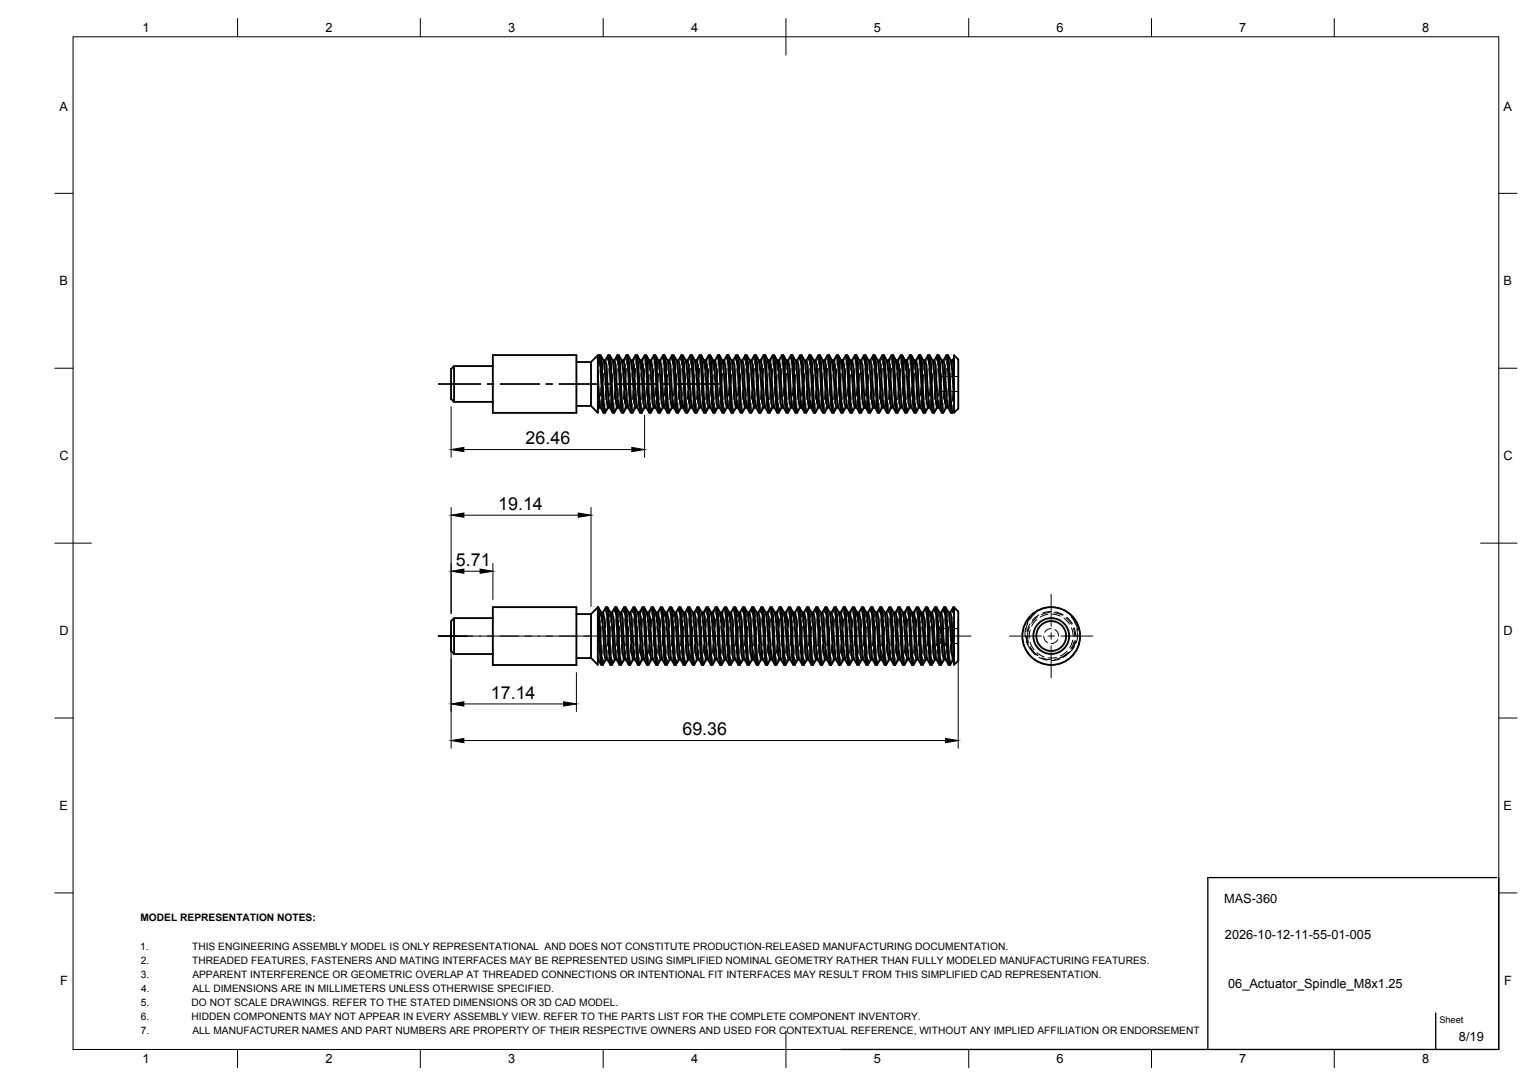
ISO-10303-21;
HEADER;
/* Generated by software containing ST-Developer
 * from STEP Tools, Inc. (www.steptools.com) 
 */

FILE_DESCRIPTION(
/* description */ (''),
/* implementation_level */ '2;1');

FILE_NAME(
/* name */ '06_Actuator_Spindle_M8x1.25.step',
/* time_stamp */ '2026-11-04T18:53:29-08:00',
/* author */ (''),
/* organization */ (''),
/* preprocessor_version */ 'ST-DEVELOPER v20.2',
/* originating_system */ 'Autodesk Translation Framework v15.17.0.0',
/* authorisation */ '');

FILE_SCHEMA (('AUTOMOTIVE_DESIGN { 1 0 10303 214 3 1 1 }'));
ENDSEC;

DATA;
#10=MECHANICAL_DESIGN_GEOMETRIC_PRESENTATION_REPRESENTATION('',(#1332),#100031);
#232=CONICAL_SURFACE('',#21595,3.6736,0.785398163397448);
#233=CONICAL_SURFACE('',#21596,3.5,0.78539816339745);
#234=CONICAL_SURFACE('',#21608,2.244,0.785398163397449);
#784=CIRCLE('',#21539,3.22275);
#785=CIRCLE('',#21579,3.933);
#786=CIRCLE('',#21580,3.933);
#787=CIRCLE('',#21582,3.22275);
#788=CIRCLE('',#21584,1.02);
#789=CIRCLE('',#21585,1.02);
#790=CIRCLE('',#21588,3.933);
#791=CIRCLE('',#21589,3.933);
#792=CIRCLE('',#21591,3.933);
#793=CIRCLE('',#21592,3.933);
#794=CIRCLE('',#21594,3.3472);
#795=CIRCLE('',#21597,3.);
#796=CIRCLE('',#21599,3.);
#797=CIRCLE('',#21601,3.95);
#798=CIRCLE('',#21603,3.95);
#799=CIRCLE('',#21605,2.448);
#800=CIRCLE('',#21607,2.448);
#801=CIRCLE('',#21609,2.04);
#1296=SHAPE_REPRESENTATION_RELATIONSHIP('SRR','None',#100106,#1314);
#1314=ADVANCED_BREP_SHAPE_REPRESENTATION('',(#1350),#100018);
#1332=STYLED_ITEM('',(#100200),#1350);
#1350=MANIFOLD_SOLID_BREP('Body1',#20122);
#1522=PLANE('',#21586);
#1523=PLANE('',#21587);
#1524=PLANE('',#21590);
#1525=PLANE('',#21593);
#1526=PLANE('',#21600);
#1527=PLANE('',#21604);
#1528=PLANE('',#21610);
#1757=FACE_BOUND('',#6951,.T.);
#1758=FACE_BOUND('',#6956,.T.);
#1759=FACE_BOUND('',#6959,.T.);
#2740=LINE('',#61994,#4027);
#2741=LINE('',#62177,#4028);
#2742=LINE('',#62607,#4029);
#2743=LINE('',#63034,#4030);
#2744=LINE('',#63490,#4031);
#2745=LINE('',#63954,#4032);
#2746=LINE('',#64297,#4033);
#2747=LINE('',#64695,#4034);
#2748=LINE('',#65028,#4035);
#2749=LINE('',#65420,#4036);
#2750=LINE('',#65803,#4037);
#2751=LINE('',#66202,#4038);
#2752=LINE('',#66758,#4039);
#2753=LINE('',#67219,#4040);
#2754=LINE('',#67749,#4041);
#2755=LINE('',#68202,#4042);
#2756=LINE('',#68741,#4043);
#2757=LINE('',#69203,#4044);
#2758=LINE('',#69714,#4045);
#2759=LINE('',#70197,#4046);
#2760=LINE('',#70661,#4047);
#2761=LINE('',#71128,#4048);
#2762=LINE('',#71592,#4049);
#2763=LINE('',#72044,#4050);
#2764=LINE('',#72530,#4051);
#2765=LINE('',#72983,#4052);
#2766=LINE('',#73456,#4053);
#2767=LINE('',#73924,#4054);
#2768=LINE('',#74396,#4055);
#2769=LINE('',#74858,#4056);
#2770=LINE('',#75318,#4057);
#2771=LINE('',#75804,#4058);
#2772=LINE('',#76261,#4059);
#2773=LINE('',#76732,#4060);
#2774=LINE('',#77194,#4061);
#2775=LINE('',#77655,#4062);
#2776=LINE('',#78092,#4063);
#2777=LINE('',#78388,#4064);
#2778=LINE('',#78748,#4065);
#2779=LINE('',#88562,#4066);
#2780=LINE('',#90954,#4067);
#2781=LINE('',#90957,#4068);
#2782=LINE('',#90962,#4069);
#2783=LINE('',#90969,#4070);
#2784=LINE('',#90976,#4071);
#2785=LINE('',#90979,#4072);
#4027=VECTOR('',#25695,3.22275);
#4028=VECTOR('',#25700,3.22275);
#4029=VECTOR('',#25703,3.22275);
#4030=VECTOR('',#25706,3.22275);
#4031=VECTOR('',#25709,3.22275);
#4032=VECTOR('',#25712,3.22275);
#4033=VECTOR('',#25715,3.22275);
#4034=VECTOR('',#25718,3.22275);
#4035=VECTOR('',#25721,3.22275);
#4036=VECTOR('',#25724,3.22275);
#4037=VECTOR('',#25727,3.22275);
#4038=VECTOR('',#25730,3.22275);
#4039=VECTOR('',#25733,3.22275);
#4040=VECTOR('',#25736,3.22275);
#4041=VECTOR('',#25739,3.22275);
#4042=VECTOR('',#25742,3.22275);
#4043=VECTOR('',#25745,3.22275);
#4044=VECTOR('',#25748,3.22275);
#4045=VECTOR('',#25751,3.22275);
#4046=VECTOR('',#25754,3.22275);
#4047=VECTOR('',#25757,3.22275);
#4048=VECTOR('',#25760,3.22275);
#4049=VECTOR('',#25763,3.22275);
#4050=VECTOR('',#25766,3.22275);
#4051=VECTOR('',#25769,3.22275);
#4052=VECTOR('',#25772,3.22275);
#4053=VECTOR('',#25775,3.22275);
#4054=VECTOR('',#25778,3.22275);
#4055=VECTOR('',#25781,3.22275);
#4056=VECTOR('',#25784,3.22275);
#4057=VECTOR('',#25787,3.22275);
#4058=VECTOR('',#25790,3.22275);
#4059=VECTOR('',#25793,3.22275);
#4060=VECTOR('',#25796,3.22275);
#4061=VECTOR('',#25799,3.22275);
#4062=VECTOR('',#25802,3.22275);
#4063=VECTOR('',#25805,3.22275);
#4064=VECTOR('',#25808,3.22275);
#4065=VECTOR('',#25811,3.22275);
#4066=VECTOR('',#25826,1.02);
#4067=VECTOR('',#25849,3.6736);
#4068=VECTOR('',#25852,3.5);
#4069=VECTOR('',#25859,3.);
#4070=VECTOR('',#25868,3.95);
#4071=VECTOR('',#25877,2.448);
#4072=VECTOR('',#25880,2.244);
#4817=CYLINDRICAL_SURFACE('',#21538,3.22275);
#4818=CYLINDRICAL_SURFACE('',#21540,3.22275);
#4819=CYLINDRICAL_SURFACE('',#21541,3.22275);
#4820=CYLINDRICAL_SURFACE('',#21542,3.22275);
#4821=CYLINDRICAL_SURFACE('',#21543,3.22275);
#4822=CYLINDRICAL_SURFACE('',#21544,3.22275);
#4823=CYLINDRICAL_SURFACE('',#21545,3.22275);
#4824=CYLINDRICAL_SURFACE('',#21546,3.22275);
#4825=CYLINDRICAL_SURFACE('',#21547,3.22275);
#4826=CYLINDRICAL_SURFACE('',#21548,3.22275);
#4827=CYLINDRICAL_SURFACE('',#21549,3.22275);
#4828=CYLINDRICAL_SURFACE('',#21550,3.22275);
#4829=CYLINDRICAL_SURFACE('',#21551,3.22275);
#4830=CYLINDRICAL_SURFACE('',#21552,3.22275);
#4831=CYLINDRICAL_SURFACE('',#21553,3.22275);
#4832=CYLINDRICAL_SURFACE('',#21554,3.22275);
#4833=CYLINDRICAL_SURFACE('',#21555,3.22275);
#4834=CYLINDRICAL_SURFACE('',#21556,3.22275);
#4835=CYLINDRICAL_SURFACE('',#21557,3.22275);
#4836=CYLINDRICAL_SURFACE('',#21558,3.22275);
#4837=CYLINDRICAL_SURFACE('',#21559,3.22275);
#4838=CYLINDRICAL_SURFACE('',#21560,3.22275);
#4839=CYLINDRICAL_SURFACE('',#21561,3.22275);
#4840=CYLINDRICAL_SURFACE('',#21562,3.22275);
#4841=CYLINDRICAL_SURFACE('',#21563,3.22275);
#4842=CYLINDRICAL_SURFACE('',#21564,3.22275);
#4843=CYLINDRICAL_SURFACE('',#21565,3.22275);
#4844=CYLINDRICAL_SURFACE('',#21566,3.22275);
#4845=CYLINDRICAL_SURFACE('',#21567,3.22275);
#4846=CYLINDRICAL_SURFACE('',#21568,3.22275);
#4847=CYLINDRICAL_SURFACE('',#21569,3.22275);
#4848=CYLINDRICAL_SURFACE('',#21570,3.22275);
#4849=CYLINDRICAL_SURFACE('',#21571,3.22275);
#4850=CYLINDRICAL_SURFACE('',#21572,3.22275);
#4851=CYLINDRICAL_SURFACE('',#21573,3.22275);
#4852=CYLINDRICAL_SURFACE('',#21574,3.22275);
#4853=CYLINDRICAL_SURFACE('',#21575,3.22275);
#4854=CYLINDRICAL_SURFACE('',#21576,3.22275);
#4855=CYLINDRICAL_SURFACE('',#21577,3.22275);
#4856=CYLINDRICAL_SURFACE('',#21578,3.933);
#4857=CYLINDRICAL_SURFACE('',#21581,3.22275);
#4858=CYLINDRICAL_SURFACE('',#21583,1.02);
#4859=CYLINDRICAL_SURFACE('',#21598,3.);
#4860=CYLINDRICAL_SURFACE('',#21602,3.95);
#4861=CYLINDRICAL_SURFACE('',#21606,2.448);
#5683=FACE_OUTER_BOUND('',#6903,.T.);
#5684=FACE_OUTER_BOUND('',#6904,.T.);
#5685=FACE_OUTER_BOUND('',#6905,.T.);
#5686=FACE_OUTER_BOUND('',#6906,.T.);
#5687=FACE_OUTER_BOUND('',#6907,.T.);
#5688=FACE_OUTER_BOUND('',#6908,.T.);
#5689=FACE_OUTER_BOUND('',#6909,.T.);
#5690=FACE_OUTER_BOUND('',#6910,.T.);
#5691=FACE_OUTER_BOUND('',#6911,.T.);
#5692=FACE_OUTER_BOUND('',#6912,.T.);
#5693=FACE_OUTER_BOUND('',#6913,.T.);
#5694=FACE_OUTER_BOUND('',#6914,.T.);
#5695=FACE_OUTER_BOUND('',#6915,.T.);
#5696=FACE_OUTER_BOUND('',#6916,.T.);
#5697=FACE_OUTER_BOUND('',#6917,.T.);
#5698=FACE_OUTER_BOUND('',#6918,.T.);
#5699=FACE_OUTER_BOUND('',#6919,.T.);
#5700=FACE_OUTER_BOUND('',#6920,.T.);
#5701=FACE_OUTER_BOUND('',#6921,.T.);
#5702=FACE_OUTER_BOUND('',#6922,.T.);
#5703=FACE_OUTER_BOUND('',#6923,.T.);
#5704=FACE_OUTER_BOUND('',#6924,.T.);
#5705=FACE_OUTER_BOUND('',#6925,.T.);
#5706=FACE_OUTER_BOUND('',#6926,.T.);
#5707=FACE_OUTER_BOUND('',#6927,.T.);
#5708=FACE_OUTER_BOUND('',#6928,.T.);
#5709=FACE_OUTER_BOUND('',#6929,.T.);
#5710=FACE_OUTER_BOUND('',#6930,.T.);
#5711=FACE_OUTER_BOUND('',#6931,.T.);
#5712=FACE_OUTER_BOUND('',#6932,.T.);
#5713=FACE_OUTER_BOUND('',#6933,.T.);
#5714=FACE_OUTER_BOUND('',#6934,.T.);
#5715=FACE_OUTER_BOUND('',#6935,.T.);
#5716=FACE_OUTER_BOUND('',#6936,.T.);
#5717=FACE_OUTER_BOUND('',#6937,.T.);
#5718=FACE_OUTER_BOUND('',#6938,.T.);
#5719=FACE_OUTER_BOUND('',#6939,.T.);
#5720=FACE_OUTER_BOUND('',#6940,.T.);
#5721=FACE_OUTER_BOUND('',#6941,.T.);
#5722=FACE_OUTER_BOUND('',#6942,.T.);
#5723=FACE_OUTER_BOUND('',#6943,.T.);
#5724=FACE_OUTER_BOUND('',#6944,.T.);
#5725=FACE_OUTER_BOUND('',#6945,.T.);
#5726=FACE_OUTER_BOUND('',#6946,.T.);
#5727=FACE_OUTER_BOUND('',#6947,.T.);
#5728=FACE_OUTER_BOUND('',#6948,.T.);
#5729=FACE_OUTER_BOUND('',#6949,.T.);
#5730=FACE_OUTER_BOUND('',#6950,.T.);
#5731=FACE_OUTER_BOUND('',#6952,.T.);
#5732=FACE_OUTER_BOUND('',#6953,.T.);
#5733=FACE_OUTER_BOUND('',#6954,.T.);
#5734=FACE_OUTER_BOUND('',#6955,.T.);
#5735=FACE_OUTER_BOUND('',#6957,.T.);
#5736=FACE_OUTER_BOUND('',#6958,.T.);
#5737=FACE_OUTER_BOUND('',#6960,.T.);
#5738=FACE_OUTER_BOUND('',#6961,.T.);
#5739=FACE_OUTER_BOUND('',#6962,.T.);
#6903=EDGE_LOOP('',(#16151,#16152,#16153,#16154));
#6904=EDGE_LOOP('',(#16155,#16156,#16157,#16158,#16159,#16160));
#6905=EDGE_LOOP('',(#16161,#16162,#16163,#16164,#16165,#16166));
#6906=EDGE_LOOP('',(#16167,#16168,#16169,#16170,#16171,#16172));
#6907=EDGE_LOOP('',(#16173,#16174,#16175,#16176,#16177));
#6908=EDGE_LOOP('',(#16178,#16179,#16180,#16181,#16182,#16183));
#6909=EDGE_LOOP('',(#16184,#16185,#16186,#16187,#16188));
#6910=EDGE_LOOP('',(#16189,#16190,#16191,#16192,#16193,#16194));
#6911=EDGE_LOOP('',(#16195,#16196,#16197,#16198,#16199));
#6912=EDGE_LOOP('',(#16200,#16201,#16202,#16203,#16204,#16205));
#6913=EDGE_LOOP('',(#16206,#16207,#16208,#16209,#16210));
#6914=EDGE_LOOP('',(#16211,#16212,#16213,#16214,#16215,#16216));
#6915=EDGE_LOOP('',(#16217,#16218,#16219,#16220,#16221));
#6916=EDGE_LOOP('',(#16222,#16223,#16224,#16225,#16226,#16227));
#6917=EDGE_LOOP('',(#16228,#16229,#16230,#16231,#16232));
#6918=EDGE_LOOP('',(#16233,#16234,#16235,#16236,#16237,#16238));
#6919=EDGE_LOOP('',(#16239,#16240,#16241,#16242,#16243));
#6920=EDGE_LOOP('',(#16244,#16245,#16246,#16247,#16248,#16249));
#6921=EDGE_LOOP('',(#16250,#16251,#16252,#16253,#16254));
#6922=EDGE_LOOP('',(#16255,#16256,#16257,#16258,#16259,#16260));
#6923=EDGE_LOOP('',(#16261,#16262,#16263,#16264,#16265));
#6924=EDGE_LOOP('',(#16266,#16267,#16268,#16269,#16270,#16271));
#6925=EDGE_LOOP('',(#16272,#16273,#16274,#16275,#16276));
#6926=EDGE_LOOP('',(#16277,#16278,#16279,#16280,#16281,#16282));
#6927=EDGE_LOOP('',(#16283,#16284,#16285,#16286,#16287,#16288));
#6928=EDGE_LOOP('',(#16289,#16290,#16291,#16292,#16293));
#6929=EDGE_LOOP('',(#16294,#16295,#16296,#16297,#16298,#16299));
#6930=EDGE_LOOP('',(#16300,#16301,#16302,#16303,#16304));
#6931=EDGE_LOOP('',(#16305,#16306,#16307,#16308,#16309,#16310));
#6932=EDGE_LOOP('',(#16311,#16312,#16313,#16314,#16315));
#6933=EDGE_LOOP('',(#16316,#16317,#16318,#16319,#16320,#16321));
#6934=EDGE_LOOP('',(#16322,#16323,#16324,#16325,#16326,#16327));
#6935=EDGE_LOOP('',(#16328,#16329,#16330,#16331,#16332));
#6936=EDGE_LOOP('',(#16333,#16334,#16335,#16336,#16337,#16338));
#6937=EDGE_LOOP('',(#16339,#16340,#16341,#16342,#16343));
#6938=EDGE_LOOP('',(#16344,#16345,#16346,#16347,#16348,#16349));
#6939=EDGE_LOOP('',(#16350,#16351,#16352,#16353,#16354,#16355));
#6940=EDGE_LOOP('',(#16356,#16357,#16358,#16359,#16360,#16361));
#6941=EDGE_LOOP('',(#16362,#16363,#16364,#16365,#16366,#16367));
#6942=EDGE_LOOP('',(#16368,#16369,#16370,#16371,#16372,#16373,#16374,#16375,
#16376,#16377,#16378,#16379,#16380,#16381,#16382,#16383,#16384,#16385,#16386,
#16387,#16388,#16389,#16390,#16391,#16392,#16393,#16394,#16395,#16396,#16397,
#16398,#16399,#16400,#16401,#16402,#16403,#16404,#16405,#16406,#16407,#16408,
#16409,#16410,#16411,#16412,#16413,#16414,#16415,#16416,#16417,#16418,#16419,
#16420,#16421,#16422,#16423,#16424,#16425,#16426,#16427,#16428,#16429,#16430,
#16431,#16432,#16433,#16434,#16435,#16436,#16437,#16438,#16439,#16440,#16441,
#16442,#16443,#16444,#16445,#16446,#16447,#16448,#16449));
#6943=EDGE_LOOP('',(#16450,#16451,#16452,#16453,#16454,#16455));
#6944=EDGE_LOOP('',(#16456,#16457,#16458,#16459));
#6945=EDGE_LOOP('',(#16460));
#6946=EDGE_LOOP('',(#16461,#16462,#16463,#16464,#16465));
#6947=EDGE_LOOP('',(#16466,#16467,#16468,#16469,#16470,#16471,#16472,#16473,
#16474,#16475,#16476,#16477,#16478,#16479,#16480,#16481,#16482,#16483,#16484,
#16485,#16486,#16487,#16488,#16489,#16490,#16491,#16492,#16493,#16494,#16495,
#16496,#16497,#16498,#16499,#16500,#16501,#16502,#16503,#16504,#16505,#16506,
#16507,#16508,#16509,#16510,#16511,#16512,#16513,#16514,#16515,#16516,#16517,
#16518,#16519,#16520,#16521,#16522,#16523,#16524,#16525,#16526,#16527,#16528,
#16529,#16530,#16531,#16532,#16533,#16534,#16535,#16536,#16537,#16538,#16539,
#16540,#16541,#16542,#16543,#16544,#16545,#16546,#16547,#16548,#16549,#16550,
#16551,#16552,#16553,#16554,#16555,#16556,#16557,#16558,#16559,#16560,#16561,
#16562,#16563,#16564,#16565,#16566,#16567,#16568,#16569,#16570,#16571,#16572,
#16573,#16574,#16575,#16576,#16577,#16578,#16579,#16580,#16581,#16582,#16583,
#16584,#16585,#16586,#16587));
#6948=EDGE_LOOP('',(#16588,#16589,#16590,#16591,#16592));
#6949=EDGE_LOOP('',(#16593,#16594,#16595,#16596,#16597,#16598,#16599,#16600,
#16601,#16602,#16603,#16604,#16605,#16606,#16607,#16608,#16609,#16610,#16611,
#16612,#16613,#16614,#16615,#16616,#16617,#16618,#16619,#16620,#16621,#16622,
#16623,#16624,#16625,#16626,#16627,#16628,#16629,#16630,#16631,#16632,#16633,
#16634,#16635,#16636,#16637,#16638,#16639,#16640,#16641,#16642,#16643,#16644,
#16645,#16646,#16647,#16648,#16649,#16650,#16651,#16652,#16653,#16654,#16655,
#16656,#16657,#16658,#16659,#16660,#16661,#16662,#16663,#16664,#16665,#16666,
#16667,#16668,#16669,#16670,#16671,#16672,#16673,#16674,#16675,#16676,#16677,
#16678,#16679,#16680,#16681,#16682,#16683,#16684,#16685,#16686,#16687,#16688,
#16689,#16690,#16691,#16692,#16693,#16694,#16695,#16696,#16697,#16698,#16699));
#6950=EDGE_LOOP('',(#16700));
#6951=EDGE_LOOP('',(#16701));
#6952=EDGE_LOOP('',(#16702,#16703,#16704,#16705,#16706,#16707,#16708));
#6953=EDGE_LOOP('',(#16709,#16710,#16711,#16712,#16713,#16714,#16715));
#6954=EDGE_LOOP('',(#16716,#16717,#16718,#16719));
#6955=EDGE_LOOP('',(#16720));
#6956=EDGE_LOOP('',(#16721));
#6957=EDGE_LOOP('',(#16722,#16723,#16724,#16725));
#6958=EDGE_LOOP('',(#16726));
#6959=EDGE_LOOP('',(#16727));
#6960=EDGE_LOOP('',(#16728,#16729,#16730,#16731));
#6961=EDGE_LOOP('',(#16732,#16733,#16734,#16735));
#6962=EDGE_LOOP('',(#16736));
#7699=B_SPLINE_CURVE_WITH_KNOTS('',3,(#61996,#61997,#61998,#61999,#62000,
#62001,#62002,#62003,#62004,#62005,#62006,#62007,#62008,#62009,#62010,#62011,
#62012,#62013,#62014,#62015,#62016,#62017,#62018,#62019,#62020,#62021,#62022,
#62023,#62024,#62025,#62026,#62027,#62028,#62029,#62030,#62031,#62032,#62033,
#62034,#62035,#62036,#62037,#62038,#62039,#62040,#62041,#62042,#62043,#62044,
#62045,#62046,#62047,#62048,#62049,#62050,#62051,#62052,#62053,#62054,#62055,
#62056,#62057,#62058,#62059,#62060,#62061,#62062,#62063,#62064,#62065,#62066,
#62067,#62068,#62069,#62070,#62071,#62072,#62073,#62074,#62075,#62076,#62077,
#62078,#62079,#62080,#62081,#62082,#62083,#62084,#62085,#62086,#62087,#62088,
#62089,#62090,#62091,#62092,#62093,#62094,#62095,#62096,#62097,#62098,#62099,
#62100,#62101,#62102,#62103,#62104),.UNSPECIFIED.,.F.,.F.,(4,3,3,3,3,3,
3,3,3,3,3,3,3,3,3,3,3,3,3,3,3,3,3,3,3,3,3,3,3,3,3,3,3,3,3,3,4),(10.3762744482256,
10.4685616448508,10.5607276261043,10.6547964435211,10.7468093354631,10.8387943991844,
10.9307772613786,11.0264024873936,11.1185108557443,11.2106815902354,11.3029864495802,
11.3132781654386,11.4065164375908,11.4996317690644,11.5926515496584,11.6856071336555,
11.7785297343733,11.8714439672823,11.9643744342891,12.0574057190744,12.15049000187,
12.2437296619365,12.3127933039653,12.4057444841292,12.4985679912201,12.5912916301099,
12.6839457888757,12.7765638151076,12.8691706791047,12.9617913353808,13.0545109207409,
13.1472819693773,13.2402091284387,13.3123084424921,13.4054129193392,13.4983783998293,
13.5490822577306),.UNSPECIFIED.);
#7700=B_SPLINE_CURVE_WITH_KNOTS('',3,(#62107,#62108,#62109,#62110,#62111,
#62112,#62113,#62114,#62115,#62116,#62117,#62118,#62119,#62120,#62121,#62122,
#62123,#62124,#62125,#62126,#62127,#62128,#62129,#62130,#62131,#62132,#62133,
#62134,#62135,#62136,#62137,#62138,#62139,#62140,#62141,#62142,#62143,#62144,
#62145,#62146,#62147,#62148,#62149,#62150,#62151,#62152,#62153,#62154,#62155,
#62156,#62157,#62158,#62159,#62160,#62161,#62162,#62163,#62164,#62165,#62166,
#62167,#62168,#62169,#62170,#62171,#62172,#62173),.UNSPECIFIED.,.F.,.F.,
(4,3,3,3,3,3,3,3,3,3,3,3,3,3,3,3,3,3,3,3,3,3,4),(11.6152142277551,11.7104709514056,
11.805672798299,11.9008419087062,11.9960272735159,12.0912269901345,12.186461164303,
12.2817499296462,12.3771800378493,12.472688391674,12.5683655133993,12.6147293662818,
12.7068652367845,12.7988611340536,12.8925181866135,12.9843156369482,13.0760684890777,
13.1678025610073,13.2628813093886,13.3547002092736,13.4465675973497,13.5385499644351,
13.5481175545326),.UNSPECIFIED.);
#7701=B_SPLINE_CURVE_WITH_KNOTS('',3,(#62179,#62180,#62181,#62182,#62183,
#62184,#62185,#62186,#62187,#62188,#62189,#62190,#62191,#62192,#62193,#62194,
#62195,#62196,#62197,#62198,#62199,#62200,#62201,#62202,#62203,#62204,#62205,
#62206,#62207,#62208,#62209,#62210,#62211,#62212,#62213,#62214,#62215,#62216,
#62217,#62218,#62219,#62220,#62221,#62222,#62223,#62224,#62225,#62226,#62227,
#62228,#62229,#62230,#62231,#62232,#62233,#62234,#62235,#62236,#62237,#62238,
#62239,#62240,#62241,#62242,#62243,#62244,#62245,#62246,#62247,#62248,#62249,
#62250,#62251,#62252,#62253,#62254,#62255,#62256,#62257,#62258,#62259,#62260,
#62261,#62262,#62263,#62264,#62265,#62266,#62267,#62268,#62269,#62270,#62271,
#62272,#62273,#62274,#62275,#62276,#62277,#62278,#62279,#62280,#62281,#62282,
#62283,#62284,#62285,#62286,#62287,#62288,#62289,#62290,#62291,#62292,#62293,
#62294,#62295,#62296,#62297,#62298,#62299,#62300,#62301,#62302,#62303,#62304,
#62305,#62306,#62307,#62308,#62309,#62310,#62311,#62312,#62313,#62314,#62315,
#62316,#62317),.UNSPECIFIED.,.F.,.F.,(4,3,3,3,3,3,3,3,3,3,3,3,3,3,3,3,3,
3,3,3,3,3,3,3,3,3,3,3,3,3,3,3,3,3,3,3,3,3,3,3,3,3,3,3,3,3,4),(15.7079632679493,
15.801862704237,15.8957881015399,15.9897621227233,16.0838725098807,16.1780606852298,
16.2724168889073,16.3108538580724,16.403934049719,16.4968882171655,16.5897439863011,
16.6825319537682,16.775284780659,16.8680272835037,16.9607842637073,17.053640404213,
17.1465483531614,17.2396115558221,17.3103689965991,17.403446464583,17.4963979243741,
17.5892510054323,17.6820363258165,17.7747865316696,17.8675264427482,17.9602808637086,
18.0531345118179,18.1460400015679,18.2391008256502,18.3098841351259,18.4029568890223,
18.495903548684,18.5887517503804,18.6815320919292,18.7742772593972,18.8670120783317,
18.9597613591359,19.0526098238704,19.1455100981482,19.2385657080346,19.3093992736527,
19.4024726918571,19.4954250802269,19.5882679505022,19.681046896648,19.7737939705685,
19.8316169097465),.UNSPECIFIED.);
#7702=B_SPLINE_CURVE_WITH_KNOTS('',3,(#62318,#62319,#62320,#62321,#62322,
#62323,#62324,#62325,#62326,#62327,#62328,#62329,#62330,#62331,#62332,#62333,
#62334,#62335,#62336,#62337,#62338,#62339,#62340,#62341,#62342,#62343,#62344,
#62345,#62346,#62347,#62348,#62349,#62350,#62351,#62352,#62353,#62354,#62355,
#62356,#62357,#62358,#62359,#62360,#62361,#62362,#62363,#62364,#62365,#62366,
#62367,#62368,#62369,#62370,#62371,#62372,#62373,#62374,#62375,#62376,#62377,
#62378,#62379,#62380,#62381,#62382,#62383,#62384,#62385,#62386,#62387,#62388,
#62389,#62390),.UNSPECIFIED.,.F.,.F.,(4,3,3,3,3,3,3,3,3,3,3,3,3,3,3,3,3,
3,3,3,3,3,3,3,4),(13.5490822577306,13.6444249231416,13.7372107374818,13.8299755857438,
13.9227442480459,14.0200140812891,14.1129202918713,14.20589203575,14.2990021749612,
14.3118235810189,14.4049182756249,14.4978873068571,14.5907582790323,14.6835618991959,
14.7763306500945,14.8690893301786,14.9618627229779,15.054735542364,15.1476603440171,
15.2407405112384,15.3113387195456,15.4149720236937,15.5182945666206,15.6210595353514,
15.7079632677657),.UNSPECIFIED.);
#7703=B_SPLINE_CURVE_WITH_KNOTS('',3,(#62392,#62393,#62394,#62395,#62396,
#62397,#62398,#62399,#62400,#62401,#62402,#62403,#62404,#62405,#62406,#62407,
#62408,#62409,#62410,#62411,#62412,#62413,#62414,#62415,#62416,#62417,#62418,
#62419,#62420,#62421,#62422,#62423,#62424,#62425,#62426,#62427,#62428,#62429,
#62430,#62431,#62432,#62433,#62434,#62435,#62436,#62437,#62438,#62439,#62440,
#62441,#62442,#62443,#62444,#62445,#62446,#62447,#62448,#62449,#62450,#62451,
#62452,#62453,#62454,#62455,#62456,#62457,#62458,#62459,#62460,#62461,#62462,
#62463,#62464),.UNSPECIFIED.,.F.,.F.,(4,3,3,3,3,3,3,3,3,3,3,3,3,3,3,3,3,
3,3,3,3,3,3,3,4),(13.5481175545326,13.6142445048086,13.7074539898319,13.8005374759601,
13.8935224081086,13.9864387418312,14.079319398333,14.1721890329815,14.2650722854203,
14.358052555288,14.4510836331598,14.5442670228022,14.6137596433353,14.7069979410332,
14.8001132987202,14.8931331061577,14.9860887178402,15.0790113467516,15.1719256083309,
15.264856104453,15.357887418871,15.4509717316316,15.5442114219034,15.6132747818621,
15.7079632679492),.UNSPECIFIED.);
#7704=B_SPLINE_CURVE_WITH_KNOTS('',3,(#62465,#62466,#62467,#62468,#62469,
#62470,#62471,#62472,#62473,#62474,#62475,#62476,#62477,#62478,#62479,#62480,
#62481,#62482,#62483,#62484,#62485,#62486,#62487,#62488,#62489,#62490,#62491,
#62492,#62493,#62494,#62495,#62496,#62497,#62498,#62499,#62500,#62501,#62502,
#62503,#62504,#62505,#62506,#62507,#62508,#62509,#62510,#62511,#62512,#62513,
#62514,#62515,#62516,#62517,#62518,#62519,#62520,#62521,#62522,#62523,#62524,
#62525,#62526,#62527,#62528,#62529,#62530,#62531,#62532,#62533,#62534,#62535,
#62536,#62537,#62538,#62539,#62540,#62541,#62542,#62543,#62544,#62545,#62546,
#62547,#62548,#62549,#62550,#62551,#62552,#62553,#62554,#62555,#62556,#62557,
#62558,#62559,#62560,#62561,#62562,#62563,#62564,#62565,#62566,#62567,#62568,
#62569,#62570,#62571,#62572,#62573,#62574,#62575,#62576,#62577,#62578,#62579,
#62580,#62581,#62582,#62583,#62584,#62585,#62586,#62587,#62588,#62589,#62590,
#62591,#62592,#62593,#62594,#62595,#62596,#62597,#62598,#62599,#62600,#62601,
#62602,#62603),.UNSPECIFIED.,.F.,.F.,(4,3,3,3,3,3,3,3,3,3,3,3,3,3,3,3,3,
3,3,3,3,3,3,3,3,3,3,3,3,3,3,3,3,3,3,3,3,3,3,3,3,3,3,3,3,3,4),(15.7079632682196,
15.7997431632769,15.8914080252224,15.9829843740528,16.0745131018752,16.1660202549873,
16.2575318536328,16.3491336017902,16.4407804137139,16.5325825781659,16.6127899203889,
16.7058910985793,16.7988663175293,16.8917431744402,16.984552195471,17.0773260480196,
17.1700895232903,17.2628673973129,17.3557441784495,17.4486726596649,17.5417560010965,
17.6123050589156,17.7053997604146,17.7983687987123,17.8912397781156,17.9840434057244,
18.076812164199,18.1695708519817,18.262344252594,18.3552170799245,18.448141889607,
18.5412220649159,18.6118201974424,18.7048774940281,18.7978084850565,18.890640828656,
18.9834050917185,19.0761340503132,19.1688525487697,19.2615854161865,19.354417423974,
19.4473011913083,19.5403403836925,19.6113353359692,19.7044230626322,19.7973722083033,
19.8322838807155),.UNSPECIFIED.);
#7705=B_SPLINE_CURVE_WITH_KNOTS('',3,(#62609,#62610,#62611,#62612,#62613,
#62614,#62615,#62616,#62617,#62618,#62619,#62620,#62621,#62622,#62623,#62624,
#62625,#62626,#62627,#62628,#62629,#62630,#62631,#62632,#62633,#62634,#62635,
#62636,#62637,#62638,#62639,#62640,#62641,#62642,#62643,#62644,#62645,#62646,
#62647,#62648,#62649,#62650,#62651,#62652,#62653,#62654,#62655,#62656,#62657,
#62658,#62659,#62660,#62661,#62662,#62663,#62664,#62665,#62666,#62667,#62668,
#62669,#62670,#62671,#62672,#62673,#62674,#62675,#62676,#62677,#62678,#62679,
#62680,#62681,#62682,#62683,#62684,#62685,#62686,#62687,#62688,#62689,#62690,
#62691,#62692,#62693,#62694,#62695,#62696,#62697,#62698,#62699,#62700,#62701,
#62702,#62703,#62704,#62705,#62706,#62707,#62708,#62709,#62710,#62711,#62712,
#62713,#62714,#62715,#62716,#62717,#62718,#62719,#62720,#62721,#62722,#62723,
#62724,#62725,#62726,#62727,#62728,#62729,#62730,#62731,#62732,#62733,#62734,
#62735,#62736,#62737,#62738,#62739,#62740,#62741,#62742,#62743,#62744),
 .UNSPECIFIED.,.F.,.F.,(4,3,3,3,3,3,3,3,3,3,3,3,3,3,3,3,3,3,3,3,3,3,3,3,
3,3,3,3,3,3,3,3,3,3,3,3,3,3,3,3,3,3,3,3,3,4),(21.9911485752977,22.1009390578722,
22.2120192264695,22.307944689233,22.4010201395792,22.4939695339534,22.5868205047926,
22.67960365598,22.7723516570805,22.8650893303511,22.9578414829215,23.0506928288605,
23.1435959940919,23.2366544809095,23.3074598277597,23.4005351530306,23.4934844215758,
23.5863352660045,23.679118290433,23.7718661646011,23.8646037109164,23.9573557366592,
24.0502069567598,24.1431099965046,24.2361683597274,24.3069749662865,24.4000502264934,
24.4929994285521,24.585850205167,24.6786331600566,24.7713809636478,24.8641184384285,
24.9568703917587,25.049721538522,25.1426245043015,25.2356827932911,25.3064901048132,
25.3995782757944,25.4925102707237,25.5853528984435,25.6781310827416,25.7708696868248,
25.8636232533134,25.9563823167374,26.0492200497298,26.1142762800646),
 .UNSPECIFIED.);
#7706=B_SPLINE_CURVE_WITH_KNOTS('',3,(#62745,#62746,#62747,#62748,#62749,
#62750,#62751,#62752,#62753,#62754,#62755,#62756,#62757,#62758,#62759,#62760,
#62761,#62762,#62763,#62764,#62765,#62766,#62767,#62768,#62769,#62770,#62771,
#62772,#62773,#62774,#62775,#62776,#62777,#62778,#62779,#62780,#62781,#62782,
#62783,#62784,#62785,#62786,#62787,#62788,#62789,#62790,#62791,#62792,#62793,
#62794,#62795,#62796,#62797,#62798,#62799,#62800,#62801,#62802,#62803,#62804,
#62805,#62806,#62807,#62808,#62809,#62810,#62811,#62812,#62813,#62814,#62815,
#62816,#62817),.UNSPECIFIED.,.F.,.F.,(4,3,3,3,3,3,3,3,3,3,3,3,3,3,3,3,3,
3,3,3,3,3,3,3,4),(19.8316169097465,19.9243614290183,20.0204996748086,20.1133834001034,
20.2111489061414,20.3089144121794,20.4019899358734,20.4949394080688,20.5877904610795,
20.6805737006823,20.7733217940077,20.8660595632167,20.9588118153459,21.0516632658938,
21.1445665387003,21.2376251368815,21.3084295507062,21.4011773356687,21.4938045011336,
21.5863363897949,21.67879825315,21.7712257642586,21.8636335735842,21.9560698252548,
21.9911485751289),.UNSPECIFIED.);
#7707=B_SPLINE_CURVE_WITH_KNOTS('',3,(#62819,#62820,#62821,#62822,#62823,
#62824,#62825,#62826,#62827,#62828,#62829,#62830,#62831,#62832,#62833,#62834,
#62835,#62836,#62837,#62838,#62839,#62840,#62841,#62842,#62843,#62844,#62845,
#62846,#62847,#62848,#62849,#62850,#62851,#62852,#62853,#62854,#62855,#62856,
#62857,#62858,#62859,#62860,#62861,#62862,#62863,#62864,#62865,#62866,#62867,
#62868,#62869,#62870,#62871,#62872,#62873,#62874,#62875,#62876,#62877,#62878,
#62879,#62880,#62881,#62882,#62883,#62884,#62885,#62886,#62887,#62888,#62889,
#62890,#62891),.UNSPECIFIED.,.F.,.F.,(4,3,3,3,3,3,3,3,3,3,3,3,3,3,3,3,3,
3,3,3,3,3,3,3,4),(19.8322838807155,19.9296047049381,20.0223747342139,20.1151201566221,
20.2078657798381,20.3006364048605,20.3935117970783,20.4864484588977,20.5795288783454,
20.6108504744959,20.7039279435914,20.796879404527,20.8897324867605,20.9825178083623,
21.0752680154586,21.1680079278048,21.2607623500554,21.353615999483,21.446521490569,
21.5395823160024,21.6103656130227,21.7152591306476,21.8197981287288,21.9237013079083,
21.9911485749378),.UNSPECIFIED.);
#7708=B_SPLINE_CURVE_WITH_KNOTS('',3,(#62892,#62893,#62894,#62895,#62896,
#62897,#62898,#62899,#62900,#62901,#62902,#62903,#62904,#62905,#62906,#62907,
#62908,#62909,#62910,#62911,#62912,#62913,#62914,#62915,#62916,#62917,#62918,
#62919,#62920,#62921,#62922,#62923,#62924,#62925,#62926,#62927,#62928,#62929,
#62930,#62931,#62932,#62933,#62934,#62935,#62936,#62937,#62938,#62939,#62940,
#62941,#62942,#62943,#62944,#62945,#62946,#62947,#62948,#62949,#62950,#62951,
#62952,#62953,#62954,#62955,#62956,#62957,#62958,#62959,#62960,#62961,#62962,
#62963,#62964,#62965,#62966,#62967,#62968,#62969,#62970,#62971,#62972,#62973,
#62974,#62975,#62976,#62977,#62978,#62979,#62980,#62981,#62982,#62983,#62984,
#62985,#62986,#62987,#62988,#62989,#62990,#62991,#62992,#62993,#62994,#62995,
#62996,#62997,#62998,#62999,#63000,#63001,#63002,#63003,#63004,#63005,#63006,
#63007,#63008,#63009,#63010,#63011,#63012,#63013,#63014,#63015,#63016,#63017,
#63018,#63019,#63020,#63021,#63022,#63023,#63024,#63025,#63026,#63027,#63028,
#63029,#63030),.UNSPECIFIED.,.F.,.F.,(4,3,3,3,3,3,3,3,3,3,3,3,3,3,3,3,3,
3,3,3,3,3,3,3,3,3,3,3,3,3,3,3,3,3,3,3,3,3,3,3,3,3,3,3,3,3,4),(21.9911485751288,
22.0847067914567,22.1782793405872,22.2718895786102,22.3656265377757,22.4594329192013,
22.5534084578545,22.6098807515494,22.7029569153201,22.7959070291147,22.8887587243788,
22.9815426045203,23.0742913371258,23.1670297435889,23.2597826301769,23.3526347068616,
23.4455386021667,23.5385978103277,23.6093958900762,23.702471413893,23.7954208862163,
23.8882719393601,23.9810551791027,24.0738032725722,24.1665410419292,24.2592932942106,
24.3521447449158,24.4450480178827,24.5381066162279,24.608911028603,24.7019859816036,
24.79493487186,24.8877853325149,24.9805679664762,25.0733154461881,25.166052594514,
25.2588042191871,25.3516550358887,25.4445576703103,25.5376156292532,25.6084261671297,
25.7015007924706,25.7944540138807,25.8872964718783,25.9800748558386,26.0728176554707,
26.1148515779882),.UNSPECIFIED.);
#7709=B_SPLINE_CURVE_WITH_KNOTS('',3,(#63036,#63037,#63038,#63039,#63040,
#63041,#63042,#63043,#63044,#63045,#63046,#63047,#63048,#63049,#63050,#63051,
#63052,#63053,#63054,#63055,#63056,#63057,#63058,#63059,#63060,#63061,#63062,
#63063,#63064,#63065,#63066,#63067,#63068,#63069,#63070,#63071,#63072,#63073,
#63074,#63075,#63076,#63077,#63078,#63079,#63080,#63081,#63082,#63083,#63084,
#63085,#63086,#63087,#63088,#63089,#63090,#63091,#63092,#63093,#63094,#63095,
#63096,#63097,#63098,#63099,#63100,#63101,#63102,#63103,#63104,#63105,#63106,
#63107,#63108,#63109,#63110,#63111,#63112,#63113,#63114,#63115,#63116,#63117,
#63118,#63119,#63120,#63121,#63122,#63123,#63124,#63125,#63126,#63127,#63128,
#63129,#63130,#63131,#63132,#63133,#63134,#63135,#63136,#63137,#63138,#63139,
#63140,#63141,#63142,#63143,#63144,#63145,#63146,#63147,#63148,#63149,#63150,
#63151,#63152,#63153,#63154,#63155,#63156,#63157,#63158,#63159,#63160,#63161,
#63162,#63163,#63164,#63165,#63166,#63167,#63168,#63169,#63170,#63171,#63172,
#63173,#63174),.UNSPECIFIED.,.F.,.F.,(4,3,3,3,3,3,3,3,3,3,3,3,3,3,3,3,3,
3,3,3,3,3,3,3,3,3,3,3,3,3,3,3,3,3,3,3,3,3,3,3,3,3,3,3,3,3,4),(28.2743338823085,
28.3050355203935,28.3981108323836,28.4910600870279,28.583910916957,28.6766939260394,
28.7694417843463,28.8621793143023,28.9549313232044,29.0477825258147,29.1406855476817,
29.2337438925711,29.3045506589203,29.3976259671484,29.4905752179945,29.5834260440944,
29.6762090493171,29.7689569037467,29.8616944298121,29.9544464348151,30.0472976335374,
30.1402006515163,30.2332589925582,30.3040657974471,30.3971411050901,30.4900903553313,
30.5829411808073,30.6757241853799,30.7684720391435,30.861209564528,30.9539615688355,
31.0468127668442,31.1397157840982,31.2327741244043,31.3035809359738,31.3966562449754,
31.4896054965963,31.5824563234711,31.6752393294658,31.7679871846652,31.8607247114976,
31.9534767172635,32.0463279167379,32.1392309354639,32.2322892772372,32.3030960745006,
32.398493560417),.UNSPECIFIED.);
#7710=B_SPLINE_CURVE_WITH_KNOTS('',3,(#63175,#63176,#63177,#63178,#63179,
#63180,#63181,#63182,#63183,#63184,#63185,#63186,#63187,#63188,#63189,#63190,
#63191,#63192,#63193,#63194,#63195,#63196,#63197,#63198,#63199,#63200,#63201,
#63202,#63203,#63204,#63205,#63206,#63207,#63208,#63209,#63210,#63211,#63212,
#63213,#63214,#63215,#63216,#63217,#63218,#63219,#63220,#63221,#63222,#63223,
#63224,#63225,#63226,#63227,#63228,#63229,#63230,#63231,#63232,#63233,#63234,
#63235,#63236,#63237,#63238,#63239,#63240,#63241,#63242,#63243,#63244,#63245,
#63246,#63247),.UNSPECIFIED.,.F.,.F.,(4,3,3,3,3,3,3,3,3,3,3,3,3,3,3,3,3,
3,3,3,3,3,3,3,4),(26.1142762800646,26.2101407617023,26.30600524334,26.3990805521692,
26.4920298036781,26.5848806305009,26.6776636365352,26.7704114918303,26.8631490188147,
26.9559010247892,27.048752224559,27.1416552436292,27.2347135858238,27.3055203818668,
27.398127088502,27.4906081096177,27.5829916645036,27.6753091644605,27.7675934136574,
27.8598697536049,27.9521635127291,28.0445556641859,28.137003309307,28.2295960455401,
28.2743338820371),.UNSPECIFIED.);
#7711=B_SPLINE_CURVE_WITH_KNOTS('',3,(#63249,#63250,#63251,#63252,#63253,
#63254,#63255,#63256,#63257,#63258,#63259,#63260,#63261,#63262,#63263,#63264,
#63265,#63266,#63267,#63268,#63269,#63270,#63271,#63272,#63273,#63274,#63275,
#63276,#63277,#63278,#63279,#63280,#63281,#63282,#63283,#63284,#63285,#63286,
#63287,#63288,#63289,#63290,#63291,#63292,#63293,#63294,#63295,#63296,#63297,
#63298,#63299,#63300,#63301,#63302,#63303,#63304,#63305,#63306,#63307,#63308,
#63309,#63310,#63311,#63312,#63313,#63314,#63315,#63316,#63317,#63318,#63319,
#63320,#63321,#63322,#63323,#63324),.UNSPECIFIED.,.F.,.F.,(4,3,3,3,3,3,
3,3,3,3,3,3,3,3,3,3,3,3,3,3,3,3,3,3,3,4),(26.1148515779882,26.2075927385225,
26.3003596186431,26.3932316639966,26.48616563344,26.5792426776218,26.6079413056565,
26.7010166309318,26.793965899482,26.8868167439165,26.9795997683517,27.0723476425272,
27.1650851888503,27.257837214602,27.3506884347121,27.4435914744667,27.5366498377001,
27.6074564441833,27.7004615096694,27.7933436061491,27.8861277750852,27.983179301891,
28.0758475566346,28.1684942988224,28.2611592745444,28.2743338823084),
 .UNSPECIFIED.);
#7712=B_SPLINE_CURVE_WITH_KNOTS('',3,(#63325,#63326,#63327,#63328,#63329,
#63330,#63331,#63332,#63333,#63334,#63335,#63336,#63337,#63338,#63339,#63340,
#63341,#63342,#63343,#63344,#63345,#63346,#63347,#63348,#63349,#63350,#63351,
#63352,#63353,#63354,#63355,#63356,#63357,#63358,#63359,#63360,#63361,#63362,
#63363,#63364,#63365,#63366,#63367,#63368,#63369,#63370,#63371,#63372,#63373,
#63374,#63375,#63376,#63377,#63378,#63379,#63380,#63381,#63382,#63383,#63384,
#63385,#63386,#63387,#63388,#63389,#63390,#63391,#63392,#63393,#63394,#63395,
#63396,#63397,#63398,#63399,#63400,#63401,#63402,#63403,#63404,#63405,#63406,
#63407,#63408,#63409,#63410,#63411,#63412,#63413,#63414,#63415,#63416,#63417,
#63418,#63419,#63420,#63421,#63422,#63423,#63424,#63425,#63426,#63427,#63428,
#63429,#63430,#63431,#63432,#63433,#63434,#63435,#63436,#63437,#63438,#63439,
#63440,#63441,#63442,#63443,#63444,#63445,#63446,#63447,#63448,#63449,#63450,
#63451,#63452,#63453,#63454,#63455,#63456,#63457,#63458,#63459,#63460,#63461,
#63462,#63463,#63464,#63465,#63466,#63467,#63468,#63469,#63470,#63471,#63472,
#63473,#63474,#63475,#63476,#63477,#63478,#63479,#63480,#63481,#63482,#63483,
#63484,#63485,#63486),.UNSPECIFIED.,.F.,.F.,(4,2,2,2,2,2,2,2,2,2,2,2,2,
2,2,2,2,2,2,2,2,2,2,2,2,2,2,2,2,2,2,2,2,2,2,2,2,2,2,2,2,2,2,2,2,2,2,2,2,
2,2,2,2,2,2,2,2,2,2,2,2,2,2,2,2,2,2,2,2,2,2,2,2,2,2,2,2,2,2,2,4),(-4.06009964275302,
-3.97992804425977,-3.96517398667009,-3.95678377382771,-3.95452870825207,
-3.9531780547404,-3.95196135775498,-3.95038794534511,-3.94698733061644,
-3.91886649491486,-3.91045137537565,-3.85776107645835,-3.82255752159171,
-3.80754592901665,-3.79758773386062,-3.79413282759724,-3.79210932390034,
-3.78993640432826,-3.78714302821738,-3.78266268571291,-3.75832162644589,
-3.70528286411963,-3.66421138389992,-3.64457413495014,-3.63430714257539,
-3.63189422565866,-3.63050841326076,-3.62929859484687,-3.62775822086802,
-3.62471682384807,-3.60590243236951,-3.5725571285863,-3.48761628522174,
-3.47943881250414,-3.47327952724946,-3.47042080337634,-3.46836213818299,
-3.46632966626124,-3.46357617879369,-3.45819033677073,-3.39359557716868,
-3.31963054963236,-3.31109910549482,-3.30883090241771,-3.30747727247695,
-3.30626125705462,-3.30469314677703,-3.30132078000891,-3.2742951446889,
-3.18912983371585,-3.16632631665581,-3.15261180098397,-3.14870379115348,
-3.1463089258773,-3.14413616406669,-3.14134342034613,-3.13686495810699,
-3.11255043628448,-3.10990108166594,-3.09652553009939,-3.09486150594946,
-3.09394210084471,-3.01861394134868,-2.9988052292843,-2.9884762911639,-2.98605865522537,
-2.98467177976948,-2.98346207776363,-2.9819232178282,-2.97878652000038,
-2.95864089803314,-2.86592438364308,-2.84329961633336,-2.82966428311039,
-2.82576435743104,-2.82337134818679,-2.82119823648568,-2.81840219482107,
-2.81260245303326,-2.73661235803911,-2.72814588356085),.UNSPECIFIED.);
#7713=B_SPLINE_CURVE_WITH_KNOTS('',3,(#63492,#63493,#63494,#63495,#63496,
#63497,#63498,#63499,#63500,#63501,#63502,#63503,#63504,#63505,#63506,#63507,
#63508,#63509,#63510,#63511,#63512,#63513,#63514,#63515,#63516,#63517,#63518,
#63519,#63520,#63521,#63522,#63523,#63524,#63525,#63526,#63527,#63528,#63529,
#63530,#63531,#63532,#63533,#63534,#63535,#63536,#63537,#63538,#63539,#63540,
#63541,#63542,#63543,#63544,#63545,#63546,#63547,#63548,#63549,#63550,#63551,
#63552,#63553,#63554,#63555,#63556,#63557,#63558,#63559,#63560,#63561,#63562,
#63563,#63564,#63565,#63566,#63567,#63568,#63569,#63570,#63571,#63572,#63573,
#63574,#63575,#63576,#63577,#63578,#63579,#63580,#63581,#63582,#63583,#63584,
#63585,#63586,#63587,#63588,#63589,#63590,#63591,#63592,#63593,#63594,#63595,
#63596,#63597,#63598,#63599,#63600,#63601,#63602,#63603,#63604,#63605,#63606,
#63607,#63608,#63609,#63610,#63611,#63612,#63613,#63614,#63615,#63616,#63617,
#63618,#63619,#63620,#63621,#63622,#63623,#63624,#63625,#63626,#63627),
 .UNSPECIFIED.,.F.,.F.,(4,3,3,3,3,3,3,3,3,3,3,3,3,3,3,3,3,3,3,3,3,3,3,3,
3,3,3,3,3,3,3,3,3,3,3,3,3,3,3,3,3,3,3,3,3,4),(34.557519189488,34.6505344770621,
34.7422837385077,34.8340075184537,34.9257316641358,35.0197091206221,35.1115640588596,
35.2066027744702,35.3016414900809,35.3947167985334,35.4876660495984,35.5805168759114,
35.6732998813377,35.7660477359647,35.8587852622214,35.951537267409,36.0443884663047,
36.1372914844509,36.2303498256485,36.3011566286076,36.3942319370643,36.4871811881334,
36.5800320144501,36.6728150198798,36.7655628745103,36.8583004007699,36.951052405961,
37.0439036048593,37.136806623008,37.2298649642077,37.3006717671344,37.3937470756148,
37.486696326708,37.5795471530493,37.672330158504,37.7650780131595,37.8578155394447,
37.9505675446612,38.0434187435853,38.1363217617599,38.2293801029855,38.3001869056612,
38.3955381070791,38.4884751037719,38.5850334075524,38.6815917113328),
 .UNSPECIFIED.);
#7714=B_SPLINE_CURVE_WITH_KNOTS('',3,(#63628,#63629,#63630,#63631,#63632,
#63633,#63634,#63635,#63636,#63637,#63638,#63639,#63640,#63641,#63642,#63643,
#63644,#63645,#63646,#63647,#63648,#63649,#63650,#63651,#63652,#63653,#63654,
#63655,#63656,#63657,#63658,#63659,#63660,#63661,#63662,#63663,#63664,#63665,
#63666,#63667,#63668,#63669,#63670,#63671,#63672,#63673,#63674,#63675,#63676,
#63677,#63678,#63679,#63680,#63681,#63682,#63683,#63684,#63685,#63686,#63687,
#63688,#63689,#63690,#63691,#63692,#63693,#63694,#63695,#63696,#63697,#63698,
#63699,#63700),.UNSPECIFIED.,.F.,.F.,(4,3,3,3,3,3,3,3,3,3,3,3,3,3,3,3,3,
3,3,3,3,3,3,3,4),(32.398493560417,32.4914400181045,32.584288739484,32.6770705647979,
32.7698178594356,32.862555445206,32.9553081292875,33.0481603497384,33.1410649461116,
33.234124163174,33.3026112130273,33.3956865213933,33.48863577237,33.5814865985929,
33.6742696039268,33.7670174584601,33.859754984622,33.9525069897136,34.0453581885121,
34.1382612065603,34.2313195476595,34.3021263515541,34.4230279815628,34.5413368973612,
34.5575191892658),.UNSPECIFIED.);
#7715=B_SPLINE_CURVE_WITH_KNOTS('',3,(#63701,#63702,#63703,#63704,#63705,
#63706,#63707,#63708,#63709,#63710,#63711,#63712,#63713,#63714,#63715,#63716,
#63717,#63718,#63719,#63720,#63721,#63722,#63723,#63724,#63725,#63726,#63727,
#63728,#63729,#63730,#63731,#63732,#63733,#63734,#63735,#63736,#63737,#63738,
#63739,#63740,#63741,#63742,#63743,#63744,#63745,#63746,#63747,#63748,#63749,
#63750,#63751,#63752,#63753,#63754,#63755,#63756,#63757,#63758,#63759,#63760,
#63761,#63762,#63763,#63764,#63765,#63766,#63767,#63768,#63769,#63770,#63771,
#63772,#63773,#63774,#63775,#63776,#63777,#63778,#63779,#63780,#63781,#63782,
#63783,#63784,#63785,#63786,#63787,#63788,#63789,#63790,#63791,#63792,#63793,
#63794,#63795,#63796,#63797,#63798,#63799,#63800,#63801,#63802,#63803,#63804,
#63805,#63806,#63807,#63808,#63809,#63810,#63811,#63812,#63813,#63814,#63815,
#63816,#63817,#63818,#63819,#63820,#63821,#63822,#63823,#63824,#63825,#63826,
#63827,#63828,#63829,#63830,#63831,#63832,#63833,#63834,#63835,#63836,#63837,
#63838,#63839,#63840,#63841,#63842,#63843,#63844,#63845,#63846,#63847,#63848,
#63849,#63850,#63851,#63852,#63853,#63854,#63855,#63856,#63857,#63858,#63859,
#63860,#63861,#63862,#63863,#63864,#63865,#63866,#63867,#63868,#63869,#63870,
#63871,#63872,#63873,#63874,#63875,#63876,#63877,#63878,#63879,#63880,#63881,
#63882,#63883,#63884,#63885,#63886,#63887,#63888,#63889,#63890,#63891,#63892,
#63893,#63894,#63895,#63896,#63897,#63898,#63899,#63900,#63901,#63902,#63903,
#63904,#63905,#63906,#63907,#63908,#63909,#63910,#63911,#63912,#63913,#63914,
#63915,#63916,#63917,#63918,#63919,#63920,#63921,#63922,#63923,#63924,#63925,
#63926,#63927,#63928,#63929,#63930,#63931,#63932,#63933,#63934,#63935,#63936,
#63937,#63938,#63939,#63940,#63941,#63942,#63943,#63944,#63945,#63946,#63947,
#63948,#63949,#63950),.UNSPECIFIED.,.F.,.F.,(4,2,2,2,2,2,2,2,2,2,2,2,2,
2,2,2,2,2,2,2,2,2,2,2,2,2,2,2,2,2,2,2,2,2,2,2,2,2,2,2,2,2,2,2,2,2,2,2,2,
2,2,2,2,2,2,2,2,2,2,2,2,2,2,2,2,2,2,2,2,2,2,2,2,2,2,2,2,2,2,2,2,2,2,2,2,
2,2,2,2,2,2,2,2,2,2,2,2,2,2,2,2,2,2,2,2,2,2,2,2,2,2,2,2,2,2,2,2,2,2,2,2,
2,2,2,4),(-2.72814588356085,-2.69177019645693,-2.67469536912849,-2.6653842791166,
-2.66304772262018,-2.66167889882582,-2.66046631150317,-2.65889895582188,
-2.65561775181486,-2.63158790163194,-2.62226201497484,-2.58316380457146,
-2.53923007112731,-2.50878040828248,-2.50381151041301,-2.50118462972761,
-2.49923549235549,-2.49680525591804,-2.49273872662273,-2.48427542112654,
-2.39726184509183,-2.37454583812146,-2.35350537375744,-2.3427389936437,
-2.34028905285507,-2.33889500416378,-2.33768617044934,-2.33615765294834,
-2.3331718265721,-2.31558103914529,-2.3114885611968,-2.21984808954366,-2.19740622093779,
-2.18385187173493,-2.17996005560742,-2.17756878509788,-2.17539512226456,
-2.17259538194739,-2.16677713791361,-2.12156670703388,-2.05122762924548,
-2.03046261082839,-2.02873442653731,-2.01974902820571,-2.01735889172253,
-2.01596410454751,-2.01475542108896,-2.01322811613195,-2.01014890330072,
-1.98368475041267,-1.93598780387023,-1.86441515715643,-1.8585190716148,
-1.85573432728855,-1.85355637139788,-1.8511808486918,-1.84735993970525,
-1.83448580519281,-1.81355154928986,-1.73889503830003,-1.7219793371213,
-1.69829405485457,-1.69502441251635,-1.69345924589282,-1.69224683121482,
-1.69087653377583,-1.68853364736509,-1.67914819348075,-1.66188264541755,
-1.61609963980977,-1.5414427893468,-1.53560596690257,-1.53280254004759,
-1.53062834547738,-1.52823883758531,-1.52435515703171,-1.51088134676842,
-1.48861763988004,-1.39802364593873,-1.39223862795602,-1.3749313452562,
-1.37196007320653,-1.37043463216816,-1.36922597841465,-1.36782958747718,
-1.36536929923475,-1.35445976583099,-1.33301233667467,-1.281722969468,-1.21874264275385,
-1.21334850096477,-1.21059263099112,-1.20855930969112,-1.20635326583741,
-1.20334556885714,-1.19640858621183,-1.12672517474231,-1.08757374952794,
-1.07608608943866,-1.05245554303779,-1.04918756186492,-1.04762263744003,
-1.04641015718119,-1.0450395089811,-1.04269538767841,-1.03329678168576,
-1.01599754217349,-0.97008734354019,-0.895598191242403,-0.889757955984397,
-0.886953712970418,-0.884779250325259,-0.882389815124442,-0.878507075747928,
-0.86504464698163,-0.842807184137572,-0.752802436087622,-0.729463685135623,
-0.726205556361693,-0.724642475779657,-0.723430104813524,-0.722058136793483,
-0.719755606108128,-0.710772727979108,-0.698275120787947),.UNSPECIFIED.);
#7716=B_SPLINE_CURVE_WITH_KNOTS('',3,(#63956,#63957,#63958,#63959,#63960,
#63961,#63962,#63963),.UNSPECIFIED.,.F.,.F.,(4,1,1,1,1,4),(40.8407078890674,
41.2987323212414,42.2982474597682,43.297762598295,44.2972777368217,44.9636567851415),
 .UNSPECIFIED.);
#7717=B_SPLINE_CURVE_WITH_KNOTS('',3,(#63964,#63965,#63966,#63967,#63968,
#63969,#63970,#63971,#63972,#63973,#63974,#63975,#63976,#63977,#63978,#63979,
#63980,#63981,#63982,#63983,#63984,#63985,#63986,#63987,#63988,#63989,#63990,
#63991,#63992,#63993,#63994,#63995,#63996,#63997,#63998,#63999,#64000,#64001,
#64002,#64003,#64004,#64005,#64006,#64007,#64008,#64009,#64010,#64011,#64012,
#64013,#64014,#64015,#64016,#64017,#64018,#64019,#64020,#64021,#64022,#64023,
#64024,#64025,#64026,#64027,#64028,#64029,#64030,#64031,#64032,#64033,#64034,
#64035,#64036),.UNSPECIFIED.,.F.,.F.,(4,3,3,3,3,3,3,3,3,3,3,3,3,3,3,3,3,
3,3,3,3,3,3,3,4),(38.6815917113328,38.7743373141285,38.8670751954702,38.9598301622261,
39.0526857539774,39.1455955076823,39.2386576504075,39.2997020441879,39.3927773526555,
39.4857266037357,39.578577430063,39.6713604355043,39.7641082901464,39.8568458164183,
39.9495978216212,40.0424490205317,40.1353520386925,40.2284103799043,40.2992171827147,
40.3954403882719,40.4915029124347,40.5873785224333,40.6831438364891,40.7787909004466,
40.8407044966676),.UNSPECIFIED.);
#7718=B_SPLINE_CURVE_WITH_KNOTS('',3,(#64038,#64039,#64040,#64041,#64042,
#64043,#64044,#64045,#64046,#64047,#64048,#64049,#64050,#64051,#64052,#64053,
#64054,#64055,#64056,#64057,#64058,#64059,#64060,#64061,#64062,#64063,#64064,
#64065,#64066,#64067,#64068,#64069,#64070,#64071,#64072,#64073,#64074,#64075,
#64076,#64077,#64078,#64079,#64080,#64081,#64082,#64083,#64084,#64085,#64086,
#64087,#64088,#64089,#64090,#64091,#64092,#64093,#64094,#64095,#64096,#64097,
#64098,#64099,#64100,#64101,#64102,#64103,#64104,#64105,#64106,#64107,#64108,
#64109,#64110,#64111,#64112,#64113,#64114,#64115,#64116,#64117,#64118,#64119,
#64120,#64121,#64122,#64123),.UNSPECIFIED.,.F.,.F.,(4,2,2,2,2,2,2,2,2,2,
2,2,2,2,2,2,2,2,2,2,2,2,2,2,2,2,2,2,2,2,2,2,2,2,2,2,2,2,2,2,2,2,4),(-0.698275120787947,
-0.694481754168329,-0.65359834429961,-0.578887684233614,-0.576569126139477,
-0.568139734998153,-0.564785870407424,-0.562739283312044,-0.560542299228753,
-0.55758817756562,-0.551187301956559,-0.518818663659694,-0.456087107595393,
-0.407076956377958,-0.40346512407881,-0.401852332517518,-0.40062951497057,
-0.399297883999417,-0.397128777122514,-0.39078755961723,-0.380253630449211,
-0.342088828524308,-0.30547068583101,-0.249936696390069,-0.244560221483311,
-0.241808730477856,-0.239776381400394,-0.237569209632325,-0.234556060611483,
-0.23122828167922,-0.209077898377296,-0.177515406120868,-0.150746248996183,
-0.112175633548954,-0.083931029342986,-0.0805266912655971,-0.0789523815532209,
-0.0777353548320273,-0.0763847196102382,-0.0749803046708111,-0.0728817699842837,
-0.0690783852891989,-0.000960649026662135),.UNSPECIFIED.);
#7719=B_SPLINE_CURVE_WITH_KNOTS('',3,(#64124,#64125,#64126,#64127,#64128,
#64129,#64130,#64131,#64132,#64133,#64134,#64135,#64136,#64137,#64138,#64139,
#64140,#64141,#64142,#64143,#64144,#64145,#64146,#64147,#64148,#64149,#64150,
#64151,#64152,#64153,#64154,#64155,#64156,#64157,#64158,#64159,#64160,#64161,
#64162,#64163,#64164,#64165,#64166,#64167,#64168,#64169,#64170,#64171,#64172,
#64173,#64174,#64175,#64176,#64177,#64178,#64179,#64180,#64181,#64182,#64183,
#64184,#64185,#64186,#64187,#64188,#64189,#64190,#64191,#64192,#64193,#64194,
#64195,#64196,#64197,#64198,#64199,#64200,#64201,#64202,#64203,#64204,#64205,
#64206,#64207,#64208,#64209,#64210,#64211,#64212,#64213,#64214,#64215,#64216,
#64217,#64218,#64219,#64220,#64221,#64222,#64223,#64224,#64225,#64226,#64227,
#64228,#64229,#64230,#64231,#64232,#64233,#64234,#64235,#64236,#64237,#64238,
#64239,#64240,#64241,#64242,#64243,#64244,#64245,#64246,#64247,#64248,#64249,
#64250,#64251,#64252,#64253,#64254,#64255,#64256,#64257,#64258,#64259,#64260,
#64261,#64262,#64263,#64264,#64265,#64266,#64267,#64268,#64269,#64270,#64271,
#64272,#64273,#64274,#64275,#64276,#64277,#64278,#64279,#64280,#64281,#64282,
#64283,#64284,#64285,#64286,#64287,#64288,#64289,#64290,#64291,#64292,#64293),
 .UNSPECIFIED.,.F.,.F.,(4,2,2,2,2,2,2,2,2,2,2,2,2,2,2,2,2,2,2,2,2,2,2,2,
2,2,2,2,2,2,2,2,2,2,2,2,2,2,2,2,2,2,2,2,2,2,2,2,2,2,2,2,2,2,2,2,2,2,2,2,
2,2,2,2,2,2,2,2,2,2,2,2,2,2,2,2,2,2,2,2,2,2,2,2,4),(-4.0612507056947,-3.99202977575391,
-3.98577881057836,-3.98222911984111,-3.97979640459323,-3.97742408197083,
-3.97524503370926,-3.97245334071522,-3.96652141533724,-3.89685826979705,
-3.86584932583547,-3.8236133732283,-3.81861094457848,-3.81717794025091,
-3.8158073704685,-3.81459495984103,-3.81303013495953,-3.8097623808746,-3.7861333078054,
-3.77473796988285,-3.7542447443314,-3.71336236918133,-3.6797773212617,-3.66791235714937,
-3.65962581215465,-3.65713960343181,-3.65473005278243,-3.6525601792093,
-3.64979354641334,-3.6454015300522,-3.62249741686864,-3.61044938039733,
-3.5968227551182,-3.54055228905148,-3.5022385741652,-3.49630373938915,-3.4942794784051,
-3.49293703422616,-3.49171784914348,-3.49012803862183,-3.48745817868347,
-3.47097173587069,-3.46779248679077,-3.43521151009245,-3.35011627573823,
-3.33783876516051,-3.33409499609949,-3.3317195680478,-3.32954142462936,
-3.32675606230569,-3.32085724289751,-3.27111715895282,-3.2322756078014,
-3.19641892663022,-3.18194008908594,-3.17366279865676,-3.17141824798157,
-3.17006989349282,-3.16885249613876,-3.16727450776883,-3.16464470905579,
-3.14895241260511,-3.05240067973554,-3.0291282786678,-3.01520770265688,
-3.0112791872356,-3.0088798054648,-3.00670819738217,-3.00392425108982,-2.99947457783985,
-2.97561243519846,-2.97408799060702,-2.97263934896084,-2.95434332048045,
-2.88206334934274,-2.86162985528179,-2.85107770609007,-2.84864352035311,
-2.84725302616619,-2.84604387431351,-2.84451053707853,-2.84150191877917,
-2.82340927730233,-2.72895044739071,-2.72876388076409),.UNSPECIFIED.);
#7720=B_SPLINE_CURVE_WITH_KNOTS('',3,(#64299,#64300,#64301,#64302,#64303,
#64304,#64305,#64306,#64307,#64308,#64309,#64310,#64311,#64312,#64313,#64314,
#64315,#64316,#64317,#64318,#64319,#64320,#64321,#64322,#64323,#64324,#64325,
#64326,#64327,#64328,#64329,#64330,#64331,#64332,#64333,#64334,#64335,#64336,
#64337,#64338,#64339,#64340,#64341,#64342,#64343,#64344,#64345,#64346,#64347,
#64348,#64349,#64350,#64351,#64352,#64353,#64354,#64355,#64356,#64357,#64358,
#64359,#64360,#64361,#64362,#64363,#64364,#64365,#64366,#64367,#64368,#64369,
#64370,#64371,#64372,#64373,#64374,#64375,#64376,#64377,#64378,#64379,#64380,
#64381,#64382,#64383,#64384,#64385,#64386,#64387,#64388,#64389,#64390,#64391,
#64392,#64393,#64394,#64395,#64396,#64397,#64398,#64399,#64400,#64401,#64402,
#64403,#64404,#64405,#64406,#64407,#64408,#64409,#64410,#64411,#64412,#64413,
#64414,#64415,#64416,#64417,#64418,#64419,#64420,#64421,#64422,#64423,#64424,
#64425,#64426,#64427,#64428,#64429,#64430,#64431,#64432,#64433,#64434,#64435,
#64436,#64437),.UNSPECIFIED.,.F.,.F.,(4,3,3,3,3,3,3,3,3,3,3,3,3,3,3,3,3,
3,3,3,3,3,3,3,3,3,3,3,3,3,3,3,3,3,3,3,3,3,3,3,3,3,3,3,3,3,4),(47.1238898038472,
47.2690103312467,47.295823152402,47.3888984608709,47.4818477119524,47.5746985382818,
47.6674815437246,47.7602293983682,47.8529669246414,47.9457189298455,48.0385701287575,
48.1314731469199,48.2245314881333,48.2953382909288,48.3884135993978,48.4813628504793,
48.5742136768088,48.6669966822516,48.7597445368951,48.8524820631684,48.9452340683726,
49.0380852672846,49.1309882854469,49.2240466266604,49.2948534294556,49.3879287379245,
49.4808779890061,49.5737288153355,49.6665118207783,49.7592596754218,49.8519972016951,
49.9447492068992,50.0376004058112,50.1305034239736,50.2235617651871,50.2943685679823,
50.3874468243774,50.480398265598,50.5762688023673,50.6690483864422,50.7617925555681,
50.8545261311983,50.9472739191532,51.0401081233949,51.1329944299035,51.2260053885434,
51.2473625597526),.UNSPECIFIED.);
#7721=B_SPLINE_CURVE_WITH_KNOTS('',3,(#64438,#64439,#64440,#64441,#64442,
#64443),.UNSPECIFIED.,.F.,.F.,(4,1,1,4),(44.9636567851415,45.2967928753485,
46.2963080138753,47.1238839646002),.UNSPECIFIED.);
#7722=B_SPLINE_CURVE_WITH_KNOTS('',3,(#64444,#64445,#64446,#64447,#64448,
#64449,#64450,#64451,#64452,#64453,#64454,#64455,#64456,#64457,#64458,#64459,
#64460,#64461,#64462,#64463,#64464,#64465,#64466,#64467,#64468,#64469,#64470,
#64471,#64472,#64473,#64474,#64475,#64476,#64477,#64478,#64479,#64480,#64481,
#64482,#64483,#64484,#64485,#64486,#64487,#64488,#64489,#64490,#64491,#64492,
#64493,#64494,#64495,#64496,#64497,#64498,#64499,#64500,#64501,#64502,#64503,
#64504,#64505,#64506,#64507,#64508,#64509,#64510,#64511,#64512,#64513,#64514,
#64515,#64516,#64517,#64518,#64519,#64520,#64521,#64522,#64523,#64524,#64525,
#64526,#64527,#64528,#64529,#64530,#64531,#64532,#64533,#64534,#64535,#64536,
#64537,#64538,#64539,#64540,#64541,#64542,#64543,#64544,#64545,#64546,#64547,
#64548,#64549,#64550,#64551,#64552,#64553,#64554,#64555,#64556,#64557,#64558,
#64559,#64560,#64561,#64562,#64563,#64564,#64565,#64566,#64567,#64568,#64569,
#64570,#64571,#64572,#64573,#64574,#64575,#64576,#64577,#64578,#64579,#64580,
#64581,#64582,#64583,#64584,#64585,#64586,#64587,#64588,#64589,#64590,#64591,
#64592,#64593,#64594,#64595,#64596,#64597,#64598,#64599,#64600,#64601,#64602,
#64603,#64604,#64605,#64606,#64607,#64608,#64609,#64610,#64611,#64612,#64613,
#64614,#64615,#64616,#64617,#64618,#64619,#64620,#64621,#64622,#64623,#64624,
#64625,#64626,#64627,#64628,#64629,#64630,#64631,#64632,#64633,#64634,#64635,
#64636,#64637,#64638,#64639,#64640,#64641,#64642,#64643,#64644,#64645,#64646,
#64647,#64648,#64649,#64650,#64651,#64652,#64653,#64654,#64655,#64656,#64657,
#64658,#64659,#64660,#64661,#64662,#64663,#64664,#64665,#64666,#64667,#64668,
#64669,#64670,#64671,#64672,#64673,#64674,#64675,#64676,#64677,#64678,#64679,
#64680,#64681,#64682,#64683,#64684,#64685,#64686,#64687,#64688,#64689,#64690,
#64691),.UNSPECIFIED.,.F.,.F.,(4,2,2,2,2,2,2,2,2,2,2,2,2,2,2,2,2,2,2,2,
2,2,2,2,2,2,2,2,2,2,2,2,2,2,2,2,2,2,2,2,2,2,2,2,2,2,2,2,2,2,2,2,2,2,2,2,
2,2,2,2,2,2,2,2,2,2,2,2,2,2,2,2,2,2,2,2,2,2,2,2,2,2,2,2,2,2,2,2,2,2,2,2,
2,2,2,2,2,2,2,2,2,2,2,2,2,2,2,2,2,2,2,2,2,2,2,2,2,2,2,2,2,2,2,4),(-2.72876388076409,
-2.70602756235829,-2.69226073086636,-2.68834769640442,-2.68595185125752,
-2.68377957454858,-2.68098937381791,-2.67521891085425,-2.5980940570774,
-2.53558913764033,-2.52768699829943,-2.52547884152408,-2.52413869965223,
-2.52291909162726,-2.52132535198181,-2.51864161040144,-2.50186592293099,
-2.49699869828275,-2.48767090755633,-2.4445283258113,-2.37305419959333,
-2.36697078421131,-2.36411985033116,-2.36193931598696,-2.3598631099989,
-2.35694252463151,-2.34915560857357,-2.34605591497491,-2.26875091452462,
-2.21225011000985,-2.20472664652994,-2.20255672876644,-2.20122508894515,
-2.20000261584029,-2.19839076081773,-2.19478300369353,-2.15157901288759,
-2.13963522134518,-2.08940052766873,-2.06236063068565,-2.04684165996687,
-2.04276264129758,-2.04032955827826,-2.03816420018406,-2.03543801766571,
-2.03117758609425,-2.00596574729667,-1.9496717496429,-1.88867971437931,
-1.8819080804077,-1.8797373446587,-1.87853822289915,-1.87744802182779,-1.87595362009319,
-1.87303552811591,-1.85260943450499,-1.81963255525067,-1.73231608544955,
-1.72708474619877,-1.72172197231819,-1.71897428525977,-1.7169431841603,
-1.71473585613343,-1.71171977789322,-1.70473385443277,-1.64117642788127,
-1.59865860289724,-1.5782920231787,-1.56051261179462,-1.55751723321027,
-1.55598671581549,-1.55477778106601,-1.55338527508967,-1.55094209177177,
-1.54026747308313,-1.51949089623647,-1.44927318145286,-1.40402799963735,
-1.39820944487283,-1.39540963885789,-1.39323596155489,-1.3908447119159,
-1.38695301317143,-1.37339996795555,-1.35095797420423,-1.25928426084271,
-1.2553040496369,-1.23757931627163,-1.23458650537719,-1.2330564434065,-1.23184742982321,
-1.23045433970987,-1.22800893195824,-1.21730619280207,-1.19645074136639,
-1.12648050037713,-1.08108697270815,-1.07526514695507,-1.07246451857569,
-1.07029053698862,-1.06789928970158,-1.06400835211364,-1.05046548273603,
-1.02804727024587,-0.936520137852073,-0.932813543499302,-0.914648270766425,
-0.911635716583265,-0.910101318196676,-0.9088918114962,-0.907501443260302,
-0.905068778167366,-0.89454260015925,-0.874187499231618,-0.783057456156521,
-0.756866100645749,-0.75228490523195,-0.749491188763659,-0.7473117221757,
-0.744940117456575,-0.741137677410085,-0.72868292852517,-0.708565803663826,
-0.698900011106378),.UNSPECIFIED.);
#7723=B_SPLINE_CURVE_WITH_KNOTS('',3,(#64697,#64698,#64699,#64700,#64701,
#64702,#64703,#64704),.UNSPECIFIED.,.F.,.F.,(4,1,1,1,1,4),(53.4070839884957,
54.2924291220894,55.2919442606161,56.2914593991429,57.2909745376696,57.5317208912133),
 .UNSPECIFIED.);
#7724=B_SPLINE_CURVE_WITH_KNOTS('',3,(#64705,#64706,#64707,#64708,#64709,
#64710,#64711,#64712,#64713,#64714,#64715,#64716,#64717,#64718,#64719,#64720,
#64721,#64722,#64723,#64724,#64725,#64726,#64727,#64728,#64729,#64730,#64731,
#64732,#64733,#64734,#64735,#64736,#64737,#64738,#64739,#64740,#64741,#64742,
#64743,#64744,#64745,#64746,#64747,#64748,#64749,#64750,#64751,#64752,#64753,
#64754,#64755,#64756,#64757,#64758,#64759,#64760,#64761,#64762,#64763,#64764,
#64765,#64766,#64767,#64768,#64769,#64770,#64771,#64772,#64773,#64774,#64775,
#64776,#64777),.UNSPECIFIED.,.F.,.F.,(4,3,3,3,3,3,3,3,3,3,3,3,3,3,3,3,3,
3,3,3,3,3,3,3,4),(51.2473625597526,51.2938837065091,51.386959014978,51.4799082660596,
51.5727590923892,51.6655420978319,51.7582899524755,51.8510274787487,51.9437794839529,
52.0366306828649,52.1295337010273,52.2225920422408,52.2933988450358,52.3864741535047,
52.4794234045863,52.5722742309156,52.6650572363584,52.7578050910019,52.8505426172751,
52.9432946224792,53.0361458213912,53.1290488395536,53.222107180767,53.2929139835626,
53.4070751110268),.UNSPECIFIED.);
#7725=B_SPLINE_CURVE_WITH_KNOTS('',3,(#64779,#64780,#64781,#64782,#64783,
#64784,#64785,#64786,#64787,#64788,#64789,#64790,#64791,#64792,#64793,#64794,
#64795,#64796,#64797,#64798,#64799,#64800,#64801,#64802,#64803,#64804,#64805,
#64806,#64807,#64808,#64809,#64810,#64811,#64812,#64813,#64814,#64815,#64816,
#64817,#64818,#64819,#64820,#64821,#64822,#64823,#64824,#64825,#64826,#64827,
#64828,#64829,#64830,#64831,#64832,#64833,#64834,#64835,#64836,#64837,#64838,
#64839,#64840,#64841,#64842,#64843,#64844,#64845,#64846,#64847,#64848,#64849,
#64850,#64851,#64852,#64853,#64854,#64855,#64856,#64857,#64858,#64859,#64860,
#64861,#64862),.UNSPECIFIED.,.F.,.F.,(4,2,2,2,2,2,2,2,2,2,2,2,2,2,2,2,2,
2,2,2,2,2,2,2,2,2,2,2,2,2,2,2,2,2,2,2,2,2,2,2,2,4),(-0.698900011106378,
-0.664621630843526,-0.616528634413205,-0.592100740903726,-0.588805704293141,
-0.587252280301598,-0.586038107846558,-0.584675991467339,-0.582416399969052,
-0.573965824956321,-0.50096915406343,-0.473014118631769,-0.459328988812959,
-0.456875210752135,-0.433699831937314,-0.429291313732653,-0.426519650652467,
-0.424349205785662,-0.42194248599253,-0.417982213918182,-0.404016206776864,
-0.380538053041719,-0.313060341648312,-0.269698333722163,-0.266089288043848,
-0.264477082834381,-0.26325443855795,-0.261922709538034,-0.260545508384321,
-0.256155984822727,-0.221941283444193,-0.195052399865455,-0.118521449148602,
-0.116433301572504,-0.107893624668228,-0.104521269988041,-0.102471308191436,
-0.100276752428945,-0.097336400912601,-0.0907751578210967,-0.0820187210215503,
-0.00096106920673559),.UNSPECIFIED.);
#7726=B_SPLINE_CURVE_WITH_KNOTS('',3,(#64863,#64864,#64865,#64866,#64867,
#64868,#64869,#64870,#64871,#64872,#64873,#64874,#64875,#64876,#64877,#64878,
#64879,#64880,#64881,#64882,#64883,#64884,#64885,#64886,#64887,#64888,#64889,
#64890,#64891,#64892,#64893,#64894,#64895,#64896,#64897,#64898,#64899,#64900,
#64901,#64902,#64903,#64904,#64905,#64906,#64907,#64908,#64909,#64910,#64911,
#64912,#64913,#64914,#64915,#64916,#64917,#64918,#64919,#64920,#64921,#64922,
#64923,#64924,#64925,#64926,#64927,#64928,#64929,#64930,#64931,#64932,#64933,
#64934,#64935,#64936,#64937,#64938,#64939,#64940,#64941,#64942,#64943,#64944,
#64945,#64946,#64947,#64948,#64949,#64950,#64951,#64952,#64953,#64954,#64955,
#64956,#64957,#64958,#64959,#64960,#64961,#64962,#64963,#64964,#64965,#64966,
#64967,#64968,#64969,#64970,#64971,#64972,#64973,#64974,#64975,#64976,#64977,
#64978,#64979,#64980,#64981,#64982,#64983,#64984,#64985,#64986,#64987,#64988,
#64989,#64990,#64991,#64992,#64993,#64994,#64995,#64996,#64997,#64998,#64999,
#65000,#65001,#65002,#65003,#65004,#65005,#65006,#65007,#65008,#65009,#65010,
#65011,#65012,#65013,#65014,#65015,#65016,#65017,#65018,#65019,#65020,#65021,
#65022,#65023,#65024),.UNSPECIFIED.,.F.,.F.,(4,2,2,2,2,2,2,2,2,2,2,2,2,
2,2,2,2,2,2,2,2,2,2,2,2,2,2,2,2,2,2,2,2,2,2,2,2,2,2,2,2,2,2,2,2,2,2,2,2,
2,2,2,2,2,2,2,2,2,2,2,2,2,2,2,2,2,2,2,2,2,2,2,2,2,2,2,2,2,2,2,4),(-4.06068215332971,
-4.01016739059331,-4.00563546502231,-4.0034750215586,-4.00204496752844,
-4.00067647320423,-3.99946368735555,-3.99789541860962,-3.99460996949297,
-3.97046173073304,-3.94341465850605,-3.92453635391737,-3.90748724446368,
-3.85923553553613,-3.84585301283487,-3.84194707613627,-3.83955247588097,
-3.83737929525466,-3.83458509090088,-3.82879611066212,-3.75232872134662,
-3.70466219579208,-3.68981300428414,-3.68141227696476,-3.67915992946697,
-3.67779944745224,-3.67658487540966,-3.67502853482328,-3.67171841939994,
-3.64683347272879,-3.5986079407557,-3.5277772219995,-3.52091448859619,-3.51791991256651,
-3.51571617170279,-3.51367980834526,-3.5103799048344,-3.50227006628849,
-3.49960685706945,-3.4225178097056,-3.36580317974603,-3.35829040904099,
-3.35612722825411,-3.3547870362861,-3.35356705766937,-3.35197239791703,
-3.34928616392161,-3.33246838087751,-3.23688512807977,-3.21377106282806,
-3.19991935773195,-3.19599730288214,-3.19359912742348,-3.19142682324009,
-3.188639494635,-3.18417941815438,-3.16015656097722,-3.15886779619432,-3.15733800062712,
-3.13904129165035,-3.1137563079839,-3.0656739991336,-3.04605268995558,-3.03579126197613,
-3.03337866513771,-3.03199287042536,-3.03078296031161,-3.02924233038554,
-3.02609695918307,-3.00574312816377,-2.91319853156648,-2.89060292282442,
-2.87698036037882,-2.87308162481383,-2.87068881823995,-2.86851554397552,
-2.86571880733699,-2.85991586749835,-2.81554783012779,-2.74408992563194,
-2.72867715037577),.UNSPECIFIED.);
#7727=B_SPLINE_CURVE_WITH_KNOTS('',3,(#65030,#65031,#65032,#65033,#65034,
#65035,#65036,#65037,#65038,#65039,#65040,#65041,#65042,#65043,#65044,#65045,
#65046,#65047,#65048,#65049,#65050,#65051,#65052,#65053,#65054,#65055,#65056,
#65057,#65058,#65059,#65060,#65061,#65062,#65063,#65064,#65065,#65066,#65067,
#65068,#65069,#65070,#65071,#65072,#65073,#65074,#65075,#65076,#65077,#65078,
#65079,#65080,#65081,#65082,#65083,#65084,#65085,#65086,#65087,#65088,#65089,
#65090,#65091,#65092,#65093,#65094,#65095,#65096,#65097,#65098,#65099,#65100,
#65101,#65102,#65103,#65104,#65105,#65106,#65107,#65108,#65109,#65110,#65111,
#65112,#65113,#65114,#65115,#65116,#65117,#65118,#65119,#65120,#65121,#65122,
#65123,#65124,#65125,#65126,#65127,#65128,#65129,#65130,#65131,#65132,#65133,
#65134,#65135,#65136,#65137,#65138,#65139,#65140,#65141,#65142,#65143,#65144,
#65145,#65146,#65147,#65148,#65149,#65150,#65151,#65152,#65153,#65154,#65155,
#65156,#65157,#65158,#65159,#65160,#65161,#65162,#65163,#65164,#65165,#65166,
#65167,#65168),.UNSPECIFIED.,.F.,.F.,(4,3,3,3,3,3,3,3,3,3,3,3,3,3,3,3,3,
3,3,3,3,3,3,3,3,3,3,3,3,3,3,3,3,3,3,3,3,3,3,3,3,3,3,3,3,3,4),(59.6902604182064,
59.7842625762968,59.8782936636862,59.9723761264494,60.0665973185503,60.1608983242092,
60.2553670544362,60.2895199532499,60.3825952617188,60.4755445128005,60.5683953391299,
60.6611783445727,60.7539261992163,60.8466637254895,60.9394157306936,61.0322669296056,
61.125169947768,61.2182282889814,61.2890350917767,61.3821104002456,61.4750596513273,
61.5679104776568,61.6606934830996,61.7534413377431,61.8461788640163,61.9389308692204,
62.0317820681324,62.1246850862947,62.2177434275082,62.2885502303035,62.3816255387724,
62.474574789854,62.5674256161836,62.6602086216264,62.75295647627,62.8456940025433,
62.9384460077475,63.0312972066595,63.1242002248218,63.2172585660352,63.2880653688302,
63.3811374997221,63.4740886781739,63.5669306360504,63.659708699058,63.7524558212429,
63.8139030978781),.UNSPECIFIED.);
#7728=B_SPLINE_CURVE_WITH_KNOTS('',3,(#65169,#65170,#65171,#65172,#65173,
#65174),.UNSPECIFIED.,.F.,.F.,(4,1,1,4),(57.5317208912133,58.2904896761964,
59.2900048147232,59.6902534604737),.UNSPECIFIED.);
#7729=B_SPLINE_CURVE_WITH_KNOTS('',3,(#65175,#65176,#65177,#65178,#65179,
#65180,#65181,#65182,#65183,#65184,#65185,#65186,#65187,#65188,#65189,#65190,
#65191,#65192,#65193,#65194,#65195,#65196,#65197,#65198,#65199,#65200,#65201,
#65202,#65203,#65204,#65205,#65206,#65207,#65208,#65209,#65210,#65211,#65212,
#65213,#65214,#65215,#65216,#65217,#65218,#65219,#65220,#65221,#65222,#65223,
#65224,#65225,#65226,#65227,#65228,#65229,#65230,#65231,#65232,#65233,#65234,
#65235,#65236,#65237,#65238,#65239,#65240,#65241,#65242,#65243,#65244,#65245,
#65246,#65247,#65248,#65249,#65250,#65251,#65252,#65253,#65254,#65255,#65256,
#65257,#65258,#65259,#65260,#65261,#65262,#65263,#65264,#65265,#65266,#65267,
#65268,#65269,#65270,#65271,#65272,#65273,#65274,#65275,#65276,#65277,#65278,
#65279,#65280,#65281,#65282,#65283,#65284,#65285,#65286,#65287,#65288,#65289,
#65290,#65291,#65292,#65293,#65294,#65295,#65296,#65297,#65298,#65299,#65300,
#65301,#65302,#65303,#65304,#65305,#65306,#65307,#65308,#65309,#65310,#65311,
#65312,#65313,#65314,#65315,#65316,#65317,#65318,#65319,#65320,#65321,#65322,
#65323,#65324,#65325,#65326,#65327,#65328,#65329,#65330,#65331,#65332,#65333,
#65334,#65335,#65336,#65337,#65338,#65339,#65340,#65341,#65342,#65343,#65344,
#65345,#65346,#65347,#65348,#65349,#65350,#65351,#65352,#65353,#65354,#65355,
#65356,#65357,#65358,#65359,#65360,#65361,#65362,#65363,#65364,#65365,#65366,
#65367,#65368,#65369,#65370,#65371,#65372,#65373,#65374,#65375,#65376,#65377,
#65378,#65379,#65380,#65381,#65382,#65383,#65384,#65385,#65386,#65387,#65388,
#65389,#65390,#65391,#65392,#65393,#65394,#65395,#65396,#65397,#65398,#65399,
#65400,#65401,#65402,#65403,#65404,#65405,#65406,#65407,#65408,#65409,#65410,
#65411,#65412,#65413,#65414,#65415,#65416),.UNSPECIFIED.,.F.,.F.,(4,2,2,
2,2,2,2,2,2,2,2,2,2,2,2,2,2,2,2,2,2,2,2,2,2,2,2,2,2,2,2,2,2,2,2,2,2,2,2,
2,2,2,2,2,2,2,2,2,2,2,2,2,2,2,2,2,2,2,2,2,2,2,2,2,2,2,2,2,2,2,2,2,2,2,2,
2,2,2,2,2,2,2,2,2,2,2,2,2,2,2,2,2,2,2,2,2,2,2,2,2,2,2,2,2,2,2,2,2,2,2,2,
2,2,2,2,2,2,2,2,2,4),(-2.72867715037577,-2.72350407496648,-2.71289780256903,
-2.71045956996983,-2.7090681448379,-2.70785905156677,-2.70632691622698,
-2.7033240763568,-2.6853563718748,-2.68156789265345,-2.59001279875908,-2.56758563996592,
-2.55403799014216,-2.55014696977012,-2.54775594541731,-2.54558234649511,
-2.54278246399505,-2.53696310998938,-2.49167948101183,-2.42159372062447,
-2.40070650571641,-2.38999416984859,-2.38754828733318,-2.38615521232169,
-2.38494638716493,-2.38341679765986,-2.38042561307028,-2.36272687962605,
-2.30347046810249,-2.23548875402994,-2.22901404479245,-2.22608979732971,
-2.22389810728979,-2.22184417016827,-2.21844985692808,-2.20977639605324,
-2.20785070940592,-2.13190923664674,-2.07019963873847,-2.06572801028936,
-2.06395013605944,-2.06270319861711,-2.06157159851997,-2.06003674240042,
-2.05703041579629,-2.03124821076372,-1.98393231425603,-1.96311396042574,
-1.91178647330223,-1.90586452634126,-1.90307477011337,-1.90089603121276,
-1.89852283013627,-1.89471261053369,-1.88193890002056,-1.86122446382206,
-1.80297127806423,-1.7460374583062,-1.74250172915425,-1.74090302913681,
-1.73968256174143,-1.73834460923278,-1.73614666178869,-1.72834864008394,
-1.66756532909262,-1.59504583184413,-1.59273614794498,-1.58429649915555,
-1.58094122807485,-1.57889461635511,-1.57669824672687,-1.57374606860842,
-1.56711899847704,-1.55825199323859,-1.53608757523221,-1.44611393163774,
-1.42265032937607,-1.41938806983371,-1.41782425288784,-1.41661188217892,
-1.41524053939206,-1.41289334816374,-1.40345803212728,-1.38606288984755,
-1.33982106713559,-1.26581435253348,-1.25996542384353,-1.25715945918686,
-1.25498474766144,-1.25259613138786,-1.2487171680703,-1.23529188428178,
-1.21313777151261,-1.12323423133126,-1.09967625403648,-1.09641051067266,
-1.09484592602631,-1.09363337371947,-1.09226227760491,-1.08991654809614,
-1.08050059269318,-1.06315678286072,-1.01708785574675,-0.942809611863748,
-0.936966950096965,-0.934162055932783,-0.931987316175677,-0.929597805724423,
-0.925715457600736,-0.912259444858125,-0.890037214079459,-0.799709511656546,
-0.776638477923404,-0.773389424747365,-0.771828023925658,-0.770615724651503,
-0.769242488722856,-0.766887502364802,-0.757361245570541,-0.739728680357567,
-0.698670975029854),.UNSPECIFIED.);
#7730=B_SPLINE_CURVE_WITH_KNOTS('',3,(#65422,#65423,#65424,#65425,#65426,
#65427,#65428,#65429),.UNSPECIFIED.,.F.,.F.,(4,1,1,1,1,4),(65.9734521657886,
66.2866107844105,67.2861259229373,68.285641061464,69.2851561999908,70.0962929016582),
 .UNSPECIFIED.);
#7731=B_SPLINE_CURVE_WITH_KNOTS('',3,(#65430,#65431,#65432,#65433,#65434,
#65435,#65436,#65437,#65438,#65439,#65440,#65441,#65442,#65443,#65444,#65445,
#65446,#65447,#65448,#65449,#65450,#65451,#65452,#65453,#65454,#65455,#65456,
#65457,#65458,#65459,#65460,#65461,#65462,#65463,#65464,#65465,#65466,#65467,
#65468,#65469,#65470,#65471,#65472,#65473,#65474,#65475,#65476,#65477,#65478,
#65479,#65480,#65481,#65482,#65483,#65484,#65485,#65486,#65487,#65488,#65489,
#65490,#65491,#65492,#65493,#65494,#65495,#65496,#65497,#65498,#65499,#65500,
#65501,#65502),.UNSPECIFIED.,.F.,.F.,(4,3,3,3,3,3,3,3,3,3,3,3,3,3,3,3,3,
3,3,3,3,3,3,3,4),(63.8139030978781,63.9066474418343,64.001880708215,64.0947651897081,
64.1911728485326,64.287580507357,64.380655815826,64.4736050669074,64.5664558932367,
64.6592388986794,64.751986753323,64.8447242795962,64.9374762848006,65.0303274837126,
65.123230501875,65.2162888430884,65.2870956458838,65.37978898859,65.4723622086882,
65.564840709142,65.6572498016576,65.7496260993385,65.8419832821929,65.9343713417692,
65.973445725386),.UNSPECIFIED.);
#7732=B_SPLINE_CURVE_WITH_KNOTS('',3,(#65504,#65505,#65506,#65507,#65508,
#65509,#65510,#65511,#65512,#65513,#65514,#65515,#65516,#65517,#65518,#65519,
#65520,#65521,#65522,#65523,#65524,#65525,#65526,#65527,#65528,#65529,#65530,
#65531,#65532,#65533,#65534,#65535,#65536,#65537,#65538,#65539,#65540,#65541,
#65542,#65543,#65544,#65545,#65546,#65547,#65548,#65549,#65550,#65551,#65552,
#65553,#65554,#65555,#65556,#65557,#65558,#65559,#65560,#65561,#65562,#65563,
#65564,#65565,#65566,#65567,#65568,#65569,#65570,#65571,#65572,#65573,#65574,
#65575,#65576,#65577,#65578,#65579,#65580,#65581,#65582,#65583,#65584,#65585,
#65586,#65587,#65588,#65589),.UNSPECIFIED.,.F.,.F.,(4,2,2,2,2,2,2,2,2,2,
2,2,2,2,2,2,2,2,2,2,2,2,2,2,2,2,2,2,2,2,2,2,2,2,2,2,2,2,2,2,2,2,4),(-0.698670975029854,
-0.692823758210332,-0.619834095291595,-0.613960179767915,-0.61117919205671,
-0.609001231608271,-0.60670600431764,-0.603057183924118,-0.598757398167659,
-0.590584728168661,-0.505518213053075,-0.472576763803538,-0.471041835003278,
-0.453279465037479,-0.450284201222689,-0.448753387532379,-0.447544037092701,
-0.446150848025735,-0.4437059697061,-0.433016337434033,-0.412200570169519,
-0.366623274314038,-0.296924322599318,-0.291577216408451,-0.28883307806977,
-0.286802414879055,-0.284744543073832,-0.281876158665878,-0.275661204429219,
-0.267397018166896,-0.247307535613368,-0.203469221567176,-0.163588703485155,
-0.155263457366295,-0.130778221950257,-0.127480746525178,-0.125926659863407,
-0.124712189090788,-0.123349980676063,-0.12104447028807,-0.1121016596629,
-0.0959764796556443,-0.000961420122294117),.UNSPECIFIED.);
#7733=B_SPLINE_CURVE_WITH_KNOTS('',3,(#65590,#65591,#65592,#65593,#65594,
#65595,#65596,#65597,#65598,#65599,#65600,#65601,#65602,#65603,#65604,#65605,
#65606,#65607,#65608,#65609,#65610,#65611,#65612,#65613,#65614,#65615,#65616,
#65617,#65618,#65619,#65620,#65621,#65622,#65623,#65624,#65625,#65626,#65627,
#65628,#65629,#65630,#65631,#65632,#65633,#65634,#65635,#65636,#65637,#65638,
#65639,#65640,#65641,#65642,#65643,#65644,#65645,#65646,#65647,#65648,#65649,
#65650,#65651,#65652,#65653,#65654,#65655,#65656,#65657,#65658,#65659,#65660,
#65661,#65662,#65663,#65664,#65665,#65666,#65667,#65668,#65669,#65670,#65671,
#65672,#65673,#65674,#65675,#65676,#65677,#65678,#65679,#65680,#65681,#65682,
#65683,#65684,#65685,#65686,#65687,#65688,#65689,#65690,#65691,#65692,#65693,
#65694,#65695,#65696,#65697,#65698,#65699,#65700,#65701,#65702,#65703,#65704,
#65705,#65706,#65707,#65708,#65709,#65710,#65711,#65712,#65713,#65714,#65715,
#65716,#65717,#65718,#65719,#65720,#65721,#65722,#65723,#65724,#65725,#65726,
#65727,#65728,#65729,#65730,#65731,#65732,#65733,#65734,#65735,#65736,#65737,
#65738,#65739,#65740,#65741,#65742,#65743,#65744,#65745,#65746,#65747,#65748,
#65749,#65750,#65751,#65752,#65753,#65754,#65755,#65756,#65757,#65758,#65759,
#65760,#65761,#65762,#65763,#65764,#65765,#65766,#65767,#65768,#65769,#65770,
#65771,#65772,#65773,#65774,#65775,#65776,#65777,#65778,#65779,#65780,#65781,
#65782,#65783,#65784,#65785,#65786,#65787,#65788,#65789,#65790,#65791,#65792,
#65793,#65794,#65795,#65796,#65797,#65798,#65799),.UNSPECIFIED.,.F.,.F.,
(4,2,2,2,2,2,2,2,2,2,2,2,2,2,2,2,2,2,2,2,2,2,2,2,2,2,2,2,2,2,2,2,2,2,2,
2,2,2,2,2,2,2,2,2,2,2,2,2,2,2,2,2,2,2,2,2,2,2,2,2,2,2,2,2,2,2,2,2,2,2,2,
2,2,2,2,2,2,2,2,2,2,2,2,2,2,2,2,2,2,2,2,2,2,2,2,2,2,2,2,2,2,2,2,2,4),(-4.03619647859404,
-4.00809560787024,-4.00448225059761,-4.00202961525425,-4.00000131875697,
-3.99805863747667,-3.99555167918774,-3.99121004393426,-3.97419108135287,
-3.97153499754223,-3.95858297357044,-3.91144482001015,-3.85027590673282,
-3.84248202592952,-3.84029403739073,-3.83896400863578,-3.83775209233207,
-3.83616637406576,-3.83266647616008,-3.77540646349739,-3.7262991672328,
-3.70047909168305,-3.69061502854576,-3.68569640163624,-3.68162020687213,
-3.67921365188643,-3.67920325006476,-3.67919269124366,-3.67918197277497,
-3.67917109195598,-3.67916004607431,-3.67914883235244,-3.6791374479344,
-3.67912588994352,-3.67911415545363,-3.67910224146535,-3.67909014493247,
-3.6790778627553,-3.67906539177035,-3.6790527287561,-3.6790398704526,-3.67902681353936,
-3.67901355459893,-3.67900009018701,-3.6789864166821,-3.67897268481082,
-3.67895802553466,-3.6789423755487,-3.67892566713863,-3.67890782795825,
-3.67674380707064,-3.67397297347634,-3.6680914963686,-3.61764329708662,
-3.5629577084575,-3.52519736541063,-3.52088099693056,-3.51913529924332,
-3.51790067272656,-3.51677258600318,-3.51523195235049,-3.51218254848548,
-3.48396307303133,-3.39891886334032,-3.3774930570738,-3.36885471474969,
-3.36438786215256,-3.36061713192714,-3.35828193829274,-3.35612484208294,
-3.35335910345943,-3.34765699647645,-3.27008450488472,-3.20884616877966,
-3.20104817914338,-3.19885982728458,-3.1975297444059,-3.19631789735988,
-3.19473242895523,-3.19205856183358,-3.17523020180477,-3.08041523800341,
-3.05747873455699,-3.04373049714645,-3.03983625825116,-3.03745477821521,
-3.03529739268434,-3.0325289217795,-3.02681273198776,-2.94973204157224,
-2.88806015314576,-2.88023589715105,-2.87804497313629,-2.87671433692944,
-2.87550270319164,-2.87391847662165,-2.87042634739002,-2.8128213530936,
-2.76383108936271,-2.73816152981094,-2.72324021783761,-2.71923333894717,
-2.71682661077525,-2.71467416823324,-2.71282346300387),.UNSPECIFIED.);
#7734=B_SPLINE_CURVE_WITH_KNOTS('',3,(#65805,#65806,#65807,#65808,#65809,
#65810,#65811,#65812,#65813,#65814,#65815,#65816,#65817,#65818,#65819,#65820,
#65821,#65822,#65823,#65824,#65825,#65826,#65827,#65828,#65829,#65830,#65831,
#65832,#65833,#65834,#65835,#65836,#65837,#65838,#65839,#65840,#65841,#65842,
#65843,#65844,#65845,#65846,#65847,#65848,#65849,#65850,#65851,#65852,#65853,
#65854,#65855,#65856,#65857,#65858,#65859,#65860,#65861,#65862,#65863,#65864,
#65865,#65866,#65867,#65868,#65869,#65870,#65871,#65872,#65873,#65874,#65875,
#65876,#65877,#65878,#65879,#65880,#65881,#65882,#65883,#65884,#65885,#65886,
#65887,#65888,#65889,#65890,#65891,#65892,#65893,#65894,#65895,#65896,#65897,
#65898,#65899,#65900,#65901,#65902,#65903,#65904,#65905,#65906,#65907,#65908,
#65909,#65910,#65911,#65912,#65913,#65914,#65915,#65916,#65917,#65918,#65919,
#65920,#65921,#65922,#65923,#65924,#65925,#65926,#65927,#65928,#65929,#65930,
#65931,#65932,#65933,#65934,#65935,#65936,#65937,#65938,#65939,#65940,#65941,
#65942,#65943,#65944,#65945,#65946),.UNSPECIFIED.,.F.,.F.,(4,3,3,3,3,3,
3,3,3,3,3,3,3,3,3,3,3,3,3,3,3,3,3,3,3,3,3,3,3,3,3,3,3,3,3,3,3,3,3,3,3,3,
3,3,3,3,3,4),(72.2566310325656,72.2837016155711,72.37677692404,72.4697261751215,
72.5625770014511,72.6553600068939,72.7481078615374,72.8408453878106,72.9335973930147,
73.0264485919267,73.1193516100891,73.2124099513025,73.2832167540979,73.3762920625668,
73.4692413136484,73.5620921399779,73.6548751454206,73.7476230000642,73.8403605263374,
73.9331125315415,74.0259637304535,74.1188667486159,74.2119250898294,74.2827318926246,
74.3758072010935,74.468756452175,74.5616072785045,74.6543902839473,74.7471381385908,
74.839875664864,74.9326276700682,75.0254788689801,75.1183818871425,75.211440228356,
75.2822470311514,75.3753223396203,75.4682715907019,75.5611224170314,75.6539054224742,
75.7466532771177,75.8393908033909,75.9321428085951,76.0249940075071,76.1178970256695,
76.210955366883,76.2817621696781,76.374851433623,76.380801467099),
 .UNSPECIFIED.);
#7735=B_SPLINE_CURVE_WITH_KNOTS('',3,(#65947,#65948,#65949,#65950,#65951,
#65952),.UNSPECIFIED.,.F.,.F.,(4,1,1,4),(70.0962929016582,70.2846713385176,
71.2841864770443,72.2566272414748),.UNSPECIFIED.);
#7736=B_SPLINE_CURVE_WITH_KNOTS('',3,(#65953,#65954,#65955,#65956,#65957,
#65958,#65959,#65960,#65961,#65962,#65963,#65964,#65965,#65966,#65967,#65968,
#65969,#65970,#65971,#65972,#65973,#65974,#65975,#65976,#65977,#65978,#65979,
#65980,#65981,#65982,#65983,#65984,#65985,#65986,#65987,#65988,#65989,#65990,
#65991,#65992,#65993,#65994,#65995,#65996,#65997,#65998,#65999,#66000,#66001,
#66002,#66003,#66004,#66005,#66006,#66007,#66008,#66009,#66010,#66011,#66012,
#66013,#66014,#66015,#66016,#66017,#66018,#66019,#66020,#66021,#66022,#66023,
#66024,#66025,#66026,#66027,#66028,#66029,#66030,#66031,#66032,#66033,#66034,
#66035,#66036,#66037,#66038,#66039,#66040,#66041,#66042,#66043,#66044,#66045,
#66046,#66047,#66048,#66049,#66050,#66051,#66052,#66053,#66054,#66055,#66056,
#66057,#66058,#66059,#66060,#66061,#66062,#66063,#66064,#66065,#66066,#66067,
#66068,#66069,#66070,#66071,#66072,#66073,#66074,#66075,#66076,#66077,#66078,
#66079,#66080,#66081,#66082,#66083,#66084,#66085,#66086,#66087,#66088,#66089,
#66090,#66091,#66092,#66093,#66094,#66095,#66096,#66097,#66098,#66099,#66100,
#66101,#66102,#66103,#66104,#66105,#66106,#66107,#66108,#66109,#66110,#66111,
#66112,#66113,#66114,#66115,#66116,#66117,#66118,#66119,#66120,#66121,#66122,
#66123,#66124,#66125,#66126,#66127,#66128,#66129,#66130,#66131,#66132,#66133,
#66134,#66135,#66136,#66137,#66138,#66139,#66140,#66141,#66142,#66143,#66144,
#66145,#66146,#66147,#66148,#66149,#66150,#66151,#66152,#66153,#66154,#66155,
#66156,#66157,#66158,#66159,#66160,#66161,#66162,#66163,#66164,#66165,#66166,
#66167,#66168,#66169,#66170,#66171,#66172,#66173,#66174,#66175,#66176,#66177,
#66178,#66179,#66180,#66181,#66182,#66183,#66184,#66185,#66186,#66187,#66188,
#66189,#66190,#66191,#66192,#66193,#66194,#66195,#66196,#66197,#66198),
 .UNSPECIFIED.,.F.,.F.,(4,2,2,2,2,2,2,2,2,2,2,2,2,2,2,2,2,2,2,2,2,2,2,2,
2,2,2,2,2,2,2,2,2,2,2,2,2,2,2,2,2,2,2,2,2,2,2,2,2,2,2,2,2,2,2,2,2,2,2,2,
2,2,2,2,2,2,2,2,2,2,2,2,2,2,2,2,2,2,2,2,2,2,2,2,2,2,2,2,2,2,2,2,2,2,2,2,
2,2,2,2,2,2,2,2,2,2,2,2,2,2,2,2,2,2,2,2,2,2,2,2,2,2,4),(-2.71282346300387,
-2.71195001267204,-2.70766508087925,-2.68614652012974,-2.59027107316476,
-2.57026216330264,-2.5598826085674,-2.55747199598722,-2.55609227919899,
-2.55489080165277,-2.55336498530999,-2.55036438706897,-2.53213835472559,
-2.53155062342198,-2.49852763948949,-2.41412170693746,-2.40185705050541,
-2.39811859083517,-2.39577148623095,-2.393604037411,-2.3908111081901,-2.38619997321621,
-2.35901042891315,-2.34699181388133,-2.3450678046571,-2.34442344452801,
-2.27062411729961,-2.24980866519993,-2.23914361759669,-2.2367120766484,
-2.23532774382593,-2.23412686365069,-2.23260779242953,-2.22963857897059,
-2.21210268904967,-2.20809273471183,-2.11706870009749,-2.09477709593845,
-2.08131325677669,-2.07744730149775,-2.07507189348216,-2.07291263164853,
-2.07013141496413,-2.06435157391243,-2.01943223056741,-1.94998010095846,
-1.9404679404936,-1.91955881753204,-1.91640663883009,-1.91487075813651,
-1.91366840032819,-1.91229549358337,-1.90991540464985,-1.89993594979191,
-1.88103433376462,-1.77069743540713,-1.767724277275,-1.75931203894651,-1.75597457548543,
-1.7539409924426,-1.75176026778187,-1.74883201311585,-1.74227081926397,
-1.73349895408688,-1.71160660346678,-1.6230273179456,-1.59881209953064,
-1.59554106945206,-1.59399853115264,-1.59279267210641,-1.59143966663562,
-1.58914870702585,-1.58024989926437,-1.56419027039911,-1.54003092374437,
-1.48200758979014,-1.46790802729868,-1.44185251571303,-1.43730028268749,
-1.43452493998363,-1.43236023742578,-1.43000513236345,-1.42623009320188,
-1.41363054025839,-1.39324757705729,-1.37106249507141,-1.29548306605084,
-1.27775242624812,-1.27477340730196,-1.27325229440039,-1.27205132246873,
-1.2706685888863,-1.26824400916414,-1.25767293758014,-1.23712697205462,
-1.16679448607912,-1.12228766638433,-1.11651573685802,-1.11373608906869,
-1.11157704807818,-1.10920087608156,-1.10533141352298,-1.09183287044736,
-1.06945994169842,-0.977920863755642,-0.957170174292333,-0.954024060577004,
-0.95248930389804,-0.951286960949317,-0.949913110514963,-0.947529108902472,
-0.937500993239768,-0.918467300685122,-0.85724353276297,-0.801741171713293,
-0.796398138609899,-0.793664512253074,-0.791645723315301,-0.789453630618654,
-0.786461699382029,-0.779546580694334,-0.723083846394838,-0.696237685186134),
 .UNSPECIFIED.);
#7737=B_SPLINE_CURVE_WITH_KNOTS('',3,(#66204,#66205,#66206,#66207,#66208,
#66209,#66210,#66211,#66212,#66213,#66214,#66215,#66216,#66217,#66218,#66219,
#66220,#66221,#66222,#66223,#66224,#66225,#66226,#66227,#66228,#66229,#66230,
#66231,#66232,#66233,#66234,#66235,#66236,#66237,#66238,#66239,#66240,#66241,
#66242,#66243,#66244,#66245,#66246,#66247,#66248,#66249,#66250,#66251,#66252,
#66253,#66254,#66255,#66256,#66257,#66258,#66259,#66260,#66261,#66262,#66263,
#66264,#66265,#66266,#66267,#66268,#66269,#66270,#66271,#66272,#66273,#66274,
#66275,#66276,#66277,#66278,#66279,#66280,#66281,#66282,#66283,#66284,#66285,
#66286,#66287,#66288,#66289,#66290,#66291,#66292,#66293,#66294,#66295,#66296,
#66297,#66298,#66299,#66300,#66301,#66302,#66303,#66304,#66305,#66306,#66307,
#66308,#66309,#66310,#66311,#66312,#66313,#66314,#66315,#66316,#66317,#66318,
#66319,#66320,#66321,#66322,#66323,#66324,#66325,#66326,#66327,#66328,#66329,
#66330,#66331,#66332,#66333,#66334,#66335,#66336,#66337,#66338,#66339,#66340,
#66341,#66342),.UNSPECIFIED.,.F.,.F.,(4,3,3,3,3,3,3,3,3,3,3,3,3,3,3,3,3,
3,3,3,3,3,3,3,3,3,3,3,3,3,3,3,3,3,3,3,3,3,3,3,3,3,3,3,3,3,4),(78.5398163397452,
78.6323777454344,78.7241557666759,78.8159095945813,78.9076650481199,79.0008256824045,
79.0927135108167,79.1865105480376,79.2803075852584,79.3733828937274,79.4663321448089,
79.5591829711384,79.6519659765812,79.7447138312248,79.837451357498,79.9302033627021,
80.023054561614,80.1159575797763,80.2090159209898,80.2798227237852,80.3728980322541,
80.4658472833355,80.5586981096652,80.6514811151079,80.7442289697515,80.8369664960247,
80.929718501229,81.022569700141,81.1154727183036,81.2085310595171,81.2793378623119,
81.3724131707809,81.4653624218621,81.5582132481916,81.6509962536344,81.7437441082779,
81.8364816345511,81.9292336397553,82.0220848386673,82.1149878568298,82.2080461980432,
82.2788530008387,82.375109601286,82.4680451601066,82.5608939237312,82.6536708061284,
82.663879402628),.UNSPECIFIED.);
#7738=B_SPLINE_CURVE_WITH_KNOTS('',3,(#66343,#66344,#66345,#66346,#66347,
#66348,#66349,#66350,#66351,#66352,#66353,#66354,#66355,#66356,#66357,#66358,
#66359,#66360,#66361,#66362,#66363,#66364,#66365,#66366,#66367,#66368,#66369,
#66370,#66371,#66372,#66373,#66374,#66375,#66376,#66377,#66378,#66379,#66380,
#66381,#66382,#66383,#66384,#66385,#66386,#66387,#66388,#66389,#66390,#66391,
#66392,#66393,#66394,#66395,#66396,#66397,#66398,#66399,#66400,#66401,#66402,
#66403,#66404,#66405,#66406,#66407,#66408,#66409,#66410,#66411,#66412,#66413,
#66414,#66415),.UNSPECIFIED.,.F.,.F.,(4,3,3,3,3,3,3,3,3,3,3,3,3,3,3,3,3,
3,3,3,3,3,3,3,4),(76.380801467099,76.4737435786687,76.5665890335125,76.6593690393854,
76.7521154870988,76.8448531975143,76.9376069776423,77.0304608283556,77.1233679280772,
77.2164285534006,77.2812773082049,77.3743526166739,77.4673018677554,77.5601526940849,
77.6529356995276,77.7456835541712,77.8384210804444,77.9311730856486,78.0240242845606,
78.116927302723,78.2099856439365,78.2807924467317,78.4009736434012,78.5186931112108,
78.5398163394889),.UNSPECIFIED.);
#7739=B_SPLINE_CURVE_WITH_KNOTS('',3,(#66417,#66418,#66419,#66420,#66421,
#66422,#66423,#66424,#66425,#66426,#66427,#66428,#66429,#66430,#66431,#66432,
#66433,#66434,#66435,#66436,#66437,#66438,#66439,#66440,#66441,#66442,#66443,
#66444,#66445,#66446,#66447,#66448,#66449,#66450,#66451,#66452,#66453,#66454,
#66455,#66456,#66457,#66458,#66459,#66460,#66461,#66462,#66463,#66464,#66465,
#66466,#66467,#66468,#66469,#66470,#66471,#66472,#66473,#66474,#66475,#66476,
#66477,#66478,#66479,#66480,#66481,#66482,#66483,#66484,#66485,#66486,#66487,
#66488,#66489,#66490,#66491,#66492,#66493,#66494,#66495,#66496,#66497,#66498,
#66499,#66500,#66501,#66502,#66503,#66504,#66505,#66506,#66507,#66508,#66509,
#66510,#66511,#66512,#66513,#66514,#66515,#66516,#66517,#66518,#66519,#66520,
#66521,#66522,#66523,#66524,#66525,#66526,#66527,#66528,#66529,#66530,#66531,
#66532,#66533,#66534,#66535,#66536,#66537,#66538,#66539,#66540,#66541,#66542,
#66543,#66544,#66545,#66546,#66547,#66548,#66549,#66550,#66551,#66552,#66553,
#66554,#66555,#66556,#66557,#66558,#66559,#66560,#66561,#66562,#66563,#66564,
#66565,#66566,#66567,#66568,#66569,#66570,#66571,#66572,#66573,#66574,#66575,
#66576,#66577,#66578),.UNSPECIFIED.,.F.,.F.,(4,2,2,2,2,2,2,2,2,2,2,2,2,
2,2,2,2,2,2,2,2,2,2,2,2,2,2,2,2,2,2,2,2,2,2,2,2,2,2,2,2,2,2,2,2,2,2,2,2,
2,2,2,2,2,2,2,2,2,2,2,2,2,2,2,2,2,2,2,2,2,2,2,2,2,2,2,2,2,2,2,4),(-0.696237685186134,
-0.675519558018449,-0.63707121428382,-0.633868815383757,-0.632289699751432,
-0.631151450179954,-0.62994933489026,-0.628297395338522,-0.626437311549927,
-0.623224737378464,-0.59937290706623,-0.551993457336766,-0.480880591906853,
-0.475023217996447,-0.472256733081436,-0.470093047332004,-0.467733078494461,
-0.463937163530348,-0.451147023877335,-0.430349155678461,-0.37587278332947,
-0.348494934235186,-0.316229019233684,-0.312760130818892,-0.311180063771606,
-0.3100031458416,-0.309999456281614,-0.309995806463445,-0.309992189866261,
-0.309988606157959,-0.309985054915406,-0.309981535819848,-0.309978048491879,
-0.309974592527943,-0.309971167610816,-0.309967773405964,-0.309964409568612,
-0.309961075745882,-0.309957771642774,-0.309954496902071,-0.30995125121917,
-0.309948034197928,-0.309944845575585,-0.30994168509736,-0.309938552419312,
-0.309935447209036,-0.309932369207409,-0.309929318090706,-0.309926293635987,
-0.30992329550613,-0.309920323410833,-0.309917377125776,-0.309915182175273,
-0.309912971521832,-0.309910765262554,-0.309908563412812,-0.309906365965786,
-0.309904172890775,-0.309901984153585,-0.309899799744197,-0.309897619594419,
-0.309895443784985,-0.309893272298244,-0.30989110505302,-0.308550667851128,
-0.307131486242876,-0.304997177291619,-0.301101797104602,-0.292132144811765,
-0.262433051302041,-0.164279929548461,-0.162678479377572,-0.154449448137997,
-0.151129851316645,-0.149090120683716,-0.146889582561246,-0.143911480787282,
-0.137139189781584,-0.128027141416022,-0.104998842794788,-0.000961222373964137),
 .UNSPECIFIED.);
#7740=B_SPLINE_CURVE_WITH_KNOTS('',3,(#66579,#66580,#66581,#66582,#66583,
#66584,#66585,#66586,#66587,#66588,#66589,#66590,#66591,#66592,#66593,#66594,
#66595,#66596,#66597,#66598,#66599,#66600,#66601,#66602,#66603,#66604,#66605,
#66606,#66607,#66608,#66609,#66610,#66611,#66612,#66613,#66614,#66615,#66616,
#66617,#66618,#66619,#66620,#66621,#66622,#66623,#66624,#66625,#66626,#66627,
#66628,#66629,#66630,#66631,#66632,#66633,#66634,#66635,#66636,#66637,#66638,
#66639,#66640,#66641,#66642,#66643,#66644,#66645,#66646,#66647,#66648,#66649,
#66650,#66651,#66652,#66653,#66654,#66655,#66656,#66657,#66658,#66659,#66660,
#66661,#66662,#66663,#66664,#66665,#66666,#66667,#66668,#66669,#66670,#66671,
#66672,#66673,#66674,#66675,#66676,#66677,#66678,#66679,#66680,#66681,#66682,
#66683,#66684,#66685,#66686,#66687,#66688,#66689,#66690,#66691,#66692,#66693,
#66694,#66695,#66696,#66697,#66698,#66699,#66700,#66701,#66702,#66703,#66704,
#66705,#66706,#66707,#66708,#66709,#66710,#66711,#66712,#66713,#66714,#66715,
#66716,#66717,#66718,#66719,#66720,#66721,#66722,#66723,#66724,#66725,#66726,
#66727,#66728,#66729,#66730,#66731,#66732,#66733,#66734,#66735,#66736,#66737,
#66738,#66739,#66740,#66741,#66742,#66743,#66744,#66745,#66746,#66747,#66748,
#66749,#66750,#66751,#66752,#66753,#66754),.UNSPECIFIED.,.F.,.F.,(4,2,2,
2,2,2,2,2,2,2,2,2,2,2,2,2,2,2,2,2,2,2,2,2,2,2,2,2,2,2,2,2,2,2,2,2,2,2,2,
2,2,2,2,2,2,2,2,2,2,2,2,2,2,2,2,2,2,2,2,2,2,2,2,2,2,2,2,2,2,2,2,2,2,2,2,
2,2,2,2,2,2,2,2,2,2,2,2,4),(-4.05943779606569,-4.05345026639121,-4.04937125481813,
-4.04778731189876,-4.04658704028464,-4.04542945739733,-4.04427265622474,
-4.04231135777569,-4.03703563664029,-4.02875353085773,-3.95031088242969,
-3.92314694508256,-3.89313164899935,-3.88818239634357,-3.88556062224259,
-3.88340436345589,-3.88089933367909,-3.8766058757658,-3.86029037889877,
-3.85691847335429,-3.84967007276564,-3.83128400784498,-3.7578363111733,
-3.73768340141623,-3.73077027769674,-3.72754503646094,-3.7256764746319,
-3.72401795386332,-3.72280903317128,-3.7216637241096,-3.72007428244317,
-3.71684927119908,-3.67775103490949,-3.63533718282447,-3.57269258993827,
-3.56634300135146,-3.56344278369877,-3.56125578350722,-3.55919647411765,
-3.55577034916008,-3.54689076585914,-3.4449722742975,-3.40946946957931,
-3.4055134280881,-3.40335586861807,-3.40192725752373,-3.40058160606482,
-3.39940508476045,-3.39786762443795,-3.39473597666216,-3.37468828546699,
-3.28193568244436,-3.25930760931743,-3.24567235800386,-3.24177351831663,
-3.23938140286203,-3.23720925216673,-3.23441465623715,-3.22861866947255,
-3.15261089554197,-3.08915493135136,-3.08119750761457,-3.07898443646193,
-3.07764351047602,-3.07642474020449,-3.07483418114361,-3.07146685277802,
-3.04290505166636,-3.00097468545075,-2.92786175903349,-2.92093316603533,
-2.91792795207206,-2.91572328851612,-2.91369092657029,-2.91093587962425,
-2.90554190084967,-2.84431123868312,-2.79134437728056,-2.76985703612609,
-2.75893672734631,-2.75647660291086,-2.75508072570095,-2.75387277482531,
-2.75234856053968,-2.7493806904627,-2.73211639887814,-2.73136055880086,
-2.72791817214398),.UNSPECIFIED.);
#7741=B_SPLINE_CURVE_WITH_KNOTS('',3,(#66760,#66761,#66762,#66763,#66764,
#66765,#66766,#66767,#66768,#66769,#66770,#66771,#66772,#66773,#66774,#66775,
#66776,#66777,#66778,#66779,#66780,#66781,#66782,#66783,#66784,#66785,#66786,
#66787,#66788,#66789,#66790,#66791,#66792,#66793,#66794,#66795,#66796,#66797,
#66798,#66799,#66800,#66801,#66802,#66803,#66804,#66805,#66806,#66807,#66808,
#66809,#66810,#66811,#66812,#66813,#66814,#66815,#66816,#66817,#66818,#66819,
#66820,#66821,#66822,#66823,#66824,#66825,#66826,#66827,#66828,#66829,#66830,
#66831,#66832,#66833,#66834,#66835,#66836,#66837,#66838,#66839,#66840,#66841,
#66842,#66843,#66844,#66845,#66846,#66847,#66848,#66849,#66850,#66851,#66852,
#66853,#66854,#66855,#66856,#66857,#66858,#66859,#66860,#66861,#66862,#66863,
#66864,#66865,#66866,#66867,#66868,#66869,#66870,#66871,#66872,#66873,#66874,
#66875,#66876,#66877,#66878,#66879,#66880,#66881,#66882,#66883,#66884,#66885,
#66886,#66887,#66888,#66889,#66890,#66891,#66892,#66893,#66894,#66895,#66896,
#66897,#66898),.UNSPECIFIED.,.F.,.F.,(4,3,3,3,3,3,3,3,3,3,3,3,3,3,3,3,3,
3,3,3,3,3,3,3,3,3,3,3,3,3,3,3,3,3,3,3,3,3,3,3,3,3,3,3,3,3,4),(84.8230016471138,
84.9221960598312,85.0217585077651,85.1215123023174,85.2215704894812,85.277398416419,
85.3704737248879,85.4634229759694,85.5562738022989,85.6490568077416,85.7418046623852,
85.8345421886584,85.9272941938625,86.0201453927745,86.1130484109369,86.2061067521504,
86.2769135549458,86.3699888634147,86.4629381144963,86.5557889408258,86.6485719462685,
86.7413198009121,86.8340573271853,86.9268093323895,87.0196605313014,87.1125635494638,
87.2056218906773,87.2764286934725,87.3695040019414,87.4624532530229,87.5553040793525,
87.6480870847952,87.7408349394388,87.833572465712,87.9263244709162,88.0191756698281,
88.1120786879905,88.205137029204,88.2759438319993,88.3690008063904,88.461940195998,
88.5547870208806,88.6475662149387,88.740312112707,88.8330399906779,88.925793178824,
88.9462551936448),.UNSPECIFIED.);
#7742=B_SPLINE_CURVE_WITH_KNOTS('',3,(#66899,#66900,#66901,#66902,#66903,
#66904,#66905,#66906,#66907,#66908,#66909,#66910,#66911,#66912,#66913,#66914,
#66915,#66916,#66917,#66918,#66919,#66920,#66921,#66922,#66923,#66924,#66925,
#66926,#66927,#66928,#66929,#66930,#66931,#66932,#66933,#66934,#66935,#66936,
#66937,#66938,#66939,#66940,#66941,#66942,#66943,#66944,#66945,#66946,#66947,
#66948,#66949,#66950,#66951,#66952,#66953,#66954,#66955,#66956,#66957,#66958,
#66959,#66960,#66961,#66962,#66963,#66964,#66965,#66966,#66967,#66968,#66969,
#66970,#66971),.UNSPECIFIED.,.F.,.F.,(4,3,3,3,3,3,3,3,3,3,3,3,3,3,3,3,3,
3,3,3,3,3,3,3,4),(82.663879402628,82.756624238485,82.8493623215592,82.9421184586138,
83.034975745376,83.1278880647113,83.2209516972694,83.2783681393655,83.3714434478346,
83.4643926989164,83.5572435252462,83.6500265306889,83.7427743853325,83.8355119116059,
83.9282639168099,84.0211151157219,84.1140181338843,84.2070764750979,84.2778832778922,
84.3739789574075,84.4699157807353,84.5656692160942,84.6613146280951,84.7568461508212,
84.8230016469248),.UNSPECIFIED.);
#7743=B_SPLINE_CURVE_WITH_KNOTS('',3,(#66972,#66973,#66974,#66975,#66976,
#66977,#66978,#66979,#66980,#66981,#66982,#66983,#66984,#66985,#66986,#66987,
#66988,#66989,#66990,#66991,#66992,#66993,#66994,#66995,#66996,#66997,#66998,
#66999,#67000,#67001,#67002,#67003,#67004,#67005,#67006,#67007,#67008,#67009,
#67010,#67011,#67012,#67013,#67014,#67015,#67016,#67017,#67018,#67019,#67020,
#67021,#67022,#67023,#67024,#67025,#67026,#67027,#67028,#67029,#67030,#67031,
#67032,#67033,#67034,#67035,#67036,#67037,#67038,#67039,#67040,#67041,#67042,
#67043,#67044,#67045,#67046,#67047,#67048,#67049,#67050,#67051,#67052,#67053,
#67054,#67055,#67056,#67057,#67058,#67059,#67060,#67061,#67062,#67063,#67064,
#67065,#67066,#67067,#67068,#67069,#67070,#67071,#67072,#67073,#67074,#67075,
#67076,#67077,#67078,#67079,#67080,#67081,#67082,#67083,#67084,#67085,#67086,
#67087,#67088,#67089,#67090,#67091,#67092,#67093,#67094,#67095,#67096,#67097,
#67098,#67099,#67100,#67101,#67102,#67103,#67104,#67105,#67106,#67107,#67108,
#67109,#67110,#67111,#67112,#67113,#67114,#67115,#67116,#67117,#67118,#67119,
#67120,#67121,#67122,#67123,#67124,#67125,#67126,#67127,#67128,#67129,#67130,
#67131,#67132,#67133,#67134,#67135,#67136,#67137,#67138,#67139,#67140,#67141,
#67142,#67143,#67144,#67145,#67146,#67147,#67148,#67149,#67150,#67151,#67152,
#67153,#67154,#67155,#67156,#67157,#67158,#67159,#67160,#67161,#67162,#67163,
#67164,#67165,#67166,#67167,#67168,#67169,#67170,#67171,#67172,#67173,#67174,
#67175,#67176,#67177,#67178,#67179,#67180,#67181,#67182,#67183,#67184,#67185,
#67186,#67187,#67188,#67189,#67190,#67191,#67192,#67193,#67194,#67195,#67196,
#67197,#67198,#67199,#67200,#67201,#67202,#67203,#67204,#67205,#67206,#67207,
#67208,#67209,#67210,#67211,#67212,#67213,#67214,#67215),.UNSPECIFIED.,
 .F.,.F.,(4,2,2,2,2,2,2,2,2,2,2,2,2,2,2,2,2,2,2,2,2,2,2,2,2,2,2,2,2,2,2,
2,2,2,2,2,2,2,2,2,2,2,2,2,2,2,2,2,2,2,2,2,2,2,2,2,2,2,2,2,2,2,2,2,2,2,2,
2,2,2,2,2,2,2,2,2,2,2,2,2,2,2,2,2,2,2,2,2,2,2,2,2,2,2,2,2,2,2,2,2,2,2,2,
2,2,2,2,2,2,2,2,2,2,2,2,2,2,2,2,2,2,4),(-2.72791817214398,-2.72757626591806,
-2.63606423622718,-2.61364743619176,-2.60010597703889,-2.59621670021499,
-2.59382673984744,-2.59165410327153,-2.58885545353705,-2.58303863684278,
-2.53777278075375,-2.46757445614939,-2.4468006529931,-2.43612968947032,
-2.43368754860676,-2.4322956772014,-2.4310873152038,-2.42955755808693,-2.42656376975906,
-2.40879609562139,-2.40362799523738,-2.36164703988015,-2.31387673393604,
-2.29115522479557,-2.27747843013807,-2.27357525369854,-2.27118208793889,
-2.26901004012297,-2.26621705573284,-2.26042974982179,-2.18406065452215,
-2.13955489082282,-2.12253517903094,-2.11324633531875,-2.11091222739375,
-2.10954426436202,-2.10833205980341,-2.10676469062215,-2.10348165207084,
-2.0793708307666,-2.07038120131137,-2.03098267213065,-2.00150754288925,
-1.98320508308051,-1.9569259361281,-1.95234162313692,-1.94954767734819,
-1.94736904150918,-1.94499935936886,-1.94120222235277,-1.9285404958871,
-1.90806703907829,-1.86348636951593,-1.85221772371789,-1.79250429774525,
-1.78936577225568,-1.78779773404084,-1.78665788573919,-1.78541928043255,
-1.78368315126966,-1.77946496675649,-1.77353820369554,-1.75739282920614,
-1.73312304476404,-1.67426543170373,-1.66107005697728,-1.65678086589297,
-1.63388940415156,-1.62949949223706,-1.62673412195209,-1.62456520901261,
-1.62215669461167,-1.618185424533,-1.60382042053993,-1.57951830025907,-1.47524112956354,
-1.46763106527624,-1.46535938045523,-1.46400507216974,-1.46291118894332,
-1.46138455471068,-1.45830817447062,-1.43196075869977,-1.38442482316929,
-1.31258924828251,-1.30669155012857,-1.30390667812202,-1.30172889928891,
-1.29935385059284,-1.2955343206081,-1.28267057289477,-1.26175827083863,
-1.18787387231184,-1.14697220243633,-1.14373246823237,-1.14213897733664,
-1.14099222527729,-1.13975828868846,-1.1380491629104,-1.13399267647375,
-1.12835480743113,-1.05489408021853,-0.989838763503215,-0.984451155629457,
-0.98169725921509,-0.979664731717884,-0.977458909751686,-0.974450370147237,
-0.967506352156097,-0.958102665041172,-0.934031818129519,-0.831849242160278,
-0.822171057473247,-0.819712181452299,-0.818301385567433,-0.817094137215332,
-0.815588126430419,-0.812613955076298,-0.790352774030541,-0.752809828950054,
-0.72170275952839,-0.698709454689423),.UNSPECIFIED.);
#7744=B_SPLINE_CURVE_WITH_KNOTS('',3,(#67221,#67222,#67223,#67224,#67225,
#67226,#67227,#67228,#67229,#67230,#67231,#67232,#67233,#67234,#67235,#67236,
#67237,#67238,#67239,#67240,#67241,#67242,#67243,#67244,#67245,#67246,#67247,
#67248,#67249,#67250,#67251,#67252,#67253,#67254,#67255,#67256,#67257,#67258,
#67259,#67260,#67261,#67262,#67263,#67264,#67265,#67266,#67267,#67268,#67269,
#67270,#67271,#67272,#67273,#67274,#67275,#67276,#67277,#67278,#67279,#67280,
#67281,#67282,#67283,#67284,#67285,#67286,#67287,#67288,#67289,#67290,#67291,
#67292,#67293,#67294,#67295,#67296,#67297,#67298,#67299,#67300,#67301,#67302,
#67303,#67304,#67305,#67306,#67307,#67308,#67309,#67310,#67311,#67312,#67313,
#67314,#67315,#67316,#67317,#67318,#67319,#67320,#67321,#67322,#67323,#67324,
#67325,#67326,#67327,#67328,#67329,#67330,#67331,#67332,#67333,#67334,#67335,
#67336,#67337,#67338,#67339,#67340,#67341,#67342,#67343,#67344,#67345,#67346,
#67347,#67348,#67349,#67350,#67351,#67352,#67353,#67354,#67355,#67356,#67357,
#67358,#67359),.UNSPECIFIED.,.F.,.F.,(4,3,3,3,3,3,3,3,3,3,3,3,3,3,3,3,3,
3,3,3,3,3,3,3,3,3,3,3,3,3,3,3,3,3,3,3,3,3,3,3,3,3,3,3,3,3,4),(91.1061869541044,
91.2531720643649,91.2744892475796,91.3675645560485,91.46051380713,91.5533646334596,
91.6461476389023,91.7388954935459,91.8316330198191,91.9243850250232,92.0172362239352,
92.1101392420976,92.2031975833111,92.2740043861063,92.3670796945753,92.4600289456567,
92.5528797719863,92.6456627774291,92.7384106320726,92.8311481583459,92.9239001635501,
93.0167513624621,93.1096543806244,93.2027127218379,93.2735195246331,93.366594833102,
93.4595440841836,93.5523949105131,93.6451779159559,93.7379257705994,93.8306632968727,
93.9234153020768,94.0162665009888,94.1091695191512,94.2022278603647,94.2730346631599,
94.3661126845117,94.4590639501153,94.5553905369303,94.6481700190462,94.7409142923435,
94.8336481781563,94.9263964823739,95.0192322633309,95.11212029076,95.2051350095969,
95.2296766446352),.UNSPECIFIED.);
#7745=B_SPLINE_CURVE_WITH_KNOTS('',3,(#67360,#67361,#67362,#67363,#67364,
#67365,#67366,#67367,#67368,#67369,#67370,#67371,#67372,#67373,#67374,#67375,
#67376,#67377,#67378,#67379,#67380,#67381,#67382,#67383,#67384,#67385,#67386,
#67387,#67388,#67389,#67390,#67391,#67392,#67393,#67394,#67395,#67396,#67397,
#67398,#67399,#67400,#67401,#67402,#67403,#67404,#67405,#67406,#67407,#67408,
#67409,#67410,#67411,#67412,#67413,#67414,#67415,#67416,#67417,#67418,#67419,
#67420,#67421,#67422,#67423,#67424,#67425,#67426,#67427,#67428,#67429,#67430,
#67431,#67432),.UNSPECIFIED.,.F.,.F.,(4,3,3,3,3,3,3,3,3,3,3,3,3,3,3,3,3,
3,3,3,3,3,3,3,4),(88.9462551936448,89.0391158747113,89.1320332819789,89.2250999323282,
89.2754589705261,89.368534278995,89.4614835300766,89.5543343564061,89.6471173618489,
89.7398652164924,89.8326027427657,89.9253547479699,90.0182059468818,90.1111089650442,
90.2041673062577,90.2749741090528,90.3666596755061,90.4591005853075,90.5505540119022,
90.6419502073382,90.7333153498863,90.8265332508942,90.9179528502677,91.0120699020928,
91.1061869539178),.UNSPECIFIED.);
#7746=B_SPLINE_CURVE_WITH_KNOTS('',3,(#67434,#67435,#67436,#67437,#67438,
#67439,#67440,#67441,#67442,#67443,#67444,#67445,#67446,#67447,#67448,#67449,
#67450,#67451,#67452,#67453,#67454,#67455,#67456,#67457,#67458,#67459,#67460,
#67461,#67462,#67463,#67464,#67465,#67466,#67467,#67468,#67469,#67470,#67471,
#67472,#67473,#67474,#67475,#67476,#67477,#67478,#67479,#67480,#67481,#67482,
#67483,#67484,#67485,#67486,#67487,#67488,#67489,#67490,#67491,#67492,#67493,
#67494,#67495,#67496,#67497,#67498,#67499,#67500,#67501,#67502,#67503,#67504,
#67505,#67506,#67507,#67508,#67509,#67510,#67511,#67512,#67513,#67514,#67515,
#67516,#67517,#67518,#67519,#67520,#67521,#67522,#67523,#67524,#67525,#67526,
#67527,#67528,#67529),.UNSPECIFIED.,.F.,.F.,(4,2,2,2,2,2,2,2,2,2,2,2,2,
2,2,2,2,2,2,2,2,2,2,2,2,2,2,2,2,2,2,2,2,2,2,2,2,2,2,2,2,2,2,2,2,2,2,4),
(-0.698709454689423,-0.666843047260533,-0.661476341095949,-0.65872745721161,
-0.656695869584792,-0.654533359844537,-0.651607160765785,-0.648348827884347,
-0.642816925899491,-0.60419136741942,-0.522692176465372,-0.518714738765864,
-0.500239647899331,-0.49721286352588,-0.495675406849351,-0.494465613389275,
-0.493077291147427,-0.490653923314244,-0.480253064841465,-0.460248997720133,
-0.432060003842914,-0.393483763796674,-0.343849805060601,-0.337942919617727,
-0.335155682029959,-0.333024184723614,-0.330711578533513,-0.328309636399378,
-0.324834993657877,-0.318771010917819,-0.272728776753478,-0.221750380227524,
-0.178215503478459,-0.174605378645141,-0.172992857261096,-0.17177004161356,
-0.170438198229673,-0.16826830305091,-0.160748296120402,-0.104322696345831,
-0.0266090166975272,-0.0167918801592759,-0.0132205824828429,-0.0111319304901992,
-0.00903511934187455,-0.00692965682314765,-0.00390544029746683,-0.000960255622328456),
 .UNSPECIFIED.);
#7747=B_SPLINE_CURVE_WITH_KNOTS('',3,(#67530,#67531,#67532,#67533,#67534,
#67535,#67536,#67537,#67538,#67539,#67540,#67541,#67542,#67543,#67544,#67545,
#67546,#67547,#67548,#67549,#67550,#67551,#67552,#67553,#67554,#67555,#67556,
#67557,#67558,#67559,#67560,#67561,#67562,#67563,#67564,#67565,#67566,#67567,
#67568,#67569,#67570,#67571,#67572,#67573,#67574,#67575,#67576,#67577,#67578,
#67579,#67580,#67581,#67582,#67583,#67584,#67585,#67586,#67587,#67588,#67589,
#67590,#67591,#67592,#67593,#67594,#67595,#67596,#67597,#67598,#67599,#67600,
#67601,#67602,#67603,#67604,#67605,#67606,#67607,#67608,#67609,#67610,#67611,
#67612,#67613,#67614,#67615,#67616,#67617,#67618,#67619,#67620,#67621,#67622,
#67623,#67624,#67625,#67626,#67627,#67628,#67629,#67630,#67631,#67632,#67633,
#67634,#67635,#67636,#67637,#67638,#67639,#67640,#67641,#67642,#67643,#67644,
#67645,#67646,#67647,#67648,#67649,#67650,#67651,#67652,#67653,#67654,#67655,
#67656,#67657,#67658,#67659,#67660,#67661,#67662,#67663,#67664,#67665,#67666,
#67667,#67668,#67669,#67670,#67671,#67672,#67673,#67674,#67675,#67676,#67677,
#67678,#67679,#67680,#67681,#67682,#67683,#67684,#67685,#67686,#67687,#67688,
#67689,#67690,#67691,#67692,#67693,#67694,#67695,#67696,#67697,#67698,#67699,
#67700,#67701,#67702,#67703,#67704,#67705,#67706,#67707,#67708,#67709,#67710,
#67711,#67712,#67713,#67714,#67715,#67716,#67717,#67718,#67719,#67720,#67721,
#67722,#67723,#67724,#67725,#67726,#67727,#67728,#67729,#67730,#67731,#67732,
#67733,#67734,#67735,#67736,#67737,#67738,#67739,#67740,#67741,#67742,#67743,
#67744,#67745),.UNSPECIFIED.,.F.,.F.,(4,2,2,2,2,2,2,2,2,2,2,2,2,2,2,2,2,
2,2,2,2,2,2,2,2,2,2,2,2,2,2,2,2,2,2,2,2,2,2,2,2,2,2,2,2,2,2,2,2,2,2,2,2,
2,2,2,2,2,2,2,2,2,2,2,2,2,2,2,2,2,2,2,2,2,2,2,2,2,2,2,2,2,2,2,2,2,2,2,2,
2,2,2,2,2,2,2,2,2,2,2,2,2,2,2,2,2,2,4),(-4.07343079861933,-4.05868086012299,
-4.00070276921845,-3.94757887152325,-3.93322662474479,-3.92499404069726,
-3.92274888238868,-3.92139757638515,-3.92017571218205,-3.91858954295225,
-3.91513791088693,-3.88524540260387,-3.84114529928722,-3.76918518529934,
-3.76518640952024,-3.76256311752847,-3.76009117896046,-3.76007768496206,
-3.76006641279559,-3.76005478721725,-3.76004279342015,-3.76003041574761,
-3.76001763766328,-3.76000444167587,-3.75999080921395,-3.75997672065096,
-3.7599621551369,-3.75994709050131,-3.75993150320342,-3.75991536818062,
-3.75989865870716,-3.75988134626247,-3.75986340042684,-3.75984478867069,
-3.75982547613537,-3.75980542545279,-3.75978459651623,-3.7597629461998,
-3.75974042808431,-3.75971699210076,-3.75969258416886,-3.75966714577552,
-3.75964061362145,-3.75961407793517,-3.75747458745472,-3.75467131028805,
-3.74903269843729,-3.67049183693619,-3.62629931062385,-3.61011557126601,
-3.60417269546198,-3.59994234018484,-3.5982003266796,-3.59695721127157,
-3.59581297562757,-3.59423857414969,-3.5910863099696,-3.53129239165828,
-3.48233396966627,-3.44807027094141,-3.44286467798937,-3.43973730486539,
-3.43690281053057,-3.43475000691286,-3.43268445406497,-3.42925470231979,
-3.42040355244149,-3.41907416512816,-3.33567645248822,-3.29983126820865,
-3.28534028525411,-3.27705013432687,-3.27479938695166,-3.27344676232086,
-3.27222512888126,-3.27064114535644,-3.26800028572343,-3.25221357285803,
-3.18228815148936,-3.12209639384945,-3.11578947928084,-3.11289038014352,
-3.11069660767051,-3.10862529989861,-3.10573986943086,-3.09821343094713,
-3.09470483027559,-3.01714854722788,-2.96042814404654,-2.95287698461928,
-2.95069935961224,-2.9493630513823,-2.94813633708804,-2.94651895044135,
-2.94289906091532,-2.89964953477856,-2.88756018818637,-2.82321089587945,
-2.79577825945987,-2.79092530355689,-2.78831755263476,-2.78617382284054,
-2.78364519987737,-2.77927657401761,-2.76227589742534,-2.75942583678824,
-2.7523504486624,-2.73686895463578),.UNSPECIFIED.);
#7748=B_SPLINE_CURVE_WITH_KNOTS('',3,(#67751,#67752,#67753,#67754,#67755,
#67756,#67757,#67758,#67759,#67760,#67761,#67762,#67763,#67764,#67765,#67766,
#67767,#67768,#67769,#67770,#67771,#67772,#67773,#67774,#67775,#67776,#67777,
#67778,#67779,#67780,#67781,#67782,#67783,#67784,#67785,#67786,#67787,#67788,
#67789,#67790,#67791,#67792,#67793,#67794,#67795,#67796,#67797,#67798,#67799,
#67800,#67801,#67802,#67803,#67804,#67805,#67806,#67807,#67808,#67809,#67810,
#67811,#67812,#67813,#67814,#67815,#67816,#67817,#67818,#67819,#67820,#67821,
#67822,#67823,#67824,#67825,#67826,#67827,#67828,#67829,#67830,#67831,#67832,
#67833,#67834,#67835,#67836,#67837,#67838,#67839,#67840,#67841,#67842,#67843,
#67844,#67845,#67846,#67847,#67848,#67849,#67850,#67851,#67852,#67853,#67854,
#67855,#67856,#67857,#67858,#67859,#67860,#67861,#67862,#67863,#67864,#67865,
#67866,#67867,#67868,#67869,#67870,#67871,#67872,#67873,#67874,#67875,#67876,
#67877,#67878,#67879,#67880,#67881,#67882,#67883,#67884,#67885,#67886,#67887,
#67888,#67889),.UNSPECIFIED.,.F.,.F.,(4,3,3,3,3,3,3,3,3,3,3,3,3,3,3,3,3,
3,3,3,3,3,3,3,3,3,3,3,3,3,3,3,3,3,3,3,3,3,3,3,3,3,3,3,3,3,4),(97.389372261552,
97.4811078775329,97.5727347819261,97.6642817274812,97.7557867563104,97.8472759289302,
97.9387752853951,98.0303675879002,98.1220101752803,98.2138004326156,98.2710952172669,
98.3641705257358,98.4571197768173,98.5499706031467,98.6427536085893,98.7355014632329,
98.828238989506,98.9209909947099,99.0138421936218,99.1067452117843,99.1998035529977,
99.2706103557937,99.3636856642626,99.4566349153438,99.5494857416735,99.6422687471163,
99.7350166017598,99.8277541280328,99.9205061332367,100.013357332149,100.106260350311,
100.199318691524,100.27012549432,100.363200802789,100.45615005387,100.5490008802,
100.641783885643,100.734531740286,100.827269266559,100.920021271764,101.012872470675,
101.105775488838,101.198833830051,101.269640632847,101.362717406679,101.455655050019,
101.513685257635),.UNSPECIFIED.);
#7749=B_SPLINE_CURVE_WITH_KNOTS('',3,(#67890,#67891,#67892,#67893,#67894,
#67895,#67896,#67897,#67898,#67899,#67900,#67901,#67902,#67903,#67904,#67905,
#67906,#67907,#67908,#67909,#67910,#67911,#67912,#67913,#67914,#67915,#67916,
#67917,#67918,#67919,#67920,#67921,#67922,#67923,#67924,#67925,#67926,#67927,
#67928,#67929,#67930,#67931,#67932,#67933,#67934,#67935,#67936,#67937,#67938,
#67939,#67940,#67941,#67942,#67943,#67944,#67945,#67946,#67947,#67948,#67949,
#67950,#67951,#67952,#67953,#67954,#67955,#67956,#67957,#67958,#67959,#67960,
#67961,#67962),.UNSPECIFIED.,.F.,.F.,(4,3,3,3,3,3,3,3,3,3,3,3,3,3,3,3,3,
3,3,3,3,3,3,3,4),(95.2296766446352,95.2725498016866,95.3656251101555,95.4585743612371,
95.5514251875666,95.6442081930094,95.736956047653,95.8296935739262,95.9224455791303,
96.0152967780422,96.1081997962046,96.2012581374181,96.2720649402134,96.3651402486823,
96.458089499764,96.5509403260934,96.6437233315362,96.7364711861798,96.829208712453,
96.9219607176573,97.0148119165692,97.1077149347317,97.2007732759451,97.2715800787402,
97.389372261284),.UNSPECIFIED.);
#7750=B_SPLINE_CURVE_WITH_KNOTS('',3,(#67963,#67964,#67965,#67966,#67967,
#67968,#67969,#67970,#67971,#67972,#67973,#67974,#67975,#67976,#67977,#67978,
#67979,#67980,#67981,#67982,#67983,#67984,#67985,#67986,#67987,#67988,#67989,
#67990,#67991,#67992,#67993,#67994,#67995,#67996,#67997,#67998,#67999,#68000,
#68001,#68002,#68003,#68004,#68005,#68006,#68007,#68008,#68009,#68010,#68011,
#68012,#68013,#68014,#68015,#68016,#68017,#68018,#68019,#68020,#68021,#68022,
#68023,#68024,#68025,#68026,#68027,#68028,#68029,#68030,#68031,#68032,#68033,
#68034,#68035,#68036,#68037,#68038,#68039,#68040,#68041,#68042,#68043,#68044,
#68045,#68046,#68047,#68048,#68049,#68050,#68051,#68052,#68053,#68054,#68055,
#68056,#68057,#68058,#68059,#68060,#68061,#68062,#68063,#68064,#68065,#68066,
#68067,#68068,#68069,#68070,#68071,#68072,#68073,#68074,#68075,#68076,#68077,
#68078,#68079,#68080,#68081,#68082,#68083,#68084,#68085,#68086,#68087,#68088,
#68089,#68090,#68091,#68092,#68093,#68094,#68095,#68096,#68097,#68098,#68099,
#68100,#68101,#68102,#68103,#68104,#68105,#68106,#68107,#68108,#68109,#68110,
#68111,#68112,#68113,#68114,#68115,#68116,#68117,#68118,#68119,#68120,#68121,
#68122,#68123,#68124,#68125,#68126,#68127,#68128,#68129,#68130,#68131,#68132,
#68133,#68134,#68135,#68136,#68137,#68138,#68139,#68140,#68141,#68142,#68143,
#68144,#68145,#68146,#68147,#68148,#68149,#68150,#68151,#68152,#68153,#68154,
#68155,#68156,#68157,#68158,#68159,#68160,#68161,#68162,#68163,#68164,#68165,
#68166,#68167,#68168,#68169,#68170,#68171,#68172,#68173,#68174,#68175,#68176,
#68177,#68178,#68179,#68180,#68181,#68182,#68183,#68184,#68185,#68186,#68187,
#68188,#68189,#68190,#68191,#68192,#68193,#68194,#68195,#68196,#68197,#68198),
 .UNSPECIFIED.,.F.,.F.,(4,2,2,2,2,2,2,2,2,2,2,2,2,2,2,2,2,2,2,2,2,2,2,2,
2,2,2,2,2,2,2,2,2,2,2,2,2,2,2,2,2,2,2,2,2,2,2,2,2,2,2,2,2,2,2,2,2,2,2,2,
2,2,2,2,2,2,2,2,2,2,2,2,2,2,2,2,2,2,2,2,2,2,2,2,2,2,2,2,2,2,2,2,2,2,2,2,
2,2,2,2,2,2,2,2,2,2,2,2,2,2,2,2,2,2,2,2,2,4),(-2.73686895463578,-2.73388730285763,
-2.66011865704339,-2.63988763936745,-2.6293958949297,-2.62696028404078,
-2.62556643453363,-2.62435276064524,-2.62281159969532,-2.61967941241045,
-2.59983448907064,-2.58191759228708,-2.53965441226648,-2.47516168097801,
-2.46814886853108,-2.46512174206217,-2.46290653940541,-2.46086833666914,
-2.4581112612923,-2.45273078577678,-2.39846961740717,-2.36789471114992,
-2.30864033319991,-2.30411095537683,-2.30232010844391,-2.30106744101009,
-2.29993312179565,-2.29839794978084,-2.29540098596644,-2.27026090131758,
-2.25842758730487,-2.21615921911973,-2.14971664683455,-2.14368826812459,
-2.14084178207042,-2.13865544145626,-2.13656674090385,-2.13301890294904,
-2.12340974795611,-2.03651462736593,-1.99755993244561,-1.98218304391205,
-1.97956310119471,-1.97798514365945,-1.97676418151719,-1.97540796471224,
-1.97314182278633,-1.96469028643018,-1.89264997288797,-1.82552428878395,
-1.82014081083182,-1.81738292016307,-1.81534447340827,-1.81312935298962,
-1.8101029698597,-1.80309471206197,-1.73997465401417,-1.69748958517456,
-1.67433022377027,-1.65820723893921,-1.65554908162721,-1.65395992169028,
-1.65273743118205,-1.65138723380575,-1.64914780072375,-1.6409780263386,
-1.62677989769963,-1.59201912493646,-1.50700320710355,-1.5040027496952,
-1.49645892661612,-1.49357055413664,-1.49149835632751,-1.48930476274978,
-1.48640779825481,-1.48011304796233,-1.42040269999896,-1.35099130777964,
-1.33420361338767,-1.33151255295096,-1.32991376317028,-1.32868986548002,
-1.32734455212532,-1.32512690971973,-1.31718074812204,-1.25420022609978,
-1.17713917059732,-1.17134014377745,-1.1685383275136,-1.16635798993175,
-1.16395425009545,-1.16003057412773,-1.14624918161625,-1.12332016493283,
-1.02892694259301,-1.01022124786251,-1.00717659223332,-1.00563227182597,
-1.00441819657332,-1.00302621045053,-1.00059944440604,-0.990228090045812,
-0.970336686344806,-0.894802018007452,-0.893861286757274,-0.892185982919815,
-0.878754979068072,-0.876472456611157,-0.851775628695121,-0.847261070117154,
-0.844452129634196,-0.842270673831992,-0.839870173828236,-0.835961861536232,
-0.822335439318625,-0.799757619653653,-0.707428796331635,-0.699700907542827),
 .UNSPECIFIED.);
#7751=B_SPLINE_CURVE_WITH_KNOTS('',3,(#68204,#68205,#68206,#68207,#68208,
#68209,#68210,#68211,#68212,#68213,#68214,#68215,#68216,#68217,#68218,#68219,
#68220,#68221,#68222,#68223,#68224,#68225,#68226,#68227,#68228,#68229,#68230,
#68231,#68232,#68233,#68234,#68235,#68236,#68237,#68238,#68239,#68240,#68241,
#68242,#68243,#68244,#68245,#68246,#68247,#68248,#68249,#68250,#68251,#68252,
#68253,#68254,#68255,#68256,#68257,#68258,#68259,#68260,#68261,#68262,#68263,
#68264,#68265,#68266,#68267,#68268,#68269,#68270,#68271,#68272,#68273,#68274,
#68275,#68276,#68277,#68278,#68279,#68280,#68281,#68282,#68283,#68284,#68285,
#68286,#68287,#68288,#68289,#68290,#68291,#68292,#68293,#68294,#68295,#68296,
#68297,#68298,#68299,#68300,#68301,#68302,#68303,#68304,#68305,#68306,#68307,
#68308,#68309,#68310,#68311,#68312,#68313,#68314,#68315,#68316,#68317,#68318,
#68319,#68320,#68321,#68322,#68323,#68324,#68325,#68326,#68327,#68328,#68329,
#68330,#68331,#68332,#68333,#68334,#68335,#68336,#68337,#68338,#68339,#68340,
#68341,#68342),.UNSPECIFIED.,.F.,.F.,(4,3,3,3,3,3,3,3,3,3,3,3,3,3,3,3,3,
3,3,3,3,3,3,3,3,3,3,3,3,3,3,3,3,3,3,3,3,3,3,3,3,3,3,3,3,3,4),(103.672557568464,
103.766647671507,103.860769614952,103.954945648423,104.049262783787,104.143661761202,
104.238228269711,104.268186048427,104.361261356896,104.454210607977,104.547061434307,
104.63984443975,104.732592294393,104.825329820666,104.91808182587,105.010933024782,
105.103836042945,105.196894384158,105.267701186954,105.360776495423,105.453725746505,
105.546576572834,105.639359578277,105.73210743292,105.824844959194,105.917596964398,
106.01044816331,106.103351181473,106.196409522686,106.267216325481,106.36029163395,
106.453240885032,106.546091711361,106.638874716804,106.731622571448,106.824360097721,
106.917112102925,107.009963301837,107.10286632,107.195924661213,107.266731464008,
107.359803164529,107.452753997043,107.545595921847,107.638373985326,107.731122073524,
107.796189056121),.UNSPECIFIED.);
#7752=B_SPLINE_CURVE_WITH_KNOTS('',3,(#68343,#68344,#68345,#68346,#68347,
#68348,#68349,#68350,#68351,#68352,#68353,#68354,#68355,#68356,#68357,#68358,
#68359,#68360,#68361,#68362,#68363,#68364,#68365,#68366,#68367,#68368,#68369,
#68370,#68371,#68372,#68373,#68374,#68375,#68376,#68377,#68378,#68379,#68380,
#68381,#68382,#68383,#68384,#68385,#68386,#68387,#68388,#68389,#68390,#68391,
#68392,#68393,#68394,#68395,#68396,#68397,#68398,#68399,#68400,#68401,#68402,
#68403,#68404,#68405,#68406,#68407,#68408,#68409,#68410,#68411,#68412),
 .UNSPECIFIED.,.F.,.F.,(4,3,3,3,3,3,3,3,3,3,3,3,3,3,3,3,3,3,3,3,3,3,3,4),
(101.513685257635,101.608119071853,101.700876645965,101.793615016353,101.886358993441,
101.982058187924,102.074941828636,102.172048800005,102.269155771374,102.362231079843,
102.455180330925,102.548031157254,102.640814162697,102.733562017341,102.826299543614,
102.919051548818,103.01190274773,103.104805765893,103.197864107106,103.268670909901,
103.371807499052,103.474650856928,103.576968184871,103.672557568288),
 .UNSPECIFIED.);
#7753=B_SPLINE_CURVE_WITH_KNOTS('',3,(#68414,#68415,#68416,#68417,#68418,
#68419,#68420,#68421,#68422,#68423,#68424,#68425,#68426,#68427,#68428,#68429,
#68430,#68431,#68432,#68433,#68434,#68435,#68436,#68437,#68438,#68439,#68440,
#68441,#68442,#68443,#68444,#68445,#68446,#68447,#68448,#68449,#68450,#68451,
#68452,#68453,#68454,#68455,#68456,#68457,#68458,#68459,#68460,#68461,#68462,
#68463,#68464,#68465,#68466,#68467,#68468,#68469,#68470,#68471,#68472,#68473,
#68474,#68475,#68476,#68477,#68478,#68479,#68480,#68481,#68482,#68483,#68484,
#68485,#68486,#68487,#68488,#68489,#68490,#68491,#68492,#68493,#68494,#68495,
#68496,#68497,#68498,#68499,#68500,#68501,#68502,#68503,#68504,#68505,#68506,
#68507,#68508,#68509,#68510,#68511,#68512,#68513,#68514,#68515,#68516,#68517,
#68518,#68519,#68520,#68521,#68522,#68523,#68524,#68525,#68526,#68527,#68528,
#68529,#68530,#68531,#68532,#68533,#68534,#68535,#68536,#68537,#68538,#68539,
#68540,#68541,#68542,#68543,#68544,#68545,#68546,#68547,#68548,#68549,#68550,
#68551,#68552,#68553,#68554,#68555,#68556,#68557,#68558,#68559,#68560,#68561,
#68562,#68563,#68564,#68565,#68566,#68567,#68568,#68569,#68570,#68571,#68572,
#68573),.UNSPECIFIED.,.F.,.F.,(4,2,2,2,2,2,2,2,2,2,2,2,2,2,2,2,2,2,2,2,
2,2,2,2,2,2,2,2,2,2,2,2,2,2,2,2,2,2,2,2,2,2,2,2,2,2,2,2,2,2,2,2,2,2,2,2,
2,2,2,2,2,2,2,2,2,2,2,2,2,2,2,2,2,2,2,2,2,2,2,4),(-0.699700907542827,-0.686276977291691,
-0.683090925269945,-0.681538817046756,-0.680323886225827,-0.67896463697359,
-0.676645519823317,-0.673816968646951,-0.668059250540234,-0.587081823132608,
-0.529188097564907,-0.52377856154388,-0.521013837396152,-0.518973503301894,
-0.51675938760021,-0.51373985575832,-0.506771888317632,-0.433021140757069,
-0.396756974035746,-0.362681609868573,-0.359151545261417,-0.357550439722318,
-0.356326037876926,-0.356323848908466,-0.356321668848628,-0.35631949503184,
-0.356317327499221,-0.356315166128531,-0.35631301087063,-0.356310861764773,
-0.356308718876209,-0.356306582117758,-0.356304451406605,-0.356302326795541,
-0.356300208305847,-0.356298095798876,-0.356295989256645,-0.356293888744311,
-0.356291794264536,-0.356289705718492,-0.356287623082072,-0.356285546382978,
-0.356283475636906,-0.356281410790512,-0.356279351818326,-0.356277298610011,
-0.356275251223554,-0.356273209631598,-0.356271173873063,-0.356269143935612,
-0.356267119756429,-0.356265101212907,-0.356263088398756,-0.356261081377777,
-0.354927488733254,-0.352714821937657,-0.350038332508006,-0.344697150099441,
-0.330767951082596,-0.295818739667679,-0.211059178126563,-0.207945712296062,
-0.200515320845831,-0.19765094718273,-0.195589496447442,-0.193401317782504,
-0.190501403999757,-0.184159968387535,-0.121984694899469,-0.0691891517033401,
-0.0603199487069786,-0.0391893757664143,-0.0360126303896894,-0.0344656778862046,
-0.0332550758510056,-0.0321181940600108,-0.0307556468514484,-0.0287583570317623,
-0.021127039844488,-0.000959563674068928),.UNSPECIFIED.);
#7754=B_SPLINE_CURVE_WITH_KNOTS('',3,(#68574,#68575,#68576,#68577,#68578,
#68579,#68580,#68581,#68582,#68583,#68584,#68585,#68586,#68587,#68588,#68589,
#68590,#68591,#68592,#68593,#68594,#68595,#68596,#68597,#68598,#68599,#68600,
#68601,#68602,#68603,#68604,#68605,#68606,#68607,#68608,#68609,#68610,#68611,
#68612,#68613,#68614,#68615,#68616,#68617,#68618,#68619,#68620,#68621,#68622,
#68623,#68624,#68625,#68626,#68627,#68628,#68629,#68630,#68631,#68632,#68633,
#68634,#68635,#68636,#68637,#68638,#68639,#68640,#68641,#68642,#68643,#68644,
#68645,#68646,#68647,#68648,#68649,#68650,#68651,#68652,#68653,#68654,#68655,
#68656,#68657,#68658,#68659,#68660,#68661,#68662,#68663,#68664,#68665,#68666,
#68667,#68668,#68669,#68670,#68671,#68672,#68673,#68674,#68675,#68676,#68677,
#68678,#68679,#68680,#68681,#68682,#68683,#68684,#68685,#68686,#68687,#68688,
#68689,#68690,#68691,#68692,#68693,#68694,#68695,#68696,#68697,#68698,#68699,
#68700,#68701,#68702,#68703,#68704,#68705,#68706,#68707,#68708,#68709,#68710,
#68711,#68712,#68713,#68714,#68715,#68716,#68717,#68718,#68719,#68720,#68721,
#68722,#68723,#68724,#68725,#68726,#68727,#68728,#68729,#68730,#68731,#68732,
#68733,#68734,#68735,#68736,#68737),.UNSPECIFIED.,.F.,.F.,(4,2,2,2,2,2,
2,2,2,2,2,2,2,2,2,2,2,2,2,2,2,2,2,2,2,2,2,2,2,2,2,2,2,2,2,2,2,2,2,2,2,2,
2,2,2,2,2,2,2,2,2,2,2,2,2,2,2,2,2,2,2,2,2,2,2,2,2,2,2,2,2,2,2,2,2,2,2,2,
2,2,2,4),(-4.06129944956447,-3.97151586264303,-3.95158912669357,-3.93917790955167,
-3.93540729509048,-3.93304290918269,-3.93086148363844,-3.92805330769949,
-3.92342290913847,-3.89628110083149,-3.88370298359696,-3.82449984179205,
-3.79387526844183,-3.78197789163054,-3.77720478610657,-3.77368640709198,
-3.7720720349562,-3.77091915711506,-3.76976961872058,-3.76816585116467,
-3.76399544257687,-3.75809392296904,-3.68917863719632,-3.62163510889708,
-3.61463414732928,-3.6116154975118,-3.6094077678175,-3.60737732831911,-3.60463210061525,
-3.59927873050048,-3.53116209791604,-3.47478810332283,-3.46036544553658,
-3.4548915060975,-3.45216734064375,-3.44993412374128,-3.44859050843053,
-3.44737828965449,-3.44581465811106,-3.44255273325622,-3.41908873370272,
-3.32918274164586,-3.30702628181322,-3.29816119141286,-3.29153503242736,
-3.28858317450383,-3.2863870081591,-3.28434055739519,-3.2809854956126,-3.27254604705071,
-3.27023564293484,-3.19767550216652,-3.16159285770879,-3.14041018890563,
-3.12959450428564,-3.12714121018804,-3.12574651895218,-3.12453791794615,
-3.1230107162738,-3.12003053070776,-3.10254433619555,-3.00756772688076,
-2.98455719726473,-2.97075187851068,-2.96683505873477,-2.96443841173925,
-2.96226639903812,-2.95947792022273,-2.95501294001386,-2.93090117019321,
-2.9122987851847,-2.91164859934651,-2.83687096950397,-2.81698081522216,
-2.80662296006521,-2.80420334496349,-2.80281613370736,-2.8016066461644,
-2.80006872129379,-2.79693615006555,-2.77688322487906,-2.72883210508927),
 .UNSPECIFIED.);
#7755=B_SPLINE_CURVE_WITH_KNOTS('',3,(#68743,#68744,#68745,#68746,#68747,
#68748,#68749,#68750,#68751,#68752,#68753,#68754,#68755,#68756,#68757,#68758,
#68759,#68760,#68761,#68762,#68763,#68764,#68765,#68766,#68767,#68768,#68769,
#68770,#68771,#68772,#68773,#68774,#68775,#68776,#68777,#68778,#68779,#68780,
#68781,#68782,#68783,#68784,#68785,#68786,#68787,#68788,#68789,#68790,#68791,
#68792,#68793,#68794,#68795,#68796,#68797,#68798,#68799,#68800,#68801,#68802,
#68803,#68804,#68805,#68806,#68807,#68808,#68809,#68810,#68811,#68812,#68813,
#68814,#68815,#68816,#68817,#68818,#68819,#68820,#68821,#68822,#68823,#68824,
#68825,#68826,#68827,#68828,#68829,#68830,#68831,#68832,#68833,#68834,#68835,
#68836,#68837,#68838,#68839,#68840,#68841,#68842,#68843,#68844,#68845,#68846,
#68847,#68848,#68849,#68850,#68851,#68852,#68853,#68854,#68855,#68856,#68857,
#68858,#68859,#68860,#68861,#68862,#68863,#68864,#68865,#68866,#68867,#68868,
#68869,#68870,#68871,#68872,#68873,#68874,#68875,#68876,#68877,#68878),
 .UNSPECIFIED.,.F.,.F.,(4,3,3,3,3,3,3,3,3,3,3,3,3,3,3,3,3,3,3,3,3,3,3,3,
3,3,3,3,3,3,3,3,3,3,3,3,3,3,3,3,3,3,3,3,3,4),(109.955742875803,110.066352379532,
110.178347846238,110.265276879588,110.358352188057,110.451301439139,110.544152265468,
110.636935270911,110.729683125555,110.822420651828,110.915172657032,111.008023855944,
111.100926874107,111.19398521532,111.264792018115,111.357867326584,111.450816577665,
111.543667403995,111.636450409438,111.729198264081,111.821935790354,111.914687795559,
112.007538994471,112.100442012633,112.193500353846,112.264307156642,112.357382465111,
112.450331716192,112.543182542522,112.635965547965,112.728713402608,112.821450928881,
112.914202934085,113.007054132997,113.09995715116,113.193015492373,113.263822295168,
113.356909923667,113.449841610519,113.542684098276,113.635462310275,113.728201109468,
113.820956427048,113.913717308636,114.00656069971,114.078874363373),
 .UNSPECIFIED.);
#7756=B_SPLINE_CURVE_WITH_KNOTS('',3,(#68879,#68880,#68881,#68882,#68883,
#68884,#68885,#68886,#68887,#68888,#68889,#68890,#68891,#68892,#68893,#68894,
#68895,#68896,#68897,#68898,#68899,#68900,#68901,#68902,#68903,#68904,#68905,
#68906,#68907,#68908,#68909,#68910,#68911,#68912,#68913,#68914,#68915,#68916,
#68917,#68918,#68919,#68920,#68921,#68922,#68923,#68924,#68925,#68926,#68927,
#68928,#68929,#68930,#68931,#68932,#68933,#68934,#68935,#68936,#68937,#68938,
#68939,#68940,#68941,#68942,#68943,#68944,#68945,#68946,#68947,#68948,#68949,
#68950,#68951),.UNSPECIFIED.,.F.,.F.,(4,3,3,3,3,3,3,3,3,3,3,3,3,3,3,3,3,
3,3,3,3,3,3,3,4),(107.796189056121,107.888934141404,107.983262256686,108.076148385988,
108.171197494262,108.266246602535,108.359321911004,108.452271162085,108.545121988415,
108.637904993858,108.730652848501,108.823390374774,108.916142379978,109.00899357889,
109.101896597053,109.194954938266,109.265761741061,109.358401812315,109.450922236623,
109.543348474802,109.635705896307,109.728032055204,109.820339659303,109.912680590917,
109.955742875643),.UNSPECIFIED.);
#7757=B_SPLINE_CURVE_WITH_KNOTS('',3,(#68952,#68953,#68954,#68955,#68956,
#68957,#68958,#68959,#68960,#68961,#68962,#68963,#68964,#68965,#68966,#68967,
#68968,#68969,#68970,#68971,#68972,#68973,#68974,#68975,#68976,#68977,#68978,
#68979,#68980,#68981,#68982,#68983,#68984,#68985,#68986,#68987,#68988,#68989,
#68990,#68991,#68992,#68993,#68994,#68995,#68996,#68997,#68998,#68999,#69000,
#69001,#69002,#69003,#69004,#69005,#69006,#69007,#69008,#69009,#69010,#69011,
#69012,#69013,#69014,#69015,#69016,#69017,#69018,#69019,#69020,#69021,#69022,
#69023,#69024,#69025,#69026,#69027,#69028,#69029,#69030,#69031,#69032,#69033,
#69034,#69035,#69036,#69037,#69038,#69039,#69040,#69041,#69042,#69043,#69044,
#69045,#69046,#69047,#69048,#69049,#69050,#69051,#69052,#69053,#69054,#69055,
#69056,#69057,#69058,#69059,#69060,#69061,#69062,#69063,#69064,#69065,#69066,
#69067,#69068,#69069,#69070,#69071,#69072,#69073,#69074,#69075,#69076,#69077,
#69078,#69079,#69080,#69081,#69082,#69083,#69084,#69085,#69086,#69087,#69088,
#69089,#69090,#69091,#69092,#69093,#69094,#69095,#69096,#69097,#69098,#69099,
#69100,#69101,#69102,#69103,#69104,#69105,#69106,#69107,#69108,#69109,#69110,
#69111,#69112,#69113,#69114,#69115,#69116,#69117,#69118,#69119,#69120,#69121,
#69122,#69123,#69124,#69125,#69126,#69127,#69128,#69129,#69130,#69131,#69132,
#69133,#69134,#69135,#69136,#69137,#69138,#69139,#69140,#69141,#69142,#69143,
#69144,#69145,#69146,#69147,#69148,#69149,#69150,#69151,#69152,#69153,#69154,
#69155,#69156,#69157,#69158,#69159,#69160,#69161,#69162,#69163,#69164,#69165,
#69166,#69167,#69168,#69169,#69170,#69171,#69172,#69173,#69174,#69175,#69176,
#69177,#69178,#69179,#69180,#69181,#69182,#69183,#69184,#69185,#69186,#69187,
#69188,#69189,#69190,#69191,#69192,#69193,#69194,#69195,#69196,#69197,#69198,
#69199),.UNSPECIFIED.,.F.,.F.,(4,2,2,2,2,2,2,2,2,2,2,2,2,2,2,2,2,2,2,2,
2,2,2,2,2,2,2,2,2,2,2,2,2,2,2,2,2,2,2,2,2,2,2,2,2,2,2,2,2,2,2,2,2,2,2,2,
2,2,2,2,2,2,2,2,2,2,2,2,2,2,2,2,2,2,2,2,2,2,2,2,2,2,2,2,2,2,2,2,2,2,2,2,
2,2,2,2,2,2,2,2,2,2,2,2,2,2,2,2,2,2,2,2,2,2,2,2,2,2,2,2,2,2,2,4),(-2.72883210508927,
-2.6841013492052,-2.66146619148852,-2.64782669258225,-2.64392664933061,
-2.64153379778537,-2.6393609802297,-2.63656552850915,-2.63076777465074,
-2.55473613567879,-2.50993870810493,-2.49287229865924,-2.48356477933245,
-2.48122871033572,-2.47986009745189,-2.47864764736345,-2.4770804028602,
-2.47379919688275,-2.44976056957312,-2.44050155878647,-2.39639801574435,
-2.32997950921624,-2.32304639898441,-2.32003989149577,-2.31783453259101,
-2.31580170768498,-2.31304630455377,-2.30765243667475,-2.24501528304617,
-2.19337101920306,-2.1719123281163,-2.16100097949913,-2.15854102102134,
-2.15714494235822,-2.15593663334916,-2.15441172994718,-2.15144180856355,
-2.13414924667854,-2.09658843617803,-2.03156058092475,-2.03115640637577,
-2.02774431840743,-2.00409062487207,-1.99965389048755,-1.9968739845647,
-1.99470301124488,-1.99230176301732,-1.98836434117902,-1.97435177457992,
-1.95086494018577,-1.85290350080089,-1.8387391983045,-1.83619038522102,
-1.83463637041616,-1.83342220206355,-1.83206060483199,-1.82975673906367,
-1.82082769340627,-1.80473550240286,-1.79142580027802,-1.69024688906587,
-1.68833882962245,-1.67850324606158,-1.67492935530327,-1.67284063072717,
-1.67066521932038,-1.66785080218272,-1.66195654730544,-1.61618253528898,
-1.52504637561318,-1.51514132746889,-1.51266220554993,-1.51124681249597,
-1.51004002260378,-1.50854012896904,-1.5055953042289,-1.48431844973386,
-1.44908562752498,-1.36528407491663,-1.36323806846359,-1.35498641881049,
-1.35166285507353,-1.34962226533088,-1.34742202800553,-1.34444649872162,
-1.33768940068295,-1.32860323088797,-1.30566737323272,-1.21109256500193,
-1.19305057683538,-1.19004395938819,-1.18851090748547,-1.18730160743296,
-1.18591051780852,-1.18347427146321,-1.17289763340506,-1.15239965219208,
-1.08045093077643,-1.03648697106238,-1.03069121398188,-1.0278956565347,
-1.02572227912818,-1.02332832774368,-1.01942540299238,-1.00576496657007,
-0.983081827162041,-0.889992956048792,-0.870192546954515,-0.867069731336651,
-0.865533440972608,-0.864323729552294,-0.862934566324437,-0.860507480771691,
-0.850057292791093,-0.829915631721224,-0.756292265417527,-0.737894637092599,
-0.732583435711295,-0.711756182889704,-0.707496295141879,-0.704770004335944,
-0.702604276151083,-0.700219330519851,-0.698829799056907),.UNSPECIFIED.);
#7758=B_SPLINE_CURVE_WITH_KNOTS('',3,(#69205,#69206,#69207,#69208,#69209,
#69210,#69211,#69212,#69213,#69214,#69215,#69216,#69217,#69218,#69219,#69220,
#69221,#69222,#69223,#69224,#69225,#69226,#69227,#69228,#69229,#69230,#69231,
#69232,#69233,#69234,#69235,#69236,#69237,#69238,#69239,#69240,#69241,#69242,
#69243,#69244,#69245,#69246,#69247,#69248,#69249,#69250,#69251,#69252,#69253,
#69254,#69255,#69256,#69257,#69258,#69259,#69260,#69261,#69262,#69263,#69264,
#69265,#69266,#69267,#69268,#69269,#69270,#69271,#69272,#69273,#69274,#69275,
#69276,#69277,#69278,#69279,#69280,#69281,#69282,#69283,#69284,#69285,#69286,
#69287,#69288,#69289,#69290,#69291,#69292,#69293,#69294,#69295,#69296,#69297,
#69298,#69299,#69300,#69301,#69302,#69303,#69304,#69305,#69306,#69307,#69308,
#69309,#69310,#69311,#69312,#69313,#69314,#69315,#69316,#69317,#69318,#69319,
#69320,#69321,#69322,#69323,#69324,#69325,#69326,#69327,#69328,#69329,#69330,
#69331,#69332,#69333,#69334,#69335,#69336,#69337,#69338,#69339,#69340,#69341,
#69342,#69343,#69344,#69345,#69346),.UNSPECIFIED.,.F.,.F.,(4,3,3,3,3,3,
3,3,3,3,3,3,3,3,3,3,3,3,3,3,3,3,3,3,3,3,3,3,3,3,3,3,3,3,3,3,3,3,3,3,3,3,
3,3,3,3,3,4),(116.238928182823,116.262367710749,116.355443019218,116.448392270299,
116.541243096629,116.634026102072,116.726773956715,116.819511482989,116.912263488193,
117.005114687105,117.098017705267,117.191076046481,117.261882849275,117.354958157744,
117.447907408825,117.540758235155,117.633541240597,117.726289095241,117.819026621514,
117.911778626718,118.00462982563,118.097532843793,118.190591185006,118.261397987802,
118.354473296271,118.447422547353,118.540273373682,118.633056379125,118.725804233769,
118.818541760042,118.911293765246,119.004144964158,119.097047982321,119.190106323534,
119.260913126329,119.353988434798,119.446937685879,119.539788512209,119.632571517652,
119.725319372295,119.818056898568,119.910808903772,120.003660102684,120.096563120847,
120.18962146206,120.260428264856,120.353515438102,120.36310897423),
 .UNSPECIFIED.);
#7759=B_SPLINE_CURVE_WITH_KNOTS('',3,(#69347,#69348,#69349,#69350,#69351,
#69352,#69353,#69354,#69355,#69356,#69357,#69358,#69359,#69360,#69361,#69362,
#69363,#69364,#69365,#69366,#69367,#69368,#69369,#69370,#69371,#69372,#69373,
#69374,#69375,#69376,#69377,#69378,#69379,#69380,#69381,#69382,#69383,#69384,
#69385,#69386,#69387,#69388,#69389,#69390,#69391,#69392,#69393,#69394,#69395,
#69396,#69397,#69398,#69399,#69400,#69401,#69402,#69403,#69404,#69405,#69406,
#69407,#69408,#69409,#69410,#69411,#69412,#69413,#69414,#69415,#69416,#69417,
#69418,#69419),.UNSPECIFIED.,.F.,.F.,(4,3,3,3,3,3,3,3,3,3,3,3,3,3,3,3,3,
3,3,3,3,3,3,3,4),(114.078874363373,114.171925674316,114.263337433695,114.356412742164,
114.449361993246,114.542212819575,114.634995825018,114.727743679662,114.820481205935,
114.913233211139,115.006084410051,115.098987428214,115.192045769427,115.262852572222,
115.355560923056,115.44814349422,115.540628385212,115.633046882578,115.725431735228,
115.817808179262,115.910201437255,116.002693497524,116.095240289185,116.187934829135,
116.238928182608),.UNSPECIFIED.);
#7760=B_SPLINE_CURVE_WITH_KNOTS('',3,(#69421,#69422,#69423,#69424,#69425,
#69426,#69427,#69428,#69429,#69430,#69431,#69432,#69433,#69434,#69435,#69436,
#69437,#69438,#69439,#69440,#69441,#69442,#69443,#69444,#69445,#69446,#69447,
#69448,#69449,#69450,#69451,#69452,#69453,#69454,#69455,#69456,#69457,#69458,
#69459,#69460,#69461,#69462,#69463,#69464,#69465,#69466,#69467,#69468,#69469,
#69470,#69471,#69472,#69473,#69474,#69475,#69476,#69477,#69478,#69479,#69480,
#69481,#69482,#69483,#69484,#69485,#69486,#69487,#69488,#69489,#69490,#69491,
#69492,#69493,#69494,#69495,#69496,#69497,#69498,#69499,#69500,#69501,#69502,
#69503,#69504,#69505,#69506,#69507,#69508,#69509,#69510,#69511,#69512,#69513,
#69514,#69515,#69516,#69517,#69518),.UNSPECIFIED.,.F.,.F.,(4,2,2,2,2,2,
2,2,2,2,2,2,2,2,2,2,2,2,2,2,2,2,2,2,2,2,2,2,2,2,2,2,2,2,2,2,2,2,2,2,2,2,
2,2,2,2,2,2,4),(-0.698829799056907,-0.696283571084546,-0.691577884397476,
-0.682320401807412,-0.658777460441537,-0.594435323804517,-0.548031763846652,
-0.544415798399543,-0.54280221646017,-0.541579234139466,-0.540247882620269,
-0.538080176332597,-0.53058121904335,-0.474473115536343,-0.407688301766228,
-0.403537468993245,-0.395057480192895,-0.386288396708483,-0.382878033263585,
-0.380820634461199,-0.378629963688585,-0.375773329976131,-0.36961868589772,
-0.361453985045792,-0.341698772604676,-0.301511021545795,-0.256424265931702,
-0.250739562221718,-0.246149332569339,-0.242452966807125,-0.224275436340046,
-0.221262349514428,-0.219727851903959,-0.218518354530284,-0.217128095134346,
-0.21469585739779,-0.204175085882081,-0.183835028169646,-0.117555057193131,
-0.104050809409281,-0.0673725117839966,-0.0618635266257452,-0.0590867455823338,
-0.0569155169559284,-0.0548907916827107,-0.0525321504819316,-0.0491630845345916,
-0.0363424731010816,-0.000959780702671639),.UNSPECIFIED.);
#7761=B_SPLINE_CURVE_WITH_KNOTS('',3,(#69519,#69520,#69521,#69522,#69523,
#69524,#69525,#69526,#69527,#69528,#69529,#69530,#69531,#69532,#69533,#69534,
#69535,#69536,#69537,#69538,#69539,#69540,#69541,#69542,#69543,#69544,#69545,
#69546,#69547,#69548,#69549,#69550,#69551,#69552,#69553,#69554,#69555,#69556,
#69557,#69558,#69559,#69560,#69561,#69562,#69563,#69564,#69565,#69566,#69567,
#69568,#69569,#69570,#69571,#69572,#69573,#69574,#69575,#69576,#69577,#69578,
#69579,#69580,#69581,#69582,#69583,#69584,#69585,#69586,#69587,#69588,#69589,
#69590,#69591,#69592,#69593,#69594,#69595,#69596,#69597,#69598,#69599,#69600,
#69601,#69602,#69603,#69604,#69605,#69606,#69607,#69608,#69609,#69610,#69611,
#69612,#69613,#69614,#69615,#69616,#69617,#69618,#69619,#69620,#69621,#69622,
#69623,#69624,#69625,#69626,#69627,#69628,#69629,#69630,#69631,#69632,#69633,
#69634,#69635,#69636,#69637,#69638,#69639,#69640,#69641,#69642,#69643,#69644,
#69645,#69646,#69647,#69648,#69649,#69650,#69651,#69652,#69653,#69654,#69655,
#69656,#69657,#69658,#69659,#69660,#69661,#69662,#69663,#69664,#69665,#69666,
#69667,#69668,#69669,#69670,#69671,#69672,#69673,#69674,#69675,#69676,#69677,
#69678,#69679,#69680,#69681,#69682,#69683,#69684,#69685,#69686,#69687,#69688,
#69689,#69690,#69691,#69692,#69693,#69694,#69695,#69696,#69697,#69698,#69699,
#69700,#69701,#69702,#69703,#69704,#69705,#69706,#69707,#69708,#69709,#69710),
 .UNSPECIFIED.,.F.,.F.,(4,2,2,2,2,2,2,2,2,2,2,2,2,2,2,2,2,2,2,2,2,2,2,2,
2,2,2,2,2,2,2,2,2,2,2,2,2,2,2,2,2,2,2,2,2,2,2,2,2,2,2,2,2,2,2,2,2,2,2,2,
2,2,2,2,2,2,2,2,2,2,2,2,2,2,2,2,2,2,2,2,2,2,2,2,2,2,2,2,2,2,2,2,2,2,2,4),
(-4.05953948686282,-4.02804717577849,-3.96639928240388,-3.95854999347298,
-3.95634738771327,-3.9550086713052,-3.9537889795346,-3.95219327647582,-3.94950221092906,
-3.93256736994538,-3.9111114248824,-3.8606273404071,-3.82470830543548,-3.80955149306956,
-3.79952132351166,-3.79607170407889,-3.79404796095421,-3.79187750704361,
-3.78910054767651,-3.7846730447942,-3.76116755294912,-3.75483229669635,
-3.69956780167767,-3.63946713098213,-3.6349485083312,-3.63316339283032,
-3.63191523201871,-3.63078535967416,-3.62925670285534,-3.62627392473511,
-3.60133038383909,-3.59959761812075,-3.56742826705854,-3.51147451009267,
-3.49038028512578,-3.48182197790361,-3.47737701085475,-3.47363453691837,
-3.47128784834473,-3.47128420386158,-3.47128054925519,-3.4712768844594,
-3.47127320949574,-3.47126952428425,-3.47126582877831,-3.47126212291703,
-3.47125840666092,-3.47125467999486,-3.47125094285677,-3.47124719524596,
-3.471243437102,-3.47123966835957,-3.47123588900434,-3.46905960782723,-3.46628384948736,
-3.46043259606198,-3.38656982718402,-3.3402154807693,-3.32279031209362,
-3.31334540447379,-3.31099794060826,-3.30962682601396,-3.30841490733978,
-3.30685201653149,-3.30359288322983,-3.28019472580136,-3.19516950811749,
-3.16978371419665,-3.15495502179838,-3.15093967076339,-3.14852122248431,
-3.14635408162173,-3.14360559448257,-3.13927118409039,-3.11727380187453,
-3.1133801939102,-3.09496196018341,-3.02118365504073,-3.00109466504002,
-2.99066586918709,-2.98824112673003,-2.98685287582207,-2.98564368408787,
-2.98410770285012,-2.98098433340946,-2.96114515167558,-2.86819425500871,
-2.84553086029295,-2.83187926459257,-2.82797827943683,-2.82558538826315,
-2.82341288808368,-2.82061833962584,-2.81482424680385,-2.7708603527225,
-2.72806160371598),.UNSPECIFIED.);
#7762=B_SPLINE_CURVE_WITH_KNOTS('',3,(#69716,#69717,#69718,#69719,#69720,
#69721,#69722,#69723,#69724,#69725,#69726,#69727,#69728,#69729,#69730,#69731,
#69732,#69733,#69734,#69735,#69736,#69737,#69738,#69739,#69740,#69741,#69742,
#69743,#69744,#69745,#69746,#69747,#69748,#69749,#69750,#69751,#69752,#69753,
#69754,#69755,#69756,#69757,#69758,#69759,#69760,#69761,#69762,#69763,#69764,
#69765,#69766,#69767,#69768,#69769,#69770,#69771,#69772,#69773,#69774,#69775,
#69776,#69777,#69778,#69779,#69780,#69781,#69782,#69783,#69784,#69785,#69786,
#69787,#69788,#69789,#69790,#69791,#69792,#69793,#69794,#69795,#69796,#69797,
#69798,#69799,#69800,#69801,#69802,#69803,#69804,#69805,#69806,#69807,#69808,
#69809,#69810,#69811,#69812,#69813,#69814,#69815,#69816,#69817,#69818,#69819,
#69820,#69821,#69822,#69823,#69824,#69825,#69826,#69827,#69828,#69829,#69830,
#69831,#69832,#69833,#69834,#69835,#69836,#69837,#69838,#69839,#69840,#69841,
#69842,#69843,#69844,#69845,#69846,#69847,#69848,#69849,#69850,#69851,#69852,
#69853,#69854),.UNSPECIFIED.,.F.,.F.,(4,3,3,3,3,3,3,3,3,3,3,3,3,3,3,3,3,
3,3,3,3,3,3,3,3,3,3,3,3,3,3,3,3,3,3,3,3,3,3,3,3,3,3,3,3,3,4),(122.522113490002,
122.614221013806,122.706029130239,122.797814360325,122.889602493242,122.98194529004,
123.073867389215,123.166420534826,123.258973680436,123.352048988905,123.444998239987,
123.537849066316,123.630632071759,123.723379926402,123.816117452676,123.90886945788,
124.001720656792,124.094623674954,124.187682016168,124.258488818963,124.351564127432,
124.444513378513,124.537364204843,124.630147210286,124.722895064929,124.815632591202,
124.908384596407,125.001235795318,125.094138813481,125.187197154694,125.25800395749,
125.351079265959,125.44402851704,125.53687934337,125.629662348812,125.722410203456,
125.815147729729,125.907899734933,126.000750933845,126.093653952008,126.186712293221,
126.257519096016,126.354681067361,126.447615201551,126.540462792668,126.633238985787,
126.646166981397),.UNSPECIFIED.);
#7763=B_SPLINE_CURVE_WITH_KNOTS('',3,(#69855,#69856,#69857,#69858,#69859,
#69860,#69861,#69862,#69863,#69864,#69865,#69866,#69867,#69868,#69869,#69870,
#69871,#69872,#69873,#69874,#69875,#69876,#69877,#69878,#69879,#69880,#69881,
#69882,#69883,#69884,#69885,#69886,#69887,#69888,#69889,#69890,#69891,#69892,
#69893,#69894,#69895,#69896,#69897,#69898,#69899,#69900,#69901,#69902,#69903,
#69904,#69905,#69906,#69907,#69908,#69909,#69910,#69911,#69912,#69913,#69914,
#69915,#69916,#69917,#69918,#69919,#69920,#69921,#69922,#69923,#69924,#69925,
#69926,#69927),.UNSPECIFIED.,.F.,.F.,(4,3,3,3,3,3,3,3,3,3,3,3,3,3,3,3,3,
3,3,3,3,3,3,3,4),(120.36310897423,120.456046782208,120.54888901282,120.641667237396,
120.734412876219,120.827150749232,120.91990566331,121.012761178263,121.105670815306,
121.198732890817,121.259943403382,121.353018711851,121.445967962932,121.538818789262,
121.631601794705,121.724349649348,121.817087175621,121.909839180825,122.002690379737,
122.095593397899,122.188651739113,122.259458541909,122.378943455942,122.496088061442,
122.522113489712),.UNSPECIFIED.);
#7764=B_SPLINE_CURVE_WITH_KNOTS('',3,(#69928,#69929,#69930,#69931,#69932,
#69933,#69934,#69935,#69936,#69937,#69938,#69939,#69940,#69941,#69942,#69943,
#69944,#69945,#69946,#69947,#69948,#69949,#69950,#69951,#69952,#69953,#69954,
#69955,#69956,#69957,#69958,#69959,#69960,#69961,#69962,#69963,#69964,#69965,
#69966,#69967,#69968,#69969,#69970,#69971,#69972,#69973,#69974,#69975,#69976,
#69977,#69978,#69979,#69980,#69981,#69982,#69983,#69984,#69985,#69986,#69987,
#69988,#69989,#69990,#69991,#69992,#69993,#69994,#69995,#69996,#69997,#69998,
#69999,#70000,#70001,#70002,#70003,#70004,#70005,#70006,#70007,#70008,#70009,
#70010,#70011,#70012,#70013,#70014,#70015,#70016,#70017,#70018,#70019,#70020,
#70021,#70022,#70023,#70024,#70025,#70026,#70027,#70028,#70029,#70030,#70031,
#70032,#70033,#70034,#70035,#70036,#70037,#70038,#70039,#70040,#70041,#70042,
#70043,#70044,#70045,#70046,#70047,#70048,#70049,#70050,#70051,#70052,#70053,
#70054,#70055,#70056,#70057,#70058,#70059,#70060,#70061,#70062,#70063,#70064,
#70065,#70066,#70067,#70068,#70069,#70070,#70071,#70072,#70073,#70074,#70075,
#70076,#70077,#70078,#70079,#70080,#70081,#70082,#70083,#70084,#70085,#70086,
#70087,#70088,#70089,#70090,#70091,#70092,#70093,#70094,#70095,#70096,#70097,
#70098,#70099,#70100,#70101,#70102,#70103,#70104,#70105,#70106,#70107,#70108,
#70109,#70110,#70111,#70112,#70113,#70114,#70115,#70116,#70117,#70118,#70119,
#70120,#70121,#70122,#70123,#70124,#70125,#70126,#70127,#70128,#70129,#70130,
#70131,#70132,#70133,#70134,#70135,#70136,#70137,#70138,#70139,#70140,#70141,
#70142,#70143,#70144,#70145,#70146,#70147,#70148,#70149,#70150,#70151,#70152,
#70153,#70154,#70155,#70156,#70157,#70158,#70159,#70160,#70161,#70162,#70163,
#70164,#70165,#70166,#70167,#70168,#70169,#70170,#70171,#70172,#70173,#70174,
#70175,#70176,#70177,#70178,#70179,#70180,#70181,#70182,#70183,#70184,#70185,
#70186,#70187,#70188,#70189,#70190,#70191,#70192,#70193),.UNSPECIFIED.,
 .F.,.F.,(4,2,2,2,2,2,2,2,2,2,2,2,2,2,2,2,2,2,2,2,2,2,2,2,2,2,2,2,2,2,2,
2,2,2,2,2,2,2,2,2,2,2,2,2,2,2,2,2,2,2,2,2,2,2,2,2,2,2,2,2,2,2,2,2,2,2,2,
2,2,2,2,2,2,2,2,2,2,2,2,2,2,2,2,2,2,2,2,2,2,2,2,2,2,2,2,2,2,2,2,2,2,2,2,
2,2,2,2,2,2,2,2,2,2,2,2,2,2,2,2,2,2,2,2,2,2,2,2,2,2,2,2,2,4),(-2.72806160371598,
-2.69888338142189,-2.67839882741157,-2.66782932224088,-2.66539423811918,
-2.66400374012005,-2.66279490550071,-2.66126238715696,-2.65825664047353,
-2.64026252180287,-2.63538895716395,-2.6270834926754,-2.54340626855923,
-2.52203106568523,-2.508956214092,-2.50511476799622,-2.50273514854462,-2.5005592320277,
-2.49778502694809,-2.49194113288248,-2.41780109569306,-2.37163929988056,
-2.35427337529901,-2.34485131700401,-2.34250587520145,-2.34113528022046,
-2.33992338574495,-2.33835994563103,-2.33509761985756,-2.31160129531681,
-2.30823998944257,-2.26456356245751,-2.19125805651105,-2.18431857555433,
-2.18131119871924,-2.17910592268382,-2.17707367981462,-2.1743198360413,
-2.16893131379304,-2.11123761132658,-2.0305335632662,-2.02205832394373,
-2.01969181789282,-2.01831646417313,-2.01722657586411,-2.01573275322975,
-2.01281629785216,-1.99242185431692,-1.95952371040605,-1.87212020111034,
-1.86792491119328,-1.86137627378458,-1.85868818720353,-1.85667220563599,
-1.85445271214574,-1.85136742998131,-1.84397572512746,-1.81167326964969,
-1.71214799531086,-1.69970928484751,-1.69726635150294,-1.69572776854459,
-1.6945181913891,-1.69313134864069,-1.69071351622612,-1.68037985450563,
-1.66056012468515,-1.58531909736759,-1.58436809280869,-1.58271914516889,
-1.56929482908524,-1.56722009427172,-1.54245182500913,-1.53794814689526,
-1.53514783971042,-1.53297423732035,-1.53058353811107,-1.52669378654129,
-1.51315796654392,-1.49075411318256,-1.39930497583082,-1.39597207984956,
-1.37739183906319,-1.37436075142821,-1.37282255047578,-1.3716129005424,
-1.37022555762943,-1.36780585411014,-1.35744952599924,-1.33756770196131,
-1.26270629800734,-1.26188754619618,-1.2614466864697,-1.2598540866088,-1.24630564923713,
-1.24467196781882,-1.2435717746257,-1.21946138662273,-1.21499601683425,
-1.2122071870316,-1.21003484446982,-1.20763777607806,-1.2037201382674,-1.18991068920238,
-1.16688886543605,-1.07180623019604,-1.05435244406824,-1.05137349378257,
-1.04984637142369,-1.04863754927178,-1.04724227673317,-1.04478717249939,
-1.03395102234872,-1.01271493268722,-0.971951618413559,-0.89790973947994,
-0.892058985882461,-0.88928272211937,-0.887105716227925,-0.884725442045078,
-0.880884125927783,-0.867821042142076,-0.846472329926201,-0.763267470149372,
-0.755653994097213,-0.731814253632982,-0.728538875876849,-0.726972421183132,
-0.725759674828243,-0.724389729536665,-0.722049112380113,-0.712877250629526,
-0.698254248219955),.UNSPECIFIED.);
#7765=B_SPLINE_CURVE_WITH_KNOTS('',3,(#70199,#70200,#70201,#70202,#70203,
#70204,#70205,#70206,#70207,#70208,#70209,#70210,#70211,#70212,#70213,#70214,
#70215,#70216,#70217,#70218,#70219,#70220,#70221,#70222,#70223,#70224,#70225,
#70226,#70227,#70228,#70229,#70230,#70231,#70232,#70233,#70234,#70235,#70236,
#70237,#70238,#70239,#70240,#70241,#70242,#70243,#70244,#70245,#70246,#70247,
#70248,#70249,#70250,#70251,#70252,#70253,#70254,#70255,#70256,#70257,#70258,
#70259,#70260,#70261,#70262,#70263,#70264,#70265,#70266,#70267,#70268,#70269,
#70270,#70271,#70272,#70273,#70274,#70275,#70276,#70277,#70278,#70279,#70280,
#70281,#70282,#70283,#70284,#70285,#70286,#70287,#70288,#70289,#70290,#70291,
#70292,#70293,#70294,#70295,#70296,#70297,#70298,#70299,#70300,#70301,#70302,
#70303,#70304,#70305,#70306,#70307,#70308,#70309,#70310,#70311,#70312,#70313,
#70314,#70315,#70316,#70317,#70318,#70319,#70320,#70321,#70322,#70323,#70324,
#70325,#70326,#70327,#70328,#70329,#70330,#70331,#70332,#70333,#70334,#70335,
#70336,#70337),.UNSPECIFIED.,.F.,.F.,(4,3,3,3,3,3,3,3,3,3,3,3,3,3,3,3,3,
3,3,3,3,3,3,3,3,3,3,3,3,3,3,3,3,3,3,3,3,3,3,3,3,3,3,3,3,3,4),(128.805298797385,
128.904677691686,129.004435593514,129.104391172187,129.204654417159,129.256064511597,
129.349139820066,129.442089071147,129.534939897477,129.62772290292,129.720470757563,
129.813208283837,129.905960289041,129.998811487953,130.091714506115,130.184772847329,
130.255579650123,130.348654958592,130.441604209673,130.534455036003,130.627238041446,
130.719985896089,130.812723422362,130.905475427566,130.998326626478,131.091229644641,
131.184287985854,131.25509478865,131.348170097119,131.441119348201,131.53397017453,
131.626753179973,131.719501034617,131.81223856089,131.904990566094,131.997841765006,
132.090744783169,132.183803124382,132.254609927177,132.347666574696,132.440605721842,
132.533452388277,132.626231507612,132.718977855737,132.811706217422,132.904461102758,
132.928545070227),.UNSPECIFIED.);
#7766=B_SPLINE_CURVE_WITH_KNOTS('',3,(#70338,#70339,#70340,#70341,#70342,
#70343,#70344,#70345,#70346,#70347,#70348,#70349,#70350,#70351,#70352,#70353,
#70354,#70355,#70356,#70357,#70358,#70359,#70360,#70361,#70362,#70363,#70364,
#70365,#70366,#70367,#70368,#70369,#70370,#70371,#70372,#70373,#70374,#70375,
#70376,#70377,#70378,#70379,#70380,#70381,#70382,#70383,#70384,#70385,#70386,
#70387,#70388,#70389,#70390,#70391,#70392,#70393,#70394,#70395,#70396,#70397,
#70398,#70399,#70400,#70401,#70402,#70403,#70404,#70405,#70406,#70407,#70408,
#70409,#70410),.UNSPECIFIED.,.F.,.F.,(4,3,3,3,3,3,3,3,3,3,3,3,3,3,3,3,3,
3,3,3,3,3,3,3,4),(126.646166981397,126.738911088157,126.83164941077,126.924406755924,
127.017265771619,127.110180690541,127.203245854743,127.257034234543,127.350109543012,
127.443058794094,127.535909620423,127.628692625866,127.721440480509,127.814178006783,
127.906930011986,127.999781210898,128.092684229061,128.185742570274,128.25654937307,
128.352519890112,128.448333313375,128.543966784371,128.639494412394,128.734912471125,
128.805298797182),.UNSPECIFIED.);
#7767=B_SPLINE_CURVE_WITH_KNOTS('',3,(#70412,#70413,#70414,#70415,#70416,
#70417,#70418,#70419,#70420,#70421,#70422,#70423,#70424,#70425,#70426,#70427,
#70428,#70429,#70430,#70431,#70432,#70433,#70434,#70435,#70436,#70437,#70438,
#70439,#70440,#70441,#70442,#70443,#70444,#70445,#70446,#70447,#70448,#70449,
#70450,#70451,#70452,#70453,#70454,#70455,#70456,#70457,#70458,#70459,#70460,
#70461,#70462,#70463,#70464,#70465,#70466,#70467,#70468,#70469,#70470,#70471,
#70472,#70473,#70474,#70475,#70476,#70477,#70478,#70479,#70480,#70481,#70482,
#70483,#70484,#70485,#70486,#70487,#70488,#70489,#70490,#70491,#70492,#70493,
#70494,#70495,#70496,#70497),.UNSPECIFIED.,.F.,.F.,(4,2,2,2,2,2,2,2,2,2,
2,2,2,2,2,2,2,2,2,2,2,2,2,2,2,2,2,2,2,2,2,2,2,2,2,2,2,2,2,2,2,2,4),(-0.698254248219955,
-0.696102458516538,-0.635703733506079,-0.57518441543688,-0.569787984618583,
-0.567031427577486,-0.56499783329478,-0.56279171896029,-0.56061624404223,
-0.555477492209153,-0.522551661170759,-0.460002500985555,-0.435548709256675,
-0.409042994892415,-0.405726524438106,-0.404145618701489,-0.402927650588259,
-0.401580471982622,-0.399341792948716,-0.391326356640898,-0.37740592219274,
-0.343734221167373,-0.305915556585983,-0.252260526407009,-0.246902563946533,
-0.24415582419305,-0.242124683685358,-0.239916596334023,-0.237737657931382,
-0.234827254215558,-0.220808933442814,-0.183594512867419,-0.155274513005722,
-0.135713331536938,-0.0865880444975021,-0.082976479782648,-0.0813637553983931,
-0.0801409672278459,-0.0788093454703919,-0.0766402066409501,-0.0740683031706375,
-0.069014208624824,-0.000960727163108736),.UNSPECIFIED.);
#7768=B_SPLINE_CURVE_WITH_KNOTS('',3,(#70498,#70499,#70500,#70501,#70502,
#70503,#70504,#70505,#70506,#70507,#70508,#70509,#70510,#70511,#70512,#70513,
#70514,#70515,#70516,#70517,#70518,#70519,#70520,#70521,#70522,#70523,#70524,
#70525,#70526,#70527,#70528,#70529,#70530,#70531,#70532,#70533,#70534,#70535,
#70536,#70537,#70538,#70539,#70540,#70541,#70542,#70543,#70544,#70545,#70546,
#70547,#70548,#70549,#70550,#70551,#70552,#70553,#70554,#70555,#70556,#70557,
#70558,#70559,#70560,#70561,#70562,#70563,#70564,#70565,#70566,#70567,#70568,
#70569,#70570,#70571,#70572,#70573,#70574,#70575,#70576,#70577,#70578,#70579,
#70580,#70581,#70582,#70583,#70584,#70585,#70586,#70587,#70588,#70589,#70590,
#70591,#70592,#70593,#70594,#70595,#70596,#70597,#70598,#70599,#70600,#70601,
#70602,#70603,#70604,#70605,#70606,#70607,#70608,#70609,#70610,#70611,#70612,
#70613,#70614,#70615,#70616,#70617,#70618,#70619,#70620,#70621,#70622,#70623,
#70624,#70625,#70626,#70627,#70628,#70629,#70630,#70631,#70632,#70633,#70634,
#70635,#70636,#70637,#70638,#70639,#70640,#70641,#70642,#70643,#70644,#70645,
#70646,#70647,#70648,#70649,#70650,#70651,#70652,#70653,#70654,#70655,#70656,
#70657),.UNSPECIFIED.,.F.,.F.,(4,2,2,2,2,2,2,2,2,2,2,2,2,2,2,2,2,2,2,2,
2,2,2,2,2,2,2,2,2,2,2,2,2,2,2,2,2,2,2,2,2,2,2,2,2,2,2,2,2,2,2,2,2,2,2,2,
2,2,2,2,2,2,2,2,2,2,2,2,2,2,2,2,2,2,2,2,2,2,2,4),(-4.06075106093832,-3.99275036976407,
-3.9870394039298,-3.98370816777374,-3.98069268381622,-3.97848566267548,
-3.97645475111405,-3.97370717918828,-3.96834418522565,-3.90077993838917,
-3.86942222463597,-3.82865236952972,-3.82115784686525,-3.81895120518124,
-3.81761144710722,-3.81639180828979,-3.81479751869627,-3.81128481555614,
-3.75311507797128,-3.70942281512221,-3.67988888438663,-3.6690300230973,
-3.66130573155778,-3.65887183688258,-3.65649879022691,-3.65432033547206,
-3.65153113825552,-3.64696413637091,-3.62102581528763,-3.60265705529881,
-3.54800463754439,-3.50467275325379,-3.49836723347806,-3.49617304162426,
-3.49483604299982,-3.49361549207006,-3.49201540129283,-3.48847143678877,
-3.45269017344621,-3.37752958586565,-3.35410805051516,-3.34488481108031,
-3.33809530996548,-3.33508634047439,-3.33288044749564,-3.33084802253915,
-3.32809452057118,-3.32270841780889,-3.26569571332101,-3.22603231864836,
-3.20121539918965,-3.18483342318615,-3.17884583715928,-3.17459385746229,
-3.17285187725894,-3.17161196867734,-3.17047308885195,-3.16890941538682,
-3.16578898478335,-3.10338486944329,-3.02806989536521,-3.01671510848104,
-3.01306663349531,-3.01072957300689,-3.00853879031984,-3.00566914982275,
-3.00082878499004,-2.96898495607456,-2.87514949668317,-2.86088624025076,
-2.85269824021717,-2.85046225338921,-2.84911585911558,-2.84789801161689,
-2.84631649294655,-2.84367454400887,-2.82774200210274,-2.82025644963418,
-2.72989675923859,-2.72842990354347),.UNSPECIFIED.);
#7769=B_SPLINE_CURVE_WITH_KNOTS('',3,(#70663,#70664,#70665,#70666,#70667,
#70668,#70669,#70670,#70671,#70672,#70673,#70674,#70675,#70676,#70677,#70678,
#70679,#70680,#70681,#70682,#70683,#70684,#70685,#70686,#70687,#70688,#70689,
#70690,#70691,#70692,#70693,#70694,#70695,#70696,#70697,#70698,#70699,#70700,
#70701,#70702,#70703,#70704,#70705,#70706,#70707,#70708,#70709,#70710,#70711,
#70712,#70713,#70714,#70715,#70716,#70717,#70718,#70719,#70720,#70721,#70722,
#70723,#70724,#70725,#70726,#70727,#70728,#70729,#70730,#70731,#70732,#70733,
#70734,#70735,#70736,#70737,#70738,#70739,#70740,#70741,#70742,#70743,#70744,
#70745,#70746,#70747,#70748,#70749,#70750,#70751,#70752,#70753,#70754,#70755,
#70756,#70757,#70758,#70759,#70760,#70761,#70762,#70763,#70764,#70765,#70766,
#70767,#70768,#70769,#70770,#70771,#70772,#70773,#70774,#70775,#70776,#70777,
#70778,#70779,#70780,#70781,#70782,#70783,#70784,#70785,#70786,#70787,#70788,
#70789,#70790,#70791,#70792,#70793,#70794,#70795,#70796,#70797,#70798,#70799,
#70800,#70801),.UNSPECIFIED.,.F.,.F.,(4,3,3,3,3,3,3,3,3,3,3,3,3,3,3,3,3,
3,3,3,3,3,3,3,3,3,3,3,3,3,3,3,3,3,3,3,3,3,3,3,3,3,3,3,3,3,4),(135.088484104361,
135.237436223158,135.253155342757,135.346230651226,135.439179902308,135.532030728637,
135.62481373408,135.717561588724,135.810299114997,135.903051120201,135.995902319113,
136.088805337276,136.181863678489,136.252670481284,136.345745789753,136.438695040834,
136.531545867164,136.624328872607,136.71707672725,136.809814253523,136.902566258727,
136.995417457639,137.088320475802,137.181378817015,137.252185619811,137.34526092828,
137.438210179361,137.531061005691,137.623844011134,137.716591865777,137.80932939205,
137.902081397254,137.994932596166,138.087835614329,138.180893955542,138.251700758337,
138.344778545276,138.4377296359,138.534512329863,138.627291714081,138.720036095634,
138.81277029574,138.905519120361,138.998356489675,139.091246249693,139.184264767409,
139.211991187604),.UNSPECIFIED.);
#7770=B_SPLINE_CURVE_WITH_KNOTS('',3,(#70802,#70803,#70804,#70805,#70806,
#70807,#70808,#70809,#70810,#70811,#70812,#70813,#70814,#70815,#70816,#70817,
#70818,#70819,#70820,#70821,#70822,#70823,#70824,#70825,#70826,#70827,#70828,
#70829,#70830,#70831,#70832,#70833,#70834,#70835,#70836,#70837,#70838,#70839,
#70840,#70841,#70842,#70843,#70844,#70845,#70846,#70847,#70848,#70849,#70850,
#70851,#70852,#70853,#70854,#70855,#70856,#70857,#70858,#70859,#70860,#70861,
#70862,#70863,#70864,#70865,#70866,#70867,#70868,#70869,#70870,#70871,#70872,
#70873,#70874),.UNSPECIFIED.,.F.,.F.,(4,3,3,3,3,3,3,3,3,3,3,3,3,3,3,3,3,
3,3,3,3,3,3,3,4),(132.928545070227,133.021407547004,133.114327621085,133.207395885124,
133.254125065704,133.347200374173,133.440149625254,133.533000451584,133.625783457027,
133.71853131167,133.811268837943,133.904020843148,133.99687204206,134.089775060222,
134.182833401435,134.25364020423,134.345326368138,134.438221085142,134.529675013034,
134.621071924508,134.712437996792,134.806449523636,134.897871489002,134.993177796584,
135.088484104166),.UNSPECIFIED.);
#7771=B_SPLINE_CURVE_WITH_KNOTS('',3,(#70875,#70876,#70877,#70878,#70879,
#70880,#70881,#70882,#70883,#70884,#70885,#70886,#70887,#70888,#70889,#70890,
#70891,#70892,#70893,#70894,#70895,#70896,#70897,#70898,#70899,#70900,#70901,
#70902,#70903,#70904,#70905,#70906,#70907,#70908,#70909,#70910,#70911,#70912,
#70913,#70914,#70915,#70916,#70917,#70918,#70919,#70920,#70921,#70922,#70923,
#70924,#70925,#70926,#70927,#70928,#70929,#70930,#70931,#70932,#70933,#70934,
#70935,#70936,#70937,#70938,#70939,#70940,#70941,#70942,#70943,#70944,#70945,
#70946,#70947,#70948,#70949,#70950,#70951,#70952,#70953,#70954,#70955,#70956,
#70957,#70958,#70959,#70960,#70961,#70962,#70963,#70964,#70965,#70966,#70967,
#70968,#70969,#70970,#70971,#70972,#70973,#70974,#70975,#70976,#70977,#70978,
#70979,#70980,#70981,#70982,#70983,#70984,#70985,#70986,#70987,#70988,#70989,
#70990,#70991,#70992,#70993,#70994,#70995,#70996,#70997,#70998,#70999,#71000,
#71001,#71002,#71003,#71004,#71005,#71006,#71007,#71008,#71009,#71010,#71011,
#71012,#71013,#71014,#71015,#71016,#71017,#71018,#71019,#71020,#71021,#71022,
#71023,#71024,#71025,#71026,#71027,#71028,#71029,#71030,#71031,#71032,#71033,
#71034,#71035,#71036,#71037,#71038,#71039,#71040,#71041,#71042,#71043,#71044,
#71045,#71046,#71047,#71048,#71049,#71050,#71051,#71052,#71053,#71054,#71055,
#71056,#71057,#71058,#71059,#71060,#71061,#71062,#71063,#71064,#71065,#71066,
#71067,#71068,#71069,#71070,#71071,#71072,#71073,#71074,#71075,#71076,#71077,
#71078,#71079,#71080,#71081,#71082,#71083,#71084,#71085,#71086,#71087,#71088,
#71089,#71090,#71091,#71092,#71093,#71094,#71095,#71096,#71097,#71098,#71099,
#71100,#71101,#71102,#71103,#71104,#71105,#71106,#71107,#71108,#71109,#71110,
#71111,#71112,#71113,#71114,#71115,#71116,#71117,#71118,#71119,#71120,#71121,
#71122,#71123,#71124),.UNSPECIFIED.,.F.,.F.,(4,2,2,2,2,2,2,2,2,2,2,2,2,
2,2,2,2,2,2,2,2,2,2,2,2,2,2,2,2,2,2,2,2,2,2,2,2,2,2,2,2,2,2,2,2,2,2,2,2,
2,2,2,2,2,2,2,2,2,2,2,2,2,2,2,2,2,2,2,2,2,2,2,2,2,2,2,2,2,2,2,2,2,2,2,2,
2,2,2,2,2,2,2,2,2,2,2,2,2,2,2,2,2,2,2,2,2,2,2,2,2,2,2,2,2,2,2,2,2,2,2,2,
2,2,2,4),(-2.72842990354347,-2.70766769512995,-2.6942083450261,-2.69032641412718,
-2.68793745525578,-2.68576341178936,-2.68295968932953,-2.67712046877146,
-2.63063934267072,-2.5880968797651,-2.55250460569061,-2.53809976652567,
-2.52985337158713,-2.52761196869737,-2.52626444661439,-2.52504706458398,
-2.52346812029311,-2.52003765440959,-2.49066090251216,-2.44506140859784,
-2.37653288206304,-2.36952857624585,-2.36650951654422,-2.36430187674465,
-2.36227179210575,-2.35952745695151,-2.3541770481256,-2.28584341494831,
-2.23778788037546,-2.21777201815287,-2.20736906762255,-2.20494608305251,
-2.20355813185942,-2.20234875391929,-2.20081195290185,-2.1977868448031,
-2.17933208759673,-2.1753358924617,-2.08437847485296,-2.06205206729347,
-2.05313873604425,-2.04648403466199,-2.0435272227084,-2.04133043614501,
-2.0392856062088,-2.03648311220173,-2.030903432398,-1.97413015221405,-1.92470006520282,
-1.9015739586996,-1.88541533275022,-1.88276232408945,-1.88117770976386,
-1.87995959945233,-1.8786151925395,-1.87638740526087,-1.8682819902373,-1.85421801922655,
-1.81989185582541,-1.73472430248931,-1.7293547575476,-1.72342226494308,
-1.72058897177721,-1.71840420938142,-1.71605222655256,-1.71233554621172,
-1.70039715851024,-1.61408834712132,-1.59029772359292,-1.56321271142551,
-1.55983930037145,-1.55827120114759,-1.55705541744229,-1.55570227929214,
-1.55343542648626,-1.54491496137658,-1.47115370504828,-1.44011485971511,
-1.43564879486142,-1.42803458413242,-1.40474841923989,-1.4003341190964,
-1.39756113872085,-1.39539111341917,-1.39298634665299,-1.38903270132803,
-1.37485292224637,-1.35098092468692,-1.25034652258437,-1.23908396608546,
-1.23672112735015,-1.23520707213294,-1.23399943703651,-1.23259510849258,
-1.23009818647201,-1.21865563785451,-1.14229811453678,-1.08350902914624,
-1.07811614283608,-1.07536084387891,-1.07332790972965,-1.07112225295888,
-1.0681150247259,-1.06117886109398,-0.990354423422638,-0.952969625905835,
-0.940083104741701,-0.933118628276231,-0.916759211860557,-0.914095936035225,
-0.912508195943698,-0.911289487506822,-0.90994636280351,-0.907724848615461,
-0.899686326135728,-0.834882493174149,-0.760393619317092,-0.754552239014083,
-0.751748112899278,-0.749574036381803,-0.747185322837953,-0.743304422160899,
-0.72985492972577,-0.707644843877127,-0.69888673766205),.UNSPECIFIED.);
#7772=B_SPLINE_CURVE_WITH_KNOTS('',3,(#71130,#71131,#71132,#71133,#71134,
#71135,#71136,#71137,#71138,#71139,#71140,#71141,#71142,#71143,#71144,#71145,
#71146,#71147,#71148,#71149,#71150,#71151,#71152,#71153,#71154,#71155,#71156,
#71157,#71158,#71159,#71160,#71161,#71162,#71163,#71164,#71165,#71166,#71167,
#71168,#71169,#71170,#71171,#71172,#71173,#71174,#71175,#71176,#71177,#71178,
#71179,#71180,#71181,#71182,#71183,#71184,#71185,#71186,#71187,#71188,#71189,
#71190,#71191,#71192,#71193,#71194,#71195,#71196,#71197,#71198,#71199,#71200,
#71201,#71202,#71203,#71204,#71205,#71206,#71207,#71208,#71209,#71210,#71211,
#71212,#71213,#71214,#71215,#71216,#71217,#71218,#71219,#71220,#71221,#71222,
#71223,#71224,#71225,#71226,#71227,#71228,#71229,#71230,#71231,#71232,#71233,
#71234,#71235,#71236,#71237,#71238,#71239,#71240,#71241,#71242,#71243,#71244,
#71245,#71246,#71247,#71248,#71249,#71250,#71251,#71252,#71253,#71254,#71255,
#71256,#71257,#71258,#71259,#71260,#71261,#71262,#71263,#71264,#71265,#71266,
#71267,#71268),.UNSPECIFIED.,.F.,.F.,(4,3,3,3,3,3,3,3,3,3,3,3,3,3,3,3,3,
3,3,3,3,3,3,3,3,3,3,3,3,3,3,3,3,3,3,3,3,3,3,3,3,3,3,3,3,3,4),(141.371669411806,
141.463384214536,141.554991223589,141.646519531568,141.738006772963,141.829479020253,
141.920962326293,142.012539031028,142.104166831879,142.195941236867,142.249761312444,
142.342836620913,142.435785871994,142.528636698324,142.621419703766,142.71416755841,
142.806905084683,142.899657089887,142.992508288799,143.085411306962,143.178469648175,
143.249276450971,143.34235175944,143.435301010522,143.528151836851,143.620934842294,
143.713682696937,143.806420223211,143.899172228415,143.992023427327,144.084926445489,
144.177984786703,144.248791589498,144.341866897967,144.434816149048,144.527666975378,
144.620449980821,144.713197835464,144.805935361737,144.898687366942,144.991538565854,
145.084441584016,145.17749992523,145.248306728025,145.341382587312,145.434319351534,
145.495979852349),.UNSPECIFIED.);
#7773=B_SPLINE_CURVE_WITH_KNOTS('',3,(#71269,#71270,#71271,#71272,#71273,
#71274,#71275,#71276,#71277,#71278,#71279,#71280,#71281,#71282,#71283,#71284,
#71285,#71286,#71287,#71288,#71289,#71290,#71291,#71292,#71293,#71294,#71295,
#71296,#71297,#71298,#71299,#71300,#71301,#71302,#71303,#71304,#71305,#71306,
#71307,#71308,#71309,#71310,#71311,#71312,#71313,#71314,#71315,#71316,#71317,
#71318,#71319,#71320,#71321,#71322,#71323,#71324,#71325,#71326,#71327,#71328,
#71329,#71330,#71331,#71332,#71333,#71334,#71335,#71336,#71337,#71338,#71339,
#71340,#71341),.UNSPECIFIED.,.F.,.F.,(4,3,3,3,3,3,3,3,3,3,3,3,3,3,3,3,3,
3,3,3,3,3,3,3,4),(139.211991187604,139.251215896864,139.344291205333,139.437240456415,
139.530091282744,139.622874288187,139.715622142831,139.808359669104,139.901111674308,
139.99396287322,140.086865891383,140.179924232596,140.250731035391,140.34380634386,
140.436755594941,140.529606421271,140.622389426714,140.715137281357,140.807874807631,
140.900626812835,140.993478011747,141.086381029909,141.179439371123,141.250246173918,
141.371669411541),.UNSPECIFIED.);
#7774=B_SPLINE_CURVE_WITH_KNOTS('',3,(#71343,#71344,#71345,#71346,#71347,
#71348,#71349,#71350,#71351,#71352,#71353,#71354,#71355,#71356,#71357,#71358,
#71359,#71360,#71361,#71362,#71363,#71364,#71365,#71366,#71367,#71368,#71369,
#71370,#71371,#71372,#71373,#71374,#71375,#71376,#71377,#71378,#71379,#71380,
#71381,#71382,#71383,#71384,#71385,#71386,#71387,#71388,#71389,#71390,#71391,
#71392,#71393,#71394,#71395,#71396,#71397,#71398,#71399,#71400,#71401,#71402,
#71403,#71404,#71405,#71406,#71407,#71408,#71409,#71410,#71411,#71412,#71413,
#71414,#71415,#71416,#71417,#71418,#71419,#71420),.UNSPECIFIED.,.F.,.F.,
(4,2,2,2,2,2,2,2,2,2,2,2,2,2,2,2,2,2,2,2,2,2,2,2,2,2,2,2,2,2,2,2,2,2,2,
2,2,2,4),(-0.69888673766205,-0.61737787321185,-0.594275608976044,-0.591026220873479,
-0.589465041978538,-0.588253091333074,-0.587117868684638,-0.585062158207513,
-0.578589646343834,-0.535932535679405,-0.486495518521697,-0.437574746740716,
-0.431689648993861,-0.428906969588854,-0.426729261503032,-0.424352620734406,
-0.420526861896465,-0.407607888619948,-0.386575505212662,-0.314006926819699,
-0.271968688127983,-0.268365761394296,-0.266754730065773,-0.265532332063873,
-0.264200190209017,-0.262822357527625,-0.258425659352045,-0.225457271361734,
-0.198905423977322,-0.168653175776428,-0.114842416928233,-0.109483429210097,
-0.106736599750281,-0.104705605295463,-0.102497882458647,-0.0994803463246609,
-0.0924869291109943,-0.0829993670765108,-0.000961141795237354),
 .UNSPECIFIED.);
#7775=B_SPLINE_CURVE_WITH_KNOTS('',3,(#71421,#71422,#71423,#71424,#71425,
#71426,#71427,#71428,#71429,#71430,#71431,#71432,#71433,#71434,#71435,#71436,
#71437,#71438,#71439,#71440,#71441,#71442,#71443,#71444,#71445,#71446,#71447,
#71448,#71449,#71450,#71451,#71452,#71453,#71454,#71455,#71456,#71457,#71458,
#71459,#71460,#71461,#71462,#71463,#71464,#71465,#71466,#71467,#71468,#71469,
#71470,#71471,#71472,#71473,#71474,#71475,#71476,#71477,#71478,#71479,#71480,
#71481,#71482,#71483,#71484,#71485,#71486,#71487,#71488,#71489,#71490,#71491,
#71492,#71493,#71494,#71495,#71496,#71497,#71498,#71499,#71500,#71501,#71502,
#71503,#71504,#71505,#71506,#71507,#71508,#71509,#71510,#71511,#71512,#71513,
#71514,#71515,#71516,#71517,#71518,#71519,#71520,#71521,#71522,#71523,#71524,
#71525,#71526,#71527,#71528,#71529,#71530,#71531,#71532,#71533,#71534,#71535,
#71536,#71537,#71538,#71539,#71540,#71541,#71542,#71543,#71544,#71545,#71546,
#71547,#71548,#71549,#71550,#71551,#71552,#71553,#71554,#71555,#71556,#71557,
#71558,#71559,#71560,#71561,#71562,#71563,#71564,#71565,#71566,#71567,#71568,
#71569,#71570,#71571,#71572,#71573,#71574,#71575,#71576,#71577,#71578,#71579,
#71580,#71581,#71582,#71583,#71584,#71585,#71586,#71587,#71588),
 .UNSPECIFIED.,.F.,.F.,(4,2,2,2,2,2,2,2,2,2,2,2,2,2,2,2,2,2,2,2,2,2,2,2,
2,2,2,2,2,2,2,2,2,2,2,2,2,2,2,2,2,2,2,2,2,2,2,2,2,2,2,2,2,2,2,2,2,2,2,2,
2,2,2,2,2,2,2,2,2,2,2,2,2,2,2,2,2,2,2,2,2,2,2,4),(-4.06093435138946,-4.01153152329989,
-4.00789799007013,-4.00586629122596,-4.00448963764063,-4.0031583524371,
-4.00193575656261,-4.00032313025772,-3.99671113649732,-3.94836980179485,
-3.93081203940535,-3.91540010078564,-3.8783489475813,-3.85346745779512,
-3.84649300711091,-3.84347886169196,-3.841271802689,-3.83924014409437,-3.83649047935593,
-3.83112019156007,-3.77619062026438,-3.74501588752085,-3.70204042269368,
-3.69068050460192,-3.68378080101615,-3.68168021627958,-3.68054226929608,
-3.67933272562805,-3.67779581283627,-3.67477078687394,-3.65632486505783,
-3.65227377042139,-3.60355190709301,-3.53018787326717,-3.52350438671813,
-3.52054201660475,-3.51834394656903,-3.51629995882664,-3.51295859473903,
-3.50460146736822,-3.50270997680874,-3.41873810735623,-3.3835693899566,
-3.369279173774,-3.36110458940688,-3.35887608705832,-3.35752108400561,-3.35630532340663,
-3.35473949451488,-3.35215100395849,-3.3372448520238,-3.23999313708196,
-3.2166081869537,-3.20263822828317,-3.19870472567385,-3.19630417514178,
-3.19413273119173,-3.19135069325714,-3.18562245873916,-3.10696899088985,
-3.04581173522982,-3.03799123386341,-3.0357910532956,-3.03445261470516,
-3.03323232429893,-3.03163469322602,-3.02810467681065,-2.97096909782754,
-2.92135992783375,-2.8951429948549,-2.87996436177344,-2.87591591822703,
-2.87348960525738,-2.87132304597746,-2.86858561631221,-2.86428873470835,
-2.84289084550076,-2.83880702740414,-2.83710395355222,-2.82351885727087,
-2.82195046521615,-2.82092381306869,-2.74570799838588,-2.72901630049176),
 .UNSPECIFIED.);
#7776=B_SPLINE_CURVE_WITH_KNOTS('',3,(#71594,#71595,#71596,#71597,#71598,
#71599,#71600,#71601,#71602,#71603,#71604,#71605,#71606,#71607,#71608,#71609,
#71610,#71611,#71612,#71613,#71614,#71615,#71616,#71617,#71618,#71619,#71620,
#71621,#71622,#71623,#71624,#71625,#71626,#71627,#71628,#71629,#71630,#71631,
#71632,#71633,#71634,#71635,#71636,#71637,#71638,#71639,#71640,#71641,#71642,
#71643,#71644,#71645,#71646,#71647,#71648,#71649,#71650,#71651,#71652,#71653,
#71654,#71655,#71656,#71657,#71658,#71659,#71660,#71661,#71662,#71663,#71664,
#71665,#71666,#71667,#71668,#71669,#71670,#71671,#71672,#71673,#71674,#71675,
#71676,#71677,#71678,#71679,#71680,#71681,#71682,#71683,#71684,#71685,#71686,
#71687,#71688,#71689,#71690,#71691,#71692,#71693,#71694,#71695,#71696,#71697,
#71698,#71699,#71700,#71701,#71702,#71703,#71704,#71705,#71706,#71707,#71708,
#71709,#71710,#71711,#71712,#71713,#71714,#71715,#71716,#71717,#71718,#71719,
#71720,#71721,#71722,#71723,#71724,#71725,#71726,#71727,#71728,#71729,#71730,
#71731,#71732),.UNSPECIFIED.,.F.,.F.,(4,3,3,3,3,3,3,3,3,3,3,3,3,3,3,3,3,
3,3,3,3,3,3,3,3,3,3,3,3,3,3,3,3,3,3,3,3,3,3,3,3,3,3,3,3,3,4),(147.654854718721,
147.749034590717,147.843249280477,147.937520831394,148.031935902181,148.126434874257,
148.221101205661,148.246852143605,148.339927452074,148.432876703156,148.525727529485,
148.618510534928,148.711258389572,148.803995915845,148.896747921049,148.989599119961,
149.082502138124,149.175560479337,149.246367282132,149.339442590601,149.432391841682,
149.525242668012,149.618025673454,149.710773528098,149.803511054371,149.896263059575,
149.989114258487,150.08201727665,150.175075617863,150.245882420659,150.338957729128,
150.431906980209,150.524757806539,150.617540811982,150.710288666625,150.803026192899,
150.895778198103,150.988629397015,151.081532415177,151.174590756391,151.245397559185,
151.338468831933,151.431419321105,151.524261223258,151.617039297619,151.709788393534,
151.778475043453),.UNSPECIFIED.);
#7777=B_SPLINE_CURVE_WITH_KNOTS('',3,(#71733,#71734,#71735,#71736,#71737,
#71738,#71739,#71740,#71741,#71742,#71743,#71744,#71745,#71746,#71747,#71748,
#71749,#71750,#71751,#71752,#71753,#71754,#71755,#71756,#71757,#71758,#71759,
#71760,#71761,#71762,#71763,#71764,#71765,#71766,#71767,#71768,#71769,#71770,
#71771,#71772,#71773,#71774,#71775,#71776,#71777,#71778,#71779,#71780,#71781,
#71782,#71783,#71784,#71785,#71786,#71787,#71788,#71789,#71790,#71791,#71792,
#71793,#71794,#71795,#71796,#71797,#71798,#71799,#71800,#71801,#71802),
 .UNSPECIFIED.,.F.,.F.,(4,3,3,3,3,3,3,3,3,3,3,3,3,3,3,3,3,3,3,3,3,3,3,4),
(145.495979852349,145.589960104124,145.682716610858,145.775454763184,145.868199371119,
145.963104994977,146.055990070736,146.151905968644,146.247821866552,146.340897175021,
146.433846426103,146.526697252432,146.619480257875,146.712228112519,146.804965638792,
146.897717643997,146.990568842909,147.083471861071,147.176530202285,147.247337005078,
147.350216986418,147.452811717714,147.554895483707,147.654854718549),
 .UNSPECIFIED.);
#7778=B_SPLINE_CURVE_WITH_KNOTS('',3,(#71803,#71804,#71805,#71806,#71807,
#71808,#71809,#71810,#71811,#71812,#71813,#71814,#71815,#71816,#71817,#71818,
#71819,#71820,#71821,#71822,#71823,#71824,#71825,#71826,#71827,#71828,#71829,
#71830,#71831,#71832,#71833,#71834,#71835,#71836,#71837,#71838,#71839,#71840,
#71841,#71842,#71843,#71844,#71845,#71846,#71847,#71848,#71849,#71850,#71851,
#71852,#71853,#71854,#71855,#71856,#71857,#71858,#71859,#71860,#71861,#71862,
#71863,#71864,#71865,#71866,#71867,#71868,#71869,#71870,#71871,#71872,#71873,
#71874,#71875,#71876,#71877,#71878,#71879,#71880,#71881,#71882,#71883,#71884,
#71885,#71886,#71887,#71888,#71889,#71890,#71891,#71892,#71893,#71894,#71895,
#71896,#71897,#71898,#71899,#71900,#71901,#71902,#71903,#71904,#71905,#71906,
#71907,#71908,#71909,#71910,#71911,#71912,#71913,#71914,#71915,#71916,#71917,
#71918,#71919,#71920,#71921,#71922,#71923,#71924,#71925,#71926,#71927,#71928,
#71929,#71930,#71931,#71932,#71933,#71934,#71935,#71936,#71937,#71938,#71939,
#71940,#71941,#71942,#71943,#71944,#71945,#71946,#71947,#71948,#71949,#71950,
#71951,#71952,#71953,#71954,#71955,#71956,#71957,#71958,#71959,#71960,#71961,
#71962,#71963,#71964,#71965,#71966,#71967,#71968,#71969,#71970,#71971,#71972,
#71973,#71974,#71975,#71976,#71977,#71978,#71979,#71980,#71981,#71982,#71983,
#71984,#71985,#71986,#71987,#71988,#71989,#71990,#71991,#71992,#71993,#71994,
#71995,#71996,#71997,#71998,#71999,#72000,#72001,#72002,#72003,#72004,#72005,
#72006,#72007,#72008,#72009,#72010,#72011,#72012,#72013,#72014,#72015,#72016,
#72017,#72018,#72019,#72020,#72021,#72022,#72023,#72024,#72025,#72026,#72027,
#72028,#72029,#72030,#72031,#72032,#72033,#72034,#72035,#72036,#72037,#72038,
#72039,#72040),.UNSPECIFIED.,.F.,.F.,(4,2,2,2,2,2,2,2,2,2,2,2,2,2,2,2,2,
2,2,2,2,2,2,2,2,2,2,2,2,2,2,2,2,2,2,2,2,2,2,2,2,2,2,2,2,2,2,2,2,2,2,2,2,
2,2,2,2,2,2,2,2,2,2,2,2,2,2,2,2,2,2,2,2,2,2,2,2,2,2,2,2,2,2,2,2,2,2,2,2,
2,2,2,2,2,2,2,2,2,2,2,2,2,2,2,2,2,2,2,2,2,2,2,2,2,2,2,2,2,4),(-2.72901630049176,
-2.72588029484488,-2.71554420431033,-2.71312586823548,-2.71173875403762,
-2.71052894744365,-2.70899008968555,-2.70595629961924,-2.6873194778769,
-2.59330998046564,-2.57046281203296,-2.55672882229577,-2.55281870986864,
-2.55042328960037,-2.54825050475498,-2.54545840305993,-2.53967951871034,
-2.46283569056572,-2.4000599990981,-2.39214097159969,-2.38993093493505,
-2.38859024706071,-2.38737056367352,-2.38577729038927,-2.38309555495988,
-2.36636665265747,-2.36348263533094,-2.3080487493928,-2.23712415971649,
-2.23126258824115,-2.22845421704563,-2.22627925759363,-2.22418772303356,
-2.22060091265583,-2.21068025805306,-2.12938578572331,-2.09248124940335,
-2.07769558917056,-2.06929209686111,-2.0670355730592,-2.06568446694449,
-2.06446765524131,-2.06289447889109,-2.05949583878602,-2.03146916409239,
-1.98357305133032,-1.91431881122955,-1.9089700478127,-1.90622580222741,
-1.90419542231494,-1.9019871110333,-1.89896650844108,-1.89195582167329,
-1.82240058939648,-1.77796017705985,-1.74836136439719,-1.74492514771631,
-1.74334489704457,-1.74212709261085,-1.74077972603305,-1.73853993891986,
-1.73031419686828,-1.71596244845137,-1.680570361235,-1.59700231945177,-1.59465226744745,
-1.58660505333646,-1.58331582383525,-1.58128151727221,-1.57907643227049,
-1.57607366703063,-1.56916411469123,-1.55981954888957,-1.53596303824289,
-1.43546509614923,-1.42402577210174,-1.42164993718324,-1.42013165984848,
-1.41892341312118,-1.41752150841245,-1.41503670331932,-1.40377937417503,
-1.32822615235987,-1.2683871392199,-1.26299112223109,-1.26023463817137,
-1.25820103060483,-1.25599483710384,-1.25298722417104,-1.24605171485911,
-1.1821508514095,-1.13971819026412,-1.12039022732583,-1.1017834573835,-1.09875077771291,
-1.09721207318116,-1.0960021810802,-1.09461473225072,-1.0921952559819,-1.08184595260976,
-1.06198529371962,-0.98695710065982,-0.945058158606808,-0.939326159771434,
-0.936543030143212,-0.93437106551414,-0.931970277146261,-0.928037154741231,
-0.914076572114394,-0.890711584586582,-0.793545756854862,-0.77844788971629,
-0.775848604212841,-0.774279368708628,-0.773062877220329,-0.771709140413467,
-0.769441699493578,-0.760923745953994,-0.698659185575319),.UNSPECIFIED.);
#7779=B_SPLINE_CURVE_WITH_KNOTS('',3,(#72046,#72047,#72048,#72049,#72050,
#72051,#72052,#72053,#72054,#72055,#72056,#72057,#72058,#72059,#72060,#72061,
#72062,#72063,#72064,#72065,#72066,#72067,#72068,#72069,#72070,#72071,#72072,
#72073,#72074,#72075,#72076,#72077,#72078,#72079,#72080,#72081,#72082,#72083,
#72084,#72085,#72086,#72087,#72088,#72089,#72090,#72091,#72092,#72093,#72094,
#72095,#72096,#72097,#72098,#72099,#72100,#72101,#72102,#72103,#72104,#72105,
#72106,#72107,#72108,#72109,#72110,#72111,#72112,#72113,#72114,#72115,#72116,
#72117,#72118,#72119,#72120,#72121,#72122,#72123,#72124,#72125,#72126,#72127,
#72128,#72129,#72130,#72131,#72132,#72133,#72134,#72135,#72136,#72137,#72138,
#72139,#72140,#72141,#72142,#72143,#72144,#72145,#72146,#72147,#72148,#72149,
#72150,#72151,#72152,#72153,#72154,#72155,#72156,#72157,#72158,#72159,#72160,
#72161,#72162,#72163,#72164,#72165,#72166,#72167,#72168,#72169,#72170,#72171,
#72172,#72173,#72174,#72175,#72176,#72177,#72178,#72179,#72180,#72181),
 .UNSPECIFIED.,.F.,.F.,(4,3,3,3,3,3,3,3,3,3,3,3,3,3,3,3,3,3,3,3,3,3,3,3,
3,3,3,3,3,3,3,3,3,3,3,3,3,3,3,3,3,3,3,3,3,4),(153.938040026209,154.04907363987,
154.161545321533,154.243942974766,154.337018283235,154.429967534316,154.522818360646,
154.615601366089,154.708349220732,154.801086747005,154.893838752209,154.986689951121,
155.079592969284,155.172651310497,155.243458113292,155.336533421761,155.429482672842,
155.522333499172,155.615116504615,155.707864359258,155.800601885531,155.893353890736,
155.986205089648,156.07910810781,156.172166449023,156.242973251819,156.336048560288,
156.42899781137,156.521848637699,156.614631643142,156.707379497786,156.800117024059,
156.892869029263,156.985720228175,157.078623246338,157.171681587551,157.242488390346,
157.335575759881,157.428507308114,157.521349741414,157.614127982882,157.706866895333,
157.799623116126,157.892384934503,157.985231229661,158.0611738712),
 .UNSPECIFIED.);
#7780=B_SPLINE_CURVE_WITH_KNOTS('',3,(#72182,#72183,#72184,#72185,#72186,
#72187,#72188,#72189,#72190,#72191,#72192,#72193,#72194,#72195,#72196,#72197,
#72198,#72199,#72200,#72201,#72202,#72203,#72204,#72205,#72206,#72207,#72208,
#72209,#72210,#72211,#72212,#72213,#72214,#72215,#72216,#72217,#72218,#72219,
#72220,#72221,#72222,#72223,#72224,#72225,#72226,#72227,#72228,#72229,#72230,
#72231,#72232,#72233,#72234,#72235,#72236,#72237,#72238,#72239,#72240,#72241,
#72242,#72243,#72244,#72245,#72246,#72247,#72248,#72249,#72250,#72251,#72252,
#72253,#72254),.UNSPECIFIED.,.F.,.F.,(4,3,3,3,3,3,3,3,3,3,3,3,3,3,3,3,3,
3,3,3,3,3,3,3,4),(151.778475043453,151.871220907862,151.964643855325,152.057531651525,
152.151222174619,152.244912697712,152.337988006181,152.430937257262,152.523788083591,
152.616571089034,152.709318943678,152.802056469951,152.894808475155,152.987659674067,
153.08056269223,153.173621033443,153.244427836239,153.337016135053,153.429485246562,
153.521860686742,153.614167880084,153.706445323099,153.798704748058,153.890999970072,
153.9380400259),.UNSPECIFIED.);
#7781=B_SPLINE_CURVE_WITH_KNOTS('',3,(#72256,#72257,#72258,#72259,#72260,
#72261,#72262,#72263,#72264,#72265,#72266,#72267,#72268,#72269,#72270,#72271,
#72272,#72273,#72274,#72275,#72276,#72277,#72278,#72279,#72280,#72281,#72282,
#72283,#72284,#72285,#72286,#72287,#72288,#72289,#72290,#72291,#72292,#72293,
#72294,#72295,#72296,#72297,#72298,#72299,#72300,#72301,#72302,#72303,#72304,
#72305,#72306,#72307,#72308,#72309,#72310,#72311,#72312,#72313,#72314,#72315,
#72316,#72317,#72318,#72319,#72320,#72321,#72322,#72323,#72324,#72325,#72326,
#72327,#72328,#72329,#72330,#72331,#72332,#72333,#72334,#72335,#72336,#72337,
#72338,#72339,#72340,#72341,#72342,#72343,#72344,#72345,#72346,#72347,#72348,
#72349,#72350,#72351,#72352,#72353,#72354,#72355,#72356,#72357,#72358,#72359,
#72360,#72361,#72362,#72363,#72364,#72365,#72366,#72367,#72368,#72369,#72370,
#72371,#72372,#72373,#72374,#72375,#72376,#72377,#72378,#72379,#72380,#72381,
#72382,#72383,#72384,#72385,#72386,#72387),.UNSPECIFIED.,.F.,.F.,(4,2,2,
2,2,2,2,2,2,2,2,2,2,2,2,2,2,2,2,2,2,2,2,2,2,2,2,2,2,2,2,2,2,2,2,2,2,2,2,
2,2,2,2,2,2,2,2,2,2,2,2,2,2,2,2,2,2,2,2,2,2,2,2,2,2,4),(-0.698659185575319,
-0.687266515453911,-0.622356187764353,-0.616969918375531,-0.614215814685308,
-0.612182701337184,-0.610019936900468,-0.607121258634964,-0.603881266552389,
-0.598394520947855,-0.560376419496656,-0.490122354470279,-0.48025461911514,
-0.456084254210486,-0.452797334160289,-0.451245263777175,-0.450031031409607,
-0.448667611165948,-0.446356722551842,-0.437352533337298,-0.421071586591021,
-0.371014250546084,-0.299259701627354,-0.29336012398568,-0.290574201590711,
-0.288395530193951,-0.288370833317646,-0.288347238818523,-0.288324689518502,
-0.288303131734123,-0.288282515070775,-0.288262792170785,-0.288243918504708,
-0.288225852161942,-0.288208553689533,-0.288191985917783,-0.288176113790564,
-0.288160904224996,-0.288146325992296,-0.288132349575939,-0.288118947105193,
-0.288106092203015,-0.288093759882848,-0.288081926500809,-0.288068418482872,
-0.288055037864439,-0.288041781084367,-0.288028646155354,-0.288015631104619,
-0.288002734006105,-0.285546058246958,-0.281311570021109,-0.276154174713262,
-0.265653300801223,-0.237507845314393,-0.170139024840153,-0.157172011659093,
-0.13312383978533,-0.129841074410973,-0.128289806795767,-0.127075677672748,
-0.125711792394532,-0.12339880635479,-0.114370410182652,-0.0980277981269592,
-0.000961400426472246),.UNSPECIFIED.);
#7782=B_SPLINE_CURVE_WITH_KNOTS('',3,(#72388,#72389,#72390,#72391,#72392,
#72393,#72394,#72395,#72396,#72397,#72398,#72399,#72400,#72401,#72402,#72403,
#72404,#72405,#72406,#72407,#72408,#72409,#72410,#72411,#72412,#72413,#72414,
#72415,#72416,#72417,#72418,#72419,#72420,#72421,#72422,#72423,#72424,#72425,
#72426,#72427,#72428,#72429,#72430,#72431,#72432,#72433,#72434,#72435,#72436,
#72437,#72438,#72439,#72440,#72441,#72442,#72443,#72444,#72445,#72446,#72447,
#72448,#72449,#72450,#72451,#72452,#72453,#72454,#72455,#72456,#72457,#72458,
#72459,#72460,#72461,#72462,#72463,#72464,#72465,#72466,#72467,#72468,#72469,
#72470,#72471,#72472,#72473,#72474,#72475,#72476,#72477,#72478,#72479,#72480,
#72481,#72482,#72483,#72484,#72485,#72486,#72487,#72488,#72489,#72490,#72491,
#72492,#72493,#72494,#72495,#72496,#72497,#72498,#72499,#72500,#72501,#72502,
#72503,#72504,#72505,#72506,#72507,#72508,#72509,#72510,#72511,#72512,#72513,
#72514,#72515,#72516,#72517,#72518,#72519,#72520,#72521,#72522,#72523,#72524,
#72525,#72526),.UNSPECIFIED.,.F.,.F.,(4,3,3,3,3,3,3,3,3,3,3,3,3,3,3,3,3,
3,3,3,3,3,3,3,3,3,3,3,3,3,3,3,3,3,3,3,3,3,3,3,3,3,3,3,3,3,4),(153.9380400259,
154.031841518464,154.125665311938,154.219534280467,154.313536546128,154.407613950455,
154.50185962512,154.545879037082,154.638954345551,154.731903596633,154.824754422962,
154.917537428405,155.010285283049,155.103022809322,155.195774814526,155.288626013438,
155.381529031601,155.474587372814,155.545394175609,155.638469484078,155.731418735159,
155.824269561489,155.917052566932,156.009800421575,156.102537947848,156.195289953053,
156.288141151965,156.381044170127,156.47410251134,156.544909314136,156.637984622605,
156.730933873686,156.823784700016,156.916567705459,157.009315560102,157.102053086375,
157.194805091579,157.287656290491,157.380559308654,157.473617649867,157.544424452662,
157.637497610758,157.730449616904,157.823291694321,157.916069797578,158.008814802925,
158.061709245204),.UNSPECIFIED.);
#7783=B_SPLINE_CURVE_WITH_KNOTS('',3,(#72532,#72533,#72534,#72535,#72536,
#72537,#72538,#72539,#72540,#72541,#72542,#72543,#72544,#72545,#72546,#72547,
#72548,#72549,#72550,#72551,#72552,#72553,#72554,#72555,#72556,#72557,#72558,
#72559,#72560,#72561,#72562,#72563,#72564,#72565,#72566,#72567,#72568,#72569,
#72570,#72571,#72572,#72573,#72574,#72575,#72576,#72577,#72578,#72579,#72580,
#72581,#72582,#72583,#72584,#72585,#72586,#72587,#72588,#72589,#72590,#72591,
#72592,#72593,#72594,#72595,#72596,#72597,#72598,#72599,#72600,#72601,#72602,
#72603,#72604,#72605,#72606,#72607,#72608,#72609,#72610,#72611,#72612,#72613,
#72614,#72615,#72616,#72617,#72618,#72619,#72620,#72621,#72622,#72623,#72624,
#72625,#72626,#72627,#72628,#72629,#72630,#72631,#72632,#72633,#72634,#72635,
#72636,#72637,#72638,#72639,#72640,#72641,#72642,#72643,#72644,#72645,#72646,
#72647,#72648,#72649,#72650,#72651,#72652,#72653,#72654,#72655,#72656,#72657,
#72658,#72659,#72660,#72661,#72662,#72663,#72664,#72665,#72666,#72667,#72668,
#72669,#72670,#72671,#72672,#72673),.UNSPECIFIED.,.F.,.F.,(4,3,3,3,3,3,
3,3,3,3,3,3,3,3,3,3,3,3,3,3,3,3,3,3,3,3,3,3,3,3,3,3,3,3,3,3,3,3,3,3,3,3,
3,3,3,3,3,4),(160.22122533308,160.241033805926,160.334109114395,160.427058365477,
160.519909191806,160.612692197249,160.705440051892,160.798177578166,160.89092958337,
160.983780782282,161.076683800445,161.169742141658,161.240548944453,161.333624252922,
161.426573504003,161.519424330333,161.612207335776,161.704955190419,161.797692716692,
161.890444721897,161.983295920809,162.076198938971,162.169257280184,162.24006408298,
162.333139391449,162.42608864253,162.51893946886,162.611722474303,162.704470328946,
162.797207855219,162.889959860423,162.982811059335,163.075714077498,163.168772418711,
163.239579221506,163.332654529975,163.425603781056,163.518454607386,163.611237612829,
163.703985467472,163.796722993745,163.88947499895,163.982326197861,164.075229216024,
164.168287557237,164.239094360033,164.332179484883,164.345416085528),
 .UNSPECIFIED.);
#7784=B_SPLINE_CURVE_WITH_KNOTS('',3,(#72674,#72675,#72676,#72677,#72678,
#72679,#72680,#72681,#72682,#72683,#72684,#72685,#72686,#72687,#72688,#72689,
#72690,#72691,#72692,#72693,#72694,#72695,#72696,#72697,#72698,#72699,#72700,
#72701,#72702,#72703,#72704,#72705,#72706,#72707,#72708,#72709,#72710,#72711,
#72712,#72713,#72714,#72715,#72716,#72717,#72718,#72719,#72720,#72721,#72722,
#72723,#72724,#72725,#72726,#72727,#72728,#72729,#72730,#72731,#72732,#72733,
#72734,#72735,#72736,#72737,#72738,#72739,#72740,#72741,#72742,#72743,#72744,
#72745,#72746),.UNSPECIFIED.,.F.,.F.,(4,3,3,3,3,3,3,3,3,3,3,3,3,3,3,3,3,
3,3,3,3,3,3,3,4),(158.0611738712,158.154226324278,158.242003528873,158.335078837342,
158.428028088423,158.520878914753,158.613661920196,158.706409774839,158.799147301112,
158.891899306317,158.984750505229,159.077653523391,159.170711864604,159.241518667399,
159.334279950863,159.426915408281,159.519453075191,159.611924161267,159.704361393212,
159.796789950703,159.889234999661,159.98177900834,160.074377343998,160.167124708233,
160.221225332896),.UNSPECIFIED.);
#7785=B_SPLINE_CURVE_WITH_KNOTS('',3,(#72748,#72749,#72750,#72751,#72752,
#72753,#72754,#72755,#72756,#72757,#72758,#72759,#72760,#72761,#72762,#72763,
#72764,#72765,#72766,#72767,#72768,#72769,#72770,#72771,#72772,#72773,#72774,
#72775,#72776,#72777,#72778,#72779,#72780,#72781,#72782,#72783,#72784,#72785,
#72786,#72787,#72788,#72789,#72790,#72791,#72792,#72793,#72794,#72795,#72796,
#72797,#72798,#72799,#72800,#72801,#72802,#72803,#72804,#72805,#72806,#72807,
#72808,#72809,#72810,#72811,#72812,#72813,#72814,#72815,#72816,#72817,#72818,
#72819,#72820,#72821,#72822,#72823),.UNSPECIFIED.,.F.,.F.,(4,3,3,3,3,3,
3,3,3,3,3,3,3,3,3,3,3,3,3,3,3,3,3,3,3,4),(158.061709245204,158.154451987715,
158.251823888583,158.344704552456,158.43765085974,158.530736002963,158.543939591189,
158.637014899658,158.729964150739,158.822814977069,158.915597982512,159.008345837155,
159.101083363429,159.193835368633,159.286686567545,159.379589585707,159.472647926921,
159.543454729716,159.636279965892,159.72898388903,159.821591754,159.914128724522,
160.006629196486,160.099109132765,160.191614229513,160.22122533308),
 .UNSPECIFIED.);
#7786=B_SPLINE_CURVE_WITH_KNOTS('',3,(#72824,#72825,#72826,#72827,#72828,
#72829,#72830,#72831,#72832,#72833,#72834,#72835,#72836,#72837,#72838,#72839,
#72840,#72841,#72842,#72843,#72844,#72845,#72846,#72847,#72848,#72849,#72850,
#72851,#72852,#72853,#72854,#72855,#72856,#72857,#72858,#72859,#72860,#72861,
#72862,#72863,#72864,#72865,#72866,#72867,#72868,#72869,#72870,#72871,#72872,
#72873,#72874,#72875,#72876,#72877,#72878,#72879,#72880,#72881,#72882,#72883,
#72884,#72885,#72886,#72887,#72888,#72889,#72890,#72891,#72892,#72893,#72894,
#72895,#72896,#72897,#72898,#72899,#72900,#72901,#72902,#72903,#72904,#72905,
#72906,#72907,#72908,#72909,#72910,#72911,#72912,#72913,#72914,#72915,#72916,
#72917,#72918,#72919,#72920,#72921,#72922,#72923,#72924,#72925,#72926,#72927,
#72928,#72929,#72930,#72931,#72932,#72933,#72934,#72935,#72936,#72937,#72938,
#72939,#72940,#72941,#72942,#72943,#72944,#72945,#72946,#72947,#72948,#72949,
#72950,#72951,#72952,#72953,#72954,#72955,#72956,#72957,#72958,#72959,#72960,
#72961,#72962,#72963,#72964,#72965,#72966,#72967,#72968,#72969,#72970,#72971,
#72972,#72973,#72974,#72975,#72976,#72977,#72978,#72979),.UNSPECIFIED.,
 .F.,.F.,(4,2,2,2,2,2,2,2,2,2,2,2,2,2,2,2,2,2,2,2,2,2,2,2,2,2,2,2,2,2,2,
2,2,2,2,2,2,2,2,2,2,2,2,2,2,2,2,2,2,2,2,2,2,2,2,2,2,2,2,2,2,2,2,2,2,2,2,
2,2,2,2,2,2,2,2,2,2,4),(-4.05945128562048,-4.041155615787,-3.96822305735629,
-3.95974543906513,-3.95748283761133,-3.95613082929757,-3.95491508830725,
-3.95334577591954,-3.9499649216044,-3.9225742929906,-3.91027746944697,-3.86234400841248,
-3.82583015536063,-3.81066255166307,-3.80062850272235,-3.79718115304648,
-3.79515755425338,-3.79298773552869,-3.79021391736335,-3.78579606338421,
-3.76244312156547,-3.7563929350647,-3.70573924716846,-3.64476492051424,
-3.6369572793063,-3.63475894152135,-3.63342124781676,-3.63220136847798,
-3.63060391511297,-3.62707284668614,-3.56994341699948,-3.51539368170489,
-3.49248589976508,-3.48340788196599,-3.47670951636516,-3.47375105999008,
-3.47154383658876,-3.46951425843179,-3.46677079532305,-3.46142264065606,
-3.39273544649311,-3.34509188086973,-3.32505480631329,-3.31464494853154,
-3.31222180014704,-3.31083399522521,-3.30962489668847,-3.30808864885882,
-3.30496345058287,-3.28507478640793,-3.26523581763717,-3.22340431140956,
-3.16086200942504,-3.15398071286598,-3.15098361266331,-3.14878015255424,
-3.14674555589994,-3.14345187975107,-3.13537402198371,-3.13267340178628,
-3.05582409796174,-2.99894158311332,-2.99139393853123,-2.98922186692513,
-2.98788995657361,-2.98666799641334,-2.98505785126534,-2.98145816821869,
-2.93978845584888,-2.88546371535253,-2.83676602464008,-2.83075906639412,
-2.8279230611756,-2.82574492911033,-2.82366419049867,-2.82013017169038,
-2.8105608213515,-2.72811779794129),.UNSPECIFIED.);
#7787=B_SPLINE_CURVE_WITH_KNOTS('',3,(#72985,#72986,#72987,#72988,#72989,
#72990,#72991,#72992,#72993,#72994,#72995,#72996,#72997,#72998,#72999,#73000,
#73001,#73002,#73003,#73004,#73005,#73006,#73007,#73008,#73009,#73010,#73011,
#73012,#73013,#73014,#73015,#73016,#73017,#73018,#73019,#73020,#73021,#73022,
#73023,#73024,#73025,#73026,#73027,#73028,#73029,#73030,#73031,#73032,#73033,
#73034,#73035,#73036,#73037,#73038,#73039,#73040,#73041,#73042,#73043,#73044,
#73045,#73046,#73047,#73048,#73049,#73050,#73051,#73052,#73053,#73054,#73055,
#73056,#73057,#73058,#73059,#73060,#73061,#73062,#73063,#73064,#73065,#73066,
#73067,#73068,#73069,#73070,#73071,#73072,#73073,#73074,#73075,#73076,#73077,
#73078,#73079,#73080,#73081,#73082,#73083,#73084,#73085,#73086,#73087,#73088,
#73089,#73090,#73091,#73092,#73093,#73094,#73095,#73096,#73097,#73098,#73099,
#73100,#73101,#73102,#73103,#73104,#73105,#73106,#73107,#73108,#73109,#73110,
#73111,#73112,#73113,#73114,#73115,#73116,#73117,#73118,#73119,#73120,#73121,
#73122,#73123),.UNSPECIFIED.,.F.,.F.,(4,3,3,3,3,3,3,3,3,3,3,3,3,3,3,3,3,
3,3,3,3,3,3,3,3,3,3,3,3,3,3,3,3,3,3,3,3,3,3,3,3,3,3,3,3,3,4),(166.504410640259,
166.596297384287,166.688136850633,166.779954822237,166.871777056864,166.963690802419,
167.055648939086,167.147767225871,167.237639775614,167.330715084083,167.423664335165,
167.516515161494,167.609298166937,167.702046021581,167.794783547854,167.887535553058,
167.98038675197,168.073289770132,168.166348111346,168.23715491414,168.330230222609,
168.42317947369,168.51603030002,168.608813305462,168.701561160106,168.794298686379,
168.887050691583,168.979901890495,169.072804908657,169.165863249871,169.236670052667,
169.329745361136,169.422694612218,169.515545438547,169.60832844399,169.701076298634,
169.793813824907,169.886565830111,169.979417029023,170.072320047186,170.165378388399,
170.236185191194,170.329275020313,170.422212993343,170.515063477816,170.607841724268,
170.6284544512),.UNSPECIFIED.);
#7788=B_SPLINE_CURVE_WITH_KNOTS('',3,(#73124,#73125,#73126,#73127,#73128,
#73129,#73130,#73131,#73132,#73133,#73134,#73135,#73136,#73137,#73138,#73139,
#73140,#73141,#73142,#73143,#73144,#73145,#73146,#73147,#73148,#73149,#73150,
#73151,#73152,#73153,#73154,#73155,#73156,#73157,#73158,#73159,#73160,#73161,
#73162,#73163,#73164,#73165,#73166,#73167,#73168,#73169,#73170,#73171,#73172,
#73173,#73174,#73175,#73176,#73177,#73178,#73179,#73180,#73181,#73182,#73183,
#73184,#73185,#73186,#73187,#73188,#73189,#73190,#73191,#73192,#73193,#73194,
#73195,#73196),.UNSPECIFIED.,.F.,.F.,(4,3,3,3,3,3,3,3,3,3,3,3,3,3,3,3,3,
3,3,3,3,3,3,3,4),(164.345416085528,164.438349632499,164.531188681243,164.623965162733,
164.716710030763,164.809448104393,164.90220419039,164.995061403628,165.087973612034,
165.181037179722,165.23860949856,165.331684807029,165.42463405811,165.51748488444,
165.610267889883,165.703015744526,165.795753270799,165.888505276004,165.981356474916,
166.074259493078,166.167317834292,166.238124637087,166.356936113553,166.47352002816,
166.504410640098),.UNSPECIFIED.);
#7789=B_SPLINE_CURVE_WITH_KNOTS('',3,(#73197,#73198,#73199,#73200,#73201,
#73202,#73203,#73204,#73205,#73206,#73207,#73208,#73209,#73210,#73211,#73212,
#73213,#73214,#73215,#73216,#73217,#73218,#73219,#73220,#73221,#73222,#73223,
#73224,#73225,#73226,#73227,#73228,#73229,#73230,#73231,#73232,#73233,#73234,
#73235,#73236,#73237,#73238,#73239,#73240,#73241,#73242,#73243,#73244,#73245,
#73246,#73247,#73248,#73249,#73250,#73251,#73252,#73253,#73254,#73255,#73256,
#73257,#73258,#73259,#73260,#73261,#73262,#73263,#73264,#73265,#73266,#73267,
#73268,#73269,#73270,#73271,#73272,#73273,#73274,#73275,#73276,#73277,#73278,
#73279,#73280,#73281,#73282,#73283,#73284,#73285,#73286,#73287,#73288,#73289,
#73290,#73291,#73292,#73293,#73294,#73295,#73296,#73297,#73298,#73299,#73300,
#73301,#73302,#73303,#73304,#73305,#73306,#73307,#73308,#73309,#73310,#73311,
#73312,#73313,#73314,#73315,#73316,#73317,#73318,#73319,#73320,#73321,#73322,
#73323,#73324,#73325,#73326,#73327,#73328,#73329,#73330,#73331,#73332,#73333,
#73334,#73335,#73336,#73337,#73338,#73339,#73340,#73341,#73342,#73343,#73344,
#73345,#73346,#73347,#73348,#73349,#73350,#73351,#73352,#73353,#73354,#73355,
#73356,#73357,#73358,#73359,#73360,#73361,#73362,#73363,#73364,#73365,#73366,
#73367,#73368,#73369,#73370,#73371,#73372,#73373,#73374,#73375,#73376,#73377,
#73378,#73379,#73380,#73381,#73382,#73383,#73384,#73385,#73386,#73387,#73388,
#73389,#73390,#73391,#73392,#73393,#73394,#73395,#73396,#73397,#73398,#73399,
#73400,#73401,#73402,#73403,#73404,#73405,#73406,#73407,#73408,#73409,#73410,
#73411,#73412,#73413,#73414,#73415,#73416,#73417,#73418,#73419,#73420,#73421,
#73422,#73423,#73424,#73425,#73426,#73427,#73428,#73429,#73430,#73431,#73432,
#73433,#73434,#73435,#73436,#73437,#73438,#73439,#73440,#73441,#73442,#73443,
#73444,#73445,#73446,#73447,#73448,#73449,#73450,#73451,#73452),
 .UNSPECIFIED.,.F.,.F.,(4,2,2,2,2,2,2,2,2,2,2,2,2,2,2,2,2,2,2,2,2,2,2,2,
2,2,2,2,2,2,2,2,2,2,2,2,2,2,2,2,2,2,2,2,2,2,2,2,2,2,2,2,2,2,2,2,2,2,2,2,
2,2,2,2,2,2,2,2,2,2,2,2,2,2,2,2,2,2,2,2,2,2,2,2,2,2,2,2,2,2,2,2,2,2,2,2,
2,2,2,2,2,2,2,2,2,2,2,2,2,2,2,2,2,2,2,2,2,2,2,2,2,2,2,2,2,2,2,4),(-2.72811779794129,
-2.72395110668382,-2.67214372911574,-2.66770327696862,-2.66593056720559,
-2.66468478331899,-2.66355240133755,-2.66201398564284,-2.65899323474141,
-2.63265304698429,-2.62727950601053,-2.58612276171778,-2.54256551362552,
-2.522557501376,-2.51010895070006,-2.50633454472439,-2.50396952913755,-2.50178871273713,
-2.49898297806673,-2.49436014269696,-2.46735794526941,-2.45451366521268,
-2.45257996453047,-2.42732072097454,-2.35444894230556,-2.34597271640488,
-2.34370972377173,-2.34235733079876,-2.34114114016076,-2.3395711107769,
-2.33618819295914,-2.30875441231986,-2.22227930203469,-2.2006097493273,
-2.19188462749187,-2.18534205429394,-2.18240550078208,-2.18021194879892,
-2.17816159727414,-2.17478554877441,-2.16622125912555,-2.16412020904491,
-2.08915274747851,-2.03056794345043,-2.02305692286148,-2.02079664516133,
-2.01944485868361,-2.01835037092282,-2.0168193746106,-2.0137214999958,-1.9863704763543,
-1.98179260014154,-1.91866485598044,-1.86807240373345,-1.86216145073006,
-1.85937396663502,-1.85719573536469,-1.85482180445761,-1.85100760403844,
-1.8381945786011,-1.8173935604341,-1.74966121054221,-1.70246644744588,-1.69885221381119,
-1.69723921972435,-1.69601660680437,-1.69468557699312,-1.69251822885215,
-1.6850189049682,-1.62888906401457,-1.55123210913802,-1.5471206336117,-1.54005485758152,
-1.53725177005974,-1.53520665040658,-1.53300968839347,-1.5300528838765,
-1.52339923649665,-1.51448732470994,-1.49216475184124,-1.40120640086452,
-1.39713375453935,-1.37866987777084,-1.37564401409106,-1.37410692220622,
-1.37289736368568,-1.37150925279333,-1.36908611389428,-1.35868416845536,
-1.33867537156219,-1.26448736477213,-1.24604259680287,-1.24474684748415,
-1.22073604873522,-1.21627691660736,-1.21348996404287,-1.21131783025235,
-1.20891971810611,-1.20499748437284,-1.1911423305844,-1.16801659902872,
-1.07231322063664,-1.05557206801261,-1.0528895752296,-1.05129602192942,
-1.05007622009373,-1.04873550241299,-1.04652563350474,-1.03860937833421,
-0.975893656646214,-0.89903356947111,-0.893254984098914,-0.890462776620163,
-0.888289796714404,-0.885894047037265,-0.881983139126685,-0.868243816872639,
-0.845382206504173,-0.755778912812782,-0.749368840161065,-0.732556805166441,
-0.729870738587598,-0.728276089402476,-0.727056060560214,-0.725715748591423,
-0.723507933882403,-0.715781123137751,-0.698279883412001),.UNSPECIFIED.);
#7790=B_SPLINE_CURVE_WITH_KNOTS('',3,(#73458,#73459,#73460,#73461,#73462,
#73463,#73464,#73465,#73466,#73467,#73468,#73469,#73470,#73471,#73472,#73473,
#73474,#73475,#73476,#73477,#73478,#73479,#73480,#73481,#73482,#73483,#73484,
#73485,#73486,#73487,#73488,#73489,#73490,#73491,#73492,#73493,#73494,#73495,
#73496,#73497,#73498,#73499,#73500,#73501,#73502,#73503,#73504,#73505,#73506,
#73507,#73508,#73509,#73510,#73511,#73512,#73513,#73514,#73515,#73516,#73517,
#73518,#73519,#73520,#73521,#73522,#73523,#73524,#73525,#73526,#73527,#73528,
#73529,#73530,#73531,#73532,#73533,#73534,#73535,#73536,#73537,#73538,#73539,
#73540,#73541,#73542,#73543,#73544,#73545,#73546,#73547,#73548,#73549,#73550,
#73551,#73552,#73553,#73554,#73555,#73556,#73557,#73558,#73559,#73560,#73561,
#73562,#73563,#73564,#73565,#73566,#73567,#73568,#73569,#73570,#73571,#73572,
#73573,#73574,#73575,#73576,#73577,#73578,#73579,#73580,#73581,#73582,#73583,
#73584,#73585,#73586,#73587,#73588,#73589,#73590,#73591,#73592,#73593,#73594,
#73595,#73596),.UNSPECIFIED.,.F.,.F.,(4,3,3,3,3,3,3,3,3,3,3,3,3,3,3,3,3,
3,3,3,3,3,3,3,3,3,3,3,3,3,3,3,3,3,3,3,3,3,3,3,3,3,3,3,3,3,4),(172.787595947656,
172.8871626731,172.987119762976,173.087281060253,173.187753394168,173.234730606774,
173.327805915243,173.420755166325,173.513605992654,173.606388998097,173.699136852741,
173.791874379014,173.884626384218,173.97747758313,174.070380601293,174.163438942506,
174.234245745301,174.32732105377,174.420270304851,174.513121131181,174.605904136624,
174.698651991267,174.79138951754,174.884141522745,174.976992721657,175.069895739819,
175.162954081032,175.233760883828,175.326836192297,175.419785443378,175.512636269708,
175.605419275151,175.698167129794,175.790904656067,175.883656661271,175.976507860183,
176.069410878346,176.162469219559,176.233276022354,176.326332345594,176.419271252874,
176.512117763458,176.604896810671,176.697643619617,176.79037247548,176.883129099829,
176.910835117971),.UNSPECIFIED.);
#7791=B_SPLINE_CURVE_WITH_KNOTS('',3,(#73597,#73598,#73599,#73600,#73601,
#73602,#73603,#73604,#73605,#73606,#73607,#73608,#73609,#73610,#73611,#73612,
#73613,#73614,#73615,#73616,#73617,#73618,#73619,#73620,#73621,#73622,#73623,
#73624,#73625,#73626,#73627,#73628,#73629,#73630,#73631,#73632,#73633,#73634,
#73635,#73636,#73637,#73638,#73639,#73640,#73641,#73642,#73643,#73644,#73645,
#73646,#73647,#73648,#73649,#73650,#73651,#73652,#73653,#73654,#73655,#73656,
#73657,#73658,#73659,#73660,#73661,#73662,#73663,#73664,#73665,#73666,#73667,
#73668,#73669),.UNSPECIFIED.,.F.,.F.,(4,3,3,3,3,3,3,3,3,3,3,3,3,3,3,3,3,
3,3,3,3,3,3,3,4),(170.6284544512,170.721197866704,170.813936466662,170.906695057718,
170.999555836272,171.092473388744,171.185540126405,171.235700329721,171.32877563819,
171.421724889271,171.514575715601,171.607358721043,171.700106575687,171.79284410196,
171.885596107164,171.978447306076,172.071350324239,172.164408665452,172.235215468247,
172.331063150332,172.426755440666,172.522271127769,172.617683064162,172.712989713064,
172.787595947439),.UNSPECIFIED.);
#7792=B_SPLINE_CURVE_WITH_KNOTS('',3,(#73671,#73672,#73673,#73674,#73675,
#73676,#73677,#73678,#73679,#73680,#73681,#73682,#73683,#73684,#73685,#73686,
#73687,#73688,#73689,#73690,#73691,#73692,#73693,#73694,#73695,#73696,#73697,
#73698,#73699,#73700,#73701,#73702,#73703,#73704,#73705,#73706,#73707,#73708,
#73709,#73710,#73711,#73712,#73713,#73714,#73715,#73716,#73717,#73718,#73719,
#73720,#73721,#73722,#73723,#73724,#73725,#73726,#73727,#73728,#73729,#73730,
#73731,#73732,#73733,#73734,#73735,#73736,#73737,#73738,#73739,#73740,#73741,
#73742,#73743,#73744,#73745,#73746,#73747,#73748,#73749,#73750,#73751,#73752,
#73753,#73754,#73755,#73756,#73757,#73758),.UNSPECIFIED.,.F.,.F.,(4,2,2,
2,2,2,2,2,2,2,2,2,2,2,2,2,2,2,2,2,2,2,2,2,2,2,2,2,2,2,2,2,2,2,2,2,2,2,2,
2,2,2,2,4),(-0.698279883412001,-0.655716239155022,-0.582384763997299,-0.580089716678059,
-0.571647991594463,-0.568292023643063,-0.566245027112785,-0.564048275461205,
-0.561889775826729,-0.556910973500573,-0.52418670685209,-0.461881483768417,
-0.429319886945314,-0.425595040338129,-0.409551507910414,-0.406903546297833,
-0.405320093762229,-0.404101759828532,-0.402755900656432,-0.400523120639394,
-0.392568704408371,-0.378793281726092,-0.345569525091147,-0.306496731668398,
-0.253420285334502,-0.248068499169068,-0.245323342899425,-0.243292601448471,
-0.241084199689339,-0.238904706007487,-0.235992792150057,-0.22194899313286,
-0.185427869244203,-0.157367425044713,-0.110411449899891,-0.0872156099288681,
-0.0839625211221422,-0.0824004538400775,-0.0811882228664128,-0.0798157059024843,
-0.0774634337029379,-0.0746186557645858,-0.0688073377720556,-0.000960765454798418),
 .UNSPECIFIED.);
#7793=B_SPLINE_CURVE_WITH_KNOTS('',3,(#73759,#73760,#73761,#73762,#73763,
#73764,#73765,#73766,#73767,#73768,#73769,#73770,#73771,#73772,#73773,#73774,
#73775,#73776,#73777,#73778,#73779,#73780,#73781,#73782,#73783,#73784,#73785,
#73786,#73787,#73788,#73789,#73790,#73791,#73792,#73793,#73794,#73795,#73796,
#73797,#73798,#73799,#73800,#73801,#73802,#73803,#73804,#73805,#73806,#73807,
#73808,#73809,#73810,#73811,#73812,#73813,#73814,#73815,#73816,#73817,#73818,
#73819,#73820,#73821,#73822,#73823,#73824,#73825,#73826,#73827,#73828,#73829,
#73830,#73831,#73832,#73833,#73834,#73835,#73836,#73837,#73838,#73839,#73840,
#73841,#73842,#73843,#73844,#73845,#73846,#73847,#73848,#73849,#73850,#73851,
#73852,#73853,#73854,#73855,#73856,#73857,#73858,#73859,#73860,#73861,#73862,
#73863,#73864,#73865,#73866,#73867,#73868,#73869,#73870,#73871,#73872,#73873,
#73874,#73875,#73876,#73877,#73878,#73879,#73880,#73881,#73882,#73883,#73884,
#73885,#73886,#73887,#73888,#73889,#73890,#73891,#73892,#73893,#73894,#73895,
#73896,#73897,#73898,#73899,#73900,#73901,#73902,#73903,#73904,#73905,#73906,
#73907,#73908,#73909,#73910,#73911,#73912,#73913,#73914,#73915,#73916,#73917,
#73918,#73919,#73920),.UNSPECIFIED.,.F.,.F.,(4,2,2,2,2,2,2,2,2,2,2,2,2,
2,2,2,2,2,2,2,2,2,2,2,2,2,2,2,2,2,2,2,2,2,2,2,2,2,2,2,2,2,2,2,2,2,2,2,2,
2,2,2,2,2,2,2,2,2,2,2,2,2,2,2,2,2,2,2,2,2,2,2,2,2,2,2,2,2,2,2,4),(-4.0614106989193,
-3.99228506372147,-3.9876033094368,-3.98469694766783,-3.98251988180079,
-3.98031316472839,-3.97828193046893,-3.97553300655311,-3.97016465951742,
-3.90361299184908,-3.87182005557505,-3.83040509925833,-3.82297583915289,
-3.82077735713258,-3.81943943627122,-3.81821925041248,-3.81662126200902,
-3.8130884750255,-3.75601465138605,-3.71827807558768,-3.683855053423,-3.67179005332648,
-3.66339375805551,-3.6608980041791,-3.65848190585864,-3.65631387026672,
-3.65356015755285,-3.64797400788947,-3.61102704137617,-3.58185610201154,
-3.5087902943652,-3.50054759970581,-3.49817514379088,-3.49678754776283,
-3.49557802092071,-3.49404043260096,-3.49101194429058,-3.47248585425543,
-3.45310768893786,-3.37788492837381,-3.35541179000501,-3.34645631485711,
-3.33982506483717,-3.33684465478391,-3.3346436528514,-3.33260437061923,
-3.32982411963792,-3.32289272752485,-3.31858543406109,-3.24097232964601,
-3.18473761487104,-3.17723174205773,-3.17506364343871,-3.17373240724197,
-3.17250978747459,-3.17089703598277,-3.16728437570639,-3.11928508348387,
-3.05839292779267,-3.03369225449793,-3.01915348230543,-3.01516469340242,
-3.01275174097405,-3.01058280133526,-3.00782284075543,-3.0022062971183,
-2.96431096727881,-2.96194062159995,-2.96100161645296,-2.96004101568985,
-2.88505864429494,-2.86519668185836,-2.85484839930311,-2.85242921512255,
-2.85104194936685,-2.84983222304432,-2.8482937448214,-2.84515920897857,
-2.82506877194222,-2.73229937467288,-2.72904212225825),.UNSPECIFIED.);
#7794=B_SPLINE_CURVE_WITH_KNOTS('',3,(#73926,#73927,#73928,#73929,#73930,
#73931,#73932,#73933,#73934,#73935,#73936,#73937,#73938,#73939,#73940,#73941,
#73942,#73943,#73944,#73945,#73946,#73947,#73948,#73949,#73950,#73951,#73952,
#73953,#73954,#73955,#73956,#73957,#73958,#73959,#73960,#73961,#73962,#73963,
#73964,#73965,#73966,#73967,#73968,#73969,#73970,#73971,#73972,#73973,#73974,
#73975,#73976,#73977,#73978,#73979,#73980,#73981,#73982,#73983,#73984,#73985,
#73986,#73987,#73988,#73989,#73990,#73991,#73992,#73993,#73994,#73995,#73996,
#73997,#73998,#73999,#74000,#74001,#74002,#74003,#74004,#74005,#74006,#74007,
#74008,#74009,#74010,#74011,#74012,#74013,#74014,#74015,#74016,#74017,#74018,
#74019,#74020,#74021,#74022,#74023,#74024,#74025,#74026,#74027,#74028,#74029,
#74030,#74031,#74032,#74033,#74034,#74035,#74036,#74037,#74038,#74039,#74040,
#74041,#74042,#74043,#74044,#74045,#74046,#74047,#74048,#74049,#74050,#74051,
#74052,#74053,#74054,#74055,#74056,#74057,#74058,#74059,#74060,#74061,#74062,
#74063,#74064),.UNSPECIFIED.,.F.,.F.,(4,3,3,3,3,3,3,3,3,3,3,3,3,3,3,3,3,
3,3,3,3,3,3,3,3,3,3,3,3,3,3,3,3,3,3,3,3,3,3,3,3,3,3,3,3,3,4),(179.070781254618,
179.221807303043,179.231821437935,179.324896746404,179.417845997485,179.510696823815,
179.603479829258,179.696227683901,179.788965210175,179.881717215379,179.974568414291,
180.067471432453,180.160529773666,180.231336576461,180.32441188493,180.417361136011,
180.510211962341,180.602994967784,180.695742822427,180.7884803487,180.881232353904,
180.974083552816,181.066986570979,181.160044912192,181.230851714988,181.323927023457,
181.416876274539,181.509727100868,181.602510106311,181.695257960955,181.787995487228,
181.880747492432,181.973598691344,182.066501709507,182.15956005072,182.230366853515,
182.323444406673,182.416395322955,182.513634181647,182.606413472028,182.699157965924,
182.791892484436,182.884641833602,182.97748080292,183.070372307203,183.163394662495,
183.194306192493),.UNSPECIFIED.);
#7795=B_SPLINE_CURVE_WITH_KNOTS('',3,(#74065,#74066,#74067,#74068,#74069,
#74070,#74071,#74072,#74073,#74074,#74075,#74076,#74077,#74078,#74079,#74080,
#74081,#74082,#74083,#74084,#74085,#74086,#74087,#74088,#74089,#74090,#74091,
#74092,#74093,#74094,#74095,#74096,#74097,#74098,#74099,#74100,#74101,#74102,
#74103,#74104,#74105,#74106,#74107,#74108,#74109,#74110,#74111,#74112,#74113,
#74114,#74115,#74116,#74117,#74118,#74119,#74120,#74121,#74122,#74123,#74124,
#74125,#74126,#74127,#74128,#74129,#74130,#74131,#74132,#74133,#74134,#74135,
#74136,#74137,#74138,#74139,#74140),.UNSPECIFIED.,.F.,.F.,(4,3,3,3,3,3,
3,3,3,3,3,3,3,3,3,3,3,3,3,3,3,3,3,3,3,4),(176.910835117971,177.003699424499,
177.09662219951,177.189692119164,177.232791160881,177.32586646935,177.418815720431,
177.511666546761,177.604449552204,177.697197406847,177.789934933121,177.882686938325,
177.975538137237,178.068441155399,178.161499496613,178.232306299408,178.323994332173,
178.417342697453,178.508798385829,178.600197264804,178.69156550965,178.786369445841,
178.877795002929,178.969259727769,179.060827527326,179.070781254415),
 .UNSPECIFIED.);
#7796=B_SPLINE_CURVE_WITH_KNOTS('',3,(#74141,#74142,#74143,#74144,#74145,
#74146,#74147,#74148,#74149,#74150,#74151,#74152,#74153,#74154,#74155,#74156,
#74157,#74158,#74159,#74160,#74161,#74162,#74163,#74164,#74165,#74166,#74167,
#74168,#74169,#74170,#74171,#74172,#74173,#74174,#74175,#74176,#74177,#74178,
#74179,#74180,#74181,#74182,#74183,#74184,#74185,#74186,#74187,#74188,#74189,
#74190,#74191,#74192,#74193,#74194,#74195,#74196,#74197,#74198,#74199,#74200,
#74201,#74202,#74203,#74204,#74205,#74206,#74207,#74208,#74209,#74210,#74211,
#74212,#74213,#74214,#74215,#74216,#74217,#74218,#74219,#74220,#74221,#74222,
#74223,#74224,#74225,#74226,#74227,#74228,#74229,#74230,#74231,#74232,#74233,
#74234,#74235,#74236,#74237,#74238,#74239,#74240,#74241,#74242,#74243,#74244,
#74245,#74246,#74247,#74248,#74249,#74250,#74251,#74252,#74253,#74254,#74255,
#74256,#74257,#74258,#74259,#74260,#74261,#74262,#74263,#74264,#74265,#74266,
#74267,#74268,#74269,#74270,#74271,#74272,#74273,#74274,#74275,#74276,#74277,
#74278,#74279,#74280,#74281,#74282,#74283,#74284,#74285,#74286,#74287,#74288,
#74289,#74290,#74291,#74292,#74293,#74294,#74295,#74296,#74297,#74298,#74299,
#74300,#74301,#74302,#74303,#74304,#74305,#74306,#74307,#74308,#74309,#74310,
#74311,#74312,#74313,#74314,#74315,#74316,#74317,#74318,#74319,#74320,#74321,
#74322,#74323,#74324,#74325,#74326,#74327,#74328,#74329,#74330,#74331,#74332,
#74333,#74334,#74335,#74336,#74337,#74338,#74339,#74340,#74341,#74342,#74343,
#74344,#74345,#74346,#74347,#74348,#74349,#74350,#74351,#74352,#74353,#74354,
#74355,#74356,#74357,#74358,#74359,#74360,#74361,#74362,#74363,#74364,#74365,
#74366,#74367,#74368,#74369,#74370,#74371,#74372,#74373,#74374,#74375,#74376,
#74377,#74378,#74379,#74380,#74381,#74382,#74383,#74384,#74385,#74386,#74387,
#74388,#74389,#74390,#74391,#74392),.UNSPECIFIED.,.F.,.F.,(4,2,2,2,2,2,
2,2,2,2,2,2,2,2,2,2,2,2,2,2,2,2,2,2,2,2,2,2,2,2,2,2,2,2,2,2,2,2,2,2,2,2,
2,2,2,2,2,2,2,2,2,2,2,2,2,2,2,2,2,2,2,2,2,2,2,2,2,2,2,2,2,2,2,2,2,2,2,2,
2,2,2,2,2,2,2,2,2,2,2,2,2,2,2,2,2,2,2,2,2,2,2,2,2,2,2,2,2,2,2,2,2,2,2,2,
2,2,2,2,2,2,2,2,2,2,2,4),(-2.72904212225825,-2.7096651709315,-2.69602545808056,
-2.69212494961878,-2.68973172616695,-2.68755851411208,-2.68476247527617,
-2.67896321621483,-2.60289747541373,-2.55810956252402,-2.54104292983353,
-2.531734842726,-2.52939845241835,-2.52802961859972,-2.52681695116883,-2.52524939679029,
-2.52196743925711,-2.49791946724824,-2.48831897280193,-2.44442462656818,
-2.37821246114565,-2.37121657832867,-2.36819874187792,-2.36599108684224,
-2.36396035244451,-2.36121417440949,-2.35585731864392,-2.28806768611129,
-2.24097684756257,-2.21987855483446,-2.20909205322214,-2.20664071608534,
-2.20524638594833,-2.20403762870615,-2.2025096226319,-2.19952604277416,
-2.18197753713693,-2.1057616669061,-2.05512938201318,-2.04826665240209,
-2.04527229631557,-2.0430688012067,-2.04103272414874,-2.03826530770182,
-2.03140910827594,-1.96482105341071,-1.92029027564777,-1.91226534281901,
-1.88762034289611,-1.88431836815378,-1.88276371444013,-1.88154949997741,
-1.88018835115652,-1.87788636516013,-1.86897814098527,-1.85293841799216,
-1.82864051509322,-1.76889916123524,-1.75624620062414,-1.75442947408398,
-1.72945902116641,-1.72494443156872,-1.72214066848004,-1.71996643204178,
-1.71757709850527,-1.71369419516701,-1.70022795258352,-1.67798121549115,
-1.58749193959003,-1.58071857266496,-1.56420097464093,-1.56152953528697,
-1.55993925426578,-1.55871998778577,-1.55737774395299,-1.5551608703745,
-1.54717265089241,-1.48324292026851,-1.40774467666465,-1.40193223307344,
-1.3991334599275,-1.39695973527136,-1.39456757618578,-1.39067246937472,
-1.37708835451865,-1.35457718661359,-1.26249713958991,-1.24151098694972,
-1.23833977044067,-1.23679385334928,-1.23558327972654,-1.2342005934865,
-1.23180260751651,-1.22173477837889,-1.2026493164265,-1.09681243331176,
-1.09099732815778,-1.08874740821701,-1.08022367300834,-1.07685411898269,
-1.07480477302285,-1.07261004571721,-1.06966802390856,-1.06309704576979,
-1.05432417256677,-1.03248820457026,-0.944742200725109,-0.941821990447943,
-0.918543457617666,-0.91528760267979,-0.913725036381304,-0.912512799338056,
-0.911140692820344,-0.908790086456956,-0.8993135626672,-0.881810415545471,
-0.796462788900646,-0.792002954519274,-0.760893371064953,-0.756081833748309,
-0.753220249612018,-0.751030370257043,-0.748689176677537,-0.74502366105497,
-0.733530766169098,-0.69895630341018),.UNSPECIFIED.);
#7797=B_SPLINE_CURVE_WITH_KNOTS('',3,(#74398,#74399,#74400,#74401,#74402,
#74403,#74404,#74405,#74406,#74407,#74408,#74409,#74410,#74411,#74412,#74413,
#74414,#74415,#74416,#74417,#74418,#74419,#74420,#74421,#74422,#74423,#74424,
#74425,#74426,#74427,#74428,#74429,#74430,#74431,#74432,#74433,#74434,#74435,
#74436,#74437,#74438,#74439,#74440,#74441,#74442,#74443,#74444,#74445,#74446,
#74447,#74448,#74449,#74450,#74451,#74452,#74453,#74454,#74455,#74456,#74457,
#74458,#74459,#74460,#74461,#74462,#74463,#74464,#74465,#74466,#74467,#74468,
#74469,#74470,#74471,#74472,#74473,#74474,#74475,#74476,#74477,#74478,#74479,
#74480,#74481,#74482,#74483,#74484,#74485,#74486,#74487,#74488,#74489,#74490,
#74491,#74492,#74493,#74494,#74495,#74496,#74497,#74498,#74499,#74500,#74501,
#74502,#74503,#74504,#74505,#74506,#74507,#74508,#74509,#74510,#74511,#74512,
#74513,#74514,#74515,#74516,#74517,#74518,#74519,#74520,#74521,#74522,#74523,
#74524,#74525,#74526,#74527,#74528,#74529,#74530,#74531,#74532,#74533,#74534,
#74535,#74536),.UNSPECIFIED.,.F.,.F.,(4,3,3,3,3,3,3,3,3,3,3,3,3,3,3,3,3,
3,3,3,3,3,3,3,3,3,3,3,3,3,3,3,3,3,3,3,3,3,3,3,3,3,3,3,3,3,4),(185.35396656206,
185.445661763843,185.537250107984,185.62876102844,185.720231746724,185.81168834625,
185.903156891666,185.994719296751,186.086333618337,186.178093488036,186.228427407622,
186.321502716091,186.414451967172,186.507302793502,186.600085798945,186.692833653589,
186.785571179862,186.878323185066,186.971174383978,187.064077402141,187.157135743354,
187.227942546149,187.321017854618,187.413967105699,187.506817932029,187.599600937472,
187.692348792115,187.785086318389,187.877838323593,187.970689522505,188.063592540667,
188.156650881881,188.227457684676,188.320532993145,188.413482244226,188.506333070556,
188.599116075998,188.691863930642,188.784601456915,188.877353462119,188.970204661031,
189.063107679194,189.156166020407,189.226972823202,189.320047778457,189.412983705485,
189.478274198416),.UNSPECIFIED.);
#7798=B_SPLINE_CURVE_WITH_KNOTS('',3,(#74537,#74538,#74539,#74540,#74541,
#74542,#74543,#74544,#74545,#74546,#74547,#74548,#74549,#74550,#74551,#74552,
#74553,#74554,#74555,#74556,#74557,#74558,#74559,#74560,#74561,#74562,#74563,
#74564,#74565,#74566,#74567,#74568,#74569,#74570,#74571,#74572,#74573,#74574,
#74575,#74576,#74577,#74578,#74579,#74580,#74581,#74582,#74583,#74584,#74585,
#74586,#74587,#74588,#74589,#74590,#74591,#74592,#74593,#74594,#74595,#74596,
#74597,#74598,#74599,#74600,#74601,#74602,#74603,#74604,#74605,#74606,#74607,
#74608,#74609),.UNSPECIFIED.,.F.,.F.,(4,3,3,3,3,3,3,3,3,3,3,3,3,3,3,3,3,
3,3,3,3,3,3,3,4),(183.194306192493,183.229881992042,183.322957300511,183.415906551592,
183.508757377922,183.601540383365,183.694288238008,183.787025764281,183.879777769486,
183.972628968398,184.06553198656,184.158590327773,184.229397130569,184.322472439038,
184.41542169012,184.508272516449,184.601055521892,184.693803376535,184.786540902809,
184.879292908013,184.972144106925,185.065047125087,185.158105466301,185.228912269095,
185.353966561798),.UNSPECIFIED.);
#7799=B_SPLINE_CURVE_WITH_KNOTS('',3,(#74611,#74612,#74613,#74614,#74615,
#74616,#74617,#74618,#74619,#74620,#74621,#74622,#74623,#74624,#74625,#74626,
#74627,#74628,#74629,#74630,#74631,#74632,#74633,#74634,#74635,#74636,#74637,
#74638,#74639,#74640,#74641,#74642,#74643,#74644,#74645,#74646,#74647,#74648,
#74649,#74650,#74651,#74652,#74653,#74654,#74655,#74656,#74657,#74658,#74659,
#74660,#74661,#74662,#74663,#74664,#74665,#74666,#74667,#74668,#74669,#74670,
#74671,#74672,#74673,#74674,#74675,#74676,#74677,#74678,#74679,#74680,#74681,
#74682,#74683,#74684,#74685,#74686,#74687,#74688),.UNSPECIFIED.,.F.,.F.,
(4,2,2,2,2,2,2,2,2,2,2,2,2,2,2,2,2,2,2,2,2,2,2,2,2,2,2,2,2,2,2,2,2,2,2,
2,2,2,4),(-0.69895630341018,-0.653222363512318,-0.595973469885204,-0.592443956624196,
-0.590846319211679,-0.589625926629394,-0.588495068878159,-0.586538692516284,
-0.580868418552731,-0.547466923850817,-0.495683828749448,-0.438965088257273,
-0.433579876649729,-0.430826256283266,-0.428793471788008,-0.426586925954228,
-0.423576601641367,-0.416624914529298,-0.4072087442495,-0.383095294269286,
-0.313154443422782,-0.273184331142939,-0.269947121986367,-0.268354061644838,
-0.267207245452141,-0.26597284971414,-0.264745458556692,-0.261806726216356,
-0.238946538780567,-0.203054838158422,-0.121755971280362,-0.111837607330222,
-0.108250977057591,-0.106159380370009,-0.103984232393372,-0.101175423469589,
-0.095312231075147,-0.0242159529617381,-0.000961145727620849),
 .UNSPECIFIED.);
#7800=B_SPLINE_CURVE_WITH_KNOTS('',3,(#74689,#74690,#74691,#74692,#74693,
#74694,#74695,#74696,#74697,#74698,#74699,#74700,#74701,#74702,#74703,#74704,
#74705,#74706,#74707,#74708,#74709,#74710,#74711,#74712,#74713,#74714,#74715,
#74716,#74717,#74718,#74719,#74720,#74721,#74722,#74723,#74724,#74725,#74726,
#74727,#74728,#74729,#74730,#74731,#74732,#74733,#74734,#74735,#74736,#74737,
#74738,#74739,#74740,#74741,#74742,#74743,#74744,#74745,#74746,#74747,#74748,
#74749,#74750,#74751,#74752,#74753,#74754,#74755,#74756,#74757,#74758,#74759,
#74760,#74761,#74762,#74763,#74764,#74765,#74766,#74767,#74768,#74769,#74770,
#74771,#74772,#74773,#74774,#74775,#74776,#74777,#74778,#74779,#74780,#74781,
#74782,#74783,#74784,#74785,#74786,#74787,#74788,#74789,#74790,#74791,#74792,
#74793,#74794,#74795,#74796,#74797,#74798,#74799,#74800,#74801,#74802,#74803,
#74804,#74805,#74806,#74807,#74808,#74809,#74810,#74811,#74812,#74813,#74814,
#74815,#74816,#74817,#74818,#74819,#74820,#74821,#74822,#74823,#74824,#74825,
#74826,#74827,#74828,#74829,#74830,#74831,#74832,#74833,#74834,#74835,#74836,
#74837,#74838,#74839,#74840,#74841,#74842,#74843,#74844,#74845,#74846,#74847,
#74848,#74849,#74850,#74851,#74852,#74853,#74854),.UNSPECIFIED.,.F.,.F.,
(4,2,2,2,2,2,2,2,2,2,2,2,2,2,2,2,2,2,2,2,2,2,2,2,2,2,2,2,2,2,2,2,2,2,2,
2,2,2,2,2,2,2,2,2,2,2,2,2,2,2,2,2,2,2,2,2,2,2,2,2,2,2,2,2,2,2,2,2,2,2,2,
2,2,2,2,2,2,2,2,2,2,2,4),(-4.06105614040862,-4.01281509053043,-4.00918237775696,
-4.00715091961412,-4.00577429085302,-4.00444297002081,-4.00322015272408,
-4.00160697777479,-3.99799269723706,-3.95063061388278,-3.93289700077417,
-3.91725583559134,-3.87962863295169,-3.85473739475367,-3.84775867645504,
-3.84474353435691,-3.8425360666918,-3.84050425667464,-3.83775472853369,
-3.83238572033902,-3.77765707346459,-3.74665168036196,-3.70336625740058,
-3.69195226863712,-3.68502734002993,-3.68292407769409,-3.68178582067001,
-3.6805762200488,-3.67904032207358,-3.67602061250708,-3.65769797190969,
-3.65326931918034,-3.63978204584763,-3.56391094538317,-3.52917299141871,
-3.52394190915962,-3.52126000404874,-3.5191181986428,-3.51666235107179,
-3.5124817117955,-3.50379872002775,-3.42153333535804,-3.38535990467376,
-3.37068115605294,-3.36513834285786,-3.36238930390365,-3.36012995751842,
-3.35878476540911,-3.35757256118003,-3.3560108768971,-3.35275979510313,
-3.32962131565407,-3.32150112954287,-3.23813619279374,-3.21678114772272,
-3.20371386731093,-3.19987208624882,-3.19749169098694,-3.19531468560247,
-3.19253857351094,-3.18668871495556,-3.11265819380833,-3.06637870434854,
-3.04897584105275,-3.03953839183453,-3.03719095473982,-3.03581952563101,
-3.03460711186989,-3.03304329301138,-3.02978120372506,-3.00632433996406,
-2.99841654155468,-2.95776715607303,-2.88427405163893,-2.87840260427826,
-2.87559216264935,-2.87341677426765,-2.87132572876852,-2.8677420163138,
-2.85784365320879,-2.77609765754925,-2.73947398900245,-2.72901306494186),
 .UNSPECIFIED.);
#7801=B_SPLINE_CURVE_WITH_KNOTS('',3,(#74860,#74861,#74862,#74863,#74864,
#74865,#74866,#74867,#74868,#74869,#74870,#74871,#74872,#74873,#74874,#74875,
#74876,#74877,#74878,#74879,#74880,#74881,#74882,#74883,#74884,#74885,#74886,
#74887,#74888,#74889,#74890,#74891,#74892,#74893,#74894,#74895,#74896,#74897,
#74898,#74899,#74900,#74901,#74902,#74903,#74904,#74905,#74906,#74907,#74908,
#74909,#74910,#74911,#74912,#74913,#74914,#74915,#74916,#74917,#74918,#74919,
#74920,#74921,#74922,#74923,#74924,#74925,#74926,#74927,#74928,#74929,#74930,
#74931,#74932,#74933,#74934,#74935,#74936,#74937,#74938,#74939,#74940,#74941,
#74942,#74943,#74944,#74945,#74946,#74947,#74948,#74949,#74950,#74951,#74952,
#74953,#74954,#74955,#74956,#74957,#74958,#74959,#74960,#74961,#74962,#74963,
#74964,#74965,#74966,#74967,#74968,#74969,#74970,#74971,#74972,#74973,#74974,
#74975,#74976,#74977,#74978,#74979,#74980,#74981,#74982,#74983,#74984,#74985,
#74986,#74987,#74988,#74989,#74990,#74991,#74992,#74993,#74994,#74995,#74996,
#74997,#74998),.UNSPECIFIED.,.F.,.F.,(4,3,3,3,3,3,3,3,3,3,3,3,3,3,3,3,3,
3,3,3,3,3,3,3,3,3,3,3,3,3,3,3,3,3,3,3,3,3,3,3,3,3,3,3,3,3,4),(191.637151868978,
191.731423354596,191.825732704026,191.920101744143,192.014616768741,192.109217785349,
192.203986010753,192.225518238783,192.318593547252,192.411542798333,192.504393624663,
192.597176630106,192.689924484749,192.782662011022,192.875414016227,192.968265215139,
193.061168233301,193.154226574514,193.225033377309,193.318108685778,193.41105793686,
193.503908763189,193.596691768632,193.689439623275,193.782177149549,193.874929154753,
193.967780353665,194.060683371827,194.15374171304,194.224548515836,194.317623824305,
194.410573075386,194.503423901716,194.596206907159,194.688954761803,194.781692288076,
194.87444429328,194.967295492192,195.060198510355,195.153256851568,195.224063654363,
195.317134501935,195.410084650361,195.502926540283,195.595704635939,195.688454781277,
195.760761063421),.UNSPECIFIED.);
#7802=B_SPLINE_CURVE_WITH_KNOTS('',3,(#74999,#75000,#75001,#75002,#75003,
#75004,#75005,#75006,#75007,#75008,#75009,#75010,#75011,#75012,#75013,#75014,
#75015,#75016,#75017,#75018,#75019,#75020,#75021,#75022,#75023,#75024,#75025,
#75026,#75027,#75028,#75029,#75030,#75031,#75032,#75033,#75034,#75035,#75036,
#75037,#75038,#75039,#75040,#75041,#75042,#75043,#75044,#75045,#75046,#75047,
#75048,#75049,#75050,#75051,#75052,#75053,#75054,#75055,#75056,#75057,#75058,
#75059,#75060,#75061,#75062,#75063,#75064,#75065,#75066,#75067,#75068),
 .UNSPECIFIED.,.F.,.F.,(4,3,3,3,3,3,3,3,3,3,3,3,3,3,3,3,3,3,3,3,3,3,3,4),
(189.478274198416,189.57180091883,189.664556387319,189.757294350647,189.850039618445,
189.944151704266,190.037038229662,190.131763095696,190.226487961729,190.319563270198,
190.41251252128,190.505363347609,190.598146353052,190.690894207695,190.783631733968,
190.876383739173,190.969234938085,191.062137956247,191.155196297461,191.226003100256,
191.328790292394,191.431140646895,191.534146257852,191.63715186881),
 .UNSPECIFIED.);
#7803=B_SPLINE_CURVE_WITH_KNOTS('',3,(#75069,#75070,#75071,#75072,#75073,
#75074,#75075,#75076,#75077,#75078,#75079,#75080,#75081,#75082,#75083,#75084,
#75085,#75086,#75087,#75088,#75089,#75090,#75091,#75092,#75093,#75094,#75095,
#75096,#75097,#75098,#75099,#75100,#75101,#75102,#75103,#75104,#75105,#75106,
#75107,#75108,#75109,#75110,#75111,#75112,#75113,#75114,#75115,#75116,#75117,
#75118,#75119,#75120,#75121,#75122,#75123,#75124,#75125,#75126,#75127,#75128,
#75129,#75130,#75131,#75132,#75133,#75134,#75135,#75136,#75137,#75138,#75139,
#75140,#75141,#75142,#75143,#75144,#75145,#75146,#75147,#75148,#75149,#75150,
#75151,#75152,#75153,#75154,#75155,#75156,#75157,#75158,#75159,#75160,#75161,
#75162,#75163,#75164,#75165,#75166,#75167,#75168,#75169,#75170,#75171,#75172,
#75173,#75174,#75175,#75176,#75177,#75178,#75179,#75180,#75181,#75182,#75183,
#75184,#75185,#75186,#75187,#75188,#75189,#75190,#75191,#75192,#75193,#75194,
#75195,#75196,#75197,#75198,#75199,#75200,#75201,#75202,#75203,#75204,#75205,
#75206,#75207,#75208,#75209,#75210,#75211,#75212,#75213,#75214,#75215,#75216,
#75217,#75218,#75219,#75220,#75221,#75222,#75223,#75224,#75225,#75226,#75227,
#75228,#75229,#75230,#75231,#75232,#75233,#75234,#75235,#75236,#75237,#75238,
#75239,#75240,#75241,#75242,#75243,#75244,#75245,#75246,#75247,#75248,#75249,
#75250,#75251,#75252,#75253,#75254,#75255,#75256,#75257,#75258,#75259,#75260,
#75261,#75262,#75263,#75264,#75265,#75266,#75267,#75268,#75269,#75270,#75271,
#75272,#75273,#75274,#75275,#75276,#75277,#75278,#75279,#75280,#75281,#75282,
#75283,#75284,#75285,#75286,#75287,#75288,#75289,#75290,#75291,#75292,#75293,
#75294,#75295,#75296,#75297,#75298,#75299,#75300,#75301,#75302,#75303,#75304,
#75305,#75306,#75307,#75308,#75309,#75310,#75311,#75312,#75313,#75314),
 .UNSPECIFIED.,.F.,.F.,(4,2,2,2,2,2,2,2,2,2,2,2,2,2,2,2,2,2,2,2,2,2,2,2,
2,2,2,2,2,2,2,2,2,2,2,2,2,2,2,2,2,2,2,2,2,2,2,2,2,2,2,2,2,2,2,2,2,2,2,2,
2,2,2,2,2,2,2,2,2,2,2,2,2,2,2,2,2,2,2,2,2,2,2,2,2,2,2,2,2,2,2,2,2,2,2,2,
2,2,2,2,2,2,2,2,2,2,2,2,2,2,2,2,2,2,2,2,2,2,2,2,2,2,4),(-2.72901306494186,
-2.72477364011638,-2.71640486488902,-2.71415145026102,-2.71280096346963,
-2.71158385092473,-2.71000915187469,-2.70739100514283,-2.69193033226944,
-2.68750566272187,-2.63576830998419,-2.56158533791962,-2.55552669117122,
-2.55268006862981,-2.55049970367852,-2.54842130129309,-2.54490219628208,
-2.53544222733974,-2.44749595013701,-2.41838914949135,-2.40238529547798,
-2.39349142334825,-2.39119028661007,-2.38982910201483,-2.38861448840587,
-2.38705885655547,-2.38375306194745,-2.35901108167993,-2.28438538781544,
-2.23833748639376,-2.23243698840548,-2.22962077866105,-2.22744450301178,
-2.22535534409205,-2.2217817092066,-2.21195290468737,-2.12895815915762,
-2.0931354471405,-2.07866495134814,-2.07039051731158,-2.06814586635709,
-2.06679727495931,-2.06557954094937,-2.06400095361309,-2.06057440453013,
-2.03141688303343,-1.95842185949297,-1.94007620069372,-1.91404559796006,
-1.90947252280475,-1.90668100432502,-1.90450158603502,-1.90212834963577,
-1.8983196141261,-1.8855650713607,-1.86489414908399,-1.81657315048713,-1.78022925891761,
-1.77208955338483,-1.76500916385351,-1.74873667024826,-1.74607715321061,
-1.74449027015011,-1.74327138853623,-1.74192717813143,-1.73970195716114,
-1.73162975110238,-1.66626549521913,-1.59234549952807,-1.58649397242468,
-1.58368735969116,-1.58151241079025,-1.57912380012112,-1.5752454417142,
-1.56182810048295,-1.53969243827198,-1.44991094673835,-1.42619877569986,
-1.42292752427725,-1.4213617844141,-1.42014901582044,-1.41877841679308,
-1.41643524069789,-1.40705154140513,-1.38979259026638,-1.34404220538955,
-1.26929918769843,-1.263462838317,-1.26068910544669,-1.25851218652711,-1.25613006982783,
-1.2522814915,-1.23915287902074,-1.21766047132007,-1.13287256271414,-1.10343549751271,
-1.10000222809799,-1.09842229768116,-1.09720429179256,-1.09585621698809,
-1.09361420501081,-1.08536886914662,-1.07097113259015,-1.03541541954631,
-0.952066357763789,-0.949787545788717,-0.941671350205491,-0.938369985271233,
-0.93633306752268,-0.934128994280459,-0.931134448914878,-0.92427390750016,
-0.876439924359826,-0.821000778995854,-0.780688685812408,-0.777451952840973,
-0.775858898687265,-0.774711981768323,-0.773477367847489,-0.771766465900398,
-0.767701893927945,-0.762050299029744,-0.69862383258841),.UNSPECIFIED.);
#7804=B_SPLINE_CURVE_WITH_KNOTS('',3,(#75320,#75321,#75322,#75323,#75324,
#75325,#75326,#75327,#75328,#75329,#75330,#75331,#75332,#75333,#75334,#75335,
#75336,#75337,#75338,#75339,#75340,#75341,#75342,#75343,#75344,#75345,#75346,
#75347,#75348,#75349,#75350,#75351,#75352,#75353,#75354,#75355,#75356,#75357,
#75358,#75359,#75360,#75361,#75362,#75363,#75364,#75365,#75366,#75367,#75368,
#75369,#75370,#75371,#75372,#75373,#75374,#75375,#75376,#75377,#75378,#75379,
#75380,#75381,#75382,#75383,#75384,#75385,#75386,#75387,#75388,#75389,#75390,
#75391,#75392,#75393,#75394,#75395,#75396,#75397,#75398,#75399,#75400,#75401,
#75402,#75403,#75404,#75405,#75406,#75407,#75408,#75409,#75410,#75411,#75412,
#75413,#75414,#75415,#75416,#75417,#75418,#75419,#75420,#75421,#75422,#75423,
#75424,#75425,#75426,#75427,#75428,#75429,#75430,#75431,#75432,#75433,#75434,
#75435,#75436,#75437,#75438,#75439,#75440,#75441,#75442,#75443,#75444,#75445,
#75446,#75447,#75448,#75449,#75450,#75451,#75452,#75453,#75454,#75455),
 .UNSPECIFIED.,.F.,.F.,(4,3,3,3,3,3,3,3,3,3,3,3,3,3,3,3,3,3,3,3,3,3,3,3,
3,3,3,3,3,3,3,3,3,3,3,3,3,3,3,3,3,3,3,3,3,4),(197.920337176455,198.031805350229,
198.144766608287,198.222609069943,198.315684378412,198.408633629494,198.501484455823,
198.594267461266,198.687015315909,198.779752842183,198.872504847387,198.965356046299,
199.058259064462,199.151317405675,199.22212420847,199.315199516939,199.40814876802,
199.50099959435,199.593782599793,199.686530454436,199.779267980709,199.872019985914,
199.964871184826,200.057774202988,200.150832544201,200.221639346997,200.314714655466,
200.407663906547,200.500514732877,200.59329773832,200.686045592963,200.778783119236,
200.87153512444,200.964386323352,201.057289341515,201.150347682728,201.221154485523,
201.314241596727,201.407173008952,201.500015390413,201.592793663975,201.685532692314,
201.7782898269,201.871052592644,201.963901834055,202.043473694958),
 .UNSPECIFIED.);
#7805=B_SPLINE_CURVE_WITH_KNOTS('',3,(#75456,#75457,#75458,#75459,#75460,
#75461,#75462,#75463,#75464,#75465,#75466,#75467,#75468,#75469,#75470,#75471,
#75472,#75473,#75474,#75475,#75476,#75477,#75478,#75479,#75480,#75481,#75482,
#75483,#75484,#75485,#75486,#75487,#75488,#75489,#75490,#75491,#75492,#75493,
#75494,#75495,#75496,#75497,#75498,#75499,#75500,#75501,#75502,#75503,#75504,
#75505,#75506,#75507,#75508,#75509,#75510,#75511,#75512,#75513,#75514,#75515,
#75516,#75517,#75518,#75519,#75520,#75521,#75522,#75523,#75524,#75525,#75526,
#75527,#75528),.UNSPECIFIED.,.F.,.F.,(4,3,3,3,3,3,3,3,3,3,3,3,3,3,3,3,3,
3,3,3,3,3,3,3,4),(195.760761063421,195.85350774476,195.946350525372,196.039240210634,
196.132291560014,196.22357879289,196.316654101359,196.40960335244,196.502454178769,
196.595237184212,196.687985038856,196.780722565129,196.873474570333,196.966325769245,
197.059228787407,197.15228712862,197.223093931416,197.315631945497,197.408051216362,
197.500377312576,197.592635711061,197.684865852227,197.777078489631,197.86932941234,
197.920337176157),.UNSPECIFIED.);
#7806=B_SPLINE_CURVE_WITH_KNOTS('',3,(#75530,#75531,#75532,#75533,#75534,
#75535,#75536,#75537,#75538,#75539,#75540,#75541,#75542,#75543,#75544,#75545,
#75546,#75547,#75548,#75549,#75550,#75551,#75552,#75553,#75554,#75555,#75556,
#75557,#75558,#75559,#75560,#75561,#75562,#75563,#75564,#75565,#75566,#75567,
#75568,#75569,#75570,#75571,#75572,#75573,#75574,#75575,#75576,#75577,#75578,
#75579,#75580,#75581,#75582,#75583,#75584,#75585,#75586,#75587,#75588,#75589,
#75590,#75591,#75592,#75593,#75594,#75595,#75596,#75597,#75598,#75599,#75600,
#75601,#75602,#75603,#75604,#75605,#75606,#75607,#75608,#75609,#75610,#75611,
#75612,#75613,#75614,#75615,#75616,#75617,#75618,#75619,#75620,#75621,#75622,
#75623,#75624,#75625,#75626,#75627,#75628,#75629,#75630,#75631,#75632,#75633,
#75634,#75635,#75636,#75637,#75638,#75639,#75640,#75641,#75642,#75643,#75644,
#75645,#75646,#75647,#75648,#75649,#75650,#75651,#75652,#75653,#75654,#75655,
#75656,#75657,#75658,#75659,#75660,#75661),.UNSPECIFIED.,.F.,.F.,(4,2,2,
2,2,2,2,2,2,2,2,2,2,2,2,2,2,2,2,2,2,2,2,2,2,2,2,2,2,2,2,2,2,2,2,2,2,2,2,
2,2,2,2,2,2,2,2,2,2,2,2,2,2,2,2,2,2,2,2,2,2,2,2,2,2,4),(-0.69862383258841,
-0.688206000384788,-0.623497102447362,-0.618109859171754,-0.61535552328661,
-0.613322367576281,-0.611159681285807,-0.608261189507177,-0.605021558347607,
-0.599535663912179,-0.561528443492525,-0.491622262480999,-0.481349664126729,
-0.457224093883082,-0.453938725562586,-0.452370224694936,-0.45115713940628,
-0.449788168472257,-0.447452320511715,-0.438156169058778,-0.421125009291424,
-0.371411706140605,-0.300422273982887,-0.294512655811967,-0.291724827940602,
-0.289545903590539,-0.2895211130373,-0.289497431938669,-0.289474802519147,
-0.28945317053688,-0.289432485096465,-0.289412698379625,-0.289393765449707,
-0.289375644026989,-0.289358294325546,-0.28934167885546,-0.289325762273646,
-0.289310511248986,-0.289295894329481,-0.289281881787081,-0.289268445533295,
-0.289255559022813,-0.289243197126645,-0.289231336030225,-0.289217823197679,
-0.289204437977887,-0.289191176814999,-0.289178037708408,-0.289165018682222,
-0.289152117811758,-0.286696323519249,-0.282464003546999,-0.277310946950807,
-0.266822157181432,-0.238722877026035,-0.173853007258257,-0.154236015493879,
-0.134054366045775,-0.130915486417587,-0.129375926588919,-0.128165853573525,
-0.126778746031436,-0.124361179437544,-0.114039305183661,-0.0942556630349844,
-0.000961385530181774),.UNSPECIFIED.);
#7807=B_SPLINE_CURVE_WITH_KNOTS('',3,(#75662,#75663,#75664,#75665,#75666,
#75667,#75668,#75669,#75670,#75671,#75672,#75673,#75674,#75675,#75676,#75677,
#75678,#75679,#75680,#75681,#75682,#75683,#75684,#75685,#75686,#75687,#75688,
#75689,#75690,#75691,#75692,#75693,#75694,#75695,#75696,#75697,#75698,#75699,
#75700,#75701,#75702,#75703,#75704,#75705,#75706,#75707,#75708,#75709,#75710,
#75711,#75712,#75713,#75714,#75715,#75716,#75717,#75718,#75719,#75720,#75721,
#75722,#75723,#75724,#75725,#75726,#75727,#75728,#75729,#75730,#75731,#75732,
#75733,#75734,#75735,#75736,#75737,#75738,#75739,#75740,#75741,#75742,#75743,
#75744,#75745,#75746,#75747,#75748,#75749,#75750,#75751,#75752,#75753,#75754,
#75755,#75756,#75757,#75758,#75759,#75760,#75761,#75762,#75763,#75764,#75765,
#75766,#75767,#75768,#75769,#75770,#75771,#75772,#75773,#75774,#75775,#75776,
#75777,#75778,#75779,#75780,#75781,#75782,#75783,#75784,#75785,#75786,#75787,
#75788,#75789,#75790,#75791,#75792,#75793,#75794,#75795,#75796,#75797,#75798,
#75799,#75800),.UNSPECIFIED.,.F.,.F.,(4,3,3,3,3,3,3,3,3,3,3,3,3,3,3,3,3,
3,3,3,3,3,3,3,3,3,3,3,3,3,3,3,3,3,3,3,3,3,3,3,3,3,3,3,3,3,4),(197.920337176157,
198.014222382866,198.108132654103,198.202090688791,198.296184290483,198.390354989505,
198.484693712474,198.52454513226,198.617620440729,198.710569691811,198.80342051814,
198.896203523583,198.988951378226,199.0816889045,199.174440909704,199.267292108616,
199.360195126778,199.453253467992,199.524060270786,199.617135579255,199.710084830336,
199.802935656666,199.895718662109,199.988466516752,200.081204043025,200.173956048229,
200.266807247141,200.359710265304,200.452768606517,200.523575409313,200.616650717782,
200.709599968864,200.802450795193,200.895233800636,200.98798165528,201.080719181553,
201.173471186757,201.266322385669,201.359225403832,201.452283745045,201.52309054784,
201.616163269426,201.709114923502,201.801956943226,201.894735022355,201.987480895189,
202.043995148801),.UNSPECIFIED.);
#7808=B_SPLINE_CURVE_WITH_KNOTS('',3,(#75806,#75807,#75808,#75809,#75810,
#75811,#75812,#75813,#75814,#75815,#75816,#75817,#75818,#75819,#75820,#75821,
#75822,#75823,#75824,#75825,#75826,#75827,#75828,#75829,#75830,#75831,#75832,
#75833,#75834,#75835,#75836,#75837,#75838,#75839,#75840,#75841,#75842,#75843,
#75844,#75845,#75846,#75847,#75848,#75849,#75850,#75851,#75852,#75853,#75854,
#75855,#75856,#75857,#75858,#75859,#75860,#75861,#75862,#75863,#75864,#75865,
#75866,#75867,#75868,#75869,#75870,#75871,#75872,#75873,#75874,#75875,#75876,
#75877,#75878,#75879,#75880,#75881,#75882,#75883,#75884,#75885,#75886,#75887,
#75888,#75889,#75890,#75891,#75892,#75893,#75894,#75895,#75896,#75897,#75898,
#75899,#75900,#75901,#75902,#75903,#75904,#75905,#75906,#75907,#75908,#75909,
#75910,#75911,#75912,#75913,#75914,#75915,#75916,#75917,#75918,#75919,#75920,
#75921,#75922,#75923,#75924,#75925,#75926,#75927,#75928,#75929,#75930,#75931,
#75932,#75933,#75934,#75935,#75936,#75937,#75938,#75939,#75940,#75941,#75942,
#75943,#75944,#75945,#75946,#75947),.UNSPECIFIED.,.F.,.F.,(4,3,3,3,3,3,
3,3,3,3,3,3,3,3,3,3,3,3,3,3,3,3,3,3,3,3,3,3,3,3,3,3,3,3,3,3,3,3,3,3,3,3,
3,3,3,3,3,4),(204.203522483337,204.219699901104,204.312775209573,204.405724460654,
204.498575286984,204.591358292427,204.68410614707,204.776843673343,204.869595678547,
204.962446877459,205.055349895621,205.148408236835,205.219215039631,205.3122903481,
205.405239599181,205.498090425511,205.590873430954,205.683621285597,205.77635881187,
205.869110817074,205.961962015986,206.054865034149,206.147923375362,206.218730178157,
206.311805486626,206.404754737707,206.497605564037,206.59038856948,206.683136424123,
206.775873950396,206.8686259556,206.961477154512,207.054380172675,207.147438513888,
207.218245316684,207.311320625153,207.404269876235,207.497120702564,207.589903708007,
207.682651562651,207.775389088924,207.868141094128,207.96099229304,208.053895311203,
208.146953652416,208.217760455211,208.310843573954,208.327722804751),
 .UNSPECIFIED.);
#7809=B_SPLINE_CURVE_WITH_KNOTS('',3,(#75948,#75949,#75950,#75951,#75952,
#75953,#75954,#75955,#75956,#75957,#75958,#75959,#75960,#75961,#75962,#75963,
#75964,#75965,#75966,#75967,#75968,#75969,#75970,#75971,#75972,#75973,#75974,
#75975,#75976,#75977,#75978,#75979,#75980,#75981,#75982,#75983,#75984,#75985,
#75986,#75987,#75988,#75989,#75990,#75991,#75992,#75993,#75994,#75995,#75996,
#75997,#75998,#75999,#76000,#76001,#76002,#76003,#76004,#76005,#76006,#76007,
#76008,#76009,#76010,#76011,#76012,#76013,#76014,#76015,#76016,#76017,#76018,
#76019,#76020),.UNSPECIFIED.,.F.,.F.,(4,3,3,3,3,3,3,3,3,3,3,3,3,3,3,3,3,
3,3,3,3,3,3,3,4),(202.043473694958,202.136527332252,202.22066962405,202.313744932519,
202.406694183601,202.49954500993,202.592328015373,202.685075870017,202.77781339629,
202.870565401494,202.963416600406,203.056319618569,203.149377959782,203.220184762577,
203.313000399415,203.405690164659,203.498282027013,203.590807109206,203.683298119373,
203.775780178135,203.868278392127,203.960875689901,204.053526894021,204.146328371649,
204.203522483032),.UNSPECIFIED.);
#7810=B_SPLINE_CURVE_WITH_KNOTS('',3,(#76022,#76023,#76024,#76025,#76026,
#76027,#76028,#76029,#76030,#76031,#76032,#76033,#76034,#76035,#76036,#76037,
#76038,#76039,#76040,#76041,#76042,#76043,#76044,#76045,#76046,#76047,#76048,
#76049,#76050,#76051,#76052,#76053,#76054,#76055,#76056,#76057,#76058,#76059,
#76060,#76061,#76062,#76063,#76064,#76065,#76066,#76067,#76068,#76069,#76070,
#76071,#76072,#76073,#76074,#76075,#76076,#76077,#76078,#76079,#76080,#76081,
#76082,#76083,#76084,#76085,#76086,#76087,#76088,#76089,#76090,#76091,#76092,
#76093,#76094,#76095,#76096,#76097),.UNSPECIFIED.,.F.,.F.,(4,3,3,3,3,3,
3,3,3,3,3,3,3,3,3,3,3,3,3,3,3,3,3,3,3,4),(202.043995148801,202.136738543329,
202.233205329089,202.326087595671,202.419036158692,202.512122828016,202.522605686367,
202.615680994836,202.708630245918,202.801481072247,202.89426407769,202.987011932334,
203.079749458607,203.172501463811,203.265352662723,203.358255680885,203.451314022099,
203.522120824893,203.614889200762,203.707536779099,203.800088879478,203.892570730299,
203.985017664774,204.077444682146,204.169899266479,204.203522483337),
 .UNSPECIFIED.);
#7811=B_SPLINE_CURVE_WITH_KNOTS('',3,(#76098,#76099,#76100,#76101,#76102,
#76103,#76104,#76105,#76106,#76107,#76108,#76109,#76110,#76111,#76112,#76113,
#76114,#76115,#76116,#76117,#76118,#76119,#76120,#76121,#76122,#76123,#76124,
#76125,#76126,#76127,#76128,#76129,#76130,#76131,#76132,#76133,#76134,#76135,
#76136,#76137,#76138,#76139,#76140,#76141,#76142,#76143,#76144,#76145,#76146,
#76147,#76148,#76149,#76150,#76151,#76152,#76153,#76154,#76155,#76156,#76157,
#76158,#76159,#76160,#76161,#76162,#76163,#76164,#76165,#76166,#76167,#76168,
#76169,#76170,#76171,#76172,#76173,#76174,#76175,#76176,#76177,#76178,#76179,
#76180,#76181,#76182,#76183,#76184,#76185,#76186,#76187,#76188,#76189,#76190,
#76191,#76192,#76193,#76194,#76195,#76196,#76197,#76198,#76199,#76200,#76201,
#76202,#76203,#76204,#76205,#76206,#76207,#76208,#76209,#76210,#76211,#76212,
#76213,#76214,#76215,#76216,#76217,#76218,#76219,#76220,#76221,#76222,#76223,
#76224,#76225,#76226,#76227,#76228,#76229,#76230,#76231,#76232,#76233,#76234,
#76235,#76236,#76237,#76238,#76239,#76240,#76241,#76242,#76243,#76244,#76245,
#76246,#76247,#76248,#76249,#76250,#76251,#76252,#76253,#76254,#76255,#76256,
#76257),.UNSPECIFIED.,.F.,.F.,(4,2,2,2,2,2,2,2,2,2,2,2,2,2,2,2,2,2,2,2,
2,2,2,2,2,2,2,2,2,2,2,2,2,2,2,2,2,2,2,2,2,2,2,2,2,2,2,2,2,2,2,2,2,2,2,2,
2,2,2,2,2,2,2,2,2,2,2,2,2,2,2,2,2,2,2,2,2,2,2,4),(-4.05986099759803,-4.02576223123953,
-3.96872201555675,-3.96116384617764,-3.95899062086544,-3.95765841144894,
-3.95643647240339,-3.954826756049,-3.95122967675135,-3.9100451979651,-3.86444290545402,
-3.8271367881249,-3.81211578674789,-3.80215777048877,-3.79870928481081,
-3.79668581398197,-3.79451411551451,-3.79172809227603,-3.78727116476695,
-3.76328723965276,-3.75678359119935,-3.7074043137533,-3.64629138354934,
-3.63847432402484,-3.63627473711878,-3.63493658034862,-3.63371649037272,
-3.63211904573086,-3.62858913687769,-3.57131498764554,-3.51638324418888,
-3.49379665177095,-3.48480907633369,-3.47816462200802,-3.47521520166415,
-3.47300924714719,-3.4709770026663,-3.46822410630542,-3.46284026184193,
-3.39804152928679,-3.32427463907567,-3.31575333375218,-3.31348614838437,
-3.31213279533161,-3.31091680218605,-3.3093484227072,-3.30597434864698,
-3.27887885092024,-3.19369867665139,-3.17095811182818,-3.16192678464934,
-3.15520190713397,-3.15223228821098,-3.15003318425868,-3.14799133516145,
-3.14520089482977,-3.13820949621613,-3.13398935005969,-3.05641953614232,
-3.00015056469761,-2.99264255687667,-2.99047428636812,-2.98914304204955,
-2.98792048552601,-2.98630791357827,-2.98269605167618,-2.93823928713803,
-2.87377305793219,-2.84909369421916,-2.83456419641673,-2.83057639883793,
-2.82816373125916,-2.82599484577514,-2.82323467753118,-2.8188632027548,
-2.79628602049327,-2.78766796436437,-2.78318617050587,-2.75237580113267,
-2.72824210628548),.UNSPECIFIED.);
#7812=B_SPLINE_CURVE_WITH_KNOTS('',3,(#76263,#76264,#76265,#76266,#76267,
#76268,#76269,#76270,#76271,#76272,#76273,#76274,#76275,#76276,#76277,#76278,
#76279,#76280,#76281,#76282,#76283,#76284,#76285,#76286,#76287,#76288,#76289,
#76290,#76291,#76292,#76293,#76294,#76295,#76296,#76297,#76298,#76299,#76300,
#76301,#76302,#76303,#76304,#76305,#76306,#76307,#76308,#76309,#76310,#76311,
#76312,#76313,#76314,#76315,#76316,#76317,#76318,#76319,#76320,#76321,#76322,
#76323,#76324,#76325,#76326,#76327,#76328,#76329,#76330,#76331,#76332,#76333,
#76334,#76335,#76336,#76337,#76338,#76339,#76340,#76341,#76342,#76343,#76344,
#76345,#76346,#76347,#76348,#76349,#76350,#76351,#76352,#76353,#76354,#76355,
#76356,#76357,#76358,#76359,#76360,#76361,#76362,#76363,#76364,#76365,#76366,
#76367,#76368,#76369,#76370,#76371,#76372,#76373,#76374,#76375,#76376,#76377,
#76378,#76379,#76380,#76381,#76382,#76383,#76384,#76385,#76386,#76387,#76388,
#76389,#76390,#76391,#76392,#76393,#76394,#76395,#76396,#76397,#76398,#76399,
#76400,#76401),.UNSPECIFIED.,.F.,.F.,(4,3,3,3,3,3,3,3,3,3,3,3,3,3,3,3,3,
3,3,3,3,3,3,3,3,3,3,3,3,3,3,3,3,3,3,3,3,3,3,3,3,3,3,3,3,3,4),(210.486707790516,
210.578625634296,210.670497716477,210.762349785492,210.85420756602,210.94615796819,
211.038153997138,211.13030926565,211.216305870791,211.30938117926,211.402330430342,
211.495181256671,211.587964262114,211.680712116758,211.773449643031,211.866201648235,
211.959052847147,212.05195586531,212.145014206523,212.215821009318,212.308896317787,
212.401845568869,212.494696395198,212.587479400641,212.680227255284,212.772964781557,
212.865716786762,212.958567985674,213.051471003836,213.144529345049,213.215336147845,
213.308411456314,213.401360707395,213.494211533725,213.586994539168,213.679742393811,
213.772479920084,213.865231925288,213.9580831242,214.050986142363,214.144044483576,
214.214851286371,214.307940588984,214.400878110334,214.493728177278,214.586506318758,
214.610741815597),.UNSPECIFIED.);
#7813=B_SPLINE_CURVE_WITH_KNOTS('',3,(#76402,#76403,#76404,#76405,#76406,
#76407,#76408,#76409,#76410,#76411,#76412,#76413,#76414,#76415,#76416,#76417,
#76418,#76419,#76420,#76421,#76422,#76423,#76424,#76425,#76426,#76427,#76428,
#76429,#76430,#76431,#76432,#76433,#76434,#76435,#76436,#76437,#76438,#76439,
#76440,#76441,#76442,#76443,#76444,#76445,#76446,#76447,#76448,#76449,#76450,
#76451,#76452,#76453,#76454,#76455,#76456,#76457,#76458,#76459,#76460,#76461,
#76462,#76463,#76464,#76465,#76466,#76467,#76468,#76469,#76470,#76471,#76472,
#76473,#76474),.UNSPECIFIED.,.F.,.F.,(4,3,3,3,3,3,3,3,3,3,3,3,3,3,3,3,3,
3,3,3,3,3,3,3,4),(208.327722804751,208.420652133282,208.513488042509,208.606262819109,
208.699006954437,208.791745266695,208.884502562575,208.977361508141,209.070276321948,
209.163341423797,209.217275593738,209.310350902207,209.403300153288,209.496150979618,
209.588933985061,209.681681839704,209.774419365978,209.867171371182,209.960022570094,
210.052925588256,210.145983929469,210.216790732264,210.334950410375,210.450987392898,
210.486707790339),.UNSPECIFIED.);
#7814=B_SPLINE_CURVE_WITH_KNOTS('',3,(#76475,#76476,#76477,#76478,#76479,
#76480,#76481,#76482,#76483,#76484,#76485,#76486,#76487,#76488,#76489,#76490,
#76491,#76492,#76493,#76494,#76495,#76496,#76497,#76498,#76499,#76500,#76501,
#76502,#76503,#76504,#76505,#76506,#76507,#76508,#76509,#76510,#76511,#76512,
#76513,#76514,#76515,#76516,#76517,#76518,#76519,#76520,#76521,#76522,#76523,
#76524,#76525,#76526,#76527,#76528,#76529,#76530,#76531,#76532,#76533,#76534,
#76535,#76536,#76537,#76538,#76539,#76540,#76541,#76542,#76543,#76544,#76545,
#76546,#76547,#76548,#76549,#76550,#76551,#76552,#76553,#76554,#76555,#76556,
#76557,#76558,#76559,#76560,#76561,#76562,#76563,#76564,#76565,#76566,#76567,
#76568,#76569,#76570,#76571,#76572,#76573,#76574,#76575,#76576,#76577,#76578,
#76579,#76580,#76581,#76582,#76583,#76584,#76585,#76586,#76587,#76588,#76589,
#76590,#76591,#76592,#76593,#76594,#76595,#76596,#76597,#76598,#76599,#76600,
#76601,#76602,#76603,#76604,#76605,#76606,#76607,#76608,#76609,#76610,#76611,
#76612,#76613,#76614,#76615,#76616,#76617,#76618,#76619,#76620,#76621,#76622,
#76623,#76624,#76625,#76626,#76627,#76628,#76629,#76630,#76631,#76632,#76633,
#76634,#76635,#76636,#76637,#76638,#76639,#76640,#76641,#76642,#76643,#76644,
#76645,#76646,#76647,#76648,#76649,#76650,#76651,#76652,#76653,#76654,#76655,
#76656,#76657,#76658,#76659,#76660,#76661,#76662,#76663,#76664,#76665,#76666,
#76667,#76668,#76669,#76670,#76671,#76672,#76673,#76674,#76675,#76676,#76677,
#76678,#76679,#76680,#76681,#76682,#76683,#76684,#76685,#76686,#76687,#76688,
#76689,#76690,#76691,#76692,#76693,#76694,#76695,#76696,#76697,#76698,#76699,
#76700,#76701,#76702,#76703,#76704,#76705,#76706,#76707,#76708,#76709,#76710,
#76711,#76712,#76713,#76714,#76715,#76716,#76717,#76718,#76719,#76720,#76721,
#76722,#76723,#76724,#76725,#76726,#76727,#76728),.UNSPECIFIED.,.F.,.F.,
(4,2,2,2,2,2,2,2,2,2,2,2,2,2,2,2,2,2,2,2,2,2,2,2,2,2,2,2,2,2,2,2,2,2,2,
2,2,2,2,2,2,2,2,2,2,2,2,2,2,2,2,2,2,2,2,2,2,2,2,2,2,2,2,2,2,2,2,2,2,2,2,
2,2,2,2,2,2,2,2,2,2,2,2,2,2,2,2,2,2,2,2,2,2,2,2,2,2,2,2,2,2,2,2,2,2,2,2,
2,2,2,2,2,2,2,2,2,2,2,2,2,2,2,2,2,2,2,4),(-2.72824210628548,-2.67852407763522,
-2.67287321466086,-2.6688095324003,-2.66709909064221,-2.66586484198403,
-2.66471828953474,-2.66312578185406,-2.65902535892125,-2.64055267506025,
-2.54774833062229,-2.52510852554374,-2.5114665411853,-2.50756594854955,
-2.50517279445116,-2.50299972483053,-2.50020398057078,-2.49440573473097,
-2.41835748719278,-2.37356069082141,-2.35649321346231,-2.34718495941917,
-2.3448486449642,-2.34347987711388,-2.34226728236056,-2.34069984098145,
-2.33741818772582,-2.31337497309463,-2.30378412772626,-2.30091872085506,
-2.25866528852906,-2.22182349637285,-2.20120518060028,-2.18847445192995,
-2.18466896546489,-2.18229687319757,-2.18011791145235,-2.17732615666466,
-2.17275093318077,-2.1466641883321,-2.13214669930338,-2.10263952289169,
-2.07570264161224,-2.03065325308063,-2.0294374316876,-2.02382022735442,
-2.02180480281561,-2.02063687971356,-2.01941507978655,-2.01777911045846,
-2.01413552917229,-1.96425809066924,-1.89487396085978,-1.88902732452201,
-1.86747550260778,-1.86316897048048,-1.86042871358817,-1.85826204701629,
-1.85583784366866,-1.85179817552488,-1.83671275203561,-1.81071424854568,
-1.76123192226472,-1.70357778772267,-1.70005372611599,-1.69845726120448,
-1.69723721782919,-1.69589835975162,-1.69369604001752,-1.68585301898887,
-1.62433239010156,-1.5461605463489,-1.54041984804851,-1.53763543573816,
-1.53546379460622,-1.53306471272793,-1.52913745393183,-1.51522927559619,
-1.4919817953294,-1.39553371564686,-1.37965592789621,-1.37701655758102,
-1.37543572110865,-1.37421787633615,-1.37287090985163,-1.37063274642979,
-1.3624233887018,-1.34811096154892,-1.3128625450552,-1.2290793513748,-1.22700430765647,
-1.21877196034975,-1.21545156787524,-1.21341151436176,-1.21121075714733,
-1.20823258703191,-1.20146112658946,-1.1923507701389,-1.16932960721208,
-1.07425177338058,-1.05678977944133,-1.05381036013184,-1.05228311815893,
-1.0510742634838,-1.0496790235126,-1.04722414799254,-1.03639168413504,-1.01516637589849,
-0.975616759790904,-0.900292475584009,-0.894472192478007,-0.891671752273947,
-0.889497670426158,-0.887106064350868,-0.883213984609284,-0.869661591757753,
-0.847222502185259,-0.758360745244659,-0.734227241895671,-0.730941726183378,
-0.729373242301046,-0.728160209938668,-0.726791342088824,-0.724455769088684,
-0.715345680138289,-0.698729442027986,-0.698305350374428),.UNSPECIFIED.);
#7815=B_SPLINE_CURVE_WITH_KNOTS('',3,(#76734,#76735,#76736,#76737,#76738,
#76739,#76740,#76741,#76742,#76743,#76744,#76745,#76746,#76747,#76748,#76749,
#76750,#76751,#76752,#76753,#76754,#76755,#76756,#76757,#76758,#76759,#76760,
#76761,#76762,#76763,#76764,#76765,#76766,#76767,#76768,#76769,#76770,#76771,
#76772,#76773,#76774,#76775,#76776,#76777,#76778,#76779,#76780,#76781,#76782,
#76783,#76784,#76785,#76786,#76787,#76788,#76789,#76790,#76791,#76792,#76793,
#76794,#76795,#76796,#76797,#76798,#76799,#76800,#76801,#76802,#76803,#76804,
#76805,#76806,#76807,#76808,#76809,#76810,#76811,#76812,#76813,#76814,#76815,
#76816,#76817,#76818,#76819,#76820,#76821,#76822,#76823,#76824,#76825,#76826,
#76827,#76828,#76829,#76830,#76831,#76832,#76833,#76834,#76835,#76836,#76837,
#76838,#76839,#76840,#76841,#76842,#76843,#76844,#76845,#76846,#76847,#76848,
#76849,#76850,#76851,#76852,#76853,#76854,#76855,#76856,#76857,#76858,#76859,
#76860,#76861,#76862,#76863,#76864,#76865,#76866,#76867,#76868,#76869,#76870,
#76871,#76872),.UNSPECIFIED.,.F.,.F.,(4,3,3,3,3,3,3,3,3,3,3,3,3,3,3,3,3,
3,3,3,3,3,3,3,3,3,3,3,3,3,3,3,3,3,3,3,3,3,3,3,3,3,3,3,3,3,4),(216.769893097926,
216.869651071983,216.969811169133,217.070182213147,217.17086776107,217.213396701952,
217.306472010421,217.399421261502,217.492272087832,217.585055093275,217.677802947918,
217.770540474191,217.863292479395,217.956143678307,218.04904669647,218.142105037683,
218.212911840478,218.305987148947,218.398936400028,218.491787226358,218.5845702318,
218.677318086444,218.770055612717,218.862807617921,218.955658816833,219.048561834995,
219.141620176209,219.212426979005,219.305502287474,219.398451538556,219.491302364886,
219.584085370329,219.676833224973,219.769570751246,219.862322756451,219.955173955363,
220.048076973526,220.14113531474,220.211942117532,220.304998119087,220.397936789095,
220.490783146426,220.583562124117,220.676309404351,220.769038764856,220.861797170051,
220.893125340463),.UNSPECIFIED.);
#7816=B_SPLINE_CURVE_WITH_KNOTS('',3,(#76873,#76874,#76875,#76876,#76877,
#76878,#76879,#76880,#76881,#76882,#76883,#76884,#76885,#76886,#76887,#76888,
#76889,#76890,#76891,#76892,#76893,#76894,#76895,#76896,#76897,#76898,#76899,
#76900,#76901,#76902,#76903,#76904,#76905,#76906,#76907,#76908,#76909,#76910,
#76911,#76912,#76913,#76914,#76915,#76916,#76917,#76918,#76919,#76920,#76921,
#76922,#76923,#76924,#76925,#76926,#76927,#76928,#76929,#76930,#76931,#76932,
#76933,#76934,#76935,#76936,#76937,#76938,#76939,#76940,#76941,#76942,#76943,
#76944,#76945),.UNSPECIFIED.,.F.,.F.,(4,3,3,3,3,3,3,3,3,3,3,3,3,3,3,3,3,
3,3,3,3,3,3,3,4),(214.610741815597,214.703484577683,214.796223492791,214.888983367554,
214.981845942894,215.074766162879,215.167834515814,215.214366424898,215.307441733367,
215.400390984448,215.493241810778,215.58602481622,215.678772670864,215.771510197137,
215.864262202342,215.957113401254,216.050016419416,216.14307476063,216.213881563425,
216.309608703086,216.405182094946,216.50058214959,216.595880461535,216.691077732157,
216.769893097696),.UNSPECIFIED.);
#7817=B_SPLINE_CURVE_WITH_KNOTS('',3,(#76947,#76948,#76949,#76950,#76951,
#76952,#76953,#76954,#76955,#76956,#76957,#76958,#76959,#76960,#76961,#76962,
#76963,#76964,#76965,#76966,#76967,#76968,#76969,#76970,#76971,#76972,#76973,
#76974,#76975,#76976,#76977,#76978,#76979,#76980,#76981,#76982,#76983,#76984,
#76985,#76986,#76987,#76988,#76989,#76990,#76991,#76992,#76993,#76994,#76995,
#76996,#76997,#76998,#76999,#77000,#77001,#77002,#77003,#77004,#77005,#77006,
#77007,#77008,#77009,#77010,#77011,#77012,#77013,#77014,#77015,#77016,#77017,
#77018,#77019,#77020,#77021,#77022,#77023,#77024,#77025,#77026,#77027,#77028,
#77029,#77030,#77031,#77032),.UNSPECIFIED.,.F.,.F.,(4,2,2,2,2,2,2,2,2,2,
2,2,2,2,2,2,2,2,2,2,2,2,2,2,2,2,2,2,2,2,2,2,2,2,2,2,2,2,2,2,2,2,4),(-0.698305350374428,
-0.656602296723661,-0.5836007993435,-0.581296347343703,-0.572859560935384,
-0.569504337187169,-0.567457413271066,-0.565260446374895,-0.562365998599244,
-0.556090346092476,-0.525063542871785,-0.463552101857718,-0.428094800229727,
-0.41086283905656,-0.407895258124277,-0.406370511292322,-0.405161787517078,
-0.403764614847878,-0.401301228903959,-0.390569851377794,-0.369562917374765,
-0.311750669171721,-0.254652755354803,-0.249264796733979,-0.246510347511368,
-0.244477230676223,-0.242270594034031,-0.240094263862954,-0.237191031589334,
-0.223294328449439,-0.187307110233393,-0.159451886526668,-0.12645111570544,
-0.104840459848454,-0.0879709537271096,-0.0852821735269327,-0.0836867663510794,
-0.0824666652261892,-0.0811268171269208,-0.0789209138754966,-0.076294655508303,
-0.0710918457574639,-0.000960804717552517),.UNSPECIFIED.);
#7818=B_SPLINE_CURVE_WITH_KNOTS('',3,(#77033,#77034,#77035,#77036,#77037,
#77038,#77039,#77040,#77041,#77042,#77043,#77044,#77045,#77046,#77047,#77048,
#77049,#77050,#77051,#77052,#77053,#77054,#77055,#77056,#77057,#77058,#77059,
#77060,#77061,#77062,#77063,#77064,#77065,#77066,#77067,#77068,#77069,#77070,
#77071,#77072,#77073,#77074,#77075,#77076,#77077,#77078,#77079,#77080,#77081,
#77082,#77083,#77084,#77085,#77086,#77087,#77088,#77089,#77090,#77091,#77092,
#77093,#77094,#77095,#77096,#77097,#77098,#77099,#77100,#77101,#77102,#77103,
#77104,#77105,#77106,#77107,#77108,#77109,#77110,#77111,#77112,#77113,#77114,
#77115,#77116,#77117,#77118,#77119,#77120,#77121,#77122,#77123,#77124,#77125,
#77126,#77127,#77128,#77129,#77130,#77131,#77132,#77133,#77134,#77135,#77136,
#77137,#77138,#77139,#77140,#77141,#77142,#77143,#77144,#77145,#77146,#77147,
#77148,#77149,#77150,#77151,#77152,#77153,#77154,#77155,#77156,#77157,#77158,
#77159,#77160,#77161,#77162,#77163,#77164,#77165,#77166,#77167,#77168,#77169,
#77170,#77171,#77172,#77173,#77174,#77175,#77176,#77177,#77178,#77179,#77180,
#77181,#77182,#77183,#77184,#77185,#77186,#77187,#77188,#77189,#77190),
 .UNSPECIFIED.,.F.,.F.,(4,2,2,2,2,2,2,2,2,2,2,2,2,2,2,2,2,2,2,2,2,2,2,2,
2,2,2,2,2,2,2,2,2,2,2,2,2,2,2,2,2,2,2,2,2,2,2,2,2,2,2,2,2,2,2,2,2,2,2,2,
2,2,2,2,2,2,2,2,2,2,2,2,2,2,2,2,2,2,4),(-4.06074652321885,-4.00420181140675,
-3.99046747971543,-3.98674482363625,-3.98424035421656,-3.98181813822638,
-3.97965121865307,-3.97690789302334,-3.97155361209754,-3.93882987105843,
-3.93475254135369,-3.90520762882977,-3.8730234492749,-3.83125007689878,
-3.82362382756395,-3.82138927291519,-3.82004326991225,-3.81882544732652,
-3.81724352392913,-3.81379724292883,-3.75215627857054,-3.70260485625695,
-3.67926851237964,-3.66536382420609,-3.66144859956524,-3.65903440907588,
-3.65686599649988,-3.65410895013348,-3.64850613561617,-3.61103029927893,
-3.55822868792299,-3.50356807558886,-3.4996998197946,-3.497990063621,-3.49675603121309,
-3.49560946577059,-3.49401663354439,-3.49077951948604,-3.45026773922722,
-3.37510109841307,-3.35479905282181,-3.34647261850833,-3.34021854013855,
-3.33734456972756,-3.33515162047842,-3.33310015854671,-3.3297184103972,
-3.32112023375118,-3.31910826908826,-3.24301297294014,-3.18148255110523,
-3.17698672771155,-3.17520505285234,-3.17395741806212,-3.17282663671404,
-3.17129486673413,-3.16830044296302,-3.14295811528901,-3.13611906064314,
-3.05370880117024,-3.03243234602709,-3.01940152557661,-3.01556419497734,
-3.01318516247597,-3.01100847128319,-3.00823148459069,-3.0023749898022,
-2.9287361382604,-2.88222220729951,-2.86474412707506,-2.8552786728533,-2.85292930212111,
-2.85155765059864,-2.85034563626801,-2.84878312725429,-2.84552656855973,
-2.82221202367707,-2.73218752784015,-2.72845886412415),.UNSPECIFIED.);
#7819=B_SPLINE_CURVE_WITH_KNOTS('',3,(#77196,#77197,#77198,#77199,#77200,
#77201,#77202,#77203,#77204,#77205,#77206,#77207,#77208,#77209,#77210,#77211,
#77212,#77213,#77214,#77215,#77216,#77217,#77218,#77219,#77220,#77221,#77222,
#77223,#77224,#77225,#77226,#77227,#77228,#77229,#77230,#77231,#77232,#77233,
#77234,#77235,#77236,#77237,#77238,#77239,#77240,#77241,#77242,#77243,#77244,
#77245,#77246,#77247,#77248,#77249,#77250,#77251,#77252,#77253,#77254,#77255,
#77256,#77257,#77258,#77259,#77260,#77261,#77262,#77263,#77264,#77265,#77266,
#77267,#77268,#77269,#77270,#77271,#77272,#77273,#77274,#77275,#77276,#77277,
#77278,#77279,#77280,#77281,#77282,#77283,#77284,#77285,#77286,#77287,#77288,
#77289,#77290,#77291,#77292,#77293,#77294,#77295,#77296,#77297,#77298,#77299,
#77300,#77301,#77302,#77303,#77304,#77305,#77306,#77307,#77308,#77309,#77310,
#77311,#77312,#77313,#77314,#77315,#77316,#77317,#77318,#77319,#77320,#77321,
#77322,#77323,#77324,#77325,#77326,#77327,#77328,#77329,#77330,#77331),
 .UNSPECIFIED.,.F.,.F.,(4,3,3,3,3,3,3,3,3,3,3,3,3,3,3,3,3,3,3,3,3,3,3,3,
3,3,3,3,3,3,3,3,3,3,3,3,3,3,3,3,3,3,3,3,3,4),(223.053078404875,223.210487533112,
223.303562841579,223.396512092659,223.489362918987,223.582145924429,223.674893779071,
223.767631305342,223.860383310545,223.953234509456,224.046137527617,224.139195868829,
224.210002671639,224.303077980105,224.396027231183,224.48887805751,224.581661062949,
224.67440891759,224.76714644386,224.859898449061,224.95274964797,225.045652666129,
225.13871100734,225.209517810166,225.302593118647,225.395542369741,225.488393196082,
225.581176201537,225.673924056193,225.766661582478,225.859413587694,225.952264786618,
226.045167804792,226.138226146017,226.209032948693,226.302110268686,226.395061011251,
226.492756092736,226.58553529333,226.678279903642,226.771014744662,226.863764622504,
226.956605203468,227.049498463682,227.142524695251,227.176621663132),
 .UNSPECIFIED.);
#7820=B_SPLINE_CURVE_WITH_KNOTS('',3,(#77332,#77333,#77334,#77335,#77336,
#77337,#77338,#77339,#77340,#77341,#77342,#77343,#77344,#77345,#77346,#77347,
#77348,#77349,#77350,#77351,#77352,#77353,#77354,#77355,#77356,#77357,#77358,
#77359,#77360,#77361,#77362,#77363,#77364,#77365,#77366,#77367,#77368,#77369,
#77370,#77371,#77372,#77373,#77374,#77375,#77376,#77377,#77378,#77379,#77380,
#77381,#77382,#77383,#77384,#77385,#77386,#77387,#77388,#77389,#77390,#77391,
#77392,#77393,#77394,#77395,#77396,#77397,#77398,#77399,#77400,#77401,#77402,
#77403,#77404,#77405,#77406,#77407),.UNSPECIFIED.,.F.,.F.,(4,3,3,3,3,3,
3,3,3,3,3,3,3,3,3,3,3,3,3,3,3,3,3,3,3,4),(220.893125340463,220.985991510786,
221.078917020852,221.171988638053,221.211457256059,221.304532564527,221.397481815608,
221.490332641937,221.583115647379,221.675863502022,221.768601028295,221.861353033499,
221.95420423241,222.047107250572,222.140165591785,222.210972394585,222.302663566803,
222.396465421535,222.487924128935,222.579326226343,222.670697886161,222.766293015787,
222.857723389603,222.949193261442,223.040767905907,223.053078404664),
 .UNSPECIFIED.);
#7821=B_SPLINE_CURVE_WITH_KNOTS('',3,(#77408,#77409,#77410,#77411,#77412,
#77413,#77414,#77415,#77416,#77417,#77418,#77419,#77420,#77421,#77422,#77423,
#77424,#77425,#77426,#77427,#77428,#77429,#77430,#77431,#77432,#77433,#77434,
#77435,#77436,#77437,#77438,#77439,#77440,#77441,#77442,#77443,#77444,#77445,
#77446,#77447,#77448,#77449,#77450,#77451,#77452,#77453,#77454,#77455,#77456,
#77457,#77458,#77459,#77460,#77461,#77462,#77463,#77464,#77465,#77466,#77467,
#77468,#77469,#77470,#77471,#77472,#77473,#77474,#77475,#77476,#77477,#77478,
#77479,#77480,#77481,#77482,#77483,#77484,#77485,#77486,#77487,#77488,#77489,
#77490,#77491,#77492,#77493,#77494,#77495,#77496,#77497,#77498,#77499,#77500,
#77501,#77502,#77503,#77504,#77505,#77506,#77507,#77508,#77509,#77510,#77511,
#77512,#77513,#77514,#77515,#77516,#77517,#77518,#77519,#77520,#77521,#77522,
#77523,#77524,#77525,#77526,#77527,#77528,#77529,#77530,#77531,#77532,#77533,
#77534,#77535,#77536,#77537,#77538,#77539,#77540,#77541,#77542,#77543,#77544,
#77545,#77546,#77547,#77548,#77549,#77550,#77551,#77552,#77553,#77554,#77555,
#77556,#77557,#77558,#77559,#77560,#77561,#77562,#77563,#77564,#77565,#77566,
#77567,#77568,#77569,#77570,#77571,#77572,#77573,#77574,#77575,#77576,#77577,
#77578,#77579,#77580,#77581,#77582,#77583,#77584,#77585,#77586,#77587,#77588,
#77589,#77590,#77591,#77592,#77593,#77594,#77595,#77596,#77597,#77598,#77599,
#77600,#77601,#77602,#77603,#77604,#77605,#77606,#77607,#77608,#77609,#77610,
#77611,#77612,#77613,#77614,#77615,#77616,#77617,#77618,#77619,#77620,#77621,
#77622,#77623,#77624,#77625,#77626,#77627,#77628,#77629,#77630,#77631,#77632,
#77633,#77634,#77635,#77636,#77637,#77638,#77639,#77640,#77641,#77642,#77643,
#77644,#77645,#77646,#77647,#77648,#77649,#77650,#77651),.UNSPECIFIED.,
 .F.,.F.,(4,2,2,2,2,2,2,2,2,2,2,2,2,2,2,2,2,2,2,2,2,2,2,2,2,2,2,2,2,2,2,
2,2,2,2,2,2,2,2,2,2,2,2,2,2,2,2,2,2,2,2,2,2,2,2,2,2,2,2,2,2,2,2,2,2,2,2,
2,2,2,2,2,2,2,2,2,2,2,2,2,2,2,2,2,2,2,2,2,2,2,2,2,2,2,2,2,2,2,2,2,2,2,2,
2,2,2,2,2,2,2,2,2,2,2,2,2,2,2,2,2,2,4),(-2.72845886412415,-2.71001279977591,
-2.69657787429951,-2.69269857406263,-2.69031027732171,-2.68813620453566,
-2.68533155419949,-2.67948715661297,-2.60527466696577,-2.55914728337796,
-2.54179073794797,-2.53237180970001,-2.53002637276707,-2.52865564050188,
-2.52744353242815,-2.52587969369927,-2.5226161019591,-2.49909467156313,
-2.43991905172684,-2.37881321260368,-2.37183825355244,-2.36882434268467,
-2.36661762755231,-2.36458640597858,-2.36183751579458,-2.35646928375539,
-2.30151500041319,-2.27032292316156,-2.21287082737795,-2.20839393884449,
-2.20661536930995,-2.20536841789368,-2.20423715498222,-2.20270323302731,
-2.19970015270593,-2.17402919617101,-2.16293092294055,-2.11020944659234,
-2.05482308593342,-2.04866328370565,-2.04579791762929,-2.04361539114066,
-2.04154405610076,-2.03864134239,-2.03096905040347,-1.99518099585338,-1.94535750253001,
-1.88874768203199,-1.88520913094023,-1.88361006582725,-1.88238970260562,
-1.88105227281296,-1.87885604177945,-1.87107282816111,-1.81051782954846,
-1.7377736667202,-1.73545842664585,-1.72702575517347,-1.72367198292562,
-1.72162588679548,-1.71942976397209,-1.71647738319536,-1.70984760486484,
-1.70097567802221,-1.67879259321744,-1.58869294089384,-1.56539872153345,
-1.56214273229629,-1.56058029499789,-1.55936824693066,-1.55799645161876,
-1.55564660270053,-1.54617606268826,-1.5286873839148,-1.48216183136456,
-1.46323556128996,-1.40881717619814,-1.40345244271557,-1.40070427770551,
-1.39867307942983,-1.39646589373025,-1.39345045557174,-1.38646801001133,
-1.32377633119451,-1.28161764831226,-1.25869018225871,-1.24214087145075,
-1.23946814558484,-1.23787760757627,-1.23665844839001,-1.23531664944845,
-1.23310120508212,-1.22512541286547,-1.16139587585269,-1.08569561489839,
-1.07988968784281,-1.07709243740587,-1.07491917577603,-1.07252679925682,
-1.06862970216058,-1.05502230906744,-1.03245745711464,-0.940054888513039,
-0.91946872661804,-0.916313859413043,-0.914771331100262,-0.913561239757791,
-0.912176688746589,-0.909769726874033,-0.899582201415185,-0.880167558926365,
-0.790388161454498,-0.784314923696493,-0.761221371325372,-0.75681819724679,
-0.754048339794272,-0.75187833410778,-0.749471100226588,-0.745507681248915,
-0.73123229426808,-0.707140932609663,-0.698901174862512),.UNSPECIFIED.);
#7822=B_SPLINE_CURVE_WITH_KNOTS('',3,(#77657,#77658,#77659,#77660,#77661,
#77662,#77663,#77664,#77665,#77666,#77667,#77668,#77669,#77670,#77671,#77672,
#77673,#77674,#77675,#77676,#77677,#77678,#77679,#77680,#77681,#77682,#77683,
#77684,#77685,#77686,#77687,#77688,#77689,#77690,#77691,#77692,#77693,#77694,
#77695,#77696,#77697,#77698,#77699,#77700,#77701,#77702,#77703,#77704,#77705,
#77706,#77707,#77708,#77709,#77710,#77711,#77712,#77713,#77714,#77715,#77716,
#77717,#77718,#77719,#77720,#77721,#77722,#77723,#77724,#77725,#77726,#77727,
#77728,#77729,#77730,#77731,#77732,#77733,#77734,#77735,#77736,#77737,#77738,
#77739,#77740,#77741,#77742,#77743,#77744,#77745,#77746,#77747,#77748,#77749,
#77750,#77751,#77752,#77753,#77754,#77755,#77756,#77757,#77758,#77759,#77760,
#77761,#77762,#77763,#77764,#77765,#77766,#77767,#77768,#77769,#77770,#77771,
#77772,#77773,#77774,#77775,#77776,#77777,#77778,#77779,#77780,#77781,#77782,
#77783,#77784,#77785,#77786,#77787,#77788,#77789,#77790,#77791,#77792,#77793,
#77794,#77795),.UNSPECIFIED.,.F.,.F.,(4,3,3,3,3,3,3,3,3,3,3,3,3,3,3,3,3,
3,3,3,3,3,3,3,3,3,3,3,3,3,3,3,3,3,3,3,3,3,3,3,3,3,3,3,3,3,4),(229.336263712314,
229.42794052537,229.51951143474,229.611006217099,229.702461675838,229.793903904296,
229.885358977926,229.976908380405,230.068510528856,230.160257179368,230.2070935028,
230.300168811201,230.393118062213,230.485968888472,230.578751893843,230.671499748413,
230.764237274613,230.856989279742,230.949840478579,231.042743496666,231.135801837804,
231.206608641326,231.299683950353,231.392633201994,231.485484028883,231.578267034885,
231.671014890088,231.763752416918,231.856504422678,231.949355622139,232.042258640847,
232.135316982596,232.206123779853,232.299199087417,232.392148337595,232.484999163024,
232.577782167573,232.670530021328,232.763267546718,232.856019551046,232.948870749098,
233.041773766408,233.134832106789,233.20563891838,233.298712979945,233.391648111515,
233.460568299342),.UNSPECIFIED.);
#7823=B_SPLINE_CURVE_WITH_KNOTS('',3,(#77796,#77797,#77798,#77799,#77800,
#77801,#77802,#77803,#77804,#77805,#77806,#77807,#77808,#77809,#77810,#77811,
#77812,#77813,#77814,#77815,#77816,#77817,#77818,#77819,#77820,#77821,#77822,
#77823,#77824,#77825,#77826,#77827,#77828,#77829,#77830,#77831,#77832,#77833,
#77834,#77835,#77836,#77837,#77838,#77839,#77840,#77841,#77842,#77843,#77844,
#77845,#77846,#77847,#77848,#77849,#77850,#77851,#77852,#77853,#77854,#77855,
#77856,#77857,#77858,#77859,#77860,#77861,#77862,#77863,#77864,#77865,#77866,
#77867,#77868),.UNSPECIFIED.,.F.,.F.,(4,3,3,3,3,3,3,3,3,3,3,3,3,3,3,3,3,
3,3,3,3,3,3,3,4),(227.176621663132,227.208548087219,227.301623395672,227.394572646738,
227.487423473051,227.580206478477,227.672954333105,227.765691859361,227.858443864549,
227.951295063444,228.04419808159,228.137256422787,228.208063225746,228.301138534298,
228.394087785463,228.486938611876,228.579721617402,228.672469472128,228.765206998484,
228.857959003771,228.950810202764,229.043713221007,229.1367715623,229.207578364273,
229.336263712055),.UNSPECIFIED.);
#7824=B_SPLINE_CURVE_WITH_KNOTS('',3,(#77870,#77871,#77872,#77873,#77874,
#77875,#77876,#77877,#77878,#77879,#77880,#77881,#77882,#77883,#77884,#77885,
#77886,#77887,#77888,#77889,#77890,#77891,#77892,#77893,#77894,#77895,#77896,
#77897,#77898,#77899,#77900,#77901,#77902,#77903,#77904,#77905,#77906,#77907,
#77908,#77909,#77910,#77911,#77912,#77913,#77914,#77915,#77916,#77917,#77918,
#77919,#77920,#77921,#77922,#77923,#77924,#77925,#77926,#77927,#77928,#77929,
#77930,#77931,#77932,#77933,#77934,#77935,#77936,#77937,#77938,#77939,#77940,
#77941,#77942,#77943,#77944,#77945,#77946,#77947,#77948,#77949),
 .UNSPECIFIED.,.F.,.F.,(4,2,2,2,2,2,2,2,2,2,2,2,2,2,2,2,2,2,2,2,2,2,2,2,
2,2,2,2,2,2,2,2,2,2,2,2,2,2,2,4),(-0.698901174862512,-0.611495796291315,
-0.596051005993559,-0.593433809350015,-0.591859456069309,-0.590642471395465,
-0.589510302508336,-0.587519147633891,-0.581576145476372,-0.545177789928452,
-0.494622345725019,-0.439993713122243,-0.434626150818557,-0.431877052633319,
-0.429845415760875,-0.427637996498952,-0.424622675931284,-0.417642456949691,
-0.35579623815866,-0.308932067628198,-0.297335225995657,-0.273758642113154,
-0.270492487481298,-0.268927908972513,-0.267715454508635,-0.266580401025271,
-0.265228370368795,-0.261099824300877,-0.229049521682879,-0.202712653639273,
-0.171785000905427,-0.117145974473519,-0.111778219304424,-0.109029046073699,
-0.106997365292933,-0.104789909502786,-0.101774559122264,-0.0947943609913781,
-0.0329865007214043,-0.000961184047303124),.UNSPECIFIED.);
#7825=B_SPLINE_CURVE_WITH_KNOTS('',3,(#77950,#77951,#77952,#77953,#77954,
#77955,#77956,#77957,#77958,#77959,#77960,#77961,#77962,#77963,#77964,#77965,
#77966,#77967,#77968,#77969,#77970,#77971,#77972,#77973,#77974,#77975,#77976,
#77977,#77978,#77979,#77980,#77981,#77982,#77983,#77984,#77985,#77986,#77987,
#77988,#77989,#77990,#77991,#77992,#77993,#77994,#77995,#77996,#77997,#77998,
#77999,#78000,#78001,#78002,#78003,#78004,#78005,#78006,#78007,#78008,#78009,
#78010,#78011,#78012,#78013,#78014,#78015,#78016,#78017,#78018,#78019,#78020,
#78021,#78022,#78023,#78024,#78025,#78026,#78027,#78028,#78029,#78030,#78031,
#78032,#78033,#78034,#78035,#78036,#78037,#78038,#78039,#78040,#78041,#78042,
#78043,#78044,#78045,#78046,#78047,#78048,#78049,#78050,#78051,#78052,#78053,
#78054,#78055,#78056,#78057,#78058,#78059,#78060,#78061,#78062,#78063,#78064,
#78065,#78066,#78067,#78068,#78069,#78070,#78071,#78072,#78073,#78074,#78075,
#78076,#78077,#78078,#78079,#78080,#78081,#78082,#78083,#78084,#78085,#78086,
#78087,#78088),.UNSPECIFIED.,.F.,.F.,(4,3,3,3,3,3,3,3,3,3,3,3,3,3,3,3,3,
3,3,3,3,3,3,3,3,3,3,3,3,3,3,3,3,3,3,3,3,3,3,3,3,3,3,3,3,3,4),(229.336263712055,
229.480732042408,229.509514426589,229.602589735044,229.695538986112,229.788389812428,
229.881172817857,229.973920672487,230.066658198747,230.159410203938,230.252261402838,
230.345164420987,230.438222762188,230.509029565116,230.602104873569,230.695054124635,
230.787904950948,230.880687956375,230.973435811002,231.066173337259,231.158925342446,
231.251776541342,231.344679559487,231.437737900684,231.508544703643,231.601620012195,
231.69456926336,231.787420089773,231.880203095299,231.972950950026,232.065688476382,
232.158440481668,232.251291680662,232.344194698905,232.437253040198,232.50805984217,
232.601138183882,232.694089688861,232.789794782308,232.882574404265,232.975318536495,
233.068052000494,233.160799602059,233.253633237029,233.346518921955,233.439528525831,
233.459730436439),.UNSPECIFIED.);
#7826=B_SPLINE_CURVE_WITH_KNOTS('',3,(#78094,#78095,#78096,#78097,#78098,
#78099,#78100,#78101,#78102,#78103,#78104,#78105,#78106,#78107,#78108,#78109,
#78110,#78111,#78112,#78113,#78114,#78115,#78116,#78117,#78118,#78119,#78120,
#78121,#78122,#78123,#78124,#78125,#78126,#78127,#78128,#78129,#78130,#78131,
#78132,#78133,#78134,#78135,#78136,#78137,#78138,#78139,#78140,#78141,#78142,
#78143,#78144,#78145,#78146,#78147,#78148,#78149,#78150,#78151,#78152,#78153,
#78154,#78155,#78156,#78157,#78158,#78159,#78160,#78161,#78162,#78163,#78164,
#78165,#78166,#78167,#78168,#78169,#78170,#78171,#78172,#78173,#78174,#78175,
#78176,#78177,#78178,#78179,#78180,#78181,#78182,#78183,#78184,#78185,#78186,
#78187,#78188,#78189,#78190,#78191,#78192,#78193,#78194,#78195,#78196,#78197,
#78198,#78199,#78200,#78201,#78202,#78203,#78204,#78205,#78206,#78207,#78208,
#78209,#78210,#78211,#78212,#78213,#78214,#78215,#78216,#78217,#78218,#78219,
#78220,#78221,#78222,#78223,#78224,#78225,#78226,#78227,#78228,#78229,#78230,
#78231,#78232),.UNSPECIFIED.,.F.,.F.,(4,3,3,3,3,3,3,3,3,3,3,3,3,3,3,3,3,
3,3,3,3,3,3,3,3,3,3,3,3,3,3,3,3,3,3,3,3,3,3,3,3,3,3,3,3,3,4),(235.619449019234,
235.713813979303,235.80821992053,235.907211023888,236.001831808201,236.096541649386,
236.191416982274,236.20418433396,236.297259643421,236.390208895436,236.483059722638,
236.575842728861,236.668590584227,236.761328111166,236.854080116978,236.946931316405,
237.039834335032,237.132892676623,237.203699472487,237.29677480437,237.389724078969,
237.482574928889,237.575357957936,237.668105836185,237.760843386037,237.853595414767,
237.946446636975,238.039349678344,238.132408042374,238.203214611014,238.296289867411,
238.389239066424,238.482089840753,238.574872794507,238.667620597668,238.760358072723,
238.853110027033,238.945961175863,239.038864144314,239.131922436942,239.20272974954,
239.295800196545,239.388750028471,239.481591937618,239.574370085677,239.667121342208,
239.743047127969),.UNSPECIFIED.);
#7827=B_SPLINE_CURVE_WITH_KNOTS('',3,(#78233,#78234,#78235,#78236,#78237,
#78238,#78239,#78240,#78241,#78242,#78243,#78244,#78245,#78246,#78247,#78248,
#78249,#78250,#78251,#78252,#78253,#78254,#78255,#78256,#78257,#78258,#78259,
#78260,#78261,#78262,#78263,#78264,#78265,#78266,#78267,#78268,#78269,#78270,
#78271,#78272,#78273,#78274,#78275,#78276,#78277,#78278,#78279,#78280,#78281,
#78282,#78283,#78284,#78285,#78286,#78287,#78288,#78289,#78290,#78291,#78292,
#78293,#78294,#78295,#78296,#78297,#78298,#78299,#78300,#78301,#78302),
 .UNSPECIFIED.,.F.,.F.,(4,3,3,3,3,3,3,3,3,3,3,3,3,3,3,3,3,3,3,3,3,3,3,4),
(233.460568299342,233.553641519038,233.646395978204,233.739133781382,233.831879737838,
233.925198317605,234.018086306996,234.111620181952,234.205154056907,234.298229369038,
234.391178623795,234.484029453808,234.576812462933,234.669560321256,234.762297851202,
234.855049860068,234.947901062601,235.040804084369,235.133862429124,235.204669195433,
235.308364151342,235.410472004582,235.514960511826,235.61944901907),
 .UNSPECIFIED.);
#7828=B_SPLINE_CURVE_WITH_KNOTS('',3,(#78304,#78305,#78306,#78307,#78308,
#78309,#78310,#78311,#78312,#78313,#78314,#78315,#78316,#78317,#78318,#78319,
#78320,#78321,#78322,#78323,#78324,#78325,#78326,#78327,#78328,#78329,#78330,
#78331,#78332,#78333,#78334,#78335,#78336,#78337,#78338,#78339,#78340,#78341,
#78342,#78343,#78344,#78345,#78346,#78347,#78348,#78349,#78350,#78351,#78352,
#78353,#78354,#78355,#78356,#78357,#78358,#78359,#78360,#78361,#78362,#78363,
#78364,#78365,#78366,#78367,#78368,#78369,#78370,#78371,#78372,#78373,#78374,
#78375,#78376),.UNSPECIFIED.,.F.,.F.,(4,3,3,3,3,3,3,3,3,3,3,3,3,3,3,3,3,
3,3,3,3,3,3,3,4),(233.459730436439,233.507574980696,233.600650289097,233.693599540109,
233.786450366367,233.879233371738,233.971981226308,234.064718752508,234.157470757637,
234.250321956474,234.34322497456,234.436283315698,234.507090119223,234.600165428251,
234.693114679893,234.785965506785,234.878748512788,234.971496367992,235.064233894824,
235.156985900585,235.249837100047,235.342740118756,235.435798460507,235.50660525775,
235.619449019234),.UNSPECIFIED.);
#7829=B_SPLINE_CURVE_WITH_KNOTS('',3,(#78377,#78378,#78379,#78380,#78381,
#78382,#78383,#78384),.UNSPECIFIED.,.F.,.F.,(4,1,1,1,1,4),(235.619457915363,
236.506120396277,237.505635534803,238.50515067333,239.504665811857,239.744094875057),
 .UNSPECIFIED.);
#7830=B_SPLINE_CURVE_WITH_KNOTS('',3,(#78390,#78391,#78392,#78393,#78394,
#78395,#78396,#78397,#78398,#78399,#78400,#78401,#78402,#78403,#78404,#78405,
#78406,#78407,#78408,#78409,#78410,#78411,#78412,#78413,#78414,#78415,#78416,
#78417,#78418,#78419,#78420,#78421,#78422,#78423,#78424,#78425,#78426,#78427,
#78428,#78429,#78430,#78431,#78432,#78433,#78434,#78435,#78436,#78437,#78438,
#78439,#78440,#78441,#78442,#78443,#78444,#78445,#78446,#78447,#78448,#78449,
#78450,#78451,#78452,#78453,#78454,#78455,#78456,#78457,#78458,#78459,#78460,
#78461,#78462,#78463,#78464,#78465,#78466,#78467,#78468,#78469,#78470,#78471,
#78472,#78473,#78474,#78475,#78476,#78477,#78478,#78479,#78480,#78481,#78482,
#78483,#78484,#78485,#78486,#78487,#78488,#78489,#78490,#78491,#78492,#78493,
#78494,#78495,#78496,#78497,#78498,#78499,#78500,#78501,#78502,#78503,#78504,
#78505,#78506,#78507,#78508,#78509,#78510,#78511,#78512,#78513,#78514,#78515,
#78516,#78517,#78518,#78519,#78520,#78521,#78522,#78523,#78524,#78525),
 .UNSPECIFIED.,.F.,.F.,(4,3,3,3,3,3,3,3,3,3,3,3,3,3,3,3,3,3,3,3,3,3,3,3,
3,3,3,3,3,3,3,3,3,3,3,3,3,3,3,3,3,3,3,3,3,4),(241.902634326701,242.014547276602,
242.128011485217,242.201275165121,242.294350730384,242.387300235814,242.480151313763,
242.572934565756,242.665682663774,242.758420429985,242.851172671426,242.944024099428,
243.036927343076,243.12998590156,243.200790303647,243.293866473918,243.386816592658,
243.479668291321,243.572452172529,243.665200904769,243.757939309439,243.850692192807,
243.943544264079,244.036448152747,244.129507352332,244.200305442174,244.293378028059,
244.386324553392,244.479172654295,244.571952945761,244.664698094259,244.757432925305,
244.850182249303,244.943030805156,245.035931197279,245.128986967606,245.199820580701,
245.292909915226,245.385843649138,245.478688419339,245.571469145869,245.664210688667,
245.756971097239,245.849737147195,245.942591646576,246.025775112553),
 .UNSPECIFIED.);
#7831=B_SPLINE_CURVE_WITH_KNOTS('',3,(#78526,#78527,#78528,#78529,#78530,
#78531,#78532,#78533,#78534,#78535,#78536,#78537,#78538,#78539,#78540,#78541,
#78542,#78543,#78544,#78545,#78546,#78547,#78548,#78549,#78550,#78551,#78552,
#78553,#78554,#78555,#78556,#78557,#78558,#78559,#78560,#78561,#78562,#78563,
#78564,#78565,#78566,#78567,#78568,#78569,#78570,#78571,#78572,#78573,#78574,
#78575,#78576,#78577,#78578,#78579,#78580,#78581,#78582,#78583,#78584,#78585,
#78586,#78587,#78588,#78589,#78590,#78591,#78592,#78593,#78594,#78595,#78596,
#78597,#78598),.UNSPECIFIED.,.F.,.F.,(4,3,3,3,3,3,3,3,3,3,3,3,3,3,3,3,3,
3,3,3,3,3,3,3,4),(239.743047127969,239.835794683293,239.928638893887,240.02153087869,
240.114583385812,240.202244888067,240.295320341527,240.38826973839,240.481120711097,
240.573903863212,240.666651864664,240.75938953771,240.85214168948,240.944993033731,
241.037896196778,241.130954680623,241.201760026594,241.29424884327,241.386619345769,
241.478897153144,241.571107792623,241.663291651751,241.755458500974,241.847666146414,
241.902634326414),.UNSPECIFIED.);
#7832=B_SPLINE_CURVE_WITH_KNOTS('',3,(#78600,#78601,#78602,#78603,#78604,
#78605),.UNSPECIFIED.,.F.,.F.,(4,1,1,4),(239.744094875057,240.504180950384,
241.50369608891,241.902627319837),.UNSPECIFIED.);
#7833=B_SPLINE_CURVE_WITH_KNOTS('',3,(#78606,#78607,#78608,#78609,#78610,
#78611,#78612,#78613,#78614,#78615,#78616,#78617,#78618,#78619,#78620,#78621,
#78622,#78623,#78624,#78625,#78626,#78627,#78628,#78629,#78630,#78631,#78632,
#78633,#78634,#78635,#78636,#78637,#78638,#78639,#78640,#78641,#78642,#78643,
#78644,#78645,#78646,#78647,#78648,#78649,#78650,#78651,#78652,#78653,#78654,
#78655,#78656,#78657,#78658,#78659,#78660,#78661,#78662,#78663,#78664,#78665,
#78666,#78667,#78668,#78669,#78670,#78671,#78672,#78673,#78674,#78675,#78676,
#78677,#78678,#78679,#78680,#78681,#78682,#78683,#78684,#78685,#78686,#78687,
#78688,#78689,#78690,#78691,#78692,#78693,#78694,#78695,#78696,#78697,#78698,
#78699,#78700,#78701,#78702,#78703,#78704,#78705,#78706,#78707,#78708,#78709,
#78710,#78711,#78712,#78713,#78714,#78715,#78716,#78717,#78718,#78719,#78720,
#78721,#78722,#78723,#78724,#78725,#78726,#78727,#78728,#78729,#78730,#78731,
#78732,#78733,#78734,#78735,#78736,#78737,#78738,#78739,#78740,#78741,#78742,
#78743,#78744),.UNSPECIFIED.,.F.,.F.,(4,3,3,3,3,3,3,3,3,3,3,3,3,3,3,3,3,
3,3,3,3,3,3,3,3,3,3,3,3,3,3,3,3,3,3,3,3,3,3,3,3,3,3,3,3,3,4),(241.902634326414,
241.996604979565,242.090603522195,242.184652469409,242.278839297194,242.373105210619,
242.467538925424,242.503211227437,242.596286557953,242.689235830694,242.782086678273,
242.87486970427,242.967617579037,243.060355124983,243.153107149387,243.245958366654,
243.338861402733,243.431919760961,243.502726365964,243.59580181966,243.68875121676,
243.781602189705,243.874385342059,243.96713334375,244.059871017034,244.152623169041,
244.245474513527,244.33837767681,244.431436160885,244.502241504491,244.59531643186,
244.688265301624,244.781115746902,244.873898373223,244.966645850041,245.059383000215,
245.152134631479,245.244985462082,245.337888114483,245.430946097903,245.501756643018,
245.594829187545,245.687780746752,245.780622969611,245.873401283084,245.966148308563,
246.026281163792),.UNSPECIFIED.);
#7834=B_SPLINE_CURVE_WITH_KNOTS('',3,(#78750,#78751,#78752,#78753,#78754,
#78755,#78756,#78757,#78758,#78759,#78760,#78761,#78762,#78763,#78764,#78765,
#78766,#78767,#78768,#78769,#78770,#78771,#78772,#78773,#78774,#78775,#78776,
#78777,#78778,#78779,#78780,#78781,#78782,#78783,#78784,#78785,#78786,#78787,
#78788,#78789,#78790,#78791,#78792,#78793,#78794,#78795,#78796,#78797,#78798,
#78799,#78800,#78801,#78802,#78803,#78804,#78805,#78806,#78807,#78808,#78809,
#78810,#78811,#78812,#78813,#78814,#78815,#78816,#78817,#78818,#78819,#78820,
#78821,#78822,#78823,#78824,#78825,#78826,#78827,#78828,#78829,#78830,#78831,
#78832,#78833,#78834,#78835,#78836,#78837,#78838,#78839,#78840,#78841,#78842,
#78843,#78844,#78845,#78846,#78847,#78848,#78849,#78850,#78851,#78852,#78853,
#78854,#78855,#78856,#78857,#78858,#78859,#78860,#78861,#78862,#78863,#78864,
#78865,#78866,#78867,#78868,#78869,#78870,#78871,#78872,#78873,#78874,#78875,
#78876,#78877,#78878,#78879,#78880,#78881,#78882,#78883,#78884,#78885,#78886,
#78887,#78888,#78889,#78890,#78891),.UNSPECIFIED.,.F.,.F.,(4,3,3,3,3,3,
3,3,3,3,3,3,3,3,3,3,3,3,3,3,3,3,3,3,3,3,3,3,3,3,3,3,3,3,3,3,3,3,3,3,3,3,
3,3,3,3,3,4),(248.185819633594,248.198365996281,248.291463087134,248.384434034099,
248.477306443604,248.570110777739,248.662879798763,248.755638305531,248.848411081612,
248.941282600742,249.034205720857,249.127283599223,249.197881134808,249.290981271026,
249.383955651114,249.47683187142,249.569640561775,249.662414271377,249.755177791293,
249.84795589757,249.940833200336,250.033762364561,250.126846646318,250.197396273335,
250.290340851261,250.38315907809,250.475878752769,250.56853093863,250.661148212794,
250.753755544434,250.846377887958,250.939101043765,251.031876711656,251.12481016674,
251.196911411862,251.290167611414,251.38329726983,251.476327792447,251.569288701951,
251.662213301877,251.755126210699,251.848052030612,251.94107355418,252.034145218454,
252.127367725925,252.196426550388,252.289631618365,252.310073042627),
 .UNSPECIFIED.);
#7835=B_SPLINE_CURVE_WITH_KNOTS('',3,(#78892,#78893,#78894,#78895,#78896,
#78897,#78898,#78899,#78900,#78901,#78902,#78903,#78904,#78905,#78906,#78907,
#78908,#78909,#78910,#78911,#78912,#78913,#78914,#78915,#78916,#78917,#78918,
#78919,#78920,#78921,#78922,#78923,#78924,#78925,#78926,#78927,#78928,#78929,
#78930,#78931,#78932,#78933,#78934,#78935,#78936,#78937,#78938,#78939,#78940,
#78941,#78942,#78943,#78944,#78945,#78946,#78947,#78948,#78949,#78950,#78951,
#78952,#78953,#78954,#78955,#78956,#78957,#78958,#78959,#78960,#78961,#78962,
#78963,#78964),.UNSPECIFIED.,.F.,.F.,(4,3,3,3,3,3,3,3,3,3,3,3,3,3,3,3,3,
3,3,3,3,3,3,3,4),(246.025775112553,246.118832148656,246.199335719228,246.292415864885,
246.385369995563,246.478225737109,246.57101369087,246.66376651257,246.756509018734,
246.849266010765,246.942122176217,247.035030157428,247.128093404009,247.198850857755,
247.291703398481,247.384429991938,247.477058559664,247.569620194277,247.662147570796,
247.75466576799,247.847199850451,247.939833337813,248.032520394819,248.125359274108,
248.185819633352),.UNSPECIFIED.);
#7836=B_SPLINE_CURVE_WITH_KNOTS('',3,(#78966,#78967,#78968,#78969,#78970,
#78971,#78972,#78973,#78974,#78975,#78976,#78977,#78978,#78979,#78980,#78981,
#78982,#78983,#78984,#78985,#78986,#78987,#78988,#78989,#78990,#78991,#78992,
#78993,#78994,#78995,#78996,#78997,#78998,#78999,#79000,#79001,#79002,#79003,
#79004,#79005,#79006,#79007,#79008,#79009,#79010,#79011,#79012,#79013,#79014,
#79015,#79016,#79017,#79018,#79019,#79020,#79021,#79022,#79023,#79024,#79025,
#79026,#79027,#79028,#79029,#79030,#79031,#79032,#79033,#79034,#79035,#79036,
#79037,#79038),.UNSPECIFIED.,.F.,.F.,(4,3,3,3,3,3,3,3,3,3,3,3,3,3,3,3,3,
3,3,3,3,3,3,3,4),(246.026281163792,246.119025485589,246.214587059578,246.307471173777,
246.40437147766,246.501271781544,246.594347953035,246.687298073003,246.780149772899,
246.872933655342,246.965682388819,247.058420794725,247.151173679327,247.244025751824,
247.336929641714,247.429988842502,247.500786920071,247.593497367521,247.686087513679,
247.778582742491,247.871008346648,247.963400609079,248.055773554489,248.148176514885,
248.185819633594),.UNSPECIFIED.);
#7837=B_SPLINE_CURVE_WITH_KNOTS('',3,(#79039,#79040,#79041,#79042,#79043,
#79044,#79045,#79046),.UNSPECIFIED.,.F.,.F.,(4,1,1,1,1,4),(248.18582614159,
248.500302058598,249.499817197125,250.499332335651,251.498847474178,252.308677356644),
 .UNSPECIFIED.);
#7838=B_SPLINE_CURVE_WITH_KNOTS('',3,(#79050,#79051,#79052,#79053,#79054,
#79055,#79056,#79057,#79058,#79059,#79060,#79061,#79062,#79063,#79064,#79065,
#79066,#79067,#79068,#79069,#79070,#79071,#79072,#79073,#79074,#79075,#79076,
#79077,#79078,#79079,#79080,#79081,#79082,#79083,#79084,#79085,#79086,#79087,
#79088,#79089,#79090,#79091,#79092,#79093,#79094,#79095,#79096,#79097,#79098,
#79099,#79100,#79101,#79102,#79103,#79104,#79105,#79106,#79107,#79108,#79109,
#79110,#79111,#79112,#79113,#79114,#79115,#79116,#79117,#79118,#79119,#79120,
#79121,#79122),.UNSPECIFIED.,.F.,.F.,(4,3,3,3,3,3,3,3,3,3,3,3,3,3,3,3,3,
3,3,3,3,3,3,3,4),(-4.09274904019422,-3.99806055410705,-3.90933401922389,
-3.82072263115133,-3.73220278454794,-3.64049561342698,-3.55208063682188,
-3.46368033464884,-3.37527351717314,-3.286838995271,-3.19830733410243,-3.10971782729645,
-3.02100177211767,-2.99854541558029,-2.91073114418483,-2.82302915589964,
-2.73541486759979,-2.64786150605922,-2.56033956926054,-2.472826981501,-2.38530167908133,
-2.29768996361524,-2.21003219394396,-2.12224023889375,-2.0613590937516),
 .UNSPECIFIED.);
#7839=B_SPLINE_CURVE_WITH_KNOTS('',3,(#79126,#79127,#79128,#79129,#79130),
 .UNSPECIFIED.,.F.,.F.,(4,1,4),(0.,0.999515138526753,1.11004521091174),
 .UNSPECIFIED.);
#7840=B_SPLINE_CURVE_WITH_KNOTS('',3,(#79132,#79133,#79134,#79135,#79136,
#79137,#79138,#79139,#79140,#79141,#79142,#79143,#79144,#79145,#79146,#79147,
#79148,#79149,#79150,#79151,#79152,#79153,#79154,#79155,#79156,#79157,#79158,
#79159,#79160,#79161,#79162,#79163,#79164,#79165,#79166,#79167,#79168,#79169,
#79170,#79171,#79172,#79173,#79174,#79175,#79176,#79177,#79178,#79179,#79180,
#79181,#79182,#79183,#79184,#79185,#79186,#79187,#79188,#79189,#79190,#79191,
#79192,#79193,#79194,#79195,#79196,#79197,#79198,#79199,#79200,#79201,#79202,
#79203,#79204,#79205,#79206,#79207,#79208,#79209,#79210,#79211,#79212,#79213,
#79214,#79215,#79216,#79217,#79218,#79219,#79220,#79221,#79222,#79223,#79224,
#79225,#79226,#79227,#79228,#79229,#79230,#79231,#79232,#79233,#79234,#79235,
#79236,#79237,#79238,#79239,#79240,#79241,#79242,#79243,#79244,#79245,#79246,
#79247,#79248,#79249,#79250,#79251,#79252,#79253,#79254,#79255,#79256,#79257,
#79258,#79259,#79260,#79261,#79262,#79263,#79264,#79265,#79266,#79267,#79268,
#79269,#79270,#79271,#79272,#79273,#79274,#79275,#79276,#79277,#79278,#79279,
#79280,#79281,#79282,#79283,#79284,#79285,#79286,#79287,#79288,#79289,#79290,
#79291,#79292,#79293,#79294,#79295,#79296,#79297,#79298,#79299,#79300,#79301,
#79302,#79303,#79304,#79305,#79306,#79307,#79308,#79309,#79310,#79311,#79312,
#79313,#79314,#79315,#79316,#79317,#79318,#79319,#79320,#79321,#79322,#79323,
#79324,#79325,#79326,#79327,#79328,#79329,#79330,#79331,#79332,#79333,#79334,
#79335,#79336,#79337,#79338,#79339,#79340,#79341,#79342,#79343,#79344,#79345,
#79346,#79347,#79348,#79349,#79350,#79351,#79352,#79353,#79354,#79355,#79356,
#79357),.UNSPECIFIED.,.F.,.F.,(4,3,3,3,3,3,3,3,3,3,3,3,3,3,3,3,3,3,3,3,
3,3,3,3,3,3,3,3,3,3,3,3,3,3,3,3,3,3,3,3,3,3,3,3,3,3,3,3,3,3,3,3,3,3,3,3,
3,3,3,3,3,3,3,3,3,3,3,3,3,3,3,3,3,3,3,4),(1.11004521091174,1.19654441799083,
1.28293646607715,1.3724481924492,1.45870649482798,1.54494140864206,1.63117580777507,
1.71743256483515,1.80378323591016,1.89018992682975,1.97672445273537,1.99903027705352,
2.08771220340936,2.17627947182013,2.26475572191515,2.35647943362329,2.44485231996562,
2.53321114595239,2.62157713365239,2.70997150502374,2.79846419126683,2.88701535992536,
2.97569427651059,2.99854541558028,3.08725486513629,3.17585242746601,3.26436169446516,
3.3560740519204,3.44448659204278,3.53288746941176,3.62129787310793,3.70973899383516,
3.79828167792104,3.88688480079563,3.97561815529859,3.99806055410704,4.08649685647091,
4.17481697886979,4.26304487091473,4.35486122362961,4.44298432440019,4.53109327174227,
4.61920955868426,4.70735467852735,4.79560005164762,4.8839047331063,4.9723402938607,
4.9975756926338,5.08615468069272,5.17461904443609,5.26299255454003,5.3547548391176,
5.44302609570133,5.53128388824983,5.61954955605335,5.70784443890993,5.79623939193333,
5.88469373435058,5.97327791518406,5.99709083116056,6.0856636771011,6.17412216660342,
6.26249007643259,6.35425456308943,6.4425209458385,6.53077414267478,6.61903549927753,
6.70732636205143,6.79571775052301,6.88416878954928,6.97275007846284,6.99660596968732,
7.09576204967982,7.19407935025374,7.29365481995553,7.39323028965731),
 .UNSPECIFIED.);
#7841=B_SPLINE_CURVE_WITH_KNOTS('',3,(#79359,#79360,#79361,#79362,#79363,
#79364,#79365,#79366,#79367,#79368),.UNSPECIFIED.,.F.,.F.,(4,1,1,1,1,1,
1,4),(7.39323051809133,7.99612110821409,8.99563624674086,9.99515138526763,
10.9946665237944,11.9941816623212,12.9936968008479,13.6764158252709),
 .UNSPECIFIED.);
#7842=B_SPLINE_CURVE_WITH_KNOTS('',3,(#79370,#79371,#79372,#79373,#79374,
#79375,#79376,#79377,#79378,#79379,#79380,#79381,#79382,#79383,#79384,#79385,
#79386,#79387,#79388,#79389,#79390,#79391,#79392,#79393,#79394,#79395,#79396,
#79397,#79398,#79399,#79400,#79401,#79402,#79403,#79404,#79405,#79406,#79407,
#79408,#79409,#79410,#79411,#79412,#79413,#79414,#79415,#79416,#79417,#79418,
#79419,#79420,#79421,#79422,#79423,#79424,#79425,#79426,#79427,#79428,#79429,
#79430,#79431,#79432,#79433,#79434,#79435,#79436,#79437,#79438,#79439,#79440,
#79441,#79442,#79443,#79444,#79445,#79446,#79447,#79448,#79449,#79450,#79451,
#79452,#79453,#79454,#79455,#79456,#79457,#79458,#79459,#79460,#79461,#79462,
#79463,#79464,#79465,#79466,#79467,#79468,#79469,#79470,#79471,#79472,#79473,
#79474,#79475,#79476,#79477,#79478,#79479,#79480,#79481,#79482,#79483,#79484,
#79485,#79486,#79487,#79488,#79489,#79490,#79491,#79492,#79493,#79494,#79495,
#79496,#79497,#79498,#79499,#79500,#79501,#79502,#79503,#79504,#79505,#79506,
#79507,#79508,#79509,#79510,#79511,#79512,#79513,#79514,#79515,#79516,#79517,
#79518,#79519,#79520,#79521,#79522,#79523,#79524,#79525,#79526,#79527,#79528,
#79529,#79530,#79531,#79532,#79533,#79534,#79535,#79536,#79537,#79538,#79539,
#79540,#79541,#79542,#79543,#79544,#79545,#79546,#79547,#79548,#79549,#79550,
#79551,#79552,#79553,#79554,#79555,#79556,#79557,#79558,#79559,#79560,#79561,
#79562,#79563,#79564,#79565,#79566,#79567,#79568,#79569,#79570,#79571,#79572,
#79573,#79574,#79575,#79576,#79577,#79578,#79579,#79580,#79581,#79582,#79583,
#79584,#79585,#79586,#79587,#79588,#79589,#79590,#79591,#79592),
 .UNSPECIFIED.,.F.,.F.,(4,3,3,3,3,3,3,3,3,3,3,3,3,3,3,3,3,3,3,3,3,3,3,3,
3,3,3,3,3,3,3,3,3,3,3,3,3,3,3,3,3,3,3,3,3,3,3,3,3,3,3,3,3,3,3,3,3,3,3,3,
3,3,3,3,3,3,3,3,3,3,3,3,3,3,4),(13.6764160373865,13.7808737156826,13.8870428275287,
13.9932119393747,14.0817664757986,14.1702062997995,14.2585552123784,14.3503266955688,
14.4385733694417,14.5268066274285,14.6150478355601,14.7033183604559,14.7916892311257,
14.880119622141,14.9686802307502,14.9927270779015,15.0812814953253,15.16972119964,
15.2580699919952,15.3498415200493,15.4380880731251,15.5263212103106,15.6145622977665,
15.7028327022423,15.7912034534845,15.8796337255028,15.9681942166741,15.9922422164282,
16.0807965719483,16.1692362130696,16.2575849410238,16.3493564927652,16.4376029788168,
16.5258360481204,16.6140770669054,16.7023474019894,16.7907180831137,16.8791482845041,
16.9677087048413,16.991757354955,17.0803117779812,17.1687514875251,17.2571002847314,
17.3488718108252,17.4371183677683,17.5253515084495,17.6135925990237,17.7018630062345,
17.790233759625,17.8786640334521,17.9672245259167,17.9912724934817,18.0798268952625,
18.1682665833952,18.2566153590514,18.348386893171,18.4366334283541,18.5248665472347,
18.6131076159914,18.7013780013908,18.7897487330894,18.8781789852675,18.9667394563144,
18.9907876320085,19.0788961928086,19.1668903635541,19.2547944509364,19.3428952860973,
19.4307012445493,19.5184950937299,19.6062986484043,19.6946242693592,19.7825588282261,
19.871079980225,19.9596011322238),.UNSPECIFIED.);
#7843=B_SPLINE_CURVE_WITH_KNOTS('',3,(#79594,#79595,#79596,#79597,#79598,
#79599,#79600,#79601,#79602,#79603,#79604,#79605,#79606,#79607,#79608,#79609,
#79610,#79611,#79612,#79613,#79614,#79615,#79616,#79617,#79618,#79619,#79620,
#79621,#79622,#79623,#79624,#79625,#79626,#79627,#79628,#79629,#79630,#79631,
#79632,#79633,#79634,#79635,#79636,#79637,#79638,#79639,#79640,#79641,#79642,
#79643,#79644,#79645,#79646,#79647,#79648,#79649,#79650,#79651,#79652,#79653,
#79654,#79655,#79656,#79657,#79658,#79659,#79660,#79661,#79662,#79663,#79664,
#79665,#79666,#79667,#79668,#79669,#79670,#79671,#79672,#79673,#79674,#79675,
#79676,#79677,#79678,#79679,#79680,#79681,#79682,#79683,#79684,#79685,#79686,
#79687,#79688,#79689,#79690,#79691,#79692,#79693,#79694,#79695,#79696,#79697,
#79698,#79699,#79700,#79701,#79702,#79703,#79704,#79705,#79706,#79707,#79708,
#79709,#79710,#79711,#79712,#79713,#79714,#79715,#79716,#79717,#79718,#79719,
#79720,#79721,#79722,#79723,#79724,#79725,#79726,#79727,#79728,#79729,#79730,
#79731,#79732,#79733,#79734,#79735,#79736,#79737,#79738,#79739,#79740,#79741,
#79742,#79743,#79744,#79745,#79746,#79747,#79748,#79749,#79750,#79751,#79752,
#79753,#79754,#79755,#79756,#79757,#79758,#79759,#79760,#79761,#79762,#79763,
#79764,#79765,#79766,#79767,#79768,#79769,#79770,#79771,#79772,#79773,#79774,
#79775,#79776,#79777,#79778,#79779,#79780,#79781,#79782,#79783,#79784,#79785,
#79786,#79787,#79788,#79789,#79790,#79791,#79792,#79793,#79794,#79795,#79796,
#79797,#79798,#79799,#79800,#79801,#79802,#79803,#79804,#79805,#79806,#79807,
#79808,#79809,#79810,#79811,#79812,#79813,#79814,#79815,#79816,#79817,#79818,
#79819,#79820,#79821,#79822),.UNSPECIFIED.,.F.,.F.,(4,3,3,3,3,3,3,3,3,3,
3,3,3,3,3,3,3,3,3,3,3,3,3,3,3,3,3,3,3,3,3,3,3,3,3,3,3,3,3,3,3,3,3,3,3,3,
3,3,3,3,3,3,3,3,3,3,3,3,3,3,3,3,3,3,3,3,3,3,3,3,3,3,3,3,3,3,4),(19.9596011324505,
19.9903027705352,20.0788571753237,20.1672968664412,20.2556456450556,20.3474171780564,
20.4356637161121,20.5238968378287,20.6121379093813,20.7004082975332,20.7887790319058,
20.8772092867154,20.9657697603104,20.989817909062,21.0783723102708,21.1668119977757,
21.2551607727494,21.3469323071043,21.4351788414715,21.5234119594882,21.6116530273334,
21.6999234117745,21.7882941424499,21.8767243935656,21.9652848635004,21.9893330475888,
22.0778874482409,22.1663271351713,22.2546759095531,22.3464474441234,22.434693977859,
22.5229270952307,22.6111681624178,22.6994385461886,22.7878092761785,22.8762395265992,
22.96479999583,22.9888481861155,23.0774025880603,23.1658422763025,23.2541910520137,
23.3459625860922,23.4342091211927,23.5224422399398,23.6106833085118,23.6989536936755,
23.787324425063,23.8757546768859,23.9643151475147,23.9883633246423,24.0769177260085,
24.1653574136662,24.2537061887876,24.3454777230853,24.4337242575869,24.5219573757327,
24.6101984437018,24.6984688282613,24.7868395590461,24.8752698102663,24.9638302802972,
24.9878784631691,25.0764328645092,25.1648725521388,25.2532213272304,25.3449928615386,
25.4332393960058,25.5214725141157,25.6097135820472,25.6979839665675,25.7863546973111,
25.8747849484889,25.9633454184758,25.9873936016958,26.1024227289662,26.2150525142496,
26.2427863701391),.UNSPECIFIED.);
#7844=B_SPLINE_CURVE_WITH_KNOTS('',3,(#79824,#79825,#79826,#79827,#79828,
#79829,#79830,#79831,#79832,#79833),.UNSPECIFIED.,.F.,.F.,(4,1,1,1,1,1,
1,4),(26.2427864396301,26.9869087402226,27.9864238787494,28.9859390172761,
29.9854541558029,30.9849692943297,31.9844844328564,32.5259717468097),
 .UNSPECIFIED.);
#7845=B_SPLINE_CURVE_WITH_KNOTS('',3,(#79835,#79836,#79837,#79838,#79839,
#79840,#79841,#79842,#79843,#79844,#79845,#79846,#79847,#79848,#79849,#79850,
#79851,#79852,#79853,#79854,#79855,#79856,#79857,#79858,#79859,#79860,#79861,
#79862,#79863,#79864,#79865,#79866,#79867,#79868,#79869,#79870,#79871,#79872,
#79873,#79874,#79875,#79876,#79877,#79878,#79879,#79880,#79881,#79882,#79883,
#79884,#79885,#79886,#79887,#79888,#79889,#79890,#79891,#79892,#79893,#79894,
#79895,#79896,#79897,#79898,#79899,#79900,#79901,#79902,#79903,#79904,#79905,
#79906,#79907,#79908,#79909,#79910,#79911,#79912,#79913,#79914,#79915,#79916,
#79917,#79918,#79919,#79920,#79921,#79922,#79923,#79924,#79925,#79926,#79927,
#79928,#79929,#79930,#79931,#79932,#79933,#79934,#79935,#79936,#79937,#79938,
#79939,#79940,#79941,#79942,#79943,#79944,#79945,#79946,#79947,#79948,#79949,
#79950,#79951,#79952,#79953,#79954,#79955,#79956,#79957,#79958,#79959,#79960,
#79961,#79962,#79963,#79964,#79965,#79966,#79967,#79968,#79969,#79970,#79971,
#79972,#79973,#79974,#79975,#79976,#79977,#79978,#79979,#79980,#79981,#79982,
#79983,#79984,#79985,#79986,#79987,#79988,#79989,#79990,#79991,#79992,#79993,
#79994,#79995,#79996,#79997,#79998,#79999,#80000,#80001,#80002,#80003,#80004,
#80005,#80006,#80007,#80008,#80009,#80010,#80011,#80012,#80013,#80014,#80015,
#80016,#80017,#80018,#80019,#80020,#80021,#80022,#80023,#80024,#80025,#80026,
#80027,#80028,#80029,#80030,#80031,#80032,#80033,#80034,#80035,#80036,#80037,
#80038,#80039,#80040,#80041,#80042,#80043,#80044,#80045,#80046,#80047,#80048,
#80049,#80050,#80051,#80052,#80053,#80054,#80055,#80056,#80057,#80058,#80059,
#80060),.UNSPECIFIED.,.F.,.F.,(4,3,3,3,3,3,3,3,3,3,3,3,3,3,3,3,3,3,3,3,
3,3,3,3,3,3,3,3,3,3,3,3,3,3,3,3,3,3,3,3,3,3,3,3,3,3,3,3,3,3,3,3,3,3,3,3,
3,3,3,3,3,3,3,3,3,3,3,3,3,3,3,3,3,3,3,4),(32.525971971786,32.6201758608884,
32.7147113282288,32.8094143342101,32.9044060802361,32.9839995713832,33.0725539728206,
33.1609936605494,33.2493424357416,33.3411139700126,33.4293605045839,33.517593622799,
33.6058346908367,33.6941050754642,33.7824758063156,33.8709060576017,33.959466527697,
33.9835147099099,34.0720691113478,34.160508799077,34.2488575742697,34.3406291085406,
34.4288756431123,34.5171087613279,34.605349829366,34.6936202139939,34.7819909448457,
34.8704211961323,34.958981666228,34.9830298484367,35.0715842498749,35.1600239376044,
35.2483727127975,35.3401442470682,35.4283907816403,35.5166238998561,35.6048649678946,
35.6931353525228,35.781506083375,35.8699363346619,35.958496804758,35.9825449869634,
36.0710993884013,36.1595390761305,36.2478878513232,36.3396593855941,36.4279059201658,
36.5161390383814,36.6043801064195,36.6926504910474,36.7810212218993,36.8694514731859,
36.9580119432816,36.9820601254902,37.0706145269282,37.1590542146575,37.2474029898504,
37.3391745241212,37.4274210586931,37.5156541769087,37.603895244947,37.6921656295751,
37.7805363604271,37.8689666117138,37.9575270818097,37.981575264017,38.0688080689725,
38.1559267275216,38.2429457173611,38.3299097067977,38.4168412476983,38.5037628572331,
38.5907342193606,38.6777330343992,38.7648291874566,38.8091570539893),
 .UNSPECIFIED.);
#7846=B_SPLINE_CURVE_WITH_KNOTS('',3,(#80062,#80063,#80064,#80065,#80066,
#80067,#80068,#80069,#80070,#80071,#80072),.UNSPECIFIED.,.F.,.F.,(4,1,1,
1,1,1,1,1,4),(38.8091570539893,38.9810904025437,39.9806055410705,40.9801206795973,
41.979635818124,42.9791509566508,43.9786660951776,44.9781812337044,45.0923423611689),
 .UNSPECIFIED.);
#7847=B_SPLINE_CURVE_WITH_KNOTS('',3,(#80074,#80075,#80076,#80077,#80078,
#80079,#80080,#80081,#80082,#80083,#80084,#80085,#80086,#80087,#80088,#80089,
#80090,#80091,#80092,#80093,#80094,#80095,#80096,#80097,#80098,#80099,#80100,
#80101,#80102,#80103,#80104,#80105,#80106,#80107,#80108,#80109,#80110,#80111,
#80112,#80113,#80114,#80115,#80116,#80117,#80118,#80119,#80120,#80121,#80122,
#80123,#80124,#80125,#80126,#80127,#80128,#80129,#80130,#80131,#80132,#80133,
#80134,#80135,#80136,#80137,#80138,#80139,#80140,#80141,#80142,#80143,#80144,
#80145,#80146,#80147,#80148,#80149,#80150,#80151,#80152,#80153,#80154,#80155,
#80156,#80157,#80158,#80159,#80160,#80161,#80162,#80163,#80164,#80165,#80166,
#80167,#80168,#80169,#80170,#80171,#80172,#80173,#80174,#80175,#80176,#80177,
#80178,#80179,#80180,#80181,#80182,#80183,#80184,#80185,#80186,#80187,#80188,
#80189,#80190,#80191,#80192,#80193,#80194,#80195,#80196,#80197,#80198,#80199,
#80200,#80201,#80202,#80203,#80204,#80205,#80206,#80207,#80208,#80209,#80210,
#80211,#80212,#80213,#80214,#80215,#80216,#80217,#80218,#80219,#80220,#80221,
#80222,#80223,#80224,#80225,#80226,#80227,#80228,#80229,#80230,#80231,#80232,
#80233,#80234,#80235,#80236,#80237,#80238,#80239,#80240,#80241,#80242,#80243,
#80244,#80245,#80246,#80247,#80248,#80249,#80250,#80251,#80252,#80253,#80254,
#80255,#80256,#80257,#80258,#80259,#80260,#80261,#80262,#80263,#80264,#80265,
#80266,#80267,#80268,#80269,#80270,#80271,#80272,#80273,#80274,#80275,#80276,
#80277,#80278,#80279,#80280,#80281,#80282,#80283,#80284,#80285,#80286,#80287,
#80288,#80289,#80290,#80291,#80292,#80293,#80294,#80295,#80296),
 .UNSPECIFIED.,.F.,.F.,(4,3,3,3,3,3,3,3,3,3,3,3,3,3,3,3,3,3,3,3,3,3,3,3,
3,3,3,3,3,3,3,3,3,3,3,3,3,3,3,3,3,3,3,3,3,3,3,3,3,3,3,3,3,3,3,3,3,3,3,3,
3,3,3,3,3,3,3,3,3,3,3,3,3,3,4),(45.0923423611689,45.1796430982707,45.2668439792167,
45.3557005283435,45.442782837144,45.5298464622534,45.6169138198322,45.7071094579319,
45.7943002142326,45.8859982932319,45.9776963722311,46.0662507736692,46.1546904613985,
46.2430392365914,46.3348107708622,46.4230573054341,46.5112904236498,46.599531491688,
46.6878018763162,46.7761726071682,46.8646028584548,46.9531633285507,46.9772115107579,
47.065765912196,47.1542055999253,47.242554375118,47.3343259093888,47.4225724439607,
47.5108055621764,47.5990466302145,47.6873170148423,47.7756877456943,47.8641179969809,
47.9526784670765,47.9767266492846,48.0652810507226,48.1537207384518,48.2420695136444,
48.3338410479152,48.4220875824871,48.5103207007027,48.598561768741,48.6868321533692,
48.7752028842212,48.8636331355078,48.9521936056038,48.9762417878114,49.0647961892494,
49.1532358769787,49.2415846521716,49.3333561864424,49.4216027210143,49.50983583923,
49.5980769072683,49.686347291896,49.7747180227479,49.863148274035,49.9517087441309,
49.9757569263381,50.064311327776,50.1527510155053,50.2410997906977,50.3328713249686,
50.4211178595405,50.5093509777562,50.5975920457948,50.6858624304227,50.7742331612748,
50.8626634125615,50.9512238826574,50.9752720648649,51.0753359098083,51.1734347141415,
51.27448107939,51.3755274446384),.UNSPECIFIED.);
#7848=B_SPLINE_CURVE_WITH_KNOTS('',3,(#80298,#80299,#80300,#80301,#80302,
#80303,#80304,#80305,#80306,#80307),.UNSPECIFIED.,.F.,.F.,(4,1,1,1,1,1,
1,4),(51.3755276683485,51.9747872033916,52.9743023419184,53.9738174804452,
54.973332618972,55.9728477574987,56.9723628960255,57.6587129755281),
 .UNSPECIFIED.);
#7849=B_SPLINE_CURVE_WITH_KNOTS('',3,(#80309,#80310,#80311,#80312,#80313,
#80314,#80315,#80316,#80317,#80318,#80319,#80320,#80321,#80322,#80323,#80324,
#80325,#80326,#80327,#80328,#80329,#80330,#80331,#80332,#80333,#80334,#80335,
#80336,#80337,#80338,#80339,#80340,#80341,#80342,#80343,#80344,#80345,#80346,
#80347,#80348,#80349,#80350,#80351,#80352,#80353,#80354,#80355,#80356,#80357,
#80358,#80359,#80360,#80361,#80362,#80363,#80364,#80365,#80366,#80367,#80368,
#80369,#80370,#80371,#80372,#80373,#80374,#80375,#80376,#80377,#80378,#80379,
#80380,#80381,#80382,#80383,#80384,#80385,#80386,#80387,#80388,#80389,#80390,
#80391,#80392,#80393,#80394,#80395,#80396,#80397,#80398,#80399,#80400,#80401,
#80402,#80403,#80404,#80405,#80406,#80407,#80408,#80409,#80410,#80411,#80412,
#80413,#80414,#80415,#80416,#80417,#80418,#80419,#80420,#80421,#80422,#80423,
#80424,#80425,#80426,#80427,#80428,#80429,#80430,#80431,#80432,#80433,#80434,
#80435,#80436,#80437,#80438,#80439,#80440,#80441,#80442,#80443,#80444,#80445,
#80446,#80447,#80448,#80449,#80450,#80451,#80452,#80453,#80454,#80455,#80456,
#80457,#80458,#80459,#80460,#80461,#80462,#80463,#80464,#80465,#80466,#80467,
#80468,#80469,#80470,#80471,#80472,#80473,#80474,#80475,#80476,#80477,#80478,
#80479,#80480,#80481,#80482,#80483,#80484,#80485,#80486,#80487,#80488,#80489,
#80490,#80491,#80492,#80493,#80494,#80495,#80496,#80497,#80498,#80499,#80500,
#80501,#80502,#80503,#80504,#80505,#80506,#80507,#80508,#80509,#80510,#80511,
#80512,#80513,#80514,#80515,#80516,#80517,#80518,#80519,#80520,#80521,#80522,
#80523,#80524,#80525,#80526,#80527,#80528,#80529,#80530,#80531),
 .UNSPECIFIED.,.F.,.F.,(4,3,3,3,3,3,3,3,3,3,3,3,3,3,3,3,3,3,3,3,3,3,3,3,
3,3,3,3,3,3,3,3,3,3,3,3,3,3,3,3,3,3,3,3,3,3,3,3,3,3,3,3,3,3,3,3,3,3,3,3,
3,3,3,3,3,3,3,3,3,3,3,3,3,3,4),(57.6587131819983,57.7635561766369,57.8696480169293,
57.9718780345523,58.0604324359903,58.1488721237196,58.2372208989125,58.3289924331833,
58.4172389677552,58.5054720859708,58.5937131540089,58.681983538637,58.7703542694889,
58.8587845207756,58.9473449908714,58.971393173079,59.059947574517,59.1483872622463,
59.2367360374391,59.3285075717099,59.4167541062818,59.5049872244974,59.5932282925357,
59.6814986771637,59.7698694080157,59.8582996593024,59.9468601293982,59.9709083116058,
60.0594627130438,60.1479024007732,60.236251175966,60.3280227102368,60.4162692448087,
60.5045023630244,60.5927434310627,60.6810138156907,60.7693845465427,60.8578147978294,
60.9463752679252,60.9704234501326,61.0589778515706,61.1474175392999,61.2357663144927,
61.3275378487635,61.4157843833353,61.5040175015509,61.5922585695892,61.6805289542171,
61.7688996850691,61.8573299363557,61.9458904064515,61.9699385886593,62.0584929900973,
62.1469326778267,62.2352814530195,62.3270529872903,62.4152995218621,62.5035326400778,
62.5917737081161,62.6800440927442,62.7684148235962,62.8568450748829,62.9454055449787,
62.9694537271861,63.0576099768535,63.1456517950404,63.2336034379488,63.3221402935183,
63.409993392867,63.4978342680855,63.5856846894268,63.6747380876961,63.7627199693434,
63.8523091259238,63.9418982825042),.UNSPECIFIED.);
#7850=B_SPLINE_CURVE_WITH_KNOTS('',3,(#80533,#80534,#80535,#80536,#80537,
#80538,#80539,#80540,#80541,#80542,#80543,#80544,#80545,#80546,#80547,#80548,
#80549,#80550,#80551,#80552,#80553,#80554,#80555,#80556,#80557,#80558,#80559,
#80560,#80561,#80562,#80563,#80564,#80565,#80566,#80567,#80568,#80569,#80570,
#80571,#80572,#80573,#80574,#80575,#80576,#80577,#80578,#80579,#80580,#80581,
#80582,#80583,#80584,#80585,#80586,#80587,#80588,#80589,#80590,#80591,#80592,
#80593,#80594,#80595,#80596,#80597,#80598,#80599,#80600,#80601,#80602,#80603,
#80604,#80605,#80606,#80607,#80608,#80609,#80610,#80611,#80612,#80613,#80614,
#80615,#80616,#80617,#80618,#80619,#80620,#80621,#80622,#80623,#80624,#80625,
#80626,#80627,#80628,#80629,#80630,#80631,#80632,#80633,#80634,#80635,#80636,
#80637,#80638,#80639,#80640,#80641,#80642,#80643,#80644,#80645,#80646,#80647,
#80648,#80649,#80650,#80651,#80652,#80653,#80654,#80655,#80656,#80657,#80658,
#80659,#80660,#80661,#80662,#80663,#80664,#80665,#80666,#80667,#80668,#80669,
#80670,#80671,#80672,#80673,#80674,#80675,#80676,#80677,#80678,#80679,#80680,
#80681,#80682,#80683,#80684,#80685,#80686,#80687,#80688,#80689,#80690,#80691,
#80692,#80693,#80694,#80695,#80696,#80697,#80698,#80699,#80700,#80701,#80702,
#80703,#80704,#80705,#80706,#80707,#80708,#80709,#80710,#80711,#80712,#80713,
#80714,#80715,#80716,#80717,#80718,#80719,#80720,#80721,#80722,#80723,#80724,
#80725,#80726,#80727,#80728,#80729,#80730,#80731,#80732,#80733,#80734,#80735,
#80736,#80737,#80738,#80739,#80740,#80741,#80742,#80743,#80744,#80745,#80746,
#80747,#80748,#80749,#80750,#80751,#80752,#80753,#80754,#80755,#80756,#80757,
#80758,#80759,#80760,#80761),.UNSPECIFIED.,.F.,.F.,(4,3,3,3,3,3,3,3,3,3,
3,3,3,3,3,3,3,3,3,3,3,3,3,3,3,3,3,3,3,3,3,3,3,3,3,3,3,3,3,3,3,3,3,3,3,3,
3,3,3,3,3,3,3,3,3,3,3,3,3,3,3,3,3,3,3,3,3,3,3,3,3,3,3,3,3,3,4),(63.9418982827076,
63.9689688657128,64.0575232671507,64.1459629548799,64.2343117300728,64.3260832643437,
64.4143297989155,64.5025629171311,64.5908039851692,64.6790743697972,64.7674451006491,
64.8558753519356,64.9444358220313,64.9684840042396,65.0570384056776,65.1454780934069,
65.2338268685997,65.3255984028705,65.4138449374424,65.502078055658,65.5903191236962,
65.6785895083243,65.7669602391763,65.8553904904629,65.9439509605588,65.9679991427663,
66.0565535442043,66.1449932319336,66.2333420071265,66.3251135413973,66.4133600759691,
66.5015931941848,66.5898342622231,66.6781046468511,66.766475377703,66.8549056289897,
66.9434660990856,66.9675142812931,67.0560686827311,67.1445083704604,67.2328571456533,
67.3246286799241,67.412875214496,67.5011083327116,67.5893494007499,67.6776197853779,
67.7659905162299,67.8544207675166,67.9429812376125,67.9670294198199,68.0555838212579,
68.1440235089871,68.2323722841799,68.3241438184508,68.4123903530226,68.5006234712382,
68.5888645392764,68.6771349239043,68.7655056547563,68.8539359060429,68.9424963761388,
68.9665445583466,69.0550989597846,69.143538647514,69.2318874227069,69.3236589569777,
69.4119054915496,69.5001386097652,69.5883796778035,69.6766500624318,69.7650207932838,
69.8534510445703,69.9420115146663,69.9660596968734,70.0804033841329,70.1924681488945,
70.2250835097423),.UNSPECIFIED.);
#7851=B_SPLINE_CURVE_WITH_KNOTS('',3,(#80763,#80764,#80765,#80766,#80767,
#80768,#80769,#80770,#80771,#80772),.UNSPECIFIED.,.F.,.F.,(4,1,1,1,1,1,
1,4),(70.2250835898872,70.9655748354001,71.9650899739269,72.9646051124537,
73.9641202509804,74.9636353895072,75.9631505280339,76.5082688970668),
 .UNSPECIFIED.);
#7852=B_SPLINE_CURVE_WITH_KNOTS('',3,(#80774,#80775,#80776,#80777,#80778,
#80779,#80780,#80781,#80782,#80783,#80784,#80785,#80786,#80787,#80788,#80789,
#80790,#80791,#80792,#80793,#80794,#80795,#80796,#80797,#80798,#80799,#80800,
#80801,#80802,#80803,#80804,#80805,#80806,#80807,#80808,#80809,#80810,#80811,
#80812,#80813,#80814,#80815,#80816,#80817,#80818,#80819,#80820,#80821,#80822,
#80823,#80824,#80825,#80826,#80827,#80828,#80829,#80830,#80831,#80832,#80833,
#80834,#80835,#80836,#80837,#80838,#80839,#80840,#80841,#80842,#80843,#80844,
#80845,#80846,#80847,#80848,#80849,#80850,#80851,#80852,#80853,#80854,#80855,
#80856,#80857,#80858,#80859,#80860,#80861,#80862,#80863,#80864,#80865,#80866,
#80867,#80868,#80869,#80870,#80871,#80872,#80873,#80874,#80875,#80876,#80877,
#80878,#80879,#80880,#80881,#80882,#80883,#80884,#80885,#80886,#80887,#80888,
#80889,#80890,#80891,#80892,#80893,#80894,#80895,#80896,#80897,#80898,#80899,
#80900,#80901,#80902,#80903,#80904,#80905,#80906,#80907,#80908,#80909,#80910,
#80911,#80912,#80913,#80914,#80915,#80916,#80917,#80918,#80919,#80920,#80921,
#80922,#80923,#80924,#80925,#80926,#80927,#80928,#80929,#80930,#80931,#80932,
#80933,#80934,#80935,#80936,#80937,#80938,#80939,#80940,#80941,#80942,#80943,
#80944,#80945,#80946,#80947,#80948,#80949,#80950,#80951,#80952,#80953,#80954,
#80955,#80956,#80957,#80958,#80959,#80960,#80961,#80962,#80963,#80964,#80965,
#80966,#80967,#80968,#80969,#80970,#80971,#80972,#80973,#80974,#80975,#80976,
#80977,#80978,#80979,#80980,#80981,#80982,#80983,#80984,#80985,#80986,#80987,
#80988,#80989,#80990,#80991,#80992,#80993,#80994,#80995,#80996,#80997,#80998,
#80999),.UNSPECIFIED.,.F.,.F.,(4,3,3,3,3,3,3,3,3,3,3,3,3,3,3,3,3,3,3,3,
3,3,3,3,3,3,3,3,3,3,3,3,3,3,3,3,3,3,3,3,3,3,3,3,3,3,3,3,3,3,3,3,3,3,3,3,
3,3,3,3,3,3,3,3,3,3,3,3,3,3,3,3,3,3,3,4),(76.5082691399735,76.6026454255836,
76.697363068653,76.7922538820692,76.8874364963458,76.9626656665607,77.0512200679987,
77.1396597557281,77.2280085309208,77.3197800651916,77.4080265997635,77.4962597179792,
77.5845007860174,77.6727711706453,77.7611419014973,77.8495721527841,77.9381326228799,
77.9621808050875,78.0507352065255,78.1391748942548,78.2275236694476,78.3192952037184,
78.4075417382902,78.4957748565058,78.584015924544,78.672286309172,78.760657040024,
78.8490872913106,78.9376477614065,78.9616959436142,79.0502503450522,79.1386900327815,
79.2270388079743,79.3188103422452,79.407056876817,79.4952899950327,79.5835310630709,
79.6718014476989,79.7601721785509,79.8486024298375,79.9371628999333,79.961211082141,
80.049765483579,80.1382051713083,80.2265539465012,80.318325480772,80.4065720153439,
80.4948051335595,80.5830462015978,80.6713165862258,80.7596873170778,80.8481175683645,
80.9366780384603,80.9607262206678,81.0492806221058,81.1377203098352,81.2260690850281,
81.3178406192989,81.4060871538708,81.4943202720864,81.5825613401247,81.6708317247528,
81.7592024556047,81.8476327068913,81.9361931769871,81.9602413591946,82.0474735219598,
82.1345915975361,82.2216101893339,82.3085738643474,82.3955051745341,82.482426637279,
82.5693987263293,82.6563983044652,82.7434972344772,82.7914542042464),
 .UNSPECIFIED.);
#7853=B_SPLINE_CURVE_WITH_KNOTS('',3,(#81001,#81002,#81003,#81004,#81005,
#81006,#81007,#81008,#81009,#81010,#81011),.UNSPECIFIED.,.F.,.F.,(4,1,1,
1,1,1,1,1,4),(82.7914542042464,82.9597564977213,83.9592716362481,84.9587867747749,
85.9583019133016,86.9578170518284,87.9573321903551,88.9568473288819,89.074639511426),
 .UNSPECIFIED.);
#7854=B_SPLINE_CURVE_WITH_KNOTS('',3,(#81013,#81014,#81015,#81016,#81017,
#81018,#81019,#81020,#81021,#81022,#81023,#81024,#81025,#81026,#81027,#81028,
#81029,#81030,#81031,#81032,#81033,#81034,#81035,#81036,#81037,#81038,#81039,
#81040,#81041,#81042,#81043,#81044,#81045,#81046,#81047,#81048,#81049,#81050,
#81051,#81052,#81053,#81054,#81055,#81056,#81057,#81058,#81059,#81060,#81061,
#81062,#81063,#81064,#81065,#81066,#81067,#81068,#81069,#81070,#81071,#81072,
#81073,#81074,#81075,#81076,#81077,#81078,#81079,#81080,#81081,#81082,#81083,
#81084,#81085,#81086,#81087,#81088,#81089,#81090,#81091,#81092,#81093,#81094,
#81095,#81096,#81097,#81098,#81099,#81100,#81101,#81102,#81103,#81104,#81105,
#81106,#81107,#81108,#81109,#81110,#81111,#81112,#81113,#81114,#81115,#81116,
#81117,#81118,#81119,#81120,#81121,#81122,#81123,#81124,#81125,#81126,#81127,
#81128,#81129,#81130,#81131,#81132,#81133,#81134,#81135,#81136,#81137,#81138,
#81139,#81140,#81141,#81142,#81143,#81144,#81145,#81146,#81147,#81148,#81149,
#81150,#81151,#81152,#81153,#81154,#81155,#81156,#81157,#81158,#81159,#81160,
#81161,#81162,#81163,#81164,#81165,#81166,#81167,#81168,#81169,#81170,#81171,
#81172,#81173,#81174,#81175,#81176,#81177,#81178,#81179,#81180,#81181,#81182,
#81183,#81184,#81185,#81186,#81187,#81188,#81189,#81190,#81191,#81192,#81193,
#81194,#81195,#81196,#81197,#81198,#81199,#81200,#81201,#81202,#81203,#81204,
#81205,#81206,#81207,#81208,#81209,#81210,#81211,#81212,#81213,#81214,#81215,
#81216,#81217,#81218,#81219,#81220,#81221,#81222,#81223,#81224,#81225,#81226,
#81227,#81228,#81229,#81230,#81231,#81232,#81233,#81234,#81235,#81236,#81237,
#81238),.UNSPECIFIED.,.F.,.F.,(4,3,3,3,3,3,3,3,3,3,3,3,3,3,3,3,3,3,3,3,
3,3,3,3,3,3,3,3,3,3,3,3,3,3,3,3,3,3,3,3,3,3,3,3,3,3,3,3,3,3,3,3,3,3,3,3,
3,3,3,3,3,3,3,3,3,3,3,3,3,3,3,3,3,3,3,4),(89.074639511426,89.1619192926847,
89.2491000317712,89.3375078362259,89.4245720601888,89.5116182563224,89.5986688526275,
89.6880922563228,89.7752668003224,89.8658146338655,89.9563624674086,90.0449168688466,
90.133356556576,90.2217053317688,90.3134768660396,90.4017234006115,90.4899565188271,
90.5781975868654,90.6664679714935,90.7548387023455,90.8432689536321,90.9318294237279,
90.9558776059354,91.0444320073733,91.1328716951027,91.2212204702956,91.3129920045664,
91.4012385391384,91.489471657354,91.5777127253922,91.6659831100203,91.7543538408723,
91.842784092159,91.9313445622549,91.9553927444622,92.0439471459002,92.1323868336295,
92.2207356088222,92.312507143093,92.4007536776648,92.4889867958805,92.5772278639185,
92.6654982485467,92.7538689793986,92.8422992306851,92.9308597007809,92.9549078829889,
93.0434622844269,93.1319019721563,93.2202507473492,93.31202228162,93.4002688161919,
93.4885019344076,93.5767430024456,93.6650133870734,93.7533841179253,93.8418143692118,
93.9303748393076,93.9544230215157,94.0429774229538,94.1314171106833,94.2197658858762,
94.311537420147,94.3997839547188,94.4880170729345,94.5762581409729,94.6645285256012,
94.7528992564532,94.8413295077404,94.9298899778364,94.9539381600425,95.0549097698975,
95.1527638742767,95.2552942368696,95.3524272501556,95.3578245994625),
 .UNSPECIFIED.);
#7855=B_SPLINE_CURVE_WITH_KNOTS('',3,(#81240,#81241,#81242,#81243,#81244,
#81245,#81246,#81247,#81248,#81249),.UNSPECIFIED.,.F.,.F.,(4,1,1,1,1,1,
1,4),(95.3578248186056,95.9534532985692,96.952968437096,97.9524835756227,
98.9519987141495,99.9515138526763,100.951028991203,101.641010125785),
 .UNSPECIFIED.);
#7856=B_SPLINE_CURVE_WITH_KNOTS('',3,(#81251,#81252,#81253,#81254,#81255,
#81256,#81257,#81258,#81259,#81260,#81261,#81262,#81263,#81264,#81265,#81266,
#81267,#81268,#81269,#81270,#81271,#81272,#81273,#81274,#81275,#81276,#81277,
#81278,#81279,#81280,#81281,#81282,#81283,#81284,#81285,#81286,#81287,#81288,
#81289,#81290,#81291,#81292,#81293,#81294,#81295,#81296,#81297,#81298,#81299,
#81300,#81301,#81302,#81303,#81304,#81305,#81306,#81307,#81308,#81309,#81310,
#81311,#81312,#81313,#81314,#81315,#81316,#81317,#81318,#81319,#81320,#81321,
#81322,#81323,#81324,#81325,#81326,#81327,#81328,#81329,#81330,#81331,#81332,
#81333,#81334,#81335,#81336,#81337,#81338,#81339,#81340,#81341,#81342,#81343,
#81344,#81345,#81346,#81347,#81348,#81349,#81350,#81351,#81352,#81353,#81354,
#81355,#81356,#81357,#81358,#81359,#81360,#81361,#81362,#81363,#81364,#81365,
#81366,#81367,#81368,#81369,#81370,#81371,#81372,#81373,#81374,#81375,#81376,
#81377,#81378,#81379,#81380,#81381,#81382,#81383,#81384,#81385,#81386,#81387,
#81388,#81389,#81390,#81391,#81392,#81393,#81394,#81395,#81396,#81397,#81398,
#81399,#81400,#81401,#81402,#81403,#81404,#81405,#81406,#81407,#81408,#81409,
#81410,#81411,#81412,#81413,#81414,#81415,#81416,#81417,#81418,#81419,#81420,
#81421,#81422,#81423,#81424,#81425,#81426,#81427,#81428,#81429,#81430,#81431,
#81432,#81433,#81434,#81435,#81436,#81437,#81438,#81439,#81440,#81441,#81442,
#81443,#81444,#81445,#81446,#81447,#81448,#81449,#81450,#81451,#81452,#81453,
#81454,#81455,#81456,#81457,#81458,#81459,#81460,#81461,#81462,#81463,#81464,
#81465,#81466,#81467,#81468,#81469,#81470,#81471,#81472,#81473),
 .UNSPECIFIED.,.F.,.F.,(4,3,3,3,3,3,3,3,3,3,3,3,3,3,3,3,3,3,3,3,3,3,3,3,
3,3,3,3,3,3,3,3,3,3,3,3,3,3,3,3,3,3,3,3,3,3,3,3,3,3,3,3,3,3,3,3,3,3,3,3,
3,3,3,3,3,3,3,3,3,3,3,3,3,3,4),(101.641010326215,101.746247243759,101.852779011131,
101.95054412973,102.039098531168,102.127538218897,102.21588699409,102.307658528361,
102.395905062932,102.484138181148,102.572379249186,102.660649633814,102.749020364665,
102.837450615952,102.926011086048,102.950059268257,103.038613669695,103.127053357424,
103.215402132616,103.307173666887,103.395420201459,103.483653319674,103.571894387712,
103.66016477234,103.748535503192,103.836965754478,103.925526224574,103.949574406783,
104.038128808221,104.12656849595,104.214917271143,104.306688805414,104.394935339986,
104.483168458202,104.57140952624,104.659679910868,104.74805064172,104.836480893007,
104.925041363102,104.94908954531,105.037643946748,105.126083634478,105.21443240967,
105.306203943941,105.394450478513,105.482683596729,105.570924664767,105.659195049395,
105.747565780248,105.835996031534,105.92455650163,105.948604683837,106.037159085275,
106.125598773004,106.213947548197,106.305719082468,106.39396561704,106.482198735256,
106.570439803294,106.658710187922,106.747080918774,106.83551117006,106.924071640156,
106.948119822364,107.036325090243,107.124415885493,107.212416411561,107.301388789214,
107.389290338596,107.477179538862,107.565078113673,107.654857443451,107.742887885958,
107.833541659372,107.924195432786),.UNSPECIFIED.);
#7857=B_SPLINE_CURVE_WITH_KNOTS('',3,(#81475,#81476,#81477,#81478,#81479,
#81480,#81481,#81482,#81483,#81484,#81485,#81486,#81487,#81488,#81489,#81490,
#81491,#81492,#81493,#81494,#81495,#81496,#81497,#81498,#81499,#81500,#81501,
#81502,#81503,#81504,#81505,#81506,#81507,#81508,#81509,#81510,#81511,#81512,
#81513,#81514,#81515,#81516,#81517,#81518,#81519,#81520,#81521,#81522,#81523,
#81524,#81525,#81526,#81527,#81528,#81529,#81530,#81531,#81532,#81533,#81534,
#81535,#81536,#81537,#81538,#81539,#81540,#81541,#81542,#81543,#81544,#81545,
#81546,#81547,#81548,#81549,#81550,#81551,#81552,#81553,#81554,#81555,#81556,
#81557,#81558,#81559,#81560,#81561,#81562,#81563,#81564,#81565,#81566,#81567,
#81568,#81569,#81570,#81571,#81572,#81573,#81574,#81575,#81576,#81577,#81578,
#81579,#81580,#81581,#81582,#81583,#81584,#81585,#81586,#81587,#81588,#81589,
#81590,#81591,#81592,#81593,#81594,#81595,#81596,#81597,#81598,#81599,#81600,
#81601,#81602,#81603,#81604,#81605,#81606,#81607,#81608,#81609,#81610,#81611,
#81612,#81613,#81614,#81615,#81616,#81617,#81618,#81619,#81620,#81621,#81622,
#81623,#81624,#81625,#81626,#81627,#81628,#81629,#81630,#81631,#81632,#81633,
#81634,#81635,#81636,#81637,#81638,#81639,#81640,#81641,#81642,#81643,#81644,
#81645,#81646,#81647,#81648,#81649,#81650,#81651,#81652,#81653,#81654,#81655,
#81656,#81657,#81658,#81659,#81660,#81661,#81662,#81663,#81664,#81665,#81666,
#81667,#81668,#81669,#81670,#81671,#81672,#81673,#81674,#81675,#81676,#81677,
#81678,#81679,#81680,#81681,#81682,#81683,#81684,#81685,#81686,#81687,#81688,
#81689,#81690,#81691,#81692,#81693,#81694,#81695,#81696,#81697,#81698,#81699,
#81700,#81701,#81702,#81703),.UNSPECIFIED.,.F.,.F.,(4,3,3,3,3,3,3,3,3,3,
3,3,3,3,3,3,3,3,3,3,3,3,3,3,3,3,3,3,3,3,3,3,3,3,3,3,3,3,3,3,3,3,3,3,3,3,
3,3,3,3,3,3,3,3,3,3,3,3,3,3,3,3,3,3,3,3,3,3,3,3,3,3,3,3,3,3,4),(107.924195432965,
107.94763496089,108.036189362328,108.124629050057,108.21297782525,108.304749359521,
108.392995894093,108.481229012309,108.569470080347,108.657740464975,108.746111195827,
108.834541447114,108.92310191721,108.947150099417,109.035704500855,109.124144188584,
109.212492963777,109.304264498048,109.39251103262,109.480744150836,109.568985218874,
109.657255603502,109.745626334354,109.834056585641,109.922617055736,109.946665237944,
110.035219639382,110.123659327112,110.212008102304,110.303779636575,110.392026171147,
110.480259289363,110.568500357401,110.65677074203,110.745141472882,110.833571724168,
110.922132194264,110.946180376471,111.034734777909,111.123174465638,111.21152324083,
111.303294775101,111.391541309673,111.479774427888,111.568015495926,111.656285880554,
111.744656611406,111.833086862692,111.921647332788,111.945695514997,112.034249916435,
112.122689604164,112.211038379357,112.302809913628,112.3910564482,112.479289566415,
112.567530634454,112.655801019082,112.744171749934,112.83260200122,112.921162471316,
112.945210653524,113.033765054962,113.122204742692,113.210553517885,113.302325052156,
113.390571586728,113.478804704944,113.567045772982,113.65531615761,113.743686888462,
113.832117139749,113.920677609846,113.944725792051,114.058407016934,114.16992096901,
114.207380649555),.UNSPECIFIED.);
#7858=B_SPLINE_CURVE_WITH_KNOTS('',3,(#81705,#81706,#81707,#81708,#81709,
#81710,#81711,#81712,#81713,#81714),.UNSPECIFIED.,.F.,.F.,(4,1,1,1,1,1,
1,4),(114.207380740144,114.944240930578,115.943756069104,116.943271207631,
117.942786346158,118.942301484685,119.941816623212,120.490566047324),
 .UNSPECIFIED.);
#7859=B_SPLINE_CURVE_WITH_KNOTS('',3,(#81716,#81717,#81718,#81719,#81720,
#81721,#81722,#81723,#81724,#81725,#81726,#81727,#81728,#81729,#81730,#81731,
#81732,#81733,#81734,#81735,#81736,#81737,#81738,#81739,#81740,#81741,#81742,
#81743,#81744,#81745,#81746,#81747,#81748,#81749,#81750,#81751,#81752,#81753,
#81754,#81755,#81756,#81757,#81758,#81759,#81760,#81761,#81762,#81763,#81764,
#81765,#81766,#81767,#81768,#81769,#81770,#81771,#81772,#81773,#81774,#81775,
#81776,#81777,#81778,#81779,#81780,#81781,#81782,#81783,#81784,#81785,#81786,
#81787,#81788,#81789,#81790,#81791,#81792,#81793,#81794,#81795,#81796,#81797,
#81798,#81799,#81800,#81801,#81802,#81803,#81804,#81805,#81806,#81807,#81808,
#81809,#81810,#81811,#81812,#81813,#81814,#81815,#81816,#81817,#81818,#81819,
#81820,#81821,#81822,#81823,#81824,#81825,#81826,#81827,#81828,#81829,#81830,
#81831,#81832,#81833,#81834,#81835,#81836,#81837,#81838,#81839,#81840,#81841,
#81842,#81843,#81844,#81845,#81846,#81847,#81848,#81849,#81850,#81851,#81852,
#81853,#81854,#81855,#81856,#81857,#81858,#81859,#81860,#81861,#81862,#81863,
#81864,#81865,#81866,#81867,#81868,#81869,#81870,#81871,#81872,#81873,#81874,
#81875,#81876,#81877,#81878,#81879,#81880,#81881,#81882,#81883,#81884,#81885,
#81886,#81887,#81888,#81889,#81890,#81891,#81892,#81893,#81894,#81895,#81896,
#81897,#81898,#81899,#81900,#81901,#81902,#81903,#81904,#81905,#81906,#81907,
#81908,#81909,#81910,#81911,#81912,#81913,#81914,#81915,#81916,#81917,#81918,
#81919,#81920,#81921,#81922,#81923,#81924,#81925,#81926,#81927,#81928,#81929,
#81930,#81931,#81932,#81933,#81934,#81935,#81936,#81937,#81938,#81939,#81940,
#81941),.UNSPECIFIED.,.F.,.F.,(4,3,3,3,3,3,3,3,3,3,3,3,3,3,3,3,3,3,3,3,
3,3,3,3,3,3,3,3,3,3,3,3,3,3,3,3,3,3,3,3,3,3,3,3,3,3,3,3,3,3,3,3,3,3,3,3,
3,3,3,3,3,3,3,3,3,3,3,3,3,3,3,3,3,3,3,4),(120.490566307756,120.585118114269,
120.680021397524,120.775103661094,120.870480885623,120.941331761738,121.029886163176,
121.118325850906,121.206674626099,121.29844616037,121.386692694942,121.474925813157,
121.563166881196,121.651437265824,121.739807996676,121.828238247963,121.916798718059,
121.940846900265,122.029401301703,122.117840989432,122.206189764625,122.297961298896,
122.386207833468,122.474440951684,122.562682019722,122.65095240435,122.739323135202,
122.827753386489,122.916313856585,122.940362038792,123.02891644023,123.117356127959,
123.205704903152,123.297476437423,123.385722971995,123.473956090211,123.562197158249,
123.650467542877,123.738838273729,123.827268525016,123.915828995112,123.939877177319,
124.028431578757,124.116871266486,124.205220041679,124.296991575949,124.385238110521,
124.473471228737,124.561712296775,124.649982681402,124.738353412254,124.826783663541,
124.915344133636,124.939392315845,125.027946717283,125.116386405012,125.204735180205,
125.296506714476,125.384753249047,125.472986367263,125.561227435301,125.649497819929,
125.737868550781,125.826298802068,125.914859272163,125.938907454372,126.026140185572,
126.11325888379,126.20027827459,126.287242825609,126.374175088105,126.461097578889,
126.548071560608,126.63507305944,126.722175935449,126.773751354504),
 .UNSPECIFIED.);
#7860=B_SPLINE_CURVE_WITH_KNOTS('',3,(#81943,#81944,#81945,#81946,#81947,
#81948,#81949,#81950,#81951,#81952,#81953),.UNSPECIFIED.,.F.,.F.,(4,1,1,
1,1,1,1,1,4),(126.773751354504,126.938422592899,127.937937731426,128.937452869952,
129.936968008479,130.936483147006,131.935998285533,132.935513424059,133.056936661683),
 .UNSPECIFIED.);
#7861=B_SPLINE_CURVE_WITH_KNOTS('',3,(#81955,#81956,#81957,#81958,#81959,
#81960,#81961,#81962,#81963,#81964,#81965,#81966,#81967,#81968,#81969,#81970,
#81971,#81972,#81973,#81974,#81975,#81976,#81977,#81978,#81979,#81980,#81981,
#81982,#81983,#81984,#81985,#81986,#81987,#81988,#81989,#81990,#81991,#81992,
#81993,#81994,#81995,#81996,#81997,#81998,#81999,#82000,#82001,#82002,#82003,
#82004,#82005,#82006,#82007,#82008,#82009,#82010,#82011,#82012,#82013,#82014,
#82015,#82016,#82017,#82018,#82019,#82020,#82021,#82022,#82023,#82024,#82025,
#82026,#82027,#82028,#82029,#82030,#82031,#82032,#82033,#82034,#82035,#82036,
#82037,#82038,#82039,#82040,#82041,#82042,#82043,#82044,#82045,#82046,#82047,
#82048,#82049,#82050,#82051,#82052,#82053,#82054,#82055,#82056,#82057,#82058,
#82059,#82060,#82061,#82062,#82063,#82064,#82065,#82066,#82067,#82068,#82069,
#82070,#82071,#82072,#82073,#82074,#82075,#82076,#82077,#82078,#82079,#82080,
#82081,#82082,#82083,#82084,#82085,#82086,#82087,#82088,#82089,#82090,#82091,
#82092,#82093,#82094,#82095,#82096,#82097,#82098,#82099,#82100,#82101,#82102,
#82103,#82104,#82105,#82106,#82107,#82108,#82109,#82110,#82111,#82112,#82113,
#82114,#82115,#82116,#82117,#82118,#82119,#82120,#82121,#82122,#82123,#82124,
#82125,#82126,#82127,#82128,#82129,#82130,#82131,#82132,#82133,#82134,#82135,
#82136,#82137,#82138,#82139,#82140,#82141,#82142,#82143,#82144,#82145,#82146,
#82147,#82148,#82149,#82150,#82151,#82152,#82153,#82154,#82155,#82156,#82157,
#82158,#82159,#82160,#82161,#82162,#82163,#82164,#82165,#82166,#82167,#82168,
#82169,#82170,#82171,#82172,#82173,#82174,#82175,#82176,#82177,#82178,#82179,
#82180),.UNSPECIFIED.,.F.,.F.,(4,3,3,3,3,3,3,3,3,3,3,3,3,3,3,3,3,3,3,3,
3,3,3,3,3,3,3,3,3,3,3,3,3,3,3,3,3,3,3,3,3,3,3,3,3,3,3,3,3,3,3,3,3,3,3,3,
3,3,3,3,3,3,3,3,3,3,3,3,3,3,3,3,3,3,3,4),(133.056936661683,133.144196640644,
133.231358408055,133.319317177371,133.406364512018,133.493394486404,133.580429539472,
133.66907929525,133.75623885054,133.845633706563,133.935028562586,134.023582964024,
134.112022651753,134.200371426946,134.292142961217,134.380389495789,134.468622614005,
134.556863682043,134.645134066671,134.733504797523,134.821935048809,134.910495518905,
134.934543701113,135.023098102551,135.111537790281,135.199886565474,135.291658099744,
135.379904634316,135.468137752532,135.556378820571,135.644649205199,135.733019936051,
135.821450187337,135.910010657433,135.93405883964,136.022613241078,136.111052928807,
136.199401703999,136.29117323827,136.379419772842,136.467652891057,136.555893959095,
136.644164343723,136.732535074575,136.820965325861,136.909525795957,136.933573978166,
137.022128379604,137.110568067333,137.198916842526,137.290688376797,137.378934911368,
137.467168029584,137.555409097622,137.64367948225,137.732050213102,137.820480464389,
137.909040934484,137.933089116693,138.021643518131,138.110083205861,138.198431981054,
138.290203515325,138.378450049897,138.466683168112,138.554924236151,138.643194620779,
138.731565351631,138.819995602918,138.908556073014,138.93260425522,139.034483630081,
139.132097818871,139.229434282969,139.326360752829,139.340121754662),
 .UNSPECIFIED.);
#7862=B_SPLINE_CURVE_WITH_KNOTS('',3,(#82182,#82183,#82184,#82185,#82186,
#82187,#82188,#82189,#82190,#82191),.UNSPECIFIED.,.F.,.F.,(4,1,1,1,1,1,
1,4),(139.340121968863,139.932119393747,140.931634532274,141.9311496708,
142.930664809327,143.930179947854,144.929695086381,145.623307276042),
 .UNSPECIFIED.);
#7863=B_SPLINE_CURVE_WITH_KNOTS('',3,(#82193,#82194,#82195,#82196,#82197,
#82198,#82199,#82200,#82201,#82202,#82203,#82204,#82205,#82206,#82207,#82208,
#82209,#82210,#82211,#82212,#82213,#82214,#82215,#82216,#82217,#82218,#82219,
#82220,#82221,#82222,#82223,#82224,#82225,#82226,#82227,#82228,#82229,#82230,
#82231,#82232,#82233,#82234,#82235,#82236,#82237,#82238,#82239,#82240,#82241,
#82242,#82243,#82244,#82245,#82246,#82247,#82248,#82249,#82250,#82251,#82252,
#82253,#82254,#82255,#82256,#82257,#82258,#82259,#82260,#82261,#82262,#82263,
#82264,#82265,#82266,#82267,#82268,#82269,#82270,#82271,#82272,#82273,#82274,
#82275,#82276,#82277,#82278,#82279,#82280,#82281,#82282,#82283,#82284,#82285,
#82286,#82287,#82288,#82289,#82290,#82291,#82292,#82293,#82294,#82295,#82296,
#82297,#82298,#82299,#82300,#82301,#82302,#82303,#82304,#82305,#82306,#82307,
#82308,#82309,#82310,#82311,#82312,#82313,#82314,#82315,#82316,#82317,#82318,
#82319,#82320,#82321,#82322,#82323,#82324,#82325,#82326,#82327,#82328,#82329,
#82330,#82331,#82332,#82333,#82334,#82335,#82336,#82337,#82338,#82339,#82340,
#82341,#82342,#82343,#82344,#82345,#82346,#82347,#82348,#82349,#82350,#82351,
#82352,#82353,#82354,#82355,#82356,#82357,#82358,#82359,#82360,#82361,#82362,
#82363,#82364,#82365,#82366,#82367,#82368,#82369,#82370,#82371,#82372,#82373,
#82374,#82375,#82376,#82377,#82378,#82379,#82380,#82381,#82382,#82383,#82384,
#82385,#82386,#82387,#82388,#82389,#82390,#82391,#82392,#82393,#82394,#82395,
#82396,#82397,#82398,#82399,#82400,#82401,#82402,#82403,#82404,#82405,#82406,
#82407,#82408,#82409,#82410,#82411,#82412,#82413,#82414,#82415),
 .UNSPECIFIED.,.F.,.F.,(4,3,3,3,3,3,3,3,3,3,3,3,3,3,3,3,3,3,3,3,3,3,3,3,
3,3,3,3,3,3,3,3,3,3,3,3,3,3,3,3,3,3,3,3,3,3,3,3,3,3,3,3,3,3,3,3,3,3,3,3,
3,3,3,3,3,3,3,3,3,3,3,3,3,3,4),(145.623307470037,145.728947897427,145.835931712352,
145.929210224907,146.017764626345,146.106204314075,146.194553089268,146.286324623538,
146.37457115811,146.462804276326,146.551045344364,146.639315728992,146.727686459845,
146.816116711131,146.904677181227,146.928725363434,147.017279764872,147.105719452601,
147.194068227794,147.285839762065,147.374086296637,147.462319414853,147.550560482891,
147.638830867519,147.727201598371,147.815631849658,147.904192319754,147.928240501961,
148.016794903399,148.105234591128,148.193583366321,148.285354900592,148.373601435164,
148.46183455338,148.550075621418,148.638346006046,148.726716736898,148.815146988185,
148.903707458281,148.927755640488,149.016310041926,149.104749729655,149.193098504848,
149.284870039118,149.37311657369,149.461349691906,149.549590759944,149.637861144571,
149.726231875423,149.81466212671,149.903222596805,149.927270779014,150.015825180452,
150.104264868181,150.192613643374,150.284385177645,150.372631712217,150.460864830432,
150.549105898471,150.637376283099,150.72574701395,150.814177265237,150.902737735333,
150.926785917541,151.015041546976,151.103182663218,151.191233414591,151.28064081067,
151.368592133533,151.456530971977,151.5444790009,151.63498239648,151.723062649854,
151.814777616538,151.906492583222),.UNSPECIFIED.);
#7864=B_SPLINE_CURVE_WITH_KNOTS('',3,(#82417,#82418,#82419,#82420,#82421,
#82422,#82423,#82424,#82425,#82426,#82427,#82428),.UNSPECIFIED.,.F.,.F.,
(4,2,1,1,1,1,1,1,4),(151.906492583222,151.926301056068,152.925816194595,
153.925331333121,154.924846471648,155.924361610175,156.923876748702,157.923391887229,
158.189674734771),.UNSPECIFIED.);
#7865=B_SPLINE_CURVE_WITH_KNOTS('',3,(#82430,#82431,#82432,#82433,#82434,
#82435,#82436,#82437,#82438,#82439,#82440,#82441,#82442,#82443,#82444,#82445,
#82446,#82447,#82448,#82449,#82450,#82451,#82452,#82453,#82454,#82455,#82456,
#82457,#82458,#82459,#82460,#82461,#82462,#82463,#82464,#82465,#82466,#82467,
#82468,#82469,#82470,#82471,#82472,#82473,#82474,#82475,#82476,#82477,#82478,
#82479,#82480,#82481,#82482,#82483,#82484,#82485,#82486,#82487,#82488,#82489,
#82490,#82491,#82492,#82493,#82494,#82495,#82496,#82497,#82498,#82499,#82500,
#82501,#82502,#82503,#82504,#82505,#82506,#82507,#82508,#82509,#82510,#82511,
#82512,#82513,#82514,#82515,#82516,#82517,#82518,#82519,#82520,#82521,#82522,
#82523,#82524,#82525,#82526,#82527,#82528,#82529,#82530,#82531,#82532,#82533,
#82534,#82535,#82536,#82537,#82538,#82539,#82540,#82541,#82542,#82543,#82544,
#82545,#82546,#82547,#82548,#82549,#82550,#82551,#82552,#82553,#82554,#82555,
#82556,#82557,#82558,#82559,#82560,#82561,#82562,#82563,#82564,#82565,#82566,
#82567,#82568,#82569,#82570,#82571,#82572,#82573,#82574,#82575,#82576,#82577,
#82578,#82579,#82580,#82581,#82582,#82583,#82584,#82585,#82586,#82587,#82588,
#82589,#82590,#82591,#82592,#82593,#82594,#82595,#82596,#82597,#82598,#82599,
#82600,#82601,#82602,#82603,#82604,#82605,#82606,#82607,#82608,#82609,#82610,
#82611,#82612,#82613,#82614,#82615,#82616,#82617,#82618,#82619,#82620,#82621,
#82622,#82623,#82624,#82625,#82626,#82627,#82628,#82629,#82630,#82631,#82632,
#82633,#82634,#82635,#82636,#82637,#82638,#82639,#82640,#82641,#82642,#82643,
#82644,#82645,#82646,#82647,#82648,#82649,#82650,#82651,#82652,#82653,#82654,
#82655),.UNSPECIFIED.,.F.,.F.,(4,3,3,3,3,3,3,3,3,3,3,3,3,3,3,3,3,3,3,3,
3,3,3,3,3,3,3,3,3,3,3,3,3,3,3,3,3,3,3,3,3,3,3,3,3,3,3,3,3,3,3,3,3,3,3,3,
3,3,3,3,3,3,3,3,3,3,3,3,3,3,3,3,3,3,3,4),(158.189677890401,158.28133153232,
158.368710202749,158.456068790346,158.543429479056,158.630814450445,158.718295863631,
158.8058337789,158.893502610368,158.922907025755,159.011461427193,159.099901114922,
159.188249890115,159.280021424386,159.368267958958,159.456501077174,159.544742145212,
159.63301252984,159.721383260692,159.809813511979,159.898373982075,159.922422164282,
160.01097656572,160.09941625345,160.187765028642,160.279536562913,160.367783097485,
160.456016215701,160.544257283739,160.632527668367,160.720898399219,160.809328650506,
160.897889120601,160.921937302809,161.010491704247,161.098931391976,161.187280167169,
161.27905170144,161.367298236012,161.455531354228,161.543772422266,161.632042806894,
161.720413537746,161.808843789033,161.897404259129,161.921452441336,162.010006842774,
162.098446530503,162.186795305695,162.278566839966,162.366813374538,162.455046492753,
162.543287560791,162.631557945419,162.719928676271,162.808358927557,162.896919397653,
162.920967579862,163.0095219813,163.097961669029,163.186310444222,163.278081978493,
163.366328513065,163.45456163128,163.542802699318,163.631073083946,163.719443814798,
163.807874066084,163.89643453618,163.920482718389,164.01167483213,164.102725861115,
164.195260195231,164.286049488575,164.379456343078,164.472863197581),
 .UNSPECIFIED.);
#7866=B_SPLINE_CURVE_WITH_KNOTS('',3,(#82657,#82658,#82659,#82660,#82661,
#82662,#82663,#82664,#82665,#82666),.UNSPECIFIED.,.F.,.F.,(4,1,1,1,1,1,
1,4),(164.472867375453,164.919997856916,165.919512995443,166.919028133969,
167.918543272496,168.918058411023,169.91757354955,170.756048504761),
 .UNSPECIFIED.);
#7867=B_SPLINE_CURVE_WITH_KNOTS('',3,(#82668,#82669,#82670,#82671,#82672,
#82673,#82674,#82675,#82676,#82677,#82678),.UNSPECIFIED.,.F.,.F.,(4,1,1,
1,1,1,1,1,4),(170.756048504761,170.917088688076,171.916603826603,172.91611896513,
173.915634103657,174.915149242183,175.91466438071,176.914179519237,177.03923381194),
 .UNSPECIFIED.);
#7868=B_SPLINE_CURVE_WITH_KNOTS('',3,(#82680,#82681,#82682,#82683,#82684,
#82685,#82686,#82687,#82688,#82689,#82690,#82691,#82692,#82693,#82694,#82695,
#82696,#82697,#82698,#82699,#82700,#82701,#82702,#82703,#82704,#82705,#82706,
#82707,#82708,#82709,#82710,#82711,#82712,#82713,#82714,#82715,#82716,#82717,
#82718,#82719,#82720,#82721,#82722,#82723,#82724,#82725,#82726,#82727,#82728,
#82729,#82730,#82731,#82732,#82733,#82734,#82735,#82736,#82737,#82738,#82739,
#82740,#82741,#82742,#82743,#82744,#82745,#82746,#82747,#82748,#82749,#82750,
#82751,#82752,#82753,#82754,#82755,#82756,#82757,#82758,#82759,#82760,#82761,
#82762,#82763,#82764,#82765,#82766,#82767,#82768,#82769,#82770,#82771,#82772,
#82773,#82774,#82775,#82776,#82777,#82778,#82779,#82780,#82781,#82782,#82783,
#82784,#82785,#82786,#82787,#82788,#82789,#82790,#82791,#82792,#82793,#82794,
#82795,#82796,#82797,#82798,#82799,#82800,#82801,#82802,#82803,#82804,#82805,
#82806,#82807,#82808,#82809,#82810,#82811,#82812,#82813,#82814,#82815,#82816,
#82817,#82818,#82819,#82820,#82821,#82822,#82823,#82824,#82825,#82826,#82827,
#82828,#82829,#82830,#82831,#82832,#82833,#82834,#82835,#82836,#82837,#82838,
#82839,#82840,#82841,#82842,#82843,#82844,#82845,#82846,#82847,#82848,#82849,
#82850,#82851,#82852,#82853,#82854,#82855,#82856,#82857,#82858,#82859,#82860,
#82861,#82862,#82863,#82864,#82865,#82866,#82867,#82868,#82869,#82870,#82871,
#82872,#82873,#82874,#82875,#82876,#82877,#82878,#82879,#82880,#82881,#82882,
#82883,#82884,#82885,#82886,#82887,#82888,#82889,#82890,#82891,#82892,#82893,
#82894,#82895,#82896,#82897,#82898,#82899,#82900,#82901,#82902,#82903,#82904,
#82905),.UNSPECIFIED.,.F.,.F.,(4,3,3,3,3,3,3,3,3,3,3,3,3,3,3,3,3,3,3,3,
3,3,3,3,3,3,3,3,3,3,3,3,3,3,3,3,3,3,3,3,3,3,3,3,3,3,3,3,3,3,3,3,3,3,3,3,
3,3,3,3,3,3,3,3,3,3,3,3,3,3,3,3,3,3,3,4),(177.03923381194,177.126475142022,
177.213619107611,177.30112855138,177.388160191197,177.475175149924,177.562195876577,
177.650070571874,177.737216360473,177.825455509119,177.913694657764,178.002249059202,
178.090688746931,178.179037522124,178.270809056395,178.359055590967,178.447288709183,
178.535529777221,178.623800161849,178.712170892701,178.800601143988,178.889161614084,
178.913209796291,179.001764197729,179.090203885458,179.17855266065,179.270324194921,
179.358570729493,179.446803847708,179.535044915746,179.623315300374,179.711686031225,
179.800116282512,179.888676752608,179.912724934817,180.001279336255,180.089719023984,
180.178067799177,180.269839333448,180.35808586802,180.446318986235,180.534560054274,
180.622830438902,180.711201169754,180.799631421041,180.888191891136,180.912240073344,
181.000794474782,181.089234162512,181.177582937705,181.269354471975,181.357601006547,
181.445834124763,181.534075192802,181.62234557743,181.710716308282,181.799146559569,
181.887707029665,181.911755211871,182.000309613309,182.088749301038,182.177098076231,
182.268869610502,182.357116145074,182.44534926329,182.533590331328,182.621860715958,
182.71023144681,182.798661698097,182.887222168193,182.911270350398,183.014057490355,
183.111436425305,183.208546480735,183.305258922378,183.322418910228),
 .UNSPECIFIED.);
#7869=B_SPLINE_CURVE_WITH_KNOTS('',3,(#82907,#82908,#82909,#82910,#82911,
#82912,#82913,#82914,#82915,#82916),.UNSPECIFIED.,.F.,.F.,(4,1,1,1,1,1,
1,4),(183.32241911912,183.910785488924,184.910300627451,185.909815765978,
186.909330904505,187.908846043031,188.908361181558,189.605604426299),
 .UNSPECIFIED.);
#7870=B_SPLINE_CURVE_WITH_KNOTS('',3,(#82918,#82919,#82920,#82921,#82922,
#82923,#82924,#82925,#82926,#82927,#82928,#82929,#82930,#82931,#82932,#82933,
#82934,#82935,#82936,#82937,#82938,#82939,#82940,#82941,#82942,#82943,#82944,
#82945,#82946,#82947,#82948,#82949,#82950,#82951,#82952,#82953,#82954,#82955,
#82956,#82957,#82958,#82959,#82960,#82961,#82962,#82963,#82964,#82965,#82966,
#82967,#82968,#82969,#82970,#82971,#82972,#82973,#82974,#82975,#82976,#82977,
#82978,#82979,#82980,#82981,#82982,#82983,#82984,#82985,#82986,#82987,#82988,
#82989,#82990,#82991,#82992,#82993,#82994,#82995,#82996,#82997,#82998,#82999,
#83000,#83001,#83002,#83003,#83004,#83005,#83006,#83007,#83008,#83009,#83010,
#83011,#83012,#83013,#83014,#83015,#83016,#83017,#83018,#83019,#83020,#83021,
#83022,#83023,#83024,#83025,#83026,#83027,#83028,#83029,#83030,#83031,#83032,
#83033,#83034,#83035,#83036,#83037,#83038,#83039,#83040,#83041,#83042,#83043,
#83044,#83045,#83046,#83047,#83048,#83049,#83050,#83051,#83052,#83053,#83054,
#83055,#83056,#83057,#83058,#83059,#83060,#83061,#83062,#83063,#83064,#83065,
#83066,#83067,#83068,#83069,#83070,#83071,#83072,#83073,#83074,#83075,#83076,
#83077,#83078,#83079,#83080,#83081,#83082,#83083,#83084,#83085,#83086,#83087,
#83088,#83089,#83090,#83091,#83092,#83093,#83094,#83095,#83096,#83097,#83098,
#83099,#83100,#83101,#83102,#83103,#83104,#83105,#83106,#83107,#83108,#83109,
#83110,#83111,#83112,#83113,#83114,#83115,#83116,#83117,#83118,#83119,#83120,
#83121,#83122,#83123,#83124,#83125,#83126,#83127,#83128,#83129,#83130,#83131,
#83132,#83133,#83134,#83135,#83136,#83137,#83138,#83139,#83140),
 .UNSPECIFIED.,.F.,.F.,(4,3,3,3,3,3,3,3,3,3,3,3,3,3,3,3,3,3,3,3,3,3,3,3,
3,3,3,3,3,3,3,3,3,3,3,3,3,3,3,3,3,3,3,3,3,3,3,3,3,3,3,3,3,3,3,3,3,3,3,3,
3,3,3,3,3,3,3,3,3,3,3,3,3,3,4),(189.605604613475,189.711658493287,189.819107013171,
189.907876320085,189.996430721523,190.084870409252,190.173219184445,190.264990718716,
190.353237253288,190.441470371503,190.529711439541,190.617981824169,190.706352555021,
190.794782806308,190.883343276404,190.907391458612,190.99594586005,191.084385547779,
191.172734322972,191.264505857242,191.352752391814,191.440985510029,191.529226578067,
191.617496962695,191.705867693547,191.794297944834,191.882858414929,191.906906597138,
191.995460998576,192.083900686305,192.172249461498,192.264020995769,192.352267530341,
192.440500648556,192.528741716595,192.617012101223,192.705382832075,192.793813083361,
192.882373553457,192.906421735665,192.994976137103,193.083415824833,193.171764600026,
193.263536134296,193.351782668868,193.440015787084,193.528256855123,193.616527239751,
193.704897970603,193.79332822189,193.881888691986,193.905936874192,193.99449127563,
194.082930963359,194.171279738552,194.263051272823,194.351297807395,194.439530925611,
194.527771993649,194.616042378277,194.704413109129,194.792843360415,194.881403830511,
194.905452012719,194.993759355444,195.081952145223,195.170054472789,195.259896380375,
195.347898808515,195.435888606357,195.523887397765,195.615112981694,195.703244301595,
195.796017017537,195.888789733479),.UNSPECIFIED.);
#7871=B_SPLINE_CURVE_WITH_KNOTS('',3,(#83142,#83143,#83144,#83145,#83146,
#83147,#83148,#83149,#83150,#83151,#83152,#83153),.UNSPECIFIED.,.F.,.F.,
(4,2,1,1,1,1,1,1,4),(195.888789733479,195.904967151245,196.904482289772,
197.903997428299,198.903512566826,199.903027705353,200.902542843879,201.902057982406,
202.171971572916),.UNSPECIFIED.);
#7872=B_SPLINE_CURVE_WITH_KNOTS('',3,(#83155,#83156,#83157,#83158,#83159,
#83160,#83161,#83162,#83163,#83164,#83165,#83166,#83167,#83168,#83169,#83170,
#83171,#83172,#83173,#83174,#83175,#83176,#83177,#83178,#83179,#83180,#83181,
#83182,#83183,#83184,#83185,#83186,#83187,#83188,#83189,#83190,#83191,#83192,
#83193,#83194,#83195,#83196,#83197,#83198,#83199,#83200,#83201,#83202,#83203,
#83204,#83205,#83206,#83207,#83208,#83209,#83210,#83211,#83212,#83213,#83214,
#83215,#83216,#83217,#83218,#83219,#83220,#83221,#83222,#83223,#83224,#83225,
#83226,#83227,#83228,#83229,#83230,#83231,#83232,#83233,#83234,#83235,#83236,
#83237,#83238,#83239,#83240,#83241,#83242,#83243,#83244,#83245,#83246,#83247,
#83248,#83249,#83250,#83251,#83252,#83253,#83254,#83255,#83256,#83257,#83258,
#83259,#83260,#83261,#83262,#83263,#83264,#83265,#83266,#83267,#83268,#83269,
#83270,#83271,#83272,#83273,#83274,#83275,#83276,#83277,#83278,#83279,#83280,
#83281,#83282,#83283,#83284,#83285,#83286,#83287,#83288,#83289,#83290,#83291,
#83292,#83293,#83294,#83295,#83296,#83297,#83298,#83299,#83300,#83301,#83302,
#83303,#83304,#83305,#83306,#83307,#83308,#83309,#83310,#83311,#83312,#83313,
#83314,#83315,#83316,#83317,#83318,#83319,#83320,#83321,#83322,#83323,#83324,
#83325,#83326,#83327,#83328,#83329,#83330,#83331,#83332,#83333,#83334,#83335,
#83336,#83337,#83338,#83339,#83340,#83341,#83342,#83343,#83344,#83345,#83346,
#83347,#83348,#83349,#83350,#83351,#83352,#83353,#83354,#83355,#83356,#83357,
#83358,#83359,#83360,#83361,#83362,#83363,#83364,#83365,#83366,#83367,#83368,
#83369,#83370,#83371,#83372,#83373,#83374,#83375,#83376,#83377,#83378,#83379,
#83380),.UNSPECIFIED.,.F.,.F.,(4,3,3,3,3,3,3,3,3,3,3,3,3,3,3,3,3,3,3,3,
3,3,3,3,3,3,3,3,3,3,3,3,3,3,3,3,3,3,3,3,3,3,3,3,3,3,3,3,3,3,3,3,3,3,3,3,
3,3,3,3,3,3,3,3,3,3,3,3,3,3,3,3,3,3,3,4),(202.171975040658,202.263174800692,
202.350584664857,202.437975665214,202.525369957242,202.612789694942,202.700306666439,
202.78788112853,202.875585818985,202.901573120933,202.990127522371,203.078567210101,
203.166915985293,203.258687519564,203.346934054136,203.435167172352,203.52340824039,
203.611678625018,203.70004935587,203.788479607157,203.877040077253,203.90108825946,
203.989642660898,204.078082348627,204.166431123819,204.25820265809,204.346449192662,
204.434682310877,204.522923378915,204.611193763543,204.699564494395,204.787994745681,
204.876555215777,204.900603397986,204.989157799424,205.077597487154,205.165946262346,
205.257717796617,205.345964331189,205.434197449405,205.522438517443,205.61070890207,
205.699079632922,205.787509884209,205.876070354305,205.900118536513,205.988672937951,
206.077112625681,206.165461400874,206.257232935144,206.345479469716,206.433712587932,
206.521953655971,206.6102240406,206.698594771452,206.787025022738,206.875585492834,
206.89963367504,206.988188076478,207.076627764207,207.164976539401,207.256748073671,
207.344994608243,207.433227726459,207.521468794497,207.609739179125,207.698109909977,
207.786540161264,207.87510063136,207.899148813567,207.990226239938,208.081164061968,
208.174663133436,208.265343039278,208.360251693558,208.455160347838),
 .UNSPECIFIED.);
#7873=B_SPLINE_CURVE_WITH_KNOTS('',3,(#83382,#83383,#83384,#83385,#83386,
#83387,#83388,#83389,#83390,#83391),.UNSPECIFIED.,.F.,.F.,(4,1,1,1,1,1,
1,4),(208.455164776037,208.898663952093,209.89817909062,210.897694229147,
211.897209367674,212.8967245062,213.896239644727,214.738345655017),
 .UNSPECIFIED.);
#7874=B_SPLINE_CURVE_WITH_KNOTS('',3,(#83393,#83394,#83395,#83396,#83397,
#83398,#83399,#83400,#83401,#83402,#83403),.UNSPECIFIED.,.F.,.F.,(4,1,1,
1,1,1,1,1,4),(214.738345655017,214.895754783254,215.895269921781,216.894785060307,
217.894300198834,218.893815337361,219.893330475888,220.892845614415,221.021530962197),
 .UNSPECIFIED.);
#7875=B_SPLINE_CURVE_WITH_KNOTS('',3,(#83405,#83406,#83407,#83408,#83409,
#83410,#83411,#83412,#83413,#83414,#83415,#83416,#83417,#83418,#83419,#83420,
#83421,#83422,#83423,#83424,#83425,#83426,#83427,#83428,#83429,#83430,#83431,
#83432,#83433,#83434,#83435,#83436,#83437,#83438,#83439,#83440,#83441,#83442,
#83443,#83444,#83445,#83446,#83447,#83448,#83449,#83450,#83451,#83452,#83453,
#83454,#83455,#83456,#83457,#83458,#83459,#83460,#83461,#83462,#83463,#83464,
#83465,#83466,#83467,#83468,#83469,#83470,#83471,#83472,#83473,#83474,#83475,
#83476,#83477,#83478,#83479,#83480,#83481,#83482,#83483,#83484,#83485,#83486,
#83487,#83488,#83489,#83490,#83491,#83492,#83493,#83494,#83495,#83496,#83497,
#83498,#83499,#83500,#83501,#83502,#83503,#83504,#83505,#83506,#83507,#83508,
#83509,#83510,#83511,#83512,#83513,#83514,#83515,#83516,#83517,#83518,#83519,
#83520,#83521,#83522,#83523,#83524,#83525,#83526,#83527,#83528,#83529,#83530,
#83531,#83532,#83533,#83534,#83535,#83536,#83537,#83538,#83539,#83540,#83541,
#83542,#83543,#83544,#83545,#83546,#83547,#83548,#83549,#83550,#83551,#83552,
#83553,#83554,#83555,#83556,#83557,#83558,#83559,#83560,#83561,#83562,#83563,
#83564,#83565,#83566,#83567,#83568,#83569,#83570,#83571,#83572,#83573,#83574,
#83575,#83576,#83577,#83578,#83579,#83580,#83581,#83582,#83583,#83584,#83585,
#83586,#83587,#83588,#83589,#83590,#83591,#83592,#83593,#83594,#83595,#83596,
#83597,#83598,#83599,#83600,#83601,#83602,#83603,#83604,#83605,#83606,#83607,
#83608,#83609,#83610,#83611,#83612,#83613,#83614,#83615,#83616,#83617,#83618,
#83619,#83620,#83621,#83622,#83623,#83624,#83625,#83626,#83627,#83628,#83629,
#83630),.UNSPECIFIED.,.F.,.F.,(4,3,3,3,3,3,3,3,3,3,3,3,3,3,3,3,3,3,3,3,
3,3,3,3,3,3,3,3,3,3,3,3,3,3,3,3,3,3,3,3,3,3,3,3,3,3,3,3,3,3,3,3,3,3,3,3,
3,3,3,3,3,3,3,3,3,3,3,3,3,3,3,3,3,3,3,4),(221.021530962197,221.108754796741,
221.195882130097,221.282941957953,221.369959096486,221.456960244626,221.543967860593,
221.63106608368,221.718199326175,221.805477327452,221.892360752941,221.980915154314,
222.069354841978,222.157703617104,222.2494751514,222.337721685902,222.425954804048,
222.514195872016,222.602466256572,222.690836987352,222.779267238567,222.867827708591,
222.891875891468,222.980430293437,223.068869981698,223.157218757425,223.248990291496,
223.3372368266,223.425469945346,223.513711013913,223.601981399067,223.690352130439,
223.778782382243,223.867342852848,223.891391029995,223.979945430572,224.068385117442,
224.156733891777,224.24850542637,224.336751960095,224.424985077469,224.513226144672,
224.601496528473,224.689867258511,224.778297508992,224.866857978299,224.890906168522,
224.979460569799,225.067900257359,225.156249032376,225.24802056671,225.336267101086,
225.4245002191,225.512741286931,225.601011671346,225.689382401977,225.777812653038,
225.866373122903,225.890421307048,225.97897571197,226.067415403196,226.155764181893,
226.247535714853,226.335782252927,226.424015374639,226.512256446163,226.600526834263,
226.688897568548,226.77732782325,226.865888296708,226.889936445575,226.987493993785,
227.084658138073,227.181562779715,227.278077411535,227.304716066149),
 .UNSPECIFIED.);
#7876=B_SPLINE_CURVE_WITH_KNOTS('',3,(#83632,#83633,#83634,#83635,#83636,
#83637,#83638,#83639,#83640,#83641),.UNSPECIFIED.,.F.,.F.,(4,1,1,1,1,1,
1,4),(227.304716269377,227.889451584102,228.888966722629,229.888481861155,
230.887996999682,231.887512138209,232.887027276736,233.587901576556),
 .UNSPECIFIED.);
#7877=B_SPLINE_CURVE_WITH_KNOTS('',3,(#83643,#83644,#83645,#83646,#83647,
#83648,#83649,#83650,#83651,#83652,#83653,#83654,#83655,#83656,#83657,#83658,
#83659,#83660,#83661,#83662,#83663,#83664,#83665,#83666,#83667,#83668,#83669,
#83670,#83671,#83672,#83673,#83674,#83675,#83676,#83677,#83678,#83679,#83680,
#83681,#83682,#83683,#83684,#83685,#83686,#83687,#83688,#83689,#83690,#83691,
#83692,#83693,#83694,#83695,#83696,#83697,#83698,#83699,#83700,#83701,#83702,
#83703,#83704,#83705,#83706,#83707,#83708,#83709,#83710,#83711,#83712,#83713,
#83714,#83715,#83716,#83717,#83718,#83719,#83720,#83721,#83722,#83723,#83724,
#83725,#83726,#83727,#83728,#83729,#83730,#83731,#83732,#83733,#83734,#83735,
#83736,#83737,#83738,#83739,#83740,#83741,#83742,#83743,#83744,#83745,#83746,
#83747,#83748,#83749,#83750,#83751,#83752,#83753,#83754,#83755,#83756,#83757,
#83758,#83759,#83760,#83761,#83762,#83763,#83764,#83765,#83766,#83767,#83768,
#83769,#83770,#83771,#83772,#83773,#83774,#83775,#83776,#83777,#83778,#83779,
#83780,#83781,#83782,#83783,#83784,#83785,#83786,#83787,#83788,#83789,#83790,
#83791,#83792,#83793,#83794,#83795,#83796,#83797,#83798,#83799,#83800,#83801,
#83802,#83803,#83804,#83805,#83806,#83807,#83808,#83809,#83810,#83811,#83812,
#83813,#83814,#83815,#83816,#83817,#83818,#83819,#83820,#83821,#83822,#83823,
#83824,#83825,#83826,#83827,#83828,#83829,#83830,#83831,#83832,#83833,#83834,
#83835,#83836,#83837,#83838,#83839,#83840,#83841,#83842,#83843,#83844,#83845,
#83846,#83847,#83848,#83849,#83850,#83851,#83852,#83853,#83854,#83855,#83856,
#83857,#83858,#83859,#83860,#83861,#83862,#83863,#83864,#83865,#83866,#83867,
#83868),.UNSPECIFIED.,.F.,.F.,(4,3,3,3,3,3,3,3,3,3,3,3,3,3,3,3,3,3,3,3,
3,3,3,3,3,3,3,3,3,3,3,3,3,3,3,3,3,3,3,3,3,3,3,3,3,3,3,3,3,3,3,3,3,3,3,3,
3,3,3,3,3,3,3,3,3,3,3,3,3,3,3,3,3,3,3,4),(233.587901756539,233.694378808573,
233.802304697791,233.886542415262,233.975097061021,234.063536990865,234.151886005719,
234.243657449228,234.331904215935,234.420137563137,234.508378856785,234.596649463416,
234.685020409845,234.773450873236,234.862011548726,234.886057553789,234.974612775169,
235.063053288167,235.151402892939,235.243174117861,235.331421487515,235.419655441421,
235.50789734487,235.596168563739,235.68454012287,235.77297119999,235.861532485909,
235.885572692316,235.974124503413,236.06256159786,236.150907779833,236.242680286209,
236.330924243718,236.419154795135,236.507393309305,236.595661155676,236.684029384112,
236.77245715074,236.861015181431,236.885087830843,236.973644590983,237.062086624006,
237.150437728593,237.24220838369,237.330457194067,237.41869256461,237.50693585923,
237.595208442402,237.68358131942,237.772013689061,237.860576220479,237.88460296937,
237.973161973041,238.061606301539,238.149959750189,238.241729544902,238.329980804653,
238.418218659028,238.506464469126,238.594739596636,238.683115047461,238.771550011202,
238.860115146021,238.884118107896,238.972460561993,239.060688395686,239.148825659066,
239.239108312124,239.327145265534,239.415169489258,239.503202570966,239.595173649107,
239.68333984933,239.771567865194,239.859922378897,239.871086883532),
 .UNSPECIFIED.);
#7878=B_SPLINE_CURVE_WITH_KNOTS('',3,(#83870,#83871,#83872,#83873,#83874,
#83875,#83876,#83877,#83878,#83879,#83880,#83881,#83882,#83883,#83884,#83885,
#83886,#83887,#83888,#83889,#83890,#83891,#83892,#83893,#83894,#83895,#83896,
#83897,#83898,#83899,#83900,#83901,#83902,#83903,#83904,#83905,#83906,#83907,
#83908,#83909,#83910,#83911,#83912,#83913,#83914,#83915,#83916,#83917,#83918,
#83919,#83920,#83921,#83922,#83923,#83924,#83925,#83926,#83927,#83928,#83929,
#83930,#83931,#83932,#83933,#83934,#83935,#83936,#83937,#83938,#83939,#83940,
#83941,#83942,#83943,#83944,#83945,#83946,#83947,#83948,#83949,#83950,#83951,
#83952,#83953,#83954,#83955,#83956,#83957,#83958,#83959,#83960,#83961,#83962,
#83963,#83964,#83965,#83966,#83967,#83968,#83969,#83970,#83971,#83972,#83973,
#83974,#83975,#83976,#83977,#83978,#83979,#83980,#83981,#83982,#83983,#83984,
#83985,#83986,#83987,#83988,#83989,#83990,#83991,#83992,#83993,#83994,#83995,
#83996,#83997,#83998,#83999,#84000,#84001,#84002,#84003,#84004,#84005,#84006,
#84007,#84008,#84009,#84010,#84011,#84012,#84013,#84014,#84015,#84016,#84017,
#84018,#84019,#84020,#84021,#84022,#84023,#84024,#84025,#84026,#84027,#84028,
#84029,#84030,#84031,#84032,#84033,#84034,#84035,#84036,#84037,#84038,#84039,
#84040,#84041,#84042,#84043,#84044,#84045,#84046,#84047,#84048,#84049,#84050),
 .UNSPECIFIED.,.F.,.F.,(4,3,3,3,3,3,3,3,3,3,3,3,3,3,3,3,3,3,3,3,3,3,3,3,
3,3,3,3,3,3,3,3,3,3,3,3,3,3,3,3,3,3,3,3,3,3,3,3,3,3,3,3,3,3,3,3,3,3,3,3,
4),(239.871086883736,239.883633246423,239.972208372219,240.060668706586,
240.149038028121,240.240801822725,240.329068529199,240.417321647942,240.505582524723,
240.593872505738,240.682262421262,240.770711641347,240.859290618007,240.88314838495,
240.97172640819,241.060189991207,241.148562903905,241.240325481352,241.32859660096,
241.416854426589,241.505120297491,241.593415553553,241.681811129969,241.770266242208,
241.858851401616,241.882663523477,241.97109354429,242.059408581874,242.147632580698,
242.239450840861,242.327573045086,242.415682201121,242.503799801744,242.591947340844,
242.680196761928,242.768506443136,242.856948365817,242.882178662003,242.970905168179,
243.059516527781,243.14803634618,243.239743527974,243.328158477201,243.416558752347,
243.504965543172,243.593400038828,243.681931674474,243.770521156149,243.859237186955,
243.88169380053,243.96950795302,244.057209821738,244.14482398992,244.232377230877,
244.319899046808,244.407411513512,244.49493669478,244.582548289539,244.670205938562,
244.757997774109,244.81888007831),.UNSPECIFIED.);
#7879=B_SPLINE_CURVE_WITH_KNOTS('',3,(#84054,#84055,#84056,#84057,#84058,
#84059,#84060,#84061),.UNSPECIFIED.,.F.,.F.,(4,1,1,1,1,4),(-246.88023921611,
-245.880724077584,-244.881208939057,-243.88169380053,-242.882178662003,
-242.853790713018),.UNSPECIFIED.);
#7880=B_SPLINE_CURVE_WITH_KNOTS('',3,(#84063,#84064,#84065,#84066,#84067,
#84068,#84069,#84070,#84071,#84072,#84073,#84074,#84075,#84076,#84077,#84078,
#84079,#84080,#84081,#84082,#84083,#84084,#84085,#84086,#84087,#84088,#84089,
#84090,#84091,#84092,#84093,#84094,#84095,#84096,#84097,#84098,#84099,#84100,
#84101,#84102,#84103,#84104,#84105,#84106,#84107,#84108,#84109,#84110,#84111,
#84112,#84113,#84114,#84115,#84116,#84117,#84118,#84119,#84120,#84121,#84122,
#84123,#84124,#84125,#84126,#84127,#84128,#84129,#84130,#84131,#84132,#84133,
#84134,#84135,#84136,#84137,#84138,#84139,#84140,#84141,#84142,#84143,#84144,
#84145,#84146,#84147,#84148,#84149,#84150,#84151,#84152,#84153,#84154,#84155,
#84156,#84157,#84158,#84159,#84160,#84161,#84162,#84163,#84164,#84165,#84166,
#84167,#84168,#84169,#84170,#84171,#84172,#84173,#84174,#84175,#84176,#84177,
#84178,#84179,#84180,#84181,#84182,#84183,#84184,#84185,#84186,#84187,#84188,
#84189,#84190,#84191,#84192,#84193,#84194,#84195,#84196,#84197,#84198,#84199,
#84200,#84201,#84202,#84203,#84204,#84205,#84206,#84207,#84208,#84209,#84210,
#84211,#84212,#84213,#84214,#84215,#84216,#84217,#84218,#84219,#84220,#84221,
#84222,#84223,#84224,#84225,#84226,#84227,#84228,#84229,#84230,#84231,#84232,
#84233,#84234,#84235,#84236,#84237,#84238,#84239,#84240,#84241,#84242,#84243,
#84244,#84245,#84246,#84247,#84248,#84249,#84250,#84251,#84252,#84253,#84254,
#84255,#84256,#84257,#84258,#84259,#84260,#84261,#84262,#84263,#84264,#84265,
#84266,#84267,#84268,#84269,#84270,#84271,#84272,#84273,#84274,#84275,#84276,
#84277,#84278,#84279,#84280,#84281,#84282,#84283,#84284,#84285),
 .UNSPECIFIED.,.F.,.F.,(4,3,3,3,3,3,3,3,3,3,3,3,3,3,3,3,3,3,3,3,3,3,3,3,
3,3,3,3,3,3,3,3,3,3,3,3,3,3,3,3,3,3,3,3,3,3,3,3,3,3,3,3,3,3,3,3,3,3,3,3,
3,3,3,3,3,3,3,3,3,3,3,3,3,3,4),(-242.853790713018,-242.765773024893,-242.677869948349,
-242.590057088657,-242.501632893009,-242.413917985828,-242.326214927956,
-242.238501828221,-242.149542252035,-242.061695811257,-241.972179667367,
-241.882663523477,-241.794084508876,-241.705620118365,-241.6172465813,-241.525484306756,
-241.437213022899,-241.348955203009,-241.260689507824,-241.172394597576,
-241.083999617283,-240.995545247635,-240.906961039838,-240.88314838495,
-240.794575532451,-240.706117036234,-240.617749119541,-240.525984635402,
-240.437718245461,-240.349465041323,-240.261203677315,-240.172912807041,
-240.084521410963,-239.996070364259,-239.907489067623,-239.883633246423,
-239.795095981985,-239.706673656451,-239.618342446681,-239.526564404333,
-239.438335833301,-239.350120795425,-239.261897905745,-239.173645778763,
-239.085293331673,-238.996881402064,-238.908339167613,-238.884118107896,
-238.795559054846,-238.707114685267,-238.618761203808,-238.526991424503,
-238.438740152753,-238.350502294075,-238.262256487372,-238.173981370968,
-238.085605942618,-237.997171008,-237.908605911828,-237.88460296937,-237.796046512253,
-237.707604724215,-237.619253806823,-237.527483059826,-237.439234291475,
-237.350998909353,-237.262755549564,-237.174482847605,-237.086109772928,
-236.997677159474,-236.909114318416,-236.885087830843,-236.778947052171,
-236.673986362008,-236.570605614479),.UNSPECIFIED.);
#7881=B_SPLINE_CURVE_WITH_KNOTS('',3,(#84287,#84288,#84289,#84290,#84291,
#84292,#84293,#84294,#84295,#84296),.UNSPECIFIED.,.F.,.F.,(4,1,1,1,1,1,
1,4),(-236.570605405839,-235.885572692316,-234.886057553789,-233.886542415262,
-232.887027276736,-231.887512138209,-230.887996999682,-230.287420098659),
 .UNSPECIFIED.);
#7882=B_SPLINE_CURVE_WITH_KNOTS('',3,(#84298,#84299,#84300,#84301,#84302,
#84303,#84304,#84305,#84306,#84307,#84308,#84309,#84310,#84311,#84312,#84313,
#84314,#84315,#84316,#84317,#84318,#84319,#84320,#84321,#84322,#84323,#84324,
#84325,#84326,#84327,#84328,#84329,#84330,#84331,#84332,#84333,#84334,#84335,
#84336,#84337,#84338,#84339,#84340,#84341,#84342,#84343,#84344,#84345,#84346,
#84347,#84348,#84349,#84350,#84351,#84352,#84353,#84354,#84355,#84356,#84357,
#84358,#84359,#84360,#84361,#84362,#84363,#84364,#84365,#84366,#84367,#84368,
#84369,#84370,#84371,#84372,#84373,#84374,#84375,#84376,#84377,#84378,#84379,
#84380,#84381,#84382,#84383,#84384,#84385,#84386,#84387,#84388,#84389,#84390,
#84391,#84392,#84393,#84394,#84395,#84396,#84397,#84398,#84399,#84400,#84401,
#84402,#84403,#84404,#84405,#84406,#84407,#84408,#84409,#84410,#84411,#84412,
#84413,#84414,#84415,#84416,#84417,#84418,#84419,#84420,#84421,#84422,#84423,
#84424,#84425,#84426,#84427,#84428,#84429,#84430,#84431,#84432,#84433,#84434,
#84435,#84436,#84437,#84438,#84439,#84440,#84441,#84442,#84443,#84444,#84445,
#84446,#84447,#84448,#84449,#84450,#84451,#84452,#84453,#84454,#84455,#84456,
#84457,#84458,#84459,#84460,#84461,#84462,#84463,#84464,#84465,#84466,#84467,
#84468,#84469,#84470,#84471,#84472,#84473,#84474,#84475,#84476,#84477,#84478,
#84479,#84480,#84481,#84482,#84483,#84484,#84485,#84486,#84487,#84488,#84489,
#84490,#84491,#84492,#84493,#84494,#84495,#84496,#84497,#84498,#84499,#84500,
#84501,#84502,#84503,#84504,#84505,#84506,#84507,#84508,#84509,#84510,#84511,
#84512,#84513,#84514,#84515,#84516,#84517,#84518,#84519,#84520,#84521,#84522,
#84523),.UNSPECIFIED.,.F.,.F.,(4,3,3,3,3,3,3,3,3,3,3,3,3,3,3,3,3,3,3,3,
3,3,3,3,3,3,3,3,3,3,3,3,3,3,3,3,3,3,3,3,3,3,3,3,3,3,3,3,3,3,3,3,3,3,3,3,
3,3,3,3,3,3,3,3,3,3,3,3,3,3,3,3,3,3,3,4),(-230.287419873382,-230.187685370325,
-230.089695435759,-229.989088648457,-229.888481861155,-229.799927438089,
-229.711487728505,-229.623138931259,-229.53136740518,-229.443120848196,
-229.354887707474,-229.266646616858,-229.178376209606,-229.090005456174,
-229.001575182305,-228.9130146898,-228.888966722629,-228.80041232085,-228.71197263272,
-228.623623857066,-228.531852322945,-228.443605787764,-228.355372668885,
-228.267131600131,-228.178861214733,-228.090490483036,-228.002060230859,
-227.913499759814,-227.889451584102,-227.800897188767,-227.712457507237,
-227.624108738331,-227.532337201737,-227.444090673634,-227.355857561944,
-227.267616500481,-227.17934612247,-227.090975398267,-227.002545153654,
-226.913984690219,-226.889936445575,-226.80138204078,-226.712942349655,
-226.624593571034,-226.532822038036,-226.444575499973,-226.35634237825,
-226.26810130669,-226.179830918531,-226.091460184152,-226.003029929335,
-225.914469455733,-225.890421307048,-225.80186690584,-225.713427218336,
-225.625078443363,-225.533306909008,-225.445060374642,-225.356827256626,
-225.268586188782,-225.180315804342,-225.091945073667,-225.003514822552,
-224.914954352618,-224.890906168522,-224.803533528896,-224.716274617417,
-224.627269639174,-224.540163709119,-224.453089248357,-224.366023837001,
-224.275576575621,-224.188419159953,-224.101213336875,-224.013898682601,
-224.00423479148),.UNSPECIFIED.);
#7883=B_SPLINE_CURVE_WITH_KNOTS('',3,(#84525,#84526,#84527,#84528,#84529,
#84530,#84531,#84532,#84533,#84534,#84535),.UNSPECIFIED.,.F.,.F.,(4,1,1,
1,1,1,1,1,4),(-224.00423479148,-223.891391029995,-222.891875891468,-221.892360752941,
-220.892845614415,-219.893330475888,-218.893815337361,-217.894300198834,
-217.7210494843),.UNSPECIFIED.);
#7884=B_SPLINE_CURVE_WITH_KNOTS('',3,(#84537,#84538,#84539,#84540,#84541,
#84542,#84543,#84544,#84545,#84546,#84547,#84548,#84549,#84550,#84551,#84552,
#84553,#84554,#84555,#84556,#84557,#84558,#84559,#84560,#84561,#84562,#84563,
#84564,#84565,#84566,#84567,#84568,#84569,#84570,#84571,#84572,#84573,#84574,
#84575,#84576,#84577,#84578,#84579,#84580,#84581,#84582,#84583,#84584,#84585,
#84586,#84587,#84588,#84589,#84590,#84591,#84592,#84593,#84594,#84595,#84596,
#84597,#84598,#84599,#84600,#84601,#84602,#84603,#84604,#84605,#84606,#84607,
#84608,#84609,#84610,#84611,#84612,#84613,#84614,#84615,#84616,#84617,#84618,
#84619,#84620,#84621,#84622,#84623,#84624,#84625,#84626,#84627,#84628,#84629,
#84630,#84631,#84632,#84633,#84634,#84635,#84636,#84637,#84638,#84639,#84640,
#84641,#84642,#84643,#84644,#84645,#84646,#84647,#84648,#84649,#84650,#84651,
#84652,#84653,#84654,#84655,#84656,#84657,#84658,#84659,#84660,#84661,#84662,
#84663,#84664,#84665,#84666,#84667,#84668,#84669,#84670,#84671,#84672,#84673,
#84674,#84675,#84676,#84677,#84678,#84679,#84680,#84681,#84682,#84683,#84684,
#84685,#84686,#84687,#84688,#84689,#84690,#84691,#84692,#84693,#84694,#84695,
#84696,#84697,#84698,#84699,#84700,#84701,#84702,#84703,#84704,#84705,#84706,
#84707,#84708,#84709,#84710,#84711,#84712,#84713,#84714,#84715,#84716,#84717,
#84718,#84719,#84720,#84721,#84722,#84723,#84724,#84725,#84726,#84727,#84728,
#84729,#84730,#84731,#84732,#84733,#84734,#84735,#84736,#84737,#84738,#84739,
#84740,#84741,#84742,#84743,#84744,#84745,#84746,#84747,#84748,#84749,#84750,
#84751,#84752,#84753,#84754,#84755,#84756,#84757,#84758,#84759,#84760,#84761,
#84762),.UNSPECIFIED.,.F.,.F.,(4,3,3,3,3,3,3,3,3,3,3,3,3,3,3,3,3,3,3,3,
3,3,3,3,3,3,3,3,3,3,3,3,3,3,3,3,3,3,3,3,3,3,3,3,3,3,3,3,3,3,3,3,3,3,3,3,
3,3,3,3,3,3,3,3,3,3,3,3,3,3,3,3,3,3,3,4),(-217.7210494843,-217.633946217353,
-217.546927581786,-217.45996462197,-217.373029360669,-217.286099284211,
-217.199151886862,-217.112114065454,-217.02502534541,-216.937804740184,
-216.894785060307,-216.806230658872,-216.717790971146,-216.629442195957,
-216.537670661685,-216.449424127116,-216.361191008904,-216.272949940869,
-216.184679556244,-216.096308825396,-216.007878574112,-215.91931810402,
-215.895269921781,-215.806715520344,-215.718275832616,-215.629927057425,
-215.538155523154,-215.449908988583,-215.361675870369,-215.273434802332,
-215.185164417706,-215.096793686855,-215.00836343557,-214.919802965476,
-214.895754783254,-214.807200381814,-214.718760694083,-214.630411918888,
-214.538640384618,-214.450393850045,-214.362160731827,-214.273919663787,
-214.185649279157,-214.097278548303,-214.008848297015,-213.920287826917,
-213.896239644727,-213.807685243289,-213.719245555561,-213.630896780368,
-213.539125246097,-213.450878711526,-213.362645593311,-213.274404525273,
-213.186134140645,-213.097763409794,-213.009333158508,-212.920772688412,
-212.8967245062,-212.808170104762,-212.719730417033,-212.63138164184,-212.53961010757,
-212.451363572998,-212.363130454783,-212.274889386745,-212.186619002118,
-212.098248271266,-212.00981801998,-211.921257549884,-211.897209367674,
-211.802221668775,-211.707535983373,-211.613032966347,-211.51880605863,
-211.437864395501),.UNSPECIFIED.);
#7885=B_SPLINE_CURVE_WITH_KNOTS('',3,(#84764,#84765,#84766,#84767,#84768,
#84769,#84770,#84771,#84772,#84773),.UNSPECIFIED.,.F.,.F.,(4,1,1,1,1,1,
1,4),(-211.43786417712,-210.897694229147,-209.89817909062,-208.898663952093,
-207.899148813567,-206.89963367504,-205.900118536513,-205.154678869941),
 .UNSPECIFIED.);
#7886=B_SPLINE_CURVE_WITH_KNOTS('',3,(#84775,#84776,#84777,#84778,#84779,
#84780,#84781,#84782,#84783,#84784,#84785,#84786,#84787,#84788,#84789,#84790,
#84791,#84792,#84793,#84794,#84795,#84796,#84797,#84798,#84799,#84800,#84801,
#84802,#84803,#84804,#84805,#84806,#84807,#84808,#84809,#84810,#84811,#84812,
#84813,#84814,#84815,#84816,#84817,#84818,#84819,#84820,#84821,#84822,#84823,
#84824,#84825,#84826,#84827,#84828,#84829,#84830,#84831,#84832,#84833,#84834,
#84835,#84836,#84837,#84838,#84839,#84840,#84841,#84842,#84843,#84844,#84845,
#84846,#84847,#84848,#84849,#84850,#84851,#84852,#84853,#84854,#84855,#84856,
#84857,#84858,#84859,#84860,#84861,#84862,#84863,#84864,#84865,#84866,#84867,
#84868,#84869,#84870,#84871,#84872,#84873,#84874,#84875,#84876,#84877,#84878,
#84879,#84880,#84881,#84882,#84883,#84884,#84885,#84886,#84887,#84888,#84889,
#84890,#84891,#84892,#84893,#84894,#84895,#84896,#84897,#84898,#84899,#84900,
#84901,#84902,#84903,#84904,#84905,#84906,#84907,#84908,#84909,#84910,#84911,
#84912,#84913,#84914,#84915,#84916,#84917,#84918,#84919,#84920,#84921,#84922,
#84923,#84924,#84925,#84926,#84927,#84928,#84929,#84930,#84931,#84932,#84933,
#84934,#84935,#84936,#84937,#84938,#84939,#84940,#84941,#84942,#84943,#84944,
#84945,#84946,#84947,#84948,#84949,#84950,#84951,#84952,#84953,#84954,#84955,
#84956,#84957,#84958,#84959,#84960,#84961,#84962,#84963,#84964,#84965,#84966,
#84967,#84968,#84969,#84970,#84971,#84972,#84973,#84974,#84975,#84976,#84977,
#84978,#84979,#84980,#84981,#84982,#84983,#84984,#84985,#84986,#84987,#84988,
#84989,#84990,#84991,#84992,#84993,#84994,#84995,#84996,#84997,#84998,#84999,
#85000,#85001,#85002,#85003),.UNSPECIFIED.,.F.,.F.,(4,3,3,3,3,3,3,3,3,3,
3,3,3,3,3,3,3,3,3,3,3,3,3,3,3,3,3,3,3,3,3,3,3,3,3,3,3,3,3,3,3,3,3,3,3,3,
3,3,3,3,3,3,3,3,3,3,3,3,3,3,3,3,3,3,3,3,3,3,3,3,3,3,3,3,3,3,4),(-205.154678738782,
-205.041978910697,-204.926813848051,-204.900603397986,-204.812048996549,
-204.723609308821,-204.635260533629,-204.543488999358,-204.455242464787,
-204.367009346572,-204.278768278535,-204.190497893908,-204.102127163057,
-204.013696911771,-203.925136441676,-203.90108825946,-203.812533858022,
-203.724094170292,-203.635745395099,-203.543973860829,-203.455727326257,
-203.367494208041,-203.279253140003,-203.190982755375,-203.102612024522,
-203.014181773236,-202.92562130314,-202.901573120933,-202.813018719495,
-202.724579031765,-202.636230256572,-202.544458722301,-202.456212187729,
-202.367979069513,-202.279738001475,-202.191467616847,-202.103096885994,
-202.014666634708,-201.926106164611,-201.902057982406,-201.813503580968,
-201.725063893239,-201.636715118046,-201.544943583775,-201.456697049203,
-201.368463930988,-201.280222862949,-201.191952478321,-201.103581747469,
-201.015151496183,-200.926591026087,-200.902542843879,-200.813988442441,
-200.725548754712,-200.63719997952,-200.545428445249,-200.457181910677,
-200.368948792462,-200.280707724424,-200.192437339796,-200.104066608944,
-200.015636357657,-199.927075887562,-199.903027705353,-199.814473303915,
-199.726033616186,-199.637684840994,-199.545913306723,-199.457666772151,
-199.369433653935,-199.281192585897,-199.19292220127,-199.104551470418,
-199.016121219131,-198.927560749036,-198.903512566826,-198.871493562761),
 .UNSPECIFIED.);
#7887=B_SPLINE_CURVE_WITH_KNOTS('',3,(#85005,#85006,#85007,#85008,#85009,
#85010,#85011,#85012,#85013,#85014,#85015,#85016,#85017,#85018,#85019,#85020,
#85021,#85022,#85023,#85024,#85025,#85026,#85027,#85028,#85029,#85030,#85031,
#85032,#85033,#85034,#85035,#85036,#85037,#85038,#85039,#85040,#85041,#85042,
#85043,#85044,#85045,#85046,#85047,#85048,#85049,#85050,#85051,#85052,#85053,
#85054,#85055,#85056,#85057,#85058,#85059,#85060,#85061,#85062,#85063,#85064,
#85065,#85066,#85067,#85068,#85069,#85070,#85071,#85072,#85073,#85074,#85075,
#85076,#85077,#85078,#85079,#85080,#85081,#85082,#85083,#85084,#85085,#85086,
#85087,#85088,#85089,#85090,#85091,#85092,#85093,#85094,#85095,#85096,#85097,
#85098,#85099,#85100,#85101,#85102,#85103,#85104,#85105,#85106,#85107,#85108,
#85109,#85110,#85111,#85112,#85113,#85114,#85115,#85116,#85117,#85118,#85119,
#85120,#85121,#85122,#85123,#85124,#85125,#85126,#85127,#85128,#85129,#85130,
#85131,#85132,#85133,#85134,#85135,#85136,#85137,#85138,#85139,#85140,#85141,
#85142,#85143,#85144,#85145,#85146,#85147,#85148,#85149,#85150,#85151,#85152,
#85153,#85154,#85155,#85156,#85157,#85158,#85159,#85160,#85161,#85162,#85163,
#85164,#85165,#85166,#85167,#85168,#85169,#85170,#85171,#85172,#85173,#85174,
#85175,#85176,#85177,#85178,#85179,#85180,#85181,#85182,#85183,#85184,#85185,
#85186,#85187,#85188,#85189,#85190,#85191,#85192,#85193,#85194,#85195,#85196,
#85197,#85198,#85199,#85200,#85201,#85202,#85203,#85204,#85205,#85206,#85207,
#85208,#85209,#85210,#85211,#85212,#85213,#85214,#85215,#85216,#85217,#85218,
#85219,#85220,#85221,#85222,#85223,#85224,#85225,#85226,#85227),
 .UNSPECIFIED.,.F.,.F.,(4,3,3,3,3,3,3,3,3,3,3,3,3,3,3,3,3,3,3,3,3,3,3,3,
3,3,3,3,3,3,3,3,3,3,3,3,3,3,3,3,3,3,3,3,3,3,3,3,3,3,3,3,3,3,3,3,3,3,3,3,
3,3,3,3,3,3,3,3,3,3,3,3,3,3,4),(-198.871493562533,-198.783408527569,-198.6954365812,
-198.607553404627,-198.519608907586,-198.431820567895,-198.344043110297,
-198.256254704546,-198.168190385484,-198.080268257862,-197.992132843081,
-197.903997428299,-197.815443026861,-197.727003339132,-197.638654563939,
-197.546883029668,-197.458636495096,-197.37040337688,-197.282162308842,
-197.193891924214,-197.105521193362,-197.017090942075,-196.928530471979,
-196.904482289772,-196.815927888334,-196.727488200604,-196.639139425411,
-196.54736789114,-196.459121356568,-196.370888238353,-196.282647170314,
-196.194376785686,-196.106006054834,-196.017575803547,-195.929015333451,
-195.904967151245,-195.816412749807,-195.727973062078,-195.639624286886,
-195.547852752615,-195.459606218043,-195.371373099828,-195.28313203179,
-195.194861647162,-195.106490916311,-195.018060665024,-194.929500194928,
-194.905452012719,-194.816897611281,-194.728457923552,-194.640109148359,
-194.548337614088,-194.460091079516,-194.371857961301,-194.283616893262,
-194.195346508634,-194.106975777782,-194.018545526496,-193.9299850564,-193.905936874192,
-193.817382472754,-193.728942785024,-193.640594009831,-193.54882247556,
-193.460575940988,-193.372342822773,-193.284101754734,-193.195831370106,
-193.107460639254,-193.019030387966,-192.93046991787,-192.906421735665,
-192.800699836041,-192.694504152843,-192.588308469644),.UNSPECIFIED.);
#7888=B_SPLINE_CURVE_WITH_KNOTS('',3,(#85229,#85230,#85231,#85232,#85233,
#85234,#85235,#85236,#85237,#85238),.UNSPECIFIED.,.F.,.F.,(4,1,1,1,1,1,
1,4),(-192.588308255582,-191.906906597138,-190.907391458612,-189.907876320085,
-188.908361181558,-187.908846043031,-186.909330904505,-186.305122948402),
 .UNSPECIFIED.);
#7889=B_SPLINE_CURVE_WITH_KNOTS('',3,(#85240,#85241,#85242,#85243,#85244,
#85245,#85246,#85247,#85248,#85249,#85250,#85251,#85252,#85253,#85254,#85255,
#85256,#85257,#85258,#85259,#85260,#85261,#85262,#85263,#85264,#85265,#85266,
#85267,#85268,#85269,#85270,#85271,#85272,#85273,#85274,#85275,#85276,#85277,
#85278,#85279,#85280,#85281,#85282,#85283,#85284,#85285,#85286,#85287,#85288,
#85289,#85290,#85291,#85292,#85293,#85294,#85295,#85296,#85297,#85298,#85299,
#85300,#85301,#85302,#85303,#85304,#85305,#85306,#85307,#85308,#85309,#85310,
#85311,#85312,#85313,#85314,#85315,#85316,#85317,#85318,#85319,#85320,#85321,
#85322,#85323,#85324,#85325,#85326,#85327,#85328,#85329,#85330,#85331,#85332,
#85333,#85334,#85335,#85336,#85337,#85338,#85339,#85340,#85341,#85342,#85343,
#85344,#85345,#85346,#85347,#85348,#85349,#85350,#85351,#85352,#85353,#85354,
#85355,#85356,#85357,#85358,#85359,#85360,#85361,#85362,#85363,#85364,#85365,
#85366,#85367,#85368,#85369,#85370,#85371,#85372,#85373,#85374,#85375,#85376,
#85377,#85378,#85379,#85380,#85381,#85382,#85383,#85384,#85385,#85386,#85387,
#85388,#85389,#85390,#85391,#85392,#85393,#85394,#85395,#85396,#85397,#85398,
#85399,#85400,#85401,#85402,#85403,#85404,#85405,#85406,#85407,#85408,#85409,
#85410,#85411,#85412,#85413,#85414,#85415,#85416,#85417,#85418,#85419,#85420,
#85421,#85422,#85423,#85424,#85425,#85426,#85427,#85428,#85429,#85430,#85431,
#85432,#85433,#85434,#85435,#85436,#85437,#85438,#85439,#85440,#85441,#85442,
#85443,#85444,#85445,#85446,#85447,#85448,#85449,#85450,#85451,#85452,#85453,
#85454,#85455,#85456,#85457,#85458,#85459,#85460,#85461,#85462,#85463,#85464,
#85465),.UNSPECIFIED.,.F.,.F.,(4,3,3,3,3,3,3,3,3,3,3,3,3,3,3,3,3,3,3,3,
3,3,3,3,3,3,3,3,3,3,3,3,3,3,3,3,3,3,3,3,3,3,3,3,3,3,3,3,3,3,3,3,3,3,3,3,
3,3,3,3,3,3,3,3,3,3,3,3,3,3,3,3,3,3,3,4),(-186.305122719083,-186.206295980807,
-186.108059058831,-186.008937412404,-185.909815765978,-185.82126136454,
-185.73282167681,-185.644472901617,-185.552701367347,-185.464454832775,
-185.376221714559,-185.28798064652,-185.199710261892,-185.11133953104,-185.022909279753,
-184.934348809657,-184.910300627451,-184.821746226013,-184.733306538283,
-184.64495776309,-184.55318622882,-184.464939694248,-184.376706576032,-184.288465507994,
-184.200195123365,-184.111824392513,-184.023394141226,-183.93483367113,
-183.910785488924,-183.822231087486,-183.733791399757,-183.645442624565,
-183.553671090294,-183.465424555722,-183.377191437507,-183.288950369469,
-183.200679984841,-183.112309253989,-183.023879002703,-182.935318532607,
-182.911270350398,-182.82271594896,-182.734276261231,-182.645927486038,
-182.554155951767,-182.465909417195,-182.377676298979,-182.289435230941,
-182.201164846313,-182.112794115461,-182.024363864175,-181.935803394079,
-181.911755211871,-181.823200810433,-181.734761122703,-181.64641234751,
-181.554640813239,-181.466394278667,-181.378161160451,-181.289920092413,
-181.201649707785,-181.113278976933,-181.024848725646,-180.93628825555,
-180.912240073344,-180.824848370936,-180.737570403042,-180.648116307815,
-180.560991488546,-180.473898053107,-180.386813595069,-180.295594606608,
-180.208417027578,-180.121190868464,-180.033854467656,-180.021937641223),
 .UNSPECIFIED.);
#7890=B_SPLINE_CURVE_WITH_KNOTS('',3,(#85467,#85468,#85469,#85470,#85471,
#85472,#85473,#85474,#85475,#85476,#85477),.UNSPECIFIED.,.F.,.F.,(4,1,1,
1,1,1,1,1,4),(-180.021937641223,-179.912724934817,-178.913209796291,-177.913694657764,
-176.914179519237,-175.91466438071,-174.915149242184,-173.915634103657,
-173.738752334043),.UNSPECIFIED.);
#7891=B_SPLINE_CURVE_WITH_KNOTS('',3,(#85479,#85480,#85481,#85482,#85483,
#85484,#85485,#85486,#85487,#85488,#85489,#85490,#85491,#85492,#85493,#85494,
#85495,#85496,#85497,#85498,#85499,#85500,#85501,#85502,#85503,#85504,#85505,
#85506,#85507,#85508,#85509,#85510,#85511,#85512,#85513,#85514,#85515,#85516,
#85517,#85518,#85519,#85520,#85521,#85522,#85523,#85524,#85525,#85526,#85527,
#85528,#85529,#85530,#85531,#85532,#85533,#85534,#85535,#85536,#85537,#85538,
#85539,#85540,#85541,#85542,#85543,#85544,#85545,#85546,#85547,#85548,#85549,
#85550,#85551,#85552,#85553,#85554,#85555,#85556,#85557,#85558,#85559,#85560,
#85561,#85562,#85563,#85564,#85565,#85566,#85567,#85568,#85569,#85570,#85571,
#85572,#85573,#85574,#85575,#85576,#85577,#85578,#85579,#85580,#85581,#85582,
#85583,#85584,#85585,#85586,#85587,#85588,#85589,#85590,#85591,#85592,#85593,
#85594,#85595,#85596,#85597,#85598,#85599,#85600,#85601,#85602,#85603,#85604,
#85605,#85606,#85607,#85608,#85609,#85610,#85611,#85612,#85613,#85614,#85615,
#85616,#85617,#85618,#85619,#85620,#85621,#85622,#85623,#85624,#85625,#85626,
#85627,#85628,#85629,#85630,#85631,#85632,#85633,#85634,#85635,#85636,#85637,
#85638,#85639,#85640,#85641,#85642,#85643,#85644,#85645,#85646,#85647,#85648,
#85649,#85650,#85651,#85652,#85653,#85654,#85655,#85656,#85657,#85658,#85659,
#85660,#85661,#85662,#85663,#85664,#85665,#85666,#85667,#85668,#85669,#85670,
#85671,#85672,#85673,#85674,#85675,#85676,#85677,#85678,#85679,#85680,#85681,
#85682,#85683,#85684,#85685,#85686,#85687,#85688,#85689,#85690,#85691,#85692,
#85693,#85694,#85695,#85696,#85697,#85698,#85699,#85700,#85701,#85702,#85703,
#85704),.UNSPECIFIED.,.F.,.F.,(4,3,3,3,3,3,3,3,3,3,3,3,3,3,3,3,3,3,3,3,
3,3,3,3,3,3,3,3,3,3,3,3,3,3,3,3,3,3,3,3,3,3,3,3,3,3,3,3,3,3,3,3,3,3,3,3,
3,3,3,3,3,3,3,3,3,3,3,3,3,3,3,3,3,3,3,4),(-173.738752334043,-173.651651184399,
-173.564633597389,-173.477670273051,-173.390733687792,-173.303801330066,
-173.216850695373,-173.129809112975,-173.0427157747,-172.955491530016,-172.91611896513,
-172.827564563692,-172.739124875963,-172.65077610077,-172.559004566499,
-172.470758031927,-172.382524913711,-172.294283845673,-172.206013461045,
-172.117642730193,-172.029212478907,-171.940652008811,-171.916603826603,
-171.828049425165,-171.739609737435,-171.651260962242,-171.559489427972,
-171.4712428934,-171.383009775184,-171.294768707145,-171.206498322517,-171.118127591665,
-171.029697340378,-170.941136870282,-170.917088688076,-170.828534286638,
-170.740094598909,-170.651745823717,-170.559974289446,-170.471727754874,
-170.383494636659,-170.295253568621,-170.206983183993,-170.118612453141,
-170.030182201854,-169.941621731759,-169.91757354955,-169.829019148112,
-169.740579460383,-169.65223068519,-169.560459150919,-169.472212616347,
-169.383979498132,-169.295738430094,-169.207468045466,-169.119097314613,
-169.030667063327,-168.942106593231,-168.918058411023,-168.829504009585,
-168.741064321855,-168.652715546662,-168.560944012392,-168.47269747782,
-168.384464359604,-168.296223291566,-168.207952906938,-168.119582176085,
-168.031151924799,-167.942591454702,-167.918543272496,-167.823739794189,
-167.729232464533,-167.634903277923,-167.54084246258,-167.45556722681),
 .UNSPECIFIED.);
#7892=B_SPLINE_CURVE_WITH_KNOTS('',3,(#85706,#85707,#85708,#85709,#85710,
#85711,#85712,#85713,#85714,#85715),.UNSPECIFIED.,.F.,.F.,(4,1,1,1,1,1,
1,4),(-167.455567026863,-166.919028133969,-165.919512995443,-164.919997856916,
-163.920482718389,-162.920967579862,-161.921452441336,-161.172381719684),
 .UNSPECIFIED.);
#7893=B_SPLINE_CURVE_WITH_KNOTS('',3,(#85717,#85718,#85719,#85720,#85721,
#85722,#85723,#85724,#85725,#85726,#85727,#85728,#85729,#85730,#85731,#85732,
#85733,#85734,#85735,#85736,#85737,#85738,#85739,#85740,#85741,#85742,#85743,
#85744,#85745,#85746,#85747,#85748,#85749,#85750,#85751,#85752,#85753,#85754,
#85755,#85756,#85757,#85758,#85759,#85760,#85761,#85762,#85763,#85764,#85765,
#85766,#85767,#85768,#85769,#85770,#85771,#85772,#85773,#85774,#85775,#85776,
#85777,#85778,#85779,#85780,#85781,#85782,#85783,#85784,#85785,#85786,#85787,
#85788,#85789,#85790,#85791,#85792,#85793,#85794,#85795,#85796,#85797,#85798,
#85799,#85800,#85801,#85802,#85803,#85804,#85805,#85806,#85807,#85808,#85809,
#85810,#85811,#85812,#85813,#85814,#85815,#85816,#85817,#85818,#85819,#85820,
#85821,#85822,#85823,#85824,#85825,#85826,#85827,#85828,#85829,#85830,#85831,
#85832,#85833,#85834,#85835,#85836,#85837,#85838,#85839,#85840,#85841,#85842,
#85843,#85844,#85845,#85846,#85847,#85848,#85849,#85850,#85851,#85852,#85853,
#85854,#85855,#85856,#85857,#85858,#85859,#85860,#85861,#85862,#85863,#85864,
#85865,#85866,#85867,#85868,#85869,#85870,#85871,#85872,#85873,#85874,#85875,
#85876,#85877,#85878,#85879,#85880,#85881,#85882,#85883,#85884,#85885,#85886,
#85887,#85888,#85889,#85890,#85891,#85892,#85893,#85894,#85895,#85896,#85897,
#85898,#85899,#85900,#85901,#85902,#85903,#85904,#85905,#85906,#85907,#85908,
#85909,#85910,#85911,#85912,#85913,#85914,#85915,#85916,#85917,#85918,#85919,
#85920,#85921,#85922,#85923,#85924,#85925,#85926,#85927,#85928,#85929,#85930,
#85931,#85932,#85933,#85934,#85935,#85936,#85937,#85938,#85939,#85940,#85941,
#85942,#85943,#85944,#85945),.UNSPECIFIED.,.F.,.F.,(4,3,3,3,3,3,3,3,3,3,
3,3,3,3,3,3,3,3,3,3,3,3,3,3,3,3,3,3,3,3,3,3,3,3,3,3,3,3,3,3,3,3,3,3,3,3,
3,3,3,3,3,3,3,3,3,3,3,3,3,3,3,3,3,3,3,3,3,3,3,3,3,3,3,3,3,3,4),(-161.172381610342,
-161.059073294057,-160.943174354892,-160.921937302809,-160.833382901371,
-160.744943213641,-160.656594438448,-160.564822904177,-160.476576369605,
-160.38834325139,-160.300102183351,-160.211831798723,-160.123461067871,
-160.035030816584,-159.946470346488,-159.922422164282,-159.833867762844,
-159.745428075115,-159.657079299922,-159.565307765651,-159.477061231079,
-159.388828112864,-159.300587044825,-159.212316660197,-159.123945929345,
-159.035515678059,-158.946955207963,-158.922907025755,-158.834352624317,
-158.745912936587,-158.657564161395,-158.565792627124,-158.477546092552,
-158.389312974336,-158.301071906298,-158.21280152167,-158.124430790818,
-158.036000539531,-157.947440069435,-157.923391887228,-157.83483748579,
-157.746397798061,-157.658049022869,-157.566277488598,-157.478030954026,
-157.389797835811,-157.301556767773,-157.213286383145,-157.124915652293,
-157.036485401007,-156.947924930911,-156.923876748702,-156.835322347264,
-156.746882659535,-156.658533884342,-156.566762350071,-156.478515815499,
-156.390282697283,-156.302041629245,-156.213771244617,-156.125400513765,
-156.036970262479,-155.948409792383,-155.924361610175,-155.835807208737,
-155.747367521008,-155.659018745815,-155.567247211544,-155.479000676972,
-155.390767558756,-155.302526490718,-155.21425610609,-155.125885375237,
-155.037455123951,-154.948894653855,-154.924846471648,-154.889196412504),
 .UNSPECIFIED.);
#7894=B_SPLINE_CURVE_WITH_KNOTS('',3,(#85947,#85948,#85949,#85950,#85951,
#85952,#85953,#85954,#85955,#85956,#85957,#85958,#85959,#85960,#85961,#85962,
#85963,#85964,#85965,#85966,#85967,#85968,#85969,#85970,#85971,#85972,#85973,
#85974,#85975,#85976,#85977,#85978,#85979,#85980,#85981,#85982,#85983,#85984,
#85985,#85986,#85987,#85988,#85989,#85990,#85991,#85992,#85993,#85994,#85995,
#85996,#85997,#85998,#85999,#86000,#86001,#86002,#86003,#86004,#86005,#86006,
#86007,#86008,#86009,#86010,#86011,#86012,#86013,#86014,#86015,#86016,#86017,
#86018,#86019,#86020,#86021,#86022,#86023,#86024,#86025,#86026,#86027,#86028,
#86029,#86030,#86031,#86032,#86033,#86034,#86035,#86036,#86037,#86038,#86039,
#86040,#86041,#86042,#86043,#86044,#86045,#86046,#86047,#86048,#86049,#86050,
#86051,#86052,#86053,#86054,#86055,#86056,#86057,#86058,#86059,#86060,#86061,
#86062,#86063,#86064,#86065,#86066,#86067,#86068,#86069,#86070,#86071,#86072,
#86073,#86074,#86075,#86076,#86077,#86078,#86079,#86080,#86081,#86082,#86083,
#86084,#86085,#86086,#86087,#86088,#86089,#86090,#86091,#86092,#86093,#86094,
#86095,#86096,#86097,#86098,#86099,#86100,#86101,#86102,#86103,#86104,#86105,
#86106,#86107,#86108,#86109,#86110,#86111,#86112,#86113,#86114,#86115,#86116,
#86117,#86118,#86119,#86120,#86121,#86122,#86123,#86124,#86125,#86126,#86127,
#86128,#86129,#86130,#86131,#86132,#86133,#86134,#86135,#86136,#86137,#86138,
#86139,#86140,#86141,#86142,#86143,#86144,#86145,#86146,#86147,#86148,#86149,
#86150,#86151,#86152,#86153,#86154,#86155,#86156,#86157,#86158,#86159,#86160,
#86161,#86162,#86163,#86164,#86165,#86166,#86167,#86168,#86169),
 .UNSPECIFIED.,.F.,.F.,(4,3,3,3,3,3,3,3,3,3,3,3,3,3,3,3,3,3,3,3,3,3,3,3,
3,3,3,3,3,3,3,3,3,3,3,3,3,3,3,3,3,3,3,3,3,3,3,3,3,3,3,3,3,3,3,3,3,3,3,3,
3,3,3,3,3,3,3,3,3,3,3,3,3,3,4),(-154.889196412254,-154.801158728298,-154.713233796906,
-154.625397253078,-154.537622184238,-154.449879442421,-154.362147142838,
-154.274403413472,-154.186569833671,-154.098691851588,-154.010667087164,
-153.925331333121,-153.836776931683,-153.748337243954,-153.659988468762,
-153.568216934491,-153.479970399919,-153.391737281704,-153.303496213666,
-153.215225829038,-153.126855098186,-153.038424846899,-152.949864376804,
-152.925816194595,-152.837261793157,-152.748822105428,-152.660473330235,
-152.568701795964,-152.480455261392,-152.392222143177,-152.303981075138,
-152.21571069051,-152.127339959658,-152.038909708372,-151.950349238276,
-151.926301056068,-151.83774665463,-151.7493069669,-151.660958191708,-151.569186657437,
-151.480940122865,-151.392707004649,-151.30446593661,-151.216195551982,
-151.12782482113,-151.039394569843,-150.950834099747,-150.926785917541,
-150.838231516103,-150.749791828374,-150.661443053181,-150.56967151891,
-150.481424984338,-150.393191866122,-150.304950798084,-150.216680413455,
-150.128309682603,-150.039879431317,-149.951318961221,-149.927270779014,
-149.838716377576,-149.750276689847,-149.661927914655,-149.570156380384,
-149.481909845812,-149.393676727597,-149.305435659559,-149.217165274931,
-149.128794544079,-149.040364292792,-148.951803822697,-148.927755640488,
-148.822446806093,-148.714229065279,-148.606011324466),.UNSPECIFIED.);
#7895=B_SPLINE_CURVE_WITH_KNOTS('',3,(#86171,#86172,#86173,#86174,#86175,
#86176,#86177,#86178,#86179,#86180),.UNSPECIFIED.,.F.,.F.,(4,1,1,1,1,1,
1,4),(-148.606011105325,-147.928240501961,-146.928725363434,-145.929210224907,
-144.929695086381,-143.930179947854,-142.930664809327,-142.322825798145),
 .UNSPECIFIED.);
#7896=B_SPLINE_CURVE_WITH_KNOTS('',3,(#86182,#86183,#86184,#86185,#86186,
#86187,#86188,#86189,#86190,#86191),.UNSPECIFIED.,.F.,.F.,(4,1,1,1,1,1,
1,4),(-142.322825798145,-141.9311496708,-140.931634532274,-139.932119393747,
-138.93260425522,-137.933089116693,-136.933573978166,-136.039640490966),
 .UNSPECIFIED.);
#7897=B_SPLINE_CURVE_WITH_KNOTS('',3,(#86193,#86194,#86195,#86196,#86197,
#86198,#86199,#86200,#86201,#86202,#86203),.UNSPECIFIED.,.F.,.F.,(4,1,1,
1,1,1,1,1,4),(-136.039640490966,-135.93405883964,-134.934543701113,-133.935028562586,
-132.935513424059,-131.935998285533,-130.936483147006,-129.936968008479,
-129.756455183786),.UNSPECIFIED.);
#7898=B_SPLINE_CURVE_WITH_KNOTS('',3,(#86205,#86206,#86207,#86208,#86209,
#86210,#86211,#86212,#86213,#86214,#86215,#86216,#86217,#86218,#86219,#86220,
#86221,#86222,#86223,#86224,#86225,#86226,#86227,#86228,#86229,#86230,#86231,
#86232,#86233,#86234,#86235,#86236,#86237,#86238,#86239,#86240,#86241,#86242,
#86243,#86244,#86245,#86246,#86247,#86248,#86249,#86250,#86251,#86252,#86253,
#86254,#86255,#86256,#86257,#86258,#86259,#86260,#86261,#86262,#86263,#86264,
#86265,#86266,#86267,#86268,#86269,#86270,#86271,#86272,#86273,#86274,#86275,
#86276,#86277,#86278,#86279,#86280,#86281,#86282,#86283,#86284,#86285,#86286,
#86287,#86288,#86289,#86290,#86291,#86292,#86293,#86294,#86295,#86296,#86297,
#86298,#86299,#86300,#86301,#86302,#86303,#86304,#86305,#86306,#86307,#86308,
#86309,#86310,#86311,#86312,#86313,#86314,#86315,#86316,#86317,#86318,#86319,
#86320,#86321,#86322,#86323,#86324,#86325,#86326,#86327,#86328,#86329,#86330,
#86331,#86332,#86333,#86334,#86335,#86336,#86337,#86338,#86339,#86340,#86341,
#86342,#86343,#86344,#86345,#86346,#86347,#86348,#86349,#86350,#86351,#86352,
#86353,#86354,#86355,#86356,#86357,#86358,#86359,#86360,#86361,#86362,#86363,
#86364,#86365,#86366,#86367,#86368,#86369,#86370,#86371,#86372,#86373,#86374,
#86375,#86376,#86377,#86378,#86379,#86380,#86381,#86382,#86383,#86384,#86385,
#86386,#86387,#86388,#86389,#86390,#86391,#86392,#86393,#86394,#86395,#86396,
#86397,#86398,#86399,#86400,#86401,#86402,#86403,#86404,#86405,#86406,#86407,
#86408,#86409,#86410,#86411,#86412,#86413,#86414,#86415,#86416,#86417,#86418,
#86419,#86420,#86421,#86422,#86423,#86424,#86425,#86426,#86427,#86428,#86429,
#86430),.UNSPECIFIED.,.F.,.F.,(4,3,3,3,3,3,3,3,3,3,3,3,3,3,3,3,3,3,3,3,
3,3,3,3,3,3,3,3,3,3,3,3,3,3,3,3,3,3,3,3,3,3,3,3,3,3,3,3,3,3,3,3,3,3,3,3,
3,3,3,3,3,3,3,3,3,3,3,3,3,3,3,3,3,3,3,4),(-129.756455183786,-129.66935498244,
-129.577867218379,-129.490904202965,-129.403965797651,-129.317029494613,
-129.230072791103,-129.143023997227,-129.05592154166,-128.968690340322,
-128.937452869952,-128.848898468514,-128.760458780785,-128.672110005592,
-128.580338471322,-128.49209193675,-128.403858818535,-128.315617750497,
-128.227347365869,-128.138976635018,-128.050546383731,-127.961985913635,
-127.937937731426,-127.849383329988,-127.760943642259,-127.672594867066,
-127.580823332796,-127.492576798224,-127.404343680008,-127.31610261197,
-127.227832227342,-127.13946149649,-127.051031245203,-126.962470775107,
-126.938422592899,-126.849868191461,-126.761428503731,-126.673079728539,
-126.581308194268,-126.493061659696,-126.40482854148,-126.316587473442,
-126.228317088813,-126.139946357961,-126.051516106674,-125.962955636579,
-125.938907454372,-125.850353052934,-125.761913365205,-125.673564590012,
-125.581793055741,-125.493546521169,-125.405313402953,-125.317072334915,
-125.228801950287,-125.140431219435,-125.052000968148,-124.963440498052,
-124.939392315845,-124.850837914407,-124.762398226678,-124.674049451486,
-124.582277917215,-124.494031382643,-124.405798264428,-124.31755719639,
-124.229286811762,-124.14091608091,-124.052485829624,-123.963925359529,
-123.939877177319,-123.845254519537,-123.750922331933,-123.656763961693,
-123.562866404263,-123.473270057579),.UNSPECIFIED.);
#7899=B_SPLINE_CURVE_WITH_KNOTS('',3,(#86432,#86433,#86434,#86435,#86436,
#86437,#86438,#86439,#86440,#86441),.UNSPECIFIED.,.F.,.F.,(4,1,1,1,1,1,
1,4),(-123.473269876606,-122.940362038792,-121.940846900265,-120.941331761738,
-119.941816623212,-118.942301484685,-117.942786346158,-117.190084569427),
 .UNSPECIFIED.);
#7900=B_SPLINE_CURVE_WITH_KNOTS('',3,(#86443,#86444,#86445,#86446,#86447,
#86448,#86449,#86450,#86451,#86452,#86453,#86454,#86455,#86456,#86457,#86458,
#86459,#86460,#86461,#86462,#86463,#86464,#86465,#86466,#86467,#86468,#86469,
#86470,#86471,#86472,#86473,#86474,#86475,#86476,#86477,#86478,#86479,#86480,
#86481,#86482,#86483,#86484,#86485,#86486,#86487,#86488,#86489,#86490,#86491,
#86492,#86493,#86494,#86495,#86496,#86497,#86498,#86499,#86500,#86501,#86502,
#86503,#86504,#86505,#86506,#86507,#86508,#86509,#86510,#86511,#86512,#86513,
#86514,#86515,#86516,#86517,#86518,#86519,#86520,#86521,#86522,#86523,#86524,
#86525,#86526,#86527,#86528,#86529,#86530,#86531,#86532,#86533,#86534,#86535,
#86536,#86537,#86538,#86539,#86540,#86541,#86542,#86543,#86544,#86545,#86546,
#86547,#86548,#86549,#86550,#86551,#86552,#86553,#86554,#86555,#86556,#86557,
#86558,#86559,#86560,#86561,#86562,#86563,#86564,#86565,#86566,#86567,#86568,
#86569,#86570,#86571,#86572,#86573,#86574,#86575,#86576,#86577,#86578,#86579,
#86580,#86581,#86582,#86583,#86584,#86585,#86586,#86587,#86588,#86589,#86590,
#86591,#86592,#86593,#86594,#86595,#86596,#86597,#86598,#86599,#86600,#86601,
#86602,#86603,#86604,#86605,#86606,#86607,#86608,#86609,#86610,#86611,#86612,
#86613,#86614,#86615,#86616,#86617,#86618,#86619,#86620,#86621,#86622,#86623,
#86624,#86625,#86626,#86627,#86628,#86629,#86630,#86631,#86632,#86633,#86634,
#86635,#86636,#86637,#86638,#86639,#86640,#86641,#86642,#86643,#86644,#86645,
#86646,#86647,#86648,#86649,#86650,#86651,#86652,#86653,#86654,#86655,#86656,
#86657,#86658,#86659,#86660,#86661,#86662,#86663,#86664,#86665,#86666,#86667,
#86668,#86669,#86670,#86671),.UNSPECIFIED.,.F.,.F.,(4,3,3,3,3,3,3,3,3,3,
3,3,3,3,3,3,3,3,3,3,3,3,3,3,3,3,3,3,3,3,3,3,3,3,3,3,3,3,3,3,3,3,3,3,3,3,
3,3,3,3,3,3,3,3,3,3,3,3,3,3,3,3,3,3,3,3,3,3,3,3,3,3,3,3,3,3,4),(-117.190084482236,
-117.076148942948,-116.959487829622,-116.943271207631,-116.854716806193,
-116.766277118464,-116.677928343272,-116.586156809001,-116.497910274429,
-116.409677156214,-116.321436088176,-116.233165703548,-116.144794972696,
-116.05636472141,-115.967804251314,-115.943756069104,-115.855201667666,
-115.766761979937,-115.678413204744,-115.586641670474,-115.498395135902,
-115.410162017687,-115.321920949649,-115.233650565021,-115.145279834169,
-115.056849582883,-114.968289112787,-114.944240930578,-114.85568652914,
-114.767246841411,-114.678898066218,-114.587126531947,-114.498879997375,
-114.410646879159,-114.322405811121,-114.234135426493,-114.145764695641,
-114.057334444354,-113.968773974258,-113.944725792051,-113.856171390613,
-113.767731702883,-113.679382927691,-113.58761139342,-113.499364858848,
-113.411131740632,-113.322890672594,-113.234620287966,-113.146249557113,
-113.057819305827,-112.969258835731,-112.945210653524,-112.856656252086,
-112.768216564357,-112.679867789164,-112.588096254893,-112.499849720321,
-112.411616602105,-112.323375534067,-112.235105149439,-112.146734418587,
-112.0583041673,-111.969743697204,-111.945695514997,-111.857141113559,-111.76870142583,
-111.680352650638,-111.588581116367,-111.500334581795,-111.41210146358,
-111.323860395542,-111.235590010914,-111.147219280062,-111.058789028776,
-110.97022855868,-110.946180376471,-110.906899262247),.UNSPECIFIED.);
#7901=B_SPLINE_CURVE_WITH_KNOTS('',3,(#86673,#86674,#86675,#86676,#86677,
#86678,#86679,#86680,#86681,#86682),.UNSPECIFIED.,.F.,.F.,(4,1,1,1,1,1,
1,4),(-110.906894042246,-109.946665237944,-108.947150099417,-107.94763496089,
-106.948119822364,-105.948604683837,-104.94908954531,-104.623720933803),
 .UNSPECIFIED.);
#7902=B_SPLINE_CURVE_WITH_KNOTS('',3,(#86684,#86685,#86686,#86687,#86688,
#86689,#86690,#86691,#86692,#86693,#86694,#86695,#86696,#86697,#86698,#86699,
#86700,#86701,#86702,#86703,#86704,#86705,#86706,#86707,#86708,#86709,#86710,
#86711,#86712,#86713,#86714,#86715,#86716,#86717,#86718,#86719,#86720,#86721,
#86722,#86723,#86724,#86725,#86726,#86727,#86728,#86729,#86730,#86731,#86732,
#86733,#86734,#86735,#86736,#86737,#86738,#86739,#86740,#86741,#86742,#86743,
#86744,#86745,#86746,#86747,#86748,#86749,#86750,#86751,#86752,#86753,#86754,
#86755,#86756,#86757,#86758,#86759,#86760,#86761,#86762,#86763,#86764,#86765,
#86766,#86767,#86768,#86769,#86770,#86771,#86772,#86773,#86774,#86775,#86776,
#86777,#86778,#86779,#86780,#86781,#86782,#86783,#86784,#86785,#86786,#86787,
#86788,#86789,#86790,#86791,#86792,#86793,#86794,#86795,#86796,#86797,#86798,
#86799,#86800,#86801,#86802,#86803,#86804,#86805,#86806,#86807,#86808,#86809,
#86810,#86811,#86812,#86813,#86814,#86815,#86816,#86817,#86818,#86819,#86820,
#86821,#86822,#86823,#86824,#86825,#86826,#86827,#86828,#86829,#86830,#86831,
#86832,#86833,#86834,#86835,#86836,#86837,#86838,#86839,#86840,#86841,#86842,
#86843,#86844,#86845,#86846,#86847,#86848,#86849,#86850,#86851,#86852,#86853,
#86854,#86855,#86856,#86857,#86858,#86859,#86860,#86861,#86862,#86863,#86864,
#86865,#86866,#86867,#86868,#86869,#86870,#86871,#86872,#86873,#86874,#86875,
#86876,#86877,#86878,#86879,#86880,#86881,#86882,#86883,#86884,#86885,#86886,
#86887,#86888,#86889,#86890,#86891,#86892,#86893,#86894,#86895,#86896,#86897,
#86898,#86899,#86900,#86901,#86902,#86903,#86904,#86905,#86906,#86907,#86908,
#86909),.UNSPECIFIED.,.F.,.F.,(4,3,3,3,3,3,3,3,3,3,3,3,3,3,3,3,3,3,3,3,
3,3,3,3,3,3,3,3,3,3,3,3,3,3,3,3,3,3,3,3,3,3,3,3,3,3,3,3,3,3,3,3,3,3,3,3,
3,3,3,3,3,3,3,3,3,3,3,3,3,3,3,3,3,3,3,4),(-104.623713955068,-104.535644705966,
-104.447593713946,-104.359539482352,-104.271460517181,-104.183279470856,
-104.095042939218,-104.006661658045,-103.949574406783,-103.861020005345,
-103.772580317616,-103.684231542424,-103.592460008153,-103.504213473581,
-103.415980355366,-103.327739287328,-103.239468902701,-103.151098171849,
-103.062667920562,-102.974107450467,-102.950059268257,-102.861504866819,
-102.77306517909,-102.684716403897,-102.592944869626,-102.504698335054,
-102.416465216839,-102.3282241488,-102.239953764172,-102.15158303332,-102.063152782034,
-101.974592311938,-101.95054412973,-101.861989728292,-101.773550040562,
-101.685201265369,-101.593429731098,-101.505183196526,-101.41695007831,
-101.328709010272,-101.240438625644,-101.152067894791,-101.063637643504,
-100.975077173408,-100.951028991203,-100.862474589765,-100.774034902036,
-100.685686126843,-100.593914592572,-100.505668058,-100.417434939784,-100.329193871746,
-100.240923487118,-100.152552756266,-100.064122504979,-99.9755620348834,
-99.9515138526763,-99.8629594512383,-99.774519763509,-99.686170988316,-99.5943994540452,
-99.5061529194733,-99.4179198012576,-99.3296787332196,-99.241408348592,
-99.15303761774,-99.0646073664534,-98.9760468963575,-98.9519987141495,-98.862422794307,
-98.7729691408607,-98.6836176547323,-98.5943606830314,-98.5051598633551,
-98.4159876281948,-98.3405286478881),.UNSPECIFIED.);
#7903=B_SPLINE_CURVE_WITH_KNOTS('',3,(#86911,#86912,#86913,#86914,#86915,
#86916,#86917,#86918,#86919,#86920),.UNSPECIFIED.,.F.,.F.,(4,1,1,1,1,1,
1,4),(-98.3405213020582,-97.9524835756228,-96.952968437096,-95.9534532985692,
-94.9539381600425,-93.9544230215157,-92.9549078829889,-92.057352313836),
 .UNSPECIFIED.);
#7904=B_SPLINE_CURVE_WITH_KNOTS('',3,(#86922,#86923,#86924,#86925,#86926,
#86927,#86928,#86929,#86930,#86931,#86932,#86933,#86934,#86935,#86936,#86937,
#86938,#86939,#86940,#86941,#86942,#86943,#86944,#86945,#86946,#86947,#86948,
#86949,#86950,#86951,#86952,#86953,#86954,#86955,#86956,#86957,#86958,#86959,
#86960,#86961,#86962,#86963,#86964,#86965,#86966,#86967,#86968,#86969,#86970,
#86971,#86972,#86973,#86974,#86975,#86976,#86977,#86978,#86979,#86980,#86981,
#86982,#86983,#86984,#86985,#86986,#86987,#86988,#86989,#86990,#86991,#86992,
#86993,#86994,#86995,#86996,#86997,#86998,#86999,#87000,#87001,#87002,#87003,
#87004,#87005,#87006,#87007,#87008,#87009,#87010,#87011,#87012,#87013,#87014,
#87015,#87016,#87017,#87018,#87019,#87020,#87021,#87022,#87023,#87024,#87025,
#87026,#87027,#87028,#87029,#87030,#87031,#87032,#87033,#87034,#87035,#87036,
#87037,#87038,#87039,#87040,#87041,#87042,#87043,#87044,#87045,#87046,#87047,
#87048,#87049,#87050,#87051,#87052,#87053,#87054,#87055,#87056,#87057,#87058,
#87059,#87060,#87061,#87062,#87063,#87064,#87065,#87066,#87067,#87068,#87069,
#87070,#87071,#87072,#87073,#87074,#87075,#87076,#87077,#87078,#87079,#87080,
#87081,#87082,#87083,#87084,#87085,#87086,#87087,#87088,#87089,#87090,#87091,
#87092,#87093,#87094,#87095,#87096,#87097,#87098,#87099,#87100,#87101,#87102,
#87103,#87104,#87105,#87106,#87107,#87108,#87109,#87110,#87111,#87112,#87113,
#87114,#87115,#87116,#87117,#87118,#87119,#87120,#87121,#87122,#87123,#87124,
#87125,#87126,#87127,#87128,#87129,#87130,#87131,#87132,#87133,#87134,#87135,
#87136,#87137,#87138,#87139,#87140,#87141,#87142,#87143,#87144,#87145,#87146,
#87147),.UNSPECIFIED.,.F.,.F.,(4,3,3,3,3,3,3,3,3,3,3,3,3,3,3,3,3,3,3,3,
3,3,3,3,3,3,3,3,3,3,3,3,3,3,3,3,3,3,3,3,3,3,3,3,3,3,3,3,3,3,3,3,3,3,3,3,
3,3,3,3,3,3,3,3,3,3,3,3,3,3,3,3,3,3,3,4),(-92.0573433407085,-91.9553927444622,
-91.8668383430241,-91.7783986552946,-91.6900498801017,-91.5982783458309,
-91.5100318112589,-91.421798693043,-91.3335576250045,-91.2452872403763,
-91.1569165095242,-91.0684862582373,-90.9799257881413,-90.9558776059354,
-90.8673232044974,-90.7788835167681,-90.6905347415753,-90.5987632073045,
-90.5105166727327,-90.422283554517,-90.3340424864788,-90.2457721018508,
-90.1574013709988,-90.0689711197121,-89.9804106496163,-89.9563624674086,
-89.8678080659707,-89.7793683782414,-89.6910196030486,-89.5992480687778,
-89.5110015342059,-89.4227684159903,-89.3345273479521,-89.2462569633242,
-89.1578862324723,-89.0694559811856,-88.9808955110898,-88.9568473288819,
-88.8682929274439,-88.7798532397146,-88.6915044645217,-88.5997329302509,
-88.511486395679,-88.4232532774634,-88.3350122094251,-88.2467418247971,
-88.1583710939451,-88.0699408426584,-87.9813803725626,-87.9573321903551,
-87.8687777889171,-87.7803381011878,-87.6919893259951,-87.6002177917242,
-87.5119712571524,-87.4237381389367,-87.3354970708985,-87.2472266862704,
-87.1588559554184,-87.0704257041317,-86.9818652340359,-86.9578170518284,
-86.8692626503904,-86.780822962661,-86.6924741874681,-86.6007026531973,
-86.5124561186254,-86.4242230004098,-86.3359819323716,-86.2477115477435,
-86.1593408168916,-86.0709105656049,-85.9823500955091,-85.9583019133016,
-85.8255508273588,-85.7741580335289),.UNSPECIFIED.);
#7905=B_SPLINE_CURVE_WITH_KNOTS('',3,(#87149,#87150,#87151,#87152,#87153,
#87154,#87155,#87156,#87157,#87158),.UNSPECIFIED.,.F.,.F.,(4,1,1,1,1,1,
1,4),(-85.7741532391098,-84.9587867747748,-83.9592716362481,-82.9597564977213,
-81.9602413591946,-80.9607262206678,-79.961211082141,-79.4909727263493),
 .UNSPECIFIED.);
#7906=B_SPLINE_CURVE_WITH_KNOTS('',3,(#87160,#87161,#87162,#87163,#87164,
#87165,#87166,#87167,#87168,#87169),.UNSPECIFIED.,.F.,.F.,(4,1,1,1,1,1,
1,4),(-79.4909727263493,-78.9616959436142,-77.9621808050875,-76.9626656665607,
-75.963150528034,-74.9636353895072,-73.9641202509805,-73.2077874191697),
 .UNSPECIFIED.);
#7907=B_SPLINE_CURVE_WITH_KNOTS('',3,(#87171,#87172,#87173,#87174,#87175,
#87176,#87177,#87178,#87179,#87180,#87181,#87182,#87183,#87184,#87185,#87186,
#87187,#87188,#87189,#87190,#87191,#87192,#87193,#87194,#87195,#87196,#87197,
#87198,#87199,#87200,#87201,#87202,#87203,#87204,#87205,#87206,#87207,#87208,
#87209,#87210,#87211,#87212,#87213,#87214,#87215,#87216,#87217,#87218,#87219,
#87220,#87221,#87222,#87223,#87224,#87225,#87226,#87227,#87228,#87229,#87230,
#87231,#87232,#87233,#87234,#87235,#87236,#87237,#87238,#87239,#87240,#87241,
#87242,#87243,#87244,#87245,#87246,#87247,#87248,#87249,#87250,#87251,#87252,
#87253,#87254,#87255,#87256,#87257,#87258,#87259,#87260,#87261,#87262,#87263,
#87264,#87265,#87266,#87267,#87268,#87269,#87270,#87271,#87272,#87273,#87274,
#87275,#87276,#87277,#87278,#87279,#87280,#87281,#87282,#87283,#87284,#87285,
#87286,#87287,#87288,#87289,#87290,#87291,#87292,#87293,#87294,#87295,#87296,
#87297,#87298,#87299,#87300,#87301,#87302,#87303,#87304,#87305,#87306,#87307,
#87308,#87309,#87310,#87311,#87312,#87313,#87314,#87315,#87316,#87317,#87318,
#87319,#87320,#87321,#87322,#87323,#87324,#87325,#87326,#87327,#87328,#87329,
#87330,#87331,#87332,#87333,#87334,#87335,#87336,#87337,#87338,#87339,#87340,
#87341,#87342,#87343,#87344,#87345,#87346,#87347,#87348,#87349,#87350,#87351,
#87352,#87353,#87354,#87355,#87356,#87357,#87358,#87359,#87360,#87361,#87362,
#87363,#87364,#87365,#87366,#87367,#87368,#87369,#87370,#87371,#87372,#87373,
#87374,#87375,#87376,#87377,#87378,#87379,#87380,#87381,#87382,#87383,#87384,
#87385,#87386,#87387,#87388,#87389,#87390,#87391,#87392,#87393,#87394,#87395,
#87396,#87397,#87398,#87399),.UNSPECIFIED.,.F.,.F.,(4,3,3,3,3,3,3,3,3,3,
3,3,3,3,3,3,3,3,3,3,3,3,3,3,3,3,3,3,3,3,3,3,3,3,3,3,3,3,3,3,3,3,3,3,3,3,
3,3,3,3,3,3,3,3,3,3,3,3,3,3,3,3,3,3,3,3,3,3,3,3,3,3,3,3,3,3,4),(-73.2077873547606,
-73.0932049597969,-72.9757514791561,-72.9646051124537,-72.8760507110156,
-72.7876110232862,-72.6992622480933,-72.6074907138225,-72.5192441792505,
-72.4310110610349,-72.3427699929966,-72.2544996083684,-72.1661288775164,
-72.0776986262297,-71.9891381561337,-71.9650899739269,-71.8765355724889,
-71.7880958847597,-71.6997471095669,-71.6079755752961,-71.5197290407243,
-71.4314959225087,-71.3432548544705,-71.2549844698426,-71.1666137389907,
-71.0781834877041,-70.9896230176082,-70.9655748354002,-70.8770204339622,
-70.7885807462329,-70.7002319710401,-70.6084604367693,-70.5202139021974,
-70.4319807839818,-70.3437397159435,-70.2554693313156,-70.1670986004636,
-70.0786683491769,-69.9901078790811,-69.9660596968734,-69.8775052954354,
-69.789065607706,-69.7007168325132,-69.6089452982423,-69.5206987636705,
-69.4324656454548,-69.3442245774165,-69.2559541927885,-69.1675834619365,
-69.0791532106498,-68.9905927405539,-68.9665445583466,-68.8779901569086,
-68.7895504691793,-68.7012016939865,-68.6094301597157,-68.5211836251439,
-68.4329505069282,-68.34470943889,-68.256439054262,-68.16806832341,-68.0796380721234,
-67.9910776020276,-67.9670294198199,-67.8784750183819,-67.7900353306526,
-67.7016865554598,-67.609915021189,-67.5216684866171,-67.4334353684015,
-67.3451943003633,-67.2569239157355,-67.1685531848836,-67.080122933597,
-66.9915624635012,-66.9675142812931,-66.9246021119901),.UNSPECIFIED.);
#7908=B_SPLINE_CURVE_WITH_KNOTS('',3,(#87401,#87402,#87403,#87404,#87405,
#87406,#87407,#87408,#87409,#87410),.UNSPECIFIED.,.F.,.F.,(4,1,1,1,1,1,
1,4),(-66.9245965145714,-65.9679991427663,-64.9684840042396,-63.9689688657128,
-62.9694537271861,-61.9699385886593,-60.9704234501325,-60.6414239154789),
 .UNSPECIFIED.);
#7909=B_SPLINE_CURVE_WITH_KNOTS('',3,(#87412,#87413,#87414,#87415,#87416,
#87417,#87418,#87419,#87420,#87421,#87422,#87423,#87424,#87425,#87426,#87427,
#87428,#87429,#87430,#87431,#87432,#87433,#87434,#87435,#87436,#87437,#87438,
#87439,#87440,#87441,#87442,#87443,#87444,#87445,#87446,#87447,#87448,#87449,
#87450,#87451,#87452,#87453,#87454,#87455,#87456,#87457,#87458,#87459,#87460,
#87461,#87462,#87463,#87464,#87465,#87466,#87467,#87468,#87469,#87470,#87471,
#87472,#87473,#87474,#87475,#87476,#87477,#87478,#87479,#87480,#87481,#87482,
#87483,#87484,#87485,#87486,#87487,#87488,#87489,#87490,#87491,#87492,#87493,
#87494,#87495,#87496,#87497,#87498,#87499,#87500,#87501,#87502,#87503,#87504,
#87505,#87506,#87507,#87508,#87509,#87510,#87511,#87512,#87513,#87514,#87515,
#87516,#87517,#87518,#87519,#87520,#87521,#87522,#87523,#87524,#87525,#87526,
#87527,#87528,#87529,#87530,#87531,#87532,#87533,#87534,#87535,#87536,#87537,
#87538,#87539,#87540,#87541,#87542,#87543,#87544,#87545,#87546,#87547,#87548,
#87549,#87550,#87551,#87552,#87553,#87554,#87555,#87556,#87557,#87558,#87559,
#87560,#87561,#87562,#87563,#87564,#87565,#87566,#87567,#87568,#87569,#87570,
#87571,#87572,#87573,#87574,#87575,#87576,#87577,#87578,#87579,#87580,#87581,
#87582,#87583,#87584,#87585,#87586,#87587,#87588,#87589,#87590,#87591,#87592,
#87593,#87594,#87595,#87596,#87597,#87598,#87599,#87600,#87601,#87602,#87603,
#87604,#87605,#87606,#87607,#87608,#87609,#87610,#87611,#87612,#87613,#87614,
#87615,#87616,#87617,#87618,#87619,#87620,#87621,#87622,#87623,#87624,#87625,
#87626,#87627,#87628,#87629,#87630,#87631,#87632,#87633,#87634,#87635,#87636,
#87637),.UNSPECIFIED.,.F.,.F.,(4,3,3,3,3,3,3,3,3,3,3,3,3,3,3,3,3,3,3,3,
3,3,3,3,3,3,3,3,3,3,3,3,3,3,3,3,3,3,3,3,3,3,3,3,3,3,3,3,3,3,3,3,3,3,3,3,
3,3,3,3,3,3,3,3,3,3,3,3,3,3,3,3,3,3,3,4),(-60.6414168048105,-60.553296060957,
-60.4651918097365,-60.3770826180884,-60.2889470544044,-60.2007081252582,
-60.1124123690869,-60.0239725402644,-59.9709083116058,-59.8823539101678,
-59.7939142224383,-59.7055654472453,-59.6137939129745,-59.5255473784026,
-59.4373142601871,-59.3490731921489,-59.2608028075208,-59.1724320766688,
-59.0840018253821,-58.9954413552862,-58.971393173079,-58.882838771641,-58.7943990839117,
-58.7060503087186,-58.6142787744478,-58.526032239876,-58.4377991216604,
-58.3495580536221,-58.2612876689941,-58.1729169381422,-58.0844866868554,
-57.9959262167595,-57.9718780345522,-57.8833236331142,-57.7948839453851,
-57.7065351701922,-57.6147636359213,-57.5265171013496,-57.4382839831339,
-57.3500429150957,-57.2617725304679,-57.173401799616,-57.0849715483293,
-56.9964110782334,-56.9723628960255,-56.8838084945875,-56.795368806858,
-56.707020031665,-56.6152484973942,-56.5270019628223,-56.4387688446066,
-56.3505277765684,-56.2622573919405,-56.1738866610886,-56.0854564098019,
-55.9968959397059,-55.9728477574987,-55.8842933560608,-55.7958536683313,
-55.7075048931387,-55.6157333588678,-55.527486824296,-55.4392537060804,
-55.3510126380422,-55.2627422534145,-55.1743715225625,-55.0859412712757,
-54.99738080118,-54.973332618972,-54.8838398296381,-54.7944684518599,-54.7051982540858,
-54.6160204771488,-54.5268978074483,-54.4378006945073,-54.3582314976309),
 .UNSPECIFIED.);
#7910=B_SPLINE_CURVE_WITH_KNOTS('',3,(#87639,#87640,#87641,#87642,#87643,
#87644,#87645,#87646,#87647,#87648),.UNSPECIFIED.,.F.,.F.,(4,1,1,1,1,1,
1,4),(-54.3582240635315,-53.9738174804452,-52.9743023419184,-51.9747872033917,
-50.9752720648649,-49.9757569263381,-48.9762417878114,-48.075055138789),
 .UNSPECIFIED.);
#7911=B_SPLINE_CURVE_WITH_KNOTS('',3,(#87650,#87651,#87652,#87653,#87654,
#87655,#87656,#87657,#87658,#87659,#87660,#87661,#87662,#87663,#87664,#87665,
#87666,#87667,#87668,#87669,#87670,#87671,#87672,#87673,#87674,#87675,#87676,
#87677,#87678,#87679,#87680,#87681,#87682,#87683,#87684,#87685,#87686,#87687,
#87688,#87689,#87690,#87691,#87692,#87693,#87694,#87695,#87696,#87697,#87698,
#87699,#87700,#87701,#87702,#87703,#87704,#87705,#87706,#87707,#87708,#87709,
#87710,#87711,#87712,#87713,#87714,#87715,#87716,#87717,#87718,#87719,#87720,
#87721,#87722,#87723,#87724,#87725,#87726,#87727,#87728,#87729,#87730,#87731,
#87732,#87733,#87734,#87735,#87736,#87737,#87738,#87739,#87740,#87741,#87742,
#87743,#87744,#87745,#87746,#87747,#87748,#87749,#87750,#87751,#87752,#87753,
#87754,#87755,#87756,#87757,#87758,#87759,#87760,#87761,#87762,#87763,#87764,
#87765,#87766,#87767,#87768,#87769,#87770,#87771,#87772,#87773,#87774,#87775,
#87776,#87777,#87778,#87779,#87780,#87781,#87782,#87783,#87784,#87785,#87786,
#87787,#87788,#87789,#87790,#87791,#87792,#87793,#87794,#87795,#87796,#87797,
#87798,#87799,#87800,#87801,#87802,#87803,#87804,#87805,#87806,#87807,#87808,
#87809,#87810,#87811,#87812,#87813,#87814,#87815,#87816,#87817,#87818,#87819,
#87820,#87821,#87822,#87823,#87824,#87825,#87826,#87827,#87828,#87829,#87830,
#87831,#87832,#87833,#87834,#87835,#87836,#87837,#87838,#87839,#87840,#87841,
#87842,#87843,#87844,#87845,#87846,#87847,#87848,#87849,#87850,#87851,#87852,
#87853,#87854,#87855,#87856,#87857,#87858,#87859,#87860,#87861,#87862,#87863,
#87864,#87865,#87866,#87867,#87868,#87869,#87870,#87871,#87872,#87873,#87874,
#87875),.UNSPECIFIED.,.F.,.F.,(4,3,3,3,3,3,3,3,3,3,3,3,3,3,3,3,3,3,3,3,
3,3,3,3,3,3,3,3,3,3,3,3,3,3,3,3,3,3,3,3,3,3,3,3,3,3,3,3,3,3,3,3,3,3,3,3,
3,3,3,3,3,3,3,3,3,3,3,3,3,3,3,3,3,3,3,4),(-48.0750461904513,-47.9767266492846,
-47.8881722478465,-47.7997325601169,-47.7113837849239,-47.6196122506532,
-47.5313657160812,-47.4431325978654,-47.3548915298271,-47.266621145199,
-47.1782504143468,-47.08982016306,-47.001259692964,-46.9772115107578,-46.8886571093199,
-46.8002174215906,-46.7118686463979,-46.620097112127,-46.5318505775552,
-46.4436174593396,-46.3553763913014,-46.2671060066735,-46.1787352758216,
-46.090305024535,-46.0017445544392,-45.9776963722311,-45.8891419707931,
-45.8007022830638,-45.712353507871,-45.6205819736002,-45.5323354390283,
-45.4441023208127,-45.3558612527744,-45.2675908681464,-45.1792201372944,
-45.0907898860077,-45.0022294159119,-44.9781812337043,-44.8896268322663,
-44.801187144537,-44.7128383693442,-44.6210668350733,-44.5328203005015,
-44.4445871822858,-44.3563461142475,-44.2680757296195,-44.1797049987675,
-44.0912747474808,-44.002714277385,-43.9786660951776,-43.8901116937396,
-43.8016720060103,-43.7133232308176,-43.6215516965467,-43.5333051619749,
-43.4450720437592,-43.3568309757211,-43.2685605910932,-43.1801898602412,
-43.0917596089546,-43.0031991388587,-42.9791509566508,-42.8905965552128,
-42.8021568674835,-42.7138080922906,-42.6220365580198,-42.533790023448,
-42.4455569052323,-42.357315837194,-42.2690454525658,-42.1806747217138,
-42.0922444704272,-42.0036840003312,-41.979635818124,-41.8482965029249,
-41.7918608832718),.UNSPECIFIED.);
#7912=B_SPLINE_CURVE_WITH_KNOTS('',3,(#87877,#87878,#87879,#87880,#87881,
#87882,#87883,#87884,#87885,#87886),.UNSPECIFIED.,.F.,.F.,(4,1,1,1,1,1,
1,4),(-41.7918564217168,-40.9801206795973,-39.9806055410705,-38.9810904025437,
-37.981575264017,-36.9820601254902,-35.9825449869635,-35.5086755760922),
 .UNSPECIFIED.);
#7913=B_SPLINE_CURVE_WITH_KNOTS('',3,(#87888,#87889,#87890,#87891,#87892,
#87893,#87894,#87895,#87896,#87897),.UNSPECIFIED.,.F.,.F.,(4,1,1,1,1,1,
1,4),(-35.5086755760922,-34.9830298484367,-33.9835147099099,-32.9839995713832,
-31.9844844328564,-30.9849692943296,-29.9854541558029,-29.2254902689126),
 .UNSPECIFIED.);
#7914=B_SPLINE_CURVE_WITH_KNOTS('',3,(#87899,#87900,#87901,#87902,#87903,
#87904,#87905,#87906,#87907,#87908,#87909,#87910,#87911,#87912,#87913,#87914,
#87915,#87916,#87917,#87918,#87919,#87920,#87921,#87922,#87923,#87924,#87925,
#87926,#87927,#87928,#87929,#87930,#87931,#87932,#87933,#87934,#87935,#87936,
#87937,#87938,#87939,#87940,#87941,#87942,#87943,#87944,#87945,#87946,#87947,
#87948,#87949,#87950,#87951,#87952,#87953,#87954,#87955,#87956,#87957,#87958,
#87959,#87960,#87961,#87962,#87963,#87964,#87965,#87966,#87967,#87968,#87969,
#87970,#87971,#87972,#87973,#87974,#87975,#87976,#87977,#87978,#87979,#87980,
#87981,#87982,#87983,#87984,#87985,#87986,#87987,#87988,#87989,#87990,#87991,
#87992,#87993,#87994,#87995,#87996,#87997,#87998,#87999,#88000,#88001,#88002,
#88003,#88004,#88005,#88006,#88007,#88008,#88009,#88010,#88011,#88012,#88013,
#88014,#88015,#88016,#88017,#88018,#88019,#88020,#88021,#88022,#88023,#88024,
#88025,#88026,#88027,#88028,#88029,#88030,#88031,#88032,#88033,#88034,#88035,
#88036,#88037,#88038,#88039,#88040,#88041,#88042,#88043,#88044,#88045,#88046,
#88047,#88048,#88049,#88050,#88051,#88052,#88053,#88054,#88055,#88056,#88057,
#88058,#88059,#88060,#88061,#88062,#88063,#88064,#88065,#88066,#88067,#88068,
#88069,#88070,#88071,#88072,#88073,#88074,#88075,#88076,#88077,#88078,#88079,
#88080,#88081,#88082,#88083,#88084,#88085,#88086,#88087,#88088,#88089,#88090,
#88091,#88092,#88093,#88094,#88095,#88096,#88097,#88098,#88099,#88100,#88101,
#88102,#88103,#88104,#88105,#88106,#88107,#88108,#88109,#88110,#88111,#88112,
#88113,#88114,#88115,#88116,#88117,#88118,#88119,#88120,#88121,#88122,#88123,
#88124),.UNSPECIFIED.,.F.,.F.,(4,3,3,3,3,3,3,3,3,3,3,3,3,3,3,3,3,3,3,3,
3,3,3,3,3,3,3,3,3,3,3,3,3,3,3,3,3,3,3,3,3,3,3,3,3,3,3,3,3,3,3,3,3,3,3,3,
3,3,3,3,3,3,3,3,3,3,3,3,3,3,3,3,3,3,3,4),(-29.2254902272523,-29.1057146222642,
-28.9859390172761,-28.8973846158514,-28.8089449281353,-28.7205961529556,
-28.6288246186798,-28.5405780841208,-28.4523449659179,-28.3641038978923,
-28.2758335132768,-28.187462782437,-28.0990325311624,-28.0104720610784,
-27.9864238787494,-27.8978694773265,-27.8094297896124,-27.7210810144349,
-27.6293094801583,-27.5410629456021,-27.4528298274022,-27.3645887593798,
-27.2763183747675,-27.1879476439314,-27.0995173926606,-27.0109569225804,
-26.9869087402226,-26.8983543387054,-26.8099146508967,-26.7215658756244,
-26.6297943413833,-26.5415478067323,-26.4533146884377,-26.3650736203208,
-26.2768032356146,-26.1884325046853,-26.1000022533219,-26.0114417831506,
-25.9873936016958,-25.8988392003665,-25.8103995127456,-25.7220507376609,
-25.6302792033494,-25.542032668884,-25.453799550774,-25.3655584828405,-25.2772880983163,
-25.1889173675661,-25.1004871163802,-25.0119266463829,-24.9878784631691,
-24.899324061796,-24.8108843741328,-24.7225355990072,-24.6307640647116,
-24.5425175302093,-24.4542844120639,-24.3660433440966,-24.2777729595402,
-24.1894022287601,-24.1009719775459,-24.0124115075223,-23.9883633246423,
-23.8998089226723,-23.8113692344095,-23.7230204586822,-23.6312489246113,
-23.5430023895063,-23.4547692707586,-23.3665282021903,-23.2782578170346,
-23.1898870856612,-23.1014568338562,-23.0128963632503,-22.9888481861155,
-22.942304961733),.UNSPECIFIED.);
#7915=B_SPLINE_CURVE_WITH_KNOTS('',3,(#88126,#88127,#88128,#88129,#88130,
#88131,#88132,#88133,#88134,#88135),.UNSPECIFIED.,.F.,.F.,(4,1,1,1,1,1,
1,4),(-22.9422988168085,-21.9893330475888,-20.989817909062,-19.9903027705353,
-18.9907876320085,-17.9912724934817,-16.991757354955,-16.6591268838038),
 .UNSPECIFIED.);
#7916=B_SPLINE_CURVE_WITH_KNOTS('',3,(#88137,#88138,#88139,#88140,#88141,
#88142,#88143,#88144,#88145,#88146,#88147,#88148,#88149,#88150,#88151,#88152,
#88153,#88154,#88155,#88156,#88157,#88158,#88159,#88160,#88161,#88162,#88163,
#88164,#88165,#88166,#88167,#88168,#88169,#88170,#88171,#88172,#88173,#88174,
#88175,#88176,#88177,#88178,#88179,#88180,#88181,#88182,#88183,#88184,#88185,
#88186,#88187,#88188,#88189,#88190,#88191,#88192,#88193,#88194,#88195,#88196,
#88197,#88198,#88199,#88200,#88201,#88202,#88203,#88204,#88205,#88206,#88207,
#88208,#88209,#88210,#88211,#88212,#88213,#88214,#88215,#88216,#88217,#88218,
#88219,#88220,#88221,#88222,#88223,#88224,#88225,#88226,#88227,#88228,#88229,
#88230,#88231,#88232,#88233,#88234,#88235,#88236,#88237,#88238,#88239,#88240,
#88241,#88242,#88243,#88244,#88245,#88246,#88247,#88248,#88249,#88250,#88251,
#88252,#88253,#88254,#88255,#88256,#88257,#88258,#88259,#88260,#88261,#88262,
#88263,#88264,#88265,#88266,#88267,#88268,#88269,#88270,#88271,#88272,#88273,
#88274,#88275,#88276,#88277,#88278,#88279,#88280,#88281,#88282,#88283,#88284,
#88285,#88286,#88287,#88288,#88289,#88290,#88291,#88292,#88293,#88294,#88295,
#88296,#88297,#88298,#88299,#88300,#88301,#88302,#88303,#88304,#88305,#88306,
#88307,#88308,#88309,#88310,#88311,#88312,#88313,#88314,#88315,#88316,#88317,
#88318,#88319,#88320,#88321,#88322,#88323,#88324,#88325,#88326,#88327,#88328,
#88329,#88330,#88331,#88332,#88333,#88334,#88335,#88336,#88337,#88338,#88339,
#88340,#88341,#88342,#88343,#88344,#88345,#88346,#88347,#88348,#88349,#88350,
#88351,#88352,#88353,#88354,#88355,#88356,#88357,#88358,#88359,#88360,#88361,
#88362),.UNSPECIFIED.,.F.,.F.,(4,3,3,3,3,3,3,3,3,3,3,3,3,3,3,3,3,3,3,3,
3,3,3,3,3,3,3,3,3,3,3,3,3,3,3,3,3,3,3,3,3,3,3,3,3,3,3,3,3,3,3,3,3,3,3,3,
3,3,3,3,3,3,3,3,3,3,3,3,3,3,3,3,3,3,3,4),(-16.6591196545534,-16.5709460304396,
-16.4827871038465,-16.3946215082956,-16.3064278775447,-16.2181295773855,
-16.1297730926494,-16.0412731937529,-15.9922422164282,-15.9036877940136,
-15.8152480856589,-15.7268992902101,-15.6351277636715,-15.5468812098802,
-15.4586480728573,-15.3704069864418,-15.2821365838848,-15.1937658358538,
-15.1053355678029,-15.0167750816777,-14.9927270779014,-14.9041725382909,
-14.8157327116674,-14.7273837970277,-14.6356123148211,-14.5473656403005,
-14.4591323821879,-14.3708911744529,-14.2826206504764,-14.1942497814962,
-14.1058193926208,-14.0172587867959,-13.9932119393747,-13.9046579005256,
-13.8162185755933,-13.7278701629882,-13.6360984927206,-13.5478523179822,
-13.4596195579839,-13.3713788461756,-13.2831088154164,-13.1947384331657,
-13.1063085278465,-13.0177483971823,-12.9936968008479,-12.9051421549328,
-12.8167022249362,-12.7283532099315,-12.6365817664802,-12.548334999631,
-12.4601016522911,-12.3718603585081,-12.2835897517449,-12.195218805191,
-12.106788341677,-12.0182276660702,-11.9941816623212,-11.90562643978,-11.8171859256139,
-11.7288363196698,-11.6370650951853,-11.5488177243544,-11.4605837692713,
-11.3723418646475,-11.284070644607,-11.195699084313,-11.107268006035,-11.0187067189732,
-10.9946665237944,-10.9052576557781,-10.815969374525,-10.7267813186863,
-10.6376836161944,-10.5486400098947,-10.4596189026895,-10.3759343473738),
 .UNSPECIFIED.);
#7917=B_SPLINE_CURVE_WITH_KNOTS('',3,(#88363,#88364,#88365,#88366,#88367,
#88368,#88369,#88370,#88371,#88372),.UNSPECIFIED.,.F.,.F.,(4,1,1,1,1,1,
1,4),(-10.375926835712,-9.99515138526762,-8.99563624674086,-7.9961211082141,
-6.99660596968734,-5.99709083116058,-4.99757569263381,-4.09275795343756),
 .UNSPECIFIED.);
#7918=B_SPLINE_CURVE_WITH_KNOTS('',3,(#88375,#88376,#88377,#88378,#88379,
#88380),.UNSPECIFIED.,.F.,.F.,(4,1,1,4),(252.308677356644,252.498362612705,
253.497877751232,254.469000888742),.UNSPECIFIED.);
#7919=B_SPLINE_CURVE_WITH_KNOTS('',3,(#88382,#88383,#88384,#88385,#88386,
#88387,#88388,#88389,#88390,#88391,#88392,#88393,#88394,#88395,#88396,#88397,
#88398,#88399,#88400,#88401,#88402,#88403,#88404,#88405,#88406,#88407,#88408,
#88409,#88410,#88411,#88412,#88413,#88414,#88415,#88416,#88417,#88418,#88419,
#88420,#88421,#88422,#88423,#88424,#88425,#88426,#88427,#88428,#88429,#88430,
#88431,#88432,#88433,#88434,#88435,#88436,#88437,#88438,#88439,#88440,#88441,
#88442,#88443,#88444,#88445,#88446,#88447,#88448,#88449,#88450,#88451),
 .UNSPECIFIED.,.F.,.F.,(4,3,3,3,3,3,3,3,3,3,3,3,3,3,3,3,3,3,3,3,3,3,3,4),
(254.469004940773,254.497392889758,254.590649119483,254.68377880781,254.77680936004,
254.869770298601,254.962694927233,255.055607864379,255.148533712202,255.241555262876,
255.334626953852,255.427849487097,255.496908028285,255.589205413268,255.681379450479,
255.775485081436,255.867500738229,255.959486608717,256.051468320863,256.147157365181,
256.239259819415,256.331422968314,256.423718068013,256.434224498135),
 .UNSPECIFIED.);
#7920=B_SPLINE_CURVE_WITH_KNOTS('',3,(#88455,#88456,#88457,#88458,#88459,
#88460,#88461,#88462,#88463,#88464,#88465,#88466,#88467,#88468,#88469,#88470,
#88471,#88472,#88473,#88474,#88475,#88476,#88477,#88478,#88479,#88480,#88481,
#88482,#88483,#88484),.UNSPECIFIED.,.F.,.F.,(4,2,2,2,2,2,2,2,2,2,2,2,2,
2,4),(8.65291084783846E-5,0.077874969031854,0.0827087440970379,0.0857834642134888,
0.0886858313289599,0.0910799432465732,0.0938706143043208,0.0986813974108899,
0.117540885301815,0.170467162182005,0.225402500043114,0.23121802579301,
0.233440203541218,0.234288768021479,0.235068244192406),.UNSPECIFIED.);
#7921=B_SPLINE_CURVE_WITH_KNOTS('',3,(#88485,#88486,#88487,#88488,#88489,
#88490,#88491,#88492,#88493,#88494,#88495,#88496,#88497,#88498,#88499,#88500,
#88501,#88502,#88503,#88504,#88505,#88506,#88507,#88508,#88509,#88510,#88511,
#88512,#88513,#88514,#88515,#88516,#88517,#88518,#88519,#88520,#88521,#88522,
#88523,#88524,#88525,#88526,#88527,#88528,#88529,#88530,#88531,#88532,#88533,
#88534,#88535,#88536,#88537,#88538,#88539,#88540,#88541,#88542,#88543,#88544,
#88545,#88546,#88547,#88548,#88549,#88550,#88551,#88552,#88553,#88554,#88555,
#88556,#88557),.UNSPECIFIED.,.F.,.F.,(4,3,3,3,3,3,3,3,3,3,3,3,3,3,3,3,3,
3,3,3,3,3,3,3,4),(252.310073042627,252.403124865208,252.496086135635,252.588989817175,
252.681865086057,252.77473659135,252.867628972223,252.960624120039,253.053676529113,
253.146877714681,253.195941688915,253.288011824282,253.379955289568,253.471800843291,
253.563583111008,253.655333096758,253.747076606481,253.838839435191,253.930714929871,
254.022647931948,254.11475605418,254.195456827442,254.323775817272,254.448100230519,
254.468996577584),.UNSPECIFIED.);
#7922=B_SPLINE_CURVE_WITH_KNOTS('',3,(#88569,#88570,#88571,#88572,#88573,
#88574,#88575,#88576,#88577,#88578,#88579,#88580,#88581,#88582,#88583,#88584,
#88585,#88586,#88587,#88588,#88589,#88590,#88591,#88592,#88593,#88594,#88595,
#88596,#88597,#88598,#88599,#88600,#88601,#88602,#88603,#88604,#88605,#88606,
#88607,#88608,#88609,#88610,#88611,#88612,#88613,#88614,#88615,#88616,#88617,
#88618,#88619,#88620,#88621,#88622,#88623,#88624,#88625,#88626,#88627,#88628,
#88629,#88630,#88631,#88632,#88633,#88634,#88635,#88636,#88637,#88638,#88639,
#88640,#88641,#88642,#88643,#88644,#88645,#88646,#88647,#88648,#88649,#88650,
#88651,#88652,#88653,#88654,#88655,#88656,#88657,#88658,#88659,#88660,#88661,
#88662),.UNSPECIFIED.,.F.,.F.,(4,3,3,3,3,3,3,3,3,3,3,3,3,3,3,3,3,3,3,3,
3,3,3,3,3,3,3,3,3,3,3,4),(-0.733254803425731,-0.716860866713633,-0.679748362314261,
-0.642635857914888,-0.636142894777821,-0.600007081989827,-0.56382585245897,
-0.553070625843985,-0.54406265969124,-0.537131974197663,-0.501769106615608,
-0.46673168776426,-0.43271025548486,-0.39921344459524,-0.394763476316668,
-0.361144611505345,-0.341796862292531,-0.307536621934649,-0.28230306870699,
-0.26968629209316,-0.261838674652597,-0.25706951547933,-0.223658877959798,
-0.190162157167782,-0.157167270601885,-0.13748660874309,-0.127812017122585,
-0.123152698597241,-0.090954045835124,-0.059210042099216,-0.0284424625824032,
0.),.UNSPECIFIED.);
#7923=B_SPLINE_CURVE_WITH_KNOTS('',3,(#88663,#88664,#88665,#88666,#88667,
#88668,#88669,#88670,#88671,#88672,#88673,#88674,#88675,#88676,#88677,#88678,
#88679,#88680,#88681,#88682,#88683,#88684,#88685,#88686,#88687,#88688,#88689,
#88690,#88691,#88692,#88693,#88694,#88695,#88696,#88697,#88698,#88699,#88700,
#88701,#88702,#88703,#88704,#88705,#88706,#88707,#88708,#88709,#88710,#88711,
#88712,#88713,#88714,#88715,#88716,#88717,#88718,#88719,#88720,#88721,#88722,
#88723,#88724,#88725,#88726,#88727,#88728,#88729,#88730,#88731,#88732,#88733,
#88734,#88735,#88736,#88737,#88738,#88739,#88740,#88741,#88742,#88743,#88744,
#88745,#88746,#88747,#88748,#88749,#88750,#88751,#88752,#88753,#88754,#88755,
#88756),.UNSPECIFIED.,.F.,.F.,(4,3,3,3,3,3,3,3,3,3,3,3,3,3,3,3,3,3,3,3,
3,3,3,3,3,3,3,3,3,3,3,4),(-0.744397949170787,-0.724090770909356,-0.692915940750181,
-0.673393480001504,-0.66080333861376,-0.655138471145222,-0.623098446486558,
-0.590256033718165,-0.579287000783627,-0.573000422069116,-0.567857258151979,
-0.534328239229759,-0.500402513905905,-0.466554389450806,-0.444853816956689,
-0.43717569305135,-0.432782155152661,-0.397866775303715,-0.379066408601939,
-0.345035254109968,-0.311004099617997,-0.300241994933858,-0.295254487285989,
-0.26002895078779,-0.224649697158664,-0.188790758835381,-0.154352341293194,
-0.14704631389687,-0.110284735422653,-0.0734773653247291,-0.0367386826623646,
0.),.UNSPECIFIED.);
#7924=B_SPLINE_CURVE_WITH_KNOTS('',3,(#89758,#89759,#89760,#89761),
 .UNSPECIFIED.,.F.,.F.,(4,4),(-0.0803409632413212,0.),.UNSPECIFIED.);
#7925=B_SPLINE_CURVE_WITH_KNOTS('',3,(#89762,#89763,#89764,#89765,#89766,
#89767,#89768,#89769,#89770,#89771,#89772,#89773,#89774,#89775,#89776,#89777,
#89778,#89779,#89780,#89781,#89782,#89783,#89784,#89785,#89786,#89787,#89788,
#89789,#89790,#89791,#89792,#89793,#89794,#89795,#89796,#89797,#89798,#89799,
#89800,#89801,#89802,#89803,#89804,#89805,#89806,#89807,#89808,#89809,#89810,
#89811,#89812,#89813,#89814,#89815,#89816,#89817,#89818,#89819,#89820,#89821,
#89822,#89823,#89824,#89825,#89826,#89827,#89828,#89829,#89830,#89831,#89832,
#89833,#89834,#89835,#89836,#89837,#89838,#89839,#89840,#89841,#89842,#89843,
#89844,#89845,#89846,#89847,#89848,#89849,#89850,#89851,#89852,#89853,#89854,
#89855),.UNSPECIFIED.,.F.,.F.,(4,3,3,3,3,3,3,3,3,3,3,3,3,3,3,3,3,3,3,3,
3,3,3,3,3,3,3,3,3,3,3,4),(-0.744397949170576,-0.724090770909119,-0.692447050614166,
-0.660803330319212,-0.655138464383618,-0.623098432155756,-0.590256016159068,
-0.579286988813744,-0.573000381486176,-0.567857225037418,-0.534328202041861,
-0.500402475785612,-0.466554351992817,-0.444853787732292,-0.437346141655956,
-0.432781471426868,-0.397866091919205,-0.37906640860182,-0.345356387811567,
-0.311004091679875,-0.300241984011793,-0.291751811164854,-0.257317537005326,
-0.221788209983448,-0.185939475150322,-0.162697040756532,-0.153848887443103,
-0.146031932641978,-0.109290096749417,-0.0724860010487071,-0.0362430005243535,
0.),.UNSPECIFIED.);
#7926=B_SPLINE_CURVE_WITH_KNOTS('',3,(#89861,#89862,#89863,#89864,#89865,
#89866,#89867,#89868,#89869,#89870,#89871,#89872,#89873,#89874,#89875,#89876,
#89877,#89878,#89879,#89880,#89881,#89882,#89883,#89884,#89885,#89886,#89887,
#89888,#89889,#89890,#89891,#89892,#89893,#89894,#89895,#89896,#89897,#89898,
#89899,#89900,#89901,#89902,#89903,#89904,#89905,#89906,#89907,#89908,#89909,
#89910,#89911,#89912,#89913,#89914,#89915,#89916,#89917,#89918,#89919,#89920,
#89921,#89922,#89923,#89924,#89925,#89926,#89927,#89928,#89929,#89930,#89931,
#89932,#89933,#89934,#89935,#89936,#89937,#89938,#89939,#89940,#89941,#89942,
#89943,#89944,#89945),.UNSPECIFIED.,.F.,.F.,(4,3,3,3,3,3,3,3,3,3,3,3,3,
3,3,3,3,3,3,3,3,3,3,3,3,3,3,3,4),(-0.73325467290433,-0.716860866713702,
-0.679748364117748,-0.642635861521795,-0.636142895543889,-0.599983228880824,
-0.563846742146268,-0.544365777261658,-0.537678149333536,-0.502312771444872,
-0.467268175507533,-0.433239334102402,-0.399213462994925,-0.394763515206197,
-0.361144657010498,-0.341796862292533,-0.307557044899139,-0.273156786925689,
-0.262814068526211,-0.257069517219618,-0.223635413959772,-0.190149431339904,
-0.157260198228449,-0.127811989049523,-0.123152691782714,-0.0909540316151254,
-0.0592100170113393,-0.0284424232172037,-2.14959275585417E-14),
 .UNSPECIFIED.);
#7927=B_SPLINE_CURVE_WITH_KNOTS('',3,(#90946,#90947,#90948,#90949),
 .UNSPECIFIED.,.F.,.F.,(4,4),(0.,0.0803420936465104),.UNSPECIFIED.);
#9035=VERTEX_POINT('',#61992);
#9036=VERTEX_POINT('',#61993);
#9037=VERTEX_POINT('',#61995);
#9038=VERTEX_POINT('',#62105);
#9039=VERTEX_POINT('',#62175);
#9040=VERTEX_POINT('',#62176);
#9041=VERTEX_POINT('',#62178);
#9042=VERTEX_POINT('',#62391);
#9043=VERTEX_POINT('',#62605);
#9044=VERTEX_POINT('',#62606);
#9045=VERTEX_POINT('',#62608);
#9046=VERTEX_POINT('',#62818);
#9047=VERTEX_POINT('',#63032);
#9048=VERTEX_POINT('',#63033);
#9049=VERTEX_POINT('',#63035);
#9050=VERTEX_POINT('',#63248);
#9051=VERTEX_POINT('',#63488);
#9052=VERTEX_POINT('',#63489);
#9053=VERTEX_POINT('',#63491);
#9054=VERTEX_POINT('',#63952);
#9055=VERTEX_POINT('',#63953);
#9056=VERTEX_POINT('',#63955);
#9057=VERTEX_POINT('',#64037);
#9058=VERTEX_POINT('',#64295);
#9059=VERTEX_POINT('',#64296);
#9060=VERTEX_POINT('',#64298);
#9061=VERTEX_POINT('',#64693);
#9062=VERTEX_POINT('',#64694);
#9063=VERTEX_POINT('',#64696);
#9064=VERTEX_POINT('',#64778);
#9065=VERTEX_POINT('',#65026);
#9066=VERTEX_POINT('',#65027);
#9067=VERTEX_POINT('',#65029);
#9068=VERTEX_POINT('',#65418);
#9069=VERTEX_POINT('',#65419);
#9070=VERTEX_POINT('',#65421);
#9071=VERTEX_POINT('',#65503);
#9072=VERTEX_POINT('',#65801);
#9073=VERTEX_POINT('',#65802);
#9074=VERTEX_POINT('',#65804);
#9075=VERTEX_POINT('',#66200);
#9076=VERTEX_POINT('',#66201);
#9077=VERTEX_POINT('',#66203);
#9078=VERTEX_POINT('',#66416);
#9079=VERTEX_POINT('',#66756);
#9080=VERTEX_POINT('',#66757);
#9081=VERTEX_POINT('',#66759);
#9082=VERTEX_POINT('',#67217);
#9083=VERTEX_POINT('',#67218);
#9084=VERTEX_POINT('',#67220);
#9085=VERTEX_POINT('',#67433);
#9086=VERTEX_POINT('',#67747);
#9087=VERTEX_POINT('',#67748);
#9088=VERTEX_POINT('',#67750);
#9089=VERTEX_POINT('',#68200);
#9090=VERTEX_POINT('',#68201);
#9091=VERTEX_POINT('',#68203);
#9092=VERTEX_POINT('',#68413);
#9093=VERTEX_POINT('',#68739);
#9094=VERTEX_POINT('',#68740);
#9095=VERTEX_POINT('',#68742);
#9096=VERTEX_POINT('',#69201);
#9097=VERTEX_POINT('',#69202);
#9098=VERTEX_POINT('',#69204);
#9099=VERTEX_POINT('',#69420);
#9100=VERTEX_POINT('',#69712);
#9101=VERTEX_POINT('',#69713);
#9102=VERTEX_POINT('',#69715);
#9103=VERTEX_POINT('',#70195);
#9104=VERTEX_POINT('',#70196);
#9105=VERTEX_POINT('',#70198);
#9106=VERTEX_POINT('',#70411);
#9107=VERTEX_POINT('',#70659);
#9108=VERTEX_POINT('',#70660);
#9109=VERTEX_POINT('',#70662);
#9110=VERTEX_POINT('',#71126);
#9111=VERTEX_POINT('',#71127);
#9112=VERTEX_POINT('',#71129);
#9113=VERTEX_POINT('',#71342);
#9114=VERTEX_POINT('',#71590);
#9115=VERTEX_POINT('',#71591);
#9116=VERTEX_POINT('',#71593);
#9117=VERTEX_POINT('',#72042);
#9118=VERTEX_POINT('',#72043);
#9119=VERTEX_POINT('',#72045);
#9120=VERTEX_POINT('',#72255);
#9121=VERTEX_POINT('',#72528);
#9122=VERTEX_POINT('',#72529);
#9123=VERTEX_POINT('',#72531);
#9124=VERTEX_POINT('',#72747);
#9125=VERTEX_POINT('',#72981);
#9126=VERTEX_POINT('',#72982);
#9127=VERTEX_POINT('',#72984);
#9128=VERTEX_POINT('',#73454);
#9129=VERTEX_POINT('',#73455);
#9130=VERTEX_POINT('',#73457);
#9131=VERTEX_POINT('',#73670);
#9132=VERTEX_POINT('',#73922);
#9133=VERTEX_POINT('',#73923);
#9134=VERTEX_POINT('',#73925);
#9135=VERTEX_POINT('',#74394);
#9136=VERTEX_POINT('',#74395);
#9137=VERTEX_POINT('',#74397);
#9138=VERTEX_POINT('',#74610);
#9139=VERTEX_POINT('',#74856);
#9140=VERTEX_POINT('',#74857);
#9141=VERTEX_POINT('',#74859);
#9142=VERTEX_POINT('',#75316);
#9143=VERTEX_POINT('',#75317);
#9144=VERTEX_POINT('',#75319);
#9145=VERTEX_POINT('',#75529);
#9146=VERTEX_POINT('',#75802);
#9147=VERTEX_POINT('',#75803);
#9148=VERTEX_POINT('',#75805);
#9149=VERTEX_POINT('',#76021);
#9150=VERTEX_POINT('',#76259);
#9151=VERTEX_POINT('',#76260);
#9152=VERTEX_POINT('',#76262);
#9153=VERTEX_POINT('',#76730);
#9154=VERTEX_POINT('',#76731);
#9155=VERTEX_POINT('',#76733);
#9156=VERTEX_POINT('',#76946);
#9157=VERTEX_POINT('',#77192);
#9158=VERTEX_POINT('',#77193);
#9159=VERTEX_POINT('',#77195);
#9160=VERTEX_POINT('',#77653);
#9161=VERTEX_POINT('',#77654);
#9162=VERTEX_POINT('',#77656);
#9163=VERTEX_POINT('',#77869);
#9164=VERTEX_POINT('',#78090);
#9165=VERTEX_POINT('',#78091);
#9166=VERTEX_POINT('',#78093);
#9167=VERTEX_POINT('',#78303);
#9168=VERTEX_POINT('',#78386);
#9169=VERTEX_POINT('',#78387);
#9170=VERTEX_POINT('',#78389);
#9171=VERTEX_POINT('',#78599);
#9172=VERTEX_POINT('',#78746);
#9173=VERTEX_POINT('',#78747);
#9174=VERTEX_POINT('',#78749);
#9175=VERTEX_POINT('',#78965);
#9176=VERTEX_POINT('',#79048);
#9177=VERTEX_POINT('',#79049);
#9178=VERTEX_POINT('',#79123);
#9179=VERTEX_POINT('',#79125);
#9180=VERTEX_POINT('',#79131);
#9181=VERTEX_POINT('',#79358);
#9182=VERTEX_POINT('',#79369);
#9183=VERTEX_POINT('',#79593);
#9184=VERTEX_POINT('',#79823);
#9185=VERTEX_POINT('',#79834);
#9186=VERTEX_POINT('',#80061);
#9187=VERTEX_POINT('',#80073);
#9188=VERTEX_POINT('',#80297);
#9189=VERTEX_POINT('',#80308);
#9190=VERTEX_POINT('',#80532);
#9191=VERTEX_POINT('',#80762);
#9192=VERTEX_POINT('',#80773);
#9193=VERTEX_POINT('',#81000);
#9194=VERTEX_POINT('',#81012);
#9195=VERTEX_POINT('',#81239);
#9196=VERTEX_POINT('',#81250);
#9197=VERTEX_POINT('',#81474);
#9198=VERTEX_POINT('',#81704);
#9199=VERTEX_POINT('',#81715);
#9200=VERTEX_POINT('',#81942);
#9201=VERTEX_POINT('',#81954);
#9202=VERTEX_POINT('',#82181);
#9203=VERTEX_POINT('',#82192);
#9204=VERTEX_POINT('',#82416);
#9205=VERTEX_POINT('',#82429);
#9206=VERTEX_POINT('',#82656);
#9207=VERTEX_POINT('',#82667);
#9208=VERTEX_POINT('',#82679);
#9209=VERTEX_POINT('',#82906);
#9210=VERTEX_POINT('',#82917);
#9211=VERTEX_POINT('',#83141);
#9212=VERTEX_POINT('',#83154);
#9213=VERTEX_POINT('',#83381);
#9214=VERTEX_POINT('',#83392);
#9215=VERTEX_POINT('',#83404);
#9216=VERTEX_POINT('',#83631);
#9217=VERTEX_POINT('',#83642);
#9218=VERTEX_POINT('',#83869);
#9219=VERTEX_POINT('',#84051);
#9220=VERTEX_POINT('',#84053);
#9221=VERTEX_POINT('',#84062);
#9222=VERTEX_POINT('',#84286);
#9223=VERTEX_POINT('',#84297);
#9224=VERTEX_POINT('',#84524);
#9225=VERTEX_POINT('',#84536);
#9226=VERTEX_POINT('',#84763);
#9227=VERTEX_POINT('',#84774);
#9228=VERTEX_POINT('',#85004);
#9229=VERTEX_POINT('',#85228);
#9230=VERTEX_POINT('',#85239);
#9231=VERTEX_POINT('',#85466);
#9232=VERTEX_POINT('',#85478);
#9233=VERTEX_POINT('',#85705);
#9234=VERTEX_POINT('',#85716);
#9235=VERTEX_POINT('',#85946);
#9236=VERTEX_POINT('',#86170);
#9237=VERTEX_POINT('',#86181);
#9238=VERTEX_POINT('',#86192);
#9239=VERTEX_POINT('',#86204);
#9240=VERTEX_POINT('',#86431);
#9241=VERTEX_POINT('',#86442);
#9242=VERTEX_POINT('',#86672);
#9243=VERTEX_POINT('',#86683);
#9244=VERTEX_POINT('',#86910);
#9245=VERTEX_POINT('',#86921);
#9246=VERTEX_POINT('',#87148);
#9247=VERTEX_POINT('',#87159);
#9248=VERTEX_POINT('',#87170);
#9249=VERTEX_POINT('',#87400);
#9250=VERTEX_POINT('',#87411);
#9251=VERTEX_POINT('',#87638);
#9252=VERTEX_POINT('',#87649);
#9253=VERTEX_POINT('',#87876);
#9254=VERTEX_POINT('',#87887);
#9255=VERTEX_POINT('',#87898);
#9256=VERTEX_POINT('',#88125);
#9257=VERTEX_POINT('',#88136);
#9258=VERTEX_POINT('',#88374);
#9259=VERTEX_POINT('',#88381);
#9260=VERTEX_POINT('',#88452);
#9261=VERTEX_POINT('',#88454);
#9262=VERTEX_POINT('',#88559);
#9263=VERTEX_POINT('',#88561);
#9264=VERTEX_POINT('',#88566);
#9265=VERTEX_POINT('',#88567);
#9266=VERTEX_POINT('',#89857);
#9267=VERTEX_POINT('',#89859);
#9268=VERTEX_POINT('',#90951);
#9269=VERTEX_POINT('',#90956);
#9270=VERTEX_POINT('',#90960);
#9271=VERTEX_POINT('',#90964);
#9272=VERTEX_POINT('',#90967);
#9273=VERTEX_POINT('',#90971);
#9274=VERTEX_POINT('',#90974);
#9275=VERTEX_POINT('',#90978);
#11550=EDGE_CURVE('',#9035,#9036,#2740,.T.);
#11551=EDGE_CURVE('',#9037,#9035,#7699,.T.);
#11552=EDGE_CURVE('',#9038,#9037,#784,.T.);
#11553=EDGE_CURVE('',#9038,#9036,#7700,.T.);
#11554=EDGE_CURVE('',#9039,#9040,#2741,.T.);
#11555=EDGE_CURVE('',#9041,#9039,#7701,.T.);
#11556=EDGE_CURVE('',#9035,#9041,#7702,.T.);
#11557=EDGE_CURVE('',#9036,#9042,#7703,.T.);
#11558=EDGE_CURVE('',#9042,#9040,#7704,.T.);
#11559=EDGE_CURVE('',#9043,#9044,#2742,.T.);
#11560=EDGE_CURVE('',#9045,#9043,#7705,.T.);
#11561=EDGE_CURVE('',#9039,#9045,#7706,.T.);
#11562=EDGE_CURVE('',#9040,#9046,#7707,.T.);
#11563=EDGE_CURVE('',#9046,#9044,#7708,.T.);
#11564=EDGE_CURVE('',#9047,#9048,#2743,.T.);
#11565=EDGE_CURVE('',#9049,#9047,#7709,.T.);
#11566=EDGE_CURVE('',#9043,#9049,#7710,.T.);
#11567=EDGE_CURVE('',#9044,#9050,#7711,.T.);
#11568=EDGE_CURVE('',#9050,#9048,#7712,.T.);
#11569=EDGE_CURVE('',#9051,#9052,#2744,.T.);
#11570=EDGE_CURVE('',#9053,#9051,#7713,.T.);
#11571=EDGE_CURVE('',#9047,#9053,#7714,.T.);
#11572=EDGE_CURVE('',#9048,#9052,#7715,.T.);
#11573=EDGE_CURVE('',#9054,#9055,#2745,.T.);
#11574=EDGE_CURVE('',#9056,#9054,#7716,.T.);
#11575=EDGE_CURVE('',#9051,#9056,#7717,.T.);
#11576=EDGE_CURVE('',#9052,#9057,#7718,.T.);
#11577=EDGE_CURVE('',#9057,#9055,#7719,.T.);
#11578=EDGE_CURVE('',#9058,#9059,#2746,.T.);
#11579=EDGE_CURVE('',#9060,#9058,#7720,.T.);
#11580=EDGE_CURVE('',#9054,#9060,#7721,.T.);
#11581=EDGE_CURVE('',#9055,#9059,#7722,.T.);
#11582=EDGE_CURVE('',#9061,#9062,#2747,.T.);
#11583=EDGE_CURVE('',#9063,#9061,#7723,.T.);
#11584=EDGE_CURVE('',#9058,#9063,#7724,.T.);
#11585=EDGE_CURVE('',#9059,#9064,#7725,.T.);
#11586=EDGE_CURVE('',#9064,#9062,#7726,.T.);
#11587=EDGE_CURVE('',#9065,#9066,#2748,.T.);
#11588=EDGE_CURVE('',#9067,#9065,#7727,.T.);
#11589=EDGE_CURVE('',#9061,#9067,#7728,.T.);
#11590=EDGE_CURVE('',#9062,#9066,#7729,.T.);
#11591=EDGE_CURVE('',#9068,#9069,#2749,.T.);
#11592=EDGE_CURVE('',#9070,#9068,#7730,.T.);
#11593=EDGE_CURVE('',#9065,#9070,#7731,.T.);
#11594=EDGE_CURVE('',#9066,#9071,#7732,.T.);
#11595=EDGE_CURVE('',#9071,#9069,#7733,.T.);
#11596=EDGE_CURVE('',#9072,#9073,#2750,.T.);
#11597=EDGE_CURVE('',#9074,#9072,#7734,.T.);
#11598=EDGE_CURVE('',#9068,#9074,#7735,.T.);
#11599=EDGE_CURVE('',#9069,#9073,#7736,.T.);
#11600=EDGE_CURVE('',#9075,#9076,#2751,.T.);
#11601=EDGE_CURVE('',#9077,#9075,#7737,.T.);
#11602=EDGE_CURVE('',#9072,#9077,#7738,.T.);
#11603=EDGE_CURVE('',#9073,#9078,#7739,.T.);
#11604=EDGE_CURVE('',#9078,#9076,#7740,.T.);
#11605=EDGE_CURVE('',#9079,#9080,#2752,.T.);
#11606=EDGE_CURVE('',#9081,#9079,#7741,.T.);
#11607=EDGE_CURVE('',#9075,#9081,#7742,.T.);
#11608=EDGE_CURVE('',#9076,#9080,#7743,.T.);
#11609=EDGE_CURVE('',#9082,#9083,#2753,.T.);
#11610=EDGE_CURVE('',#9084,#9082,#7744,.T.);
#11611=EDGE_CURVE('',#9079,#9084,#7745,.T.);
#11612=EDGE_CURVE('',#9080,#9085,#7746,.T.);
#11613=EDGE_CURVE('',#9085,#9083,#7747,.T.);
#11614=EDGE_CURVE('',#9086,#9087,#2754,.T.);
#11615=EDGE_CURVE('',#9088,#9086,#7748,.T.);
#11616=EDGE_CURVE('',#9082,#9088,#7749,.T.);
#11617=EDGE_CURVE('',#9083,#9087,#7750,.T.);
#11618=EDGE_CURVE('',#9089,#9090,#2755,.T.);
#11619=EDGE_CURVE('',#9091,#9089,#7751,.T.);
#11620=EDGE_CURVE('',#9086,#9091,#7752,.T.);
#11621=EDGE_CURVE('',#9087,#9092,#7753,.T.);
#11622=EDGE_CURVE('',#9092,#9090,#7754,.T.);
#11623=EDGE_CURVE('',#9093,#9094,#2756,.T.);
#11624=EDGE_CURVE('',#9095,#9093,#7755,.T.);
#11625=EDGE_CURVE('',#9089,#9095,#7756,.T.);
#11626=EDGE_CURVE('',#9090,#9094,#7757,.T.);
#11627=EDGE_CURVE('',#9096,#9097,#2757,.T.);
#11628=EDGE_CURVE('',#9098,#9096,#7758,.T.);
#11629=EDGE_CURVE('',#9093,#9098,#7759,.T.);
#11630=EDGE_CURVE('',#9094,#9099,#7760,.T.);
#11631=EDGE_CURVE('',#9099,#9097,#7761,.T.);
#11632=EDGE_CURVE('',#9100,#9101,#2758,.T.);
#11633=EDGE_CURVE('',#9102,#9100,#7762,.T.);
#11634=EDGE_CURVE('',#9096,#9102,#7763,.T.);
#11635=EDGE_CURVE('',#9097,#9101,#7764,.T.);
#11636=EDGE_CURVE('',#9103,#9104,#2759,.T.);
#11637=EDGE_CURVE('',#9105,#9103,#7765,.T.);
#11638=EDGE_CURVE('',#9100,#9105,#7766,.T.);
#11639=EDGE_CURVE('',#9101,#9106,#7767,.T.);
#11640=EDGE_CURVE('',#9106,#9104,#7768,.T.);
#11641=EDGE_CURVE('',#9107,#9108,#2760,.T.);
#11642=EDGE_CURVE('',#9109,#9107,#7769,.T.);
#11643=EDGE_CURVE('',#9103,#9109,#7770,.T.);
#11644=EDGE_CURVE('',#9104,#9108,#7771,.T.);
#11645=EDGE_CURVE('',#9110,#9111,#2761,.T.);
#11646=EDGE_CURVE('',#9112,#9110,#7772,.T.);
#11647=EDGE_CURVE('',#9107,#9112,#7773,.T.);
#11648=EDGE_CURVE('',#9108,#9113,#7774,.T.);
#11649=EDGE_CURVE('',#9113,#9111,#7775,.T.);
#11650=EDGE_CURVE('',#9114,#9115,#2762,.T.);
#11651=EDGE_CURVE('',#9116,#9114,#7776,.T.);
#11652=EDGE_CURVE('',#9110,#9116,#7777,.T.);
#11653=EDGE_CURVE('',#9111,#9115,#7778,.T.);
#11654=EDGE_CURVE('',#9117,#9118,#2763,.T.);
#11655=EDGE_CURVE('',#9119,#9117,#7779,.T.);
#11656=EDGE_CURVE('',#9114,#9119,#7780,.T.);
#11657=EDGE_CURVE('',#9115,#9120,#7781,.T.);
#11658=EDGE_CURVE('',#9120,#9118,#7782,.T.);
#11659=EDGE_CURVE('',#9121,#9122,#2764,.T.);
#11660=EDGE_CURVE('',#9123,#9121,#7783,.T.);
#11661=EDGE_CURVE('',#9117,#9123,#7784,.T.);
#11662=EDGE_CURVE('',#9118,#9124,#7785,.T.);
#11663=EDGE_CURVE('',#9124,#9122,#7786,.T.);
#11664=EDGE_CURVE('',#9125,#9126,#2765,.T.);
#11665=EDGE_CURVE('',#9127,#9125,#7787,.T.);
#11666=EDGE_CURVE('',#9121,#9127,#7788,.T.);
#11667=EDGE_CURVE('',#9122,#9126,#7789,.T.);
#11668=EDGE_CURVE('',#9128,#9129,#2766,.T.);
#11669=EDGE_CURVE('',#9130,#9128,#7790,.T.);
#11670=EDGE_CURVE('',#9125,#9130,#7791,.T.);
#11671=EDGE_CURVE('',#9126,#9131,#7792,.T.);
#11672=EDGE_CURVE('',#9131,#9129,#7793,.T.);
#11673=EDGE_CURVE('',#9132,#9133,#2767,.T.);
#11674=EDGE_CURVE('',#9134,#9132,#7794,.T.);
#11675=EDGE_CURVE('',#9128,#9134,#7795,.T.);
#11676=EDGE_CURVE('',#9129,#9133,#7796,.T.);
#11677=EDGE_CURVE('',#9135,#9136,#2768,.T.);
#11678=EDGE_CURVE('',#9137,#9135,#7797,.T.);
#11679=EDGE_CURVE('',#9132,#9137,#7798,.T.);
#11680=EDGE_CURVE('',#9133,#9138,#7799,.T.);
#11681=EDGE_CURVE('',#9138,#9136,#7800,.T.);
#11682=EDGE_CURVE('',#9139,#9140,#2769,.T.);
#11683=EDGE_CURVE('',#9141,#9139,#7801,.T.);
#11684=EDGE_CURVE('',#9135,#9141,#7802,.T.);
#11685=EDGE_CURVE('',#9136,#9140,#7803,.T.);
#11686=EDGE_CURVE('',#9142,#9143,#2770,.T.);
#11687=EDGE_CURVE('',#9144,#9142,#7804,.T.);
#11688=EDGE_CURVE('',#9139,#9144,#7805,.T.);
#11689=EDGE_CURVE('',#9140,#9145,#7806,.T.);
#11690=EDGE_CURVE('',#9145,#9143,#7807,.T.);
#11691=EDGE_CURVE('',#9146,#9147,#2771,.T.);
#11692=EDGE_CURVE('',#9148,#9146,#7808,.T.);
#11693=EDGE_CURVE('',#9142,#9148,#7809,.T.);
#11694=EDGE_CURVE('',#9143,#9149,#7810,.T.);
#11695=EDGE_CURVE('',#9149,#9147,#7811,.T.);
#11696=EDGE_CURVE('',#9150,#9151,#2772,.T.);
#11697=EDGE_CURVE('',#9152,#9150,#7812,.T.);
#11698=EDGE_CURVE('',#9146,#9152,#7813,.T.);
#11699=EDGE_CURVE('',#9147,#9151,#7814,.T.);
#11700=EDGE_CURVE('',#9153,#9154,#2773,.T.);
#11701=EDGE_CURVE('',#9155,#9153,#7815,.T.);
#11702=EDGE_CURVE('',#9150,#9155,#7816,.T.);
#11703=EDGE_CURVE('',#9151,#9156,#7817,.T.);
#11704=EDGE_CURVE('',#9156,#9154,#7818,.T.);
#11705=EDGE_CURVE('',#9157,#9158,#2774,.T.);
#11706=EDGE_CURVE('',#9159,#9157,#7819,.T.);
#11707=EDGE_CURVE('',#9153,#9159,#7820,.T.);
#11708=EDGE_CURVE('',#9154,#9158,#7821,.T.);
#11709=EDGE_CURVE('',#9160,#9161,#2775,.T.);
#11710=EDGE_CURVE('',#9162,#9160,#7822,.T.);
#11711=EDGE_CURVE('',#9157,#9162,#7823,.T.);
#11712=EDGE_CURVE('',#9158,#9163,#7824,.T.);
#11713=EDGE_CURVE('',#9163,#9161,#7825,.T.);
#11714=EDGE_CURVE('',#9164,#9165,#2776,.T.);
#11715=EDGE_CURVE('',#9166,#9164,#7826,.T.);
#11716=EDGE_CURVE('',#9160,#9166,#7827,.T.);
#11717=EDGE_CURVE('',#9161,#9167,#7828,.T.);
#11718=EDGE_CURVE('',#9167,#9165,#7829,.T.);
#11719=EDGE_CURVE('',#9168,#9169,#2777,.T.);
#11720=EDGE_CURVE('',#9170,#9168,#7830,.T.);
#11721=EDGE_CURVE('',#9164,#9170,#7831,.T.);
#11722=EDGE_CURVE('',#9165,#9171,#7832,.T.);
#11723=EDGE_CURVE('',#9171,#9169,#7833,.T.);
#11724=EDGE_CURVE('',#9172,#9173,#2778,.T.);
#11725=EDGE_CURVE('',#9174,#9172,#7834,.T.);
#11726=EDGE_CURVE('',#9168,#9174,#7835,.T.);
#11727=EDGE_CURVE('',#9169,#9175,#7836,.T.);
#11728=EDGE_CURVE('',#9175,#9173,#7837,.T.);
#11729=EDGE_CURVE('',#9176,#9177,#7838,.T.);
#11730=EDGE_CURVE('',#9177,#9178,#785,.T.);
#11731=EDGE_CURVE('',#9178,#9179,#7839,.T.);
#11732=EDGE_CURVE('',#9179,#9180,#7840,.T.);
#11733=EDGE_CURVE('',#9180,#9181,#7841,.T.);
#11734=EDGE_CURVE('',#9181,#9182,#7842,.T.);
#11735=EDGE_CURVE('',#9182,#9183,#7843,.T.);
#11736=EDGE_CURVE('',#9183,#9184,#7844,.T.);
#11737=EDGE_CURVE('',#9184,#9185,#7845,.T.);
#11738=EDGE_CURVE('',#9185,#9186,#7846,.T.);
#11739=EDGE_CURVE('',#9186,#9187,#7847,.T.);
#11740=EDGE_CURVE('',#9187,#9188,#7848,.T.);
#11741=EDGE_CURVE('',#9188,#9189,#7849,.T.);
#11742=EDGE_CURVE('',#9189,#9190,#7850,.T.);
#11743=EDGE_CURVE('',#9190,#9191,#7851,.T.);
#11744=EDGE_CURVE('',#9191,#9192,#7852,.T.);
#11745=EDGE_CURVE('',#9192,#9193,#7853,.T.);
#11746=EDGE_CURVE('',#9193,#9194,#7854,.T.);
#11747=EDGE_CURVE('',#9194,#9195,#7855,.T.);
#11748=EDGE_CURVE('',#9195,#9196,#7856,.T.);
#11749=EDGE_CURVE('',#9196,#9197,#7857,.T.);
#11750=EDGE_CURVE('',#9197,#9198,#7858,.T.);
#11751=EDGE_CURVE('',#9198,#9199,#7859,.T.);
#11752=EDGE_CURVE('',#9199,#9200,#7860,.T.);
#11753=EDGE_CURVE('',#9200,#9201,#7861,.T.);
#11754=EDGE_CURVE('',#9201,#9202,#7862,.T.);
#11755=EDGE_CURVE('',#9202,#9203,#7863,.T.);
#11756=EDGE_CURVE('',#9203,#9204,#7864,.T.);
#11757=EDGE_CURVE('',#9204,#9205,#7865,.T.);
#11758=EDGE_CURVE('',#9205,#9206,#7866,.T.);
#11759=EDGE_CURVE('',#9206,#9207,#7867,.T.);
#11760=EDGE_CURVE('',#9207,#9208,#7868,.T.);
#11761=EDGE_CURVE('',#9208,#9209,#7869,.T.);
#11762=EDGE_CURVE('',#9209,#9210,#7870,.T.);
#11763=EDGE_CURVE('',#9210,#9211,#7871,.T.);
#11764=EDGE_CURVE('',#9211,#9212,#7872,.T.);
#11765=EDGE_CURVE('',#9212,#9213,#7873,.T.);
#11766=EDGE_CURVE('',#9213,#9214,#7874,.T.);
#11767=EDGE_CURVE('',#9214,#9215,#7875,.T.);
#11768=EDGE_CURVE('',#9215,#9216,#7876,.T.);
#11769=EDGE_CURVE('',#9216,#9217,#7877,.T.);
#11770=EDGE_CURVE('',#9217,#9218,#7878,.T.);
#11771=EDGE_CURVE('',#9219,#9218,#786,.F.);
#11772=EDGE_CURVE('',#9219,#9220,#7879,.T.);
#11773=EDGE_CURVE('',#9220,#9221,#7880,.T.);
#11774=EDGE_CURVE('',#9221,#9222,#7881,.T.);
#11775=EDGE_CURVE('',#9222,#9223,#7882,.T.);
#11776=EDGE_CURVE('',#9223,#9224,#7883,.T.);
#11777=EDGE_CURVE('',#9224,#9225,#7884,.T.);
#11778=EDGE_CURVE('',#9225,#9226,#7885,.T.);
#11779=EDGE_CURVE('',#9226,#9227,#7886,.T.);
#11780=EDGE_CURVE('',#9227,#9228,#7887,.T.);
#11781=EDGE_CURVE('',#9228,#9229,#7888,.T.);
#11782=EDGE_CURVE('',#9229,#9230,#7889,.T.);
#11783=EDGE_CURVE('',#9230,#9231,#7890,.T.);
#11784=EDGE_CURVE('',#9231,#9232,#7891,.T.);
#11785=EDGE_CURVE('',#9232,#9233,#7892,.T.);
#11786=EDGE_CURVE('',#9233,#9234,#7893,.T.);
#11787=EDGE_CURVE('',#9234,#9235,#7894,.T.);
#11788=EDGE_CURVE('',#9235,#9236,#7895,.T.);
#11789=EDGE_CURVE('',#9236,#9237,#7896,.T.);
#11790=EDGE_CURVE('',#9237,#9238,#7897,.T.);
#11791=EDGE_CURVE('',#9238,#9239,#7898,.T.);
#11792=EDGE_CURVE('',#9239,#9240,#7899,.T.);
#11793=EDGE_CURVE('',#9240,#9241,#7900,.T.);
#11794=EDGE_CURVE('',#9241,#9242,#7901,.T.);
#11795=EDGE_CURVE('',#9242,#9243,#7902,.T.);
#11796=EDGE_CURVE('',#9243,#9244,#7903,.T.);
#11797=EDGE_CURVE('',#9244,#9245,#7904,.T.);
#11798=EDGE_CURVE('',#9245,#9246,#7905,.T.);
#11799=EDGE_CURVE('',#9246,#9247,#7906,.T.);
#11800=EDGE_CURVE('',#9247,#9248,#7907,.T.);
#11801=EDGE_CURVE('',#9248,#9249,#7908,.T.);
#11802=EDGE_CURVE('',#9249,#9250,#7909,.T.);
#11803=EDGE_CURVE('',#9250,#9251,#7910,.T.);
#11804=EDGE_CURVE('',#9251,#9252,#7911,.T.);
#11805=EDGE_CURVE('',#9252,#9253,#7912,.T.);
#11806=EDGE_CURVE('',#9253,#9254,#7913,.T.);
#11807=EDGE_CURVE('',#9254,#9255,#7914,.T.);
#11808=EDGE_CURVE('',#9255,#9256,#7915,.T.);
#11809=EDGE_CURVE('',#9256,#9257,#7916,.T.);
#11810=EDGE_CURVE('',#9257,#9176,#7917,.T.);
#11811=EDGE_CURVE('',#9173,#9258,#7918,.T.);
#11812=EDGE_CURVE('',#9258,#9259,#7919,.T.);
#11813=EDGE_CURVE('',#9260,#9259,#787,.T.);
#11814=EDGE_CURVE('',#9261,#9260,#7920,.T.);
#11815=EDGE_CURVE('',#9172,#9261,#7921,.T.);
#11816=EDGE_CURVE('',#9262,#9262,#788,.T.);
#11817=EDGE_CURVE('',#9262,#9263,#2779,.T.);
#11818=EDGE_CURVE('',#9263,#9263,#789,.T.);
#11819=EDGE_CURVE('',#9264,#9265,#790,.F.);
#11820=EDGE_CURVE('',#9264,#9260,#7922,.T.);
#11821=EDGE_CURVE('',#9259,#9219,#7923,.T.);
#11822=EDGE_CURVE('',#9265,#9219,#791,.F.);
#11823=EDGE_CURVE('',#9218,#9264,#7924,.T.);
#11824=EDGE_CURVE('',#9037,#9178,#7925,.T.);
#11825=EDGE_CURVE('',#9178,#9266,#792,.T.);
#11826=EDGE_CURVE('',#9266,#9267,#793,.T.);
#11827=EDGE_CURVE('',#9267,#9038,#7926,.T.);
#11828=EDGE_CURVE('',#9267,#9177,#7927,.T.);
#11829=EDGE_CURVE('',#9268,#9268,#794,.T.);
#11830=EDGE_CURVE('',#9266,#9268,#2780,.T.);
#11831=EDGE_CURVE('',#9265,#9269,#2781,.T.);
#11832=EDGE_CURVE('',#9269,#9269,#795,.T.);
#11833=EDGE_CURVE('',#9270,#9270,#796,.T.);
#11834=EDGE_CURVE('',#9270,#9269,#2782,.T.);
#11835=EDGE_CURVE('',#9271,#9271,#797,.T.);
#11836=EDGE_CURVE('',#9272,#9272,#798,.T.);
#11837=EDGE_CURVE('',#9272,#9271,#2783,.T.);
#11838=EDGE_CURVE('',#9273,#9273,#799,.T.);
#11839=EDGE_CURVE('',#9274,#9274,#800,.T.);
#11840=EDGE_CURVE('',#9274,#9273,#2784,.T.);
#11841=EDGE_CURVE('',#9274,#9275,#2785,.T.);
#11842=EDGE_CURVE('',#9275,#9275,#801,.T.);
#16151=ORIENTED_EDGE('',*,*,#11550,.F.);
#16152=ORIENTED_EDGE('',*,*,#11551,.F.);
#16153=ORIENTED_EDGE('',*,*,#11552,.F.);
#16154=ORIENTED_EDGE('',*,*,#11553,.T.);
#16155=ORIENTED_EDGE('',*,*,#11554,.F.);
#16156=ORIENTED_EDGE('',*,*,#11555,.F.);
#16157=ORIENTED_EDGE('',*,*,#11556,.F.);
#16158=ORIENTED_EDGE('',*,*,#11550,.T.);
#16159=ORIENTED_EDGE('',*,*,#11557,.T.);
#16160=ORIENTED_EDGE('',*,*,#11558,.T.);
#16161=ORIENTED_EDGE('',*,*,#11559,.F.);
#16162=ORIENTED_EDGE('',*,*,#11560,.F.);
#16163=ORIENTED_EDGE('',*,*,#11561,.F.);
#16164=ORIENTED_EDGE('',*,*,#11554,.T.);
#16165=ORIENTED_EDGE('',*,*,#11562,.T.);
#16166=ORIENTED_EDGE('',*,*,#11563,.T.);
#16167=ORIENTED_EDGE('',*,*,#11564,.F.);
#16168=ORIENTED_EDGE('',*,*,#11565,.F.);
#16169=ORIENTED_EDGE('',*,*,#11566,.F.);
#16170=ORIENTED_EDGE('',*,*,#11559,.T.);
#16171=ORIENTED_EDGE('',*,*,#11567,.T.);
#16172=ORIENTED_EDGE('',*,*,#11568,.T.);
#16173=ORIENTED_EDGE('',*,*,#11569,.F.);
#16174=ORIENTED_EDGE('',*,*,#11570,.F.);
#16175=ORIENTED_EDGE('',*,*,#11571,.F.);
#16176=ORIENTED_EDGE('',*,*,#11564,.T.);
#16177=ORIENTED_EDGE('',*,*,#11572,.T.);
#16178=ORIENTED_EDGE('',*,*,#11573,.F.);
#16179=ORIENTED_EDGE('',*,*,#11574,.F.);
#16180=ORIENTED_EDGE('',*,*,#11575,.F.);
#16181=ORIENTED_EDGE('',*,*,#11569,.T.);
#16182=ORIENTED_EDGE('',*,*,#11576,.T.);
#16183=ORIENTED_EDGE('',*,*,#11577,.T.);
#16184=ORIENTED_EDGE('',*,*,#11578,.F.);
#16185=ORIENTED_EDGE('',*,*,#11579,.F.);
#16186=ORIENTED_EDGE('',*,*,#11580,.F.);
#16187=ORIENTED_EDGE('',*,*,#11573,.T.);
#16188=ORIENTED_EDGE('',*,*,#11581,.T.);
#16189=ORIENTED_EDGE('',*,*,#11582,.F.);
#16190=ORIENTED_EDGE('',*,*,#11583,.F.);
#16191=ORIENTED_EDGE('',*,*,#11584,.F.);
#16192=ORIENTED_EDGE('',*,*,#11578,.T.);
#16193=ORIENTED_EDGE('',*,*,#11585,.T.);
#16194=ORIENTED_EDGE('',*,*,#11586,.T.);
#16195=ORIENTED_EDGE('',*,*,#11587,.F.);
#16196=ORIENTED_EDGE('',*,*,#11588,.F.);
#16197=ORIENTED_EDGE('',*,*,#11589,.F.);
#16198=ORIENTED_EDGE('',*,*,#11582,.T.);
#16199=ORIENTED_EDGE('',*,*,#11590,.T.);
#16200=ORIENTED_EDGE('',*,*,#11591,.F.);
#16201=ORIENTED_EDGE('',*,*,#11592,.F.);
#16202=ORIENTED_EDGE('',*,*,#11593,.F.);
#16203=ORIENTED_EDGE('',*,*,#11587,.T.);
#16204=ORIENTED_EDGE('',*,*,#11594,.T.);
#16205=ORIENTED_EDGE('',*,*,#11595,.T.);
#16206=ORIENTED_EDGE('',*,*,#11596,.F.);
#16207=ORIENTED_EDGE('',*,*,#11597,.F.);
#16208=ORIENTED_EDGE('',*,*,#11598,.F.);
#16209=ORIENTED_EDGE('',*,*,#11591,.T.);
#16210=ORIENTED_EDGE('',*,*,#11599,.T.);
#16211=ORIENTED_EDGE('',*,*,#11600,.F.);
#16212=ORIENTED_EDGE('',*,*,#11601,.F.);
#16213=ORIENTED_EDGE('',*,*,#11602,.F.);
#16214=ORIENTED_EDGE('',*,*,#11596,.T.);
#16215=ORIENTED_EDGE('',*,*,#11603,.T.);
#16216=ORIENTED_EDGE('',*,*,#11604,.T.);
#16217=ORIENTED_EDGE('',*,*,#11605,.F.);
#16218=ORIENTED_EDGE('',*,*,#11606,.F.);
#16219=ORIENTED_EDGE('',*,*,#11607,.F.);
#16220=ORIENTED_EDGE('',*,*,#11600,.T.);
#16221=ORIENTED_EDGE('',*,*,#11608,.T.);
#16222=ORIENTED_EDGE('',*,*,#11609,.F.);
#16223=ORIENTED_EDGE('',*,*,#11610,.F.);
#16224=ORIENTED_EDGE('',*,*,#11611,.F.);
#16225=ORIENTED_EDGE('',*,*,#11605,.T.);
#16226=ORIENTED_EDGE('',*,*,#11612,.T.);
#16227=ORIENTED_EDGE('',*,*,#11613,.T.);
#16228=ORIENTED_EDGE('',*,*,#11614,.F.);
#16229=ORIENTED_EDGE('',*,*,#11615,.F.);
#16230=ORIENTED_EDGE('',*,*,#11616,.F.);
#16231=ORIENTED_EDGE('',*,*,#11609,.T.);
#16232=ORIENTED_EDGE('',*,*,#11617,.T.);
#16233=ORIENTED_EDGE('',*,*,#11618,.F.);
#16234=ORIENTED_EDGE('',*,*,#11619,.F.);
#16235=ORIENTED_EDGE('',*,*,#11620,.F.);
#16236=ORIENTED_EDGE('',*,*,#11614,.T.);
#16237=ORIENTED_EDGE('',*,*,#11621,.T.);
#16238=ORIENTED_EDGE('',*,*,#11622,.T.);
#16239=ORIENTED_EDGE('',*,*,#11623,.F.);
#16240=ORIENTED_EDGE('',*,*,#11624,.F.);
#16241=ORIENTED_EDGE('',*,*,#11625,.F.);
#16242=ORIENTED_EDGE('',*,*,#11618,.T.);
#16243=ORIENTED_EDGE('',*,*,#11626,.T.);
#16244=ORIENTED_EDGE('',*,*,#11627,.F.);
#16245=ORIENTED_EDGE('',*,*,#11628,.F.);
#16246=ORIENTED_EDGE('',*,*,#11629,.F.);
#16247=ORIENTED_EDGE('',*,*,#11623,.T.);
#16248=ORIENTED_EDGE('',*,*,#11630,.T.);
#16249=ORIENTED_EDGE('',*,*,#11631,.T.);
#16250=ORIENTED_EDGE('',*,*,#11632,.F.);
#16251=ORIENTED_EDGE('',*,*,#11633,.F.);
#16252=ORIENTED_EDGE('',*,*,#11634,.F.);
#16253=ORIENTED_EDGE('',*,*,#11627,.T.);
#16254=ORIENTED_EDGE('',*,*,#11635,.T.);
#16255=ORIENTED_EDGE('',*,*,#11636,.F.);
#16256=ORIENTED_EDGE('',*,*,#11637,.F.);
#16257=ORIENTED_EDGE('',*,*,#11638,.F.);
#16258=ORIENTED_EDGE('',*,*,#11632,.T.);
#16259=ORIENTED_EDGE('',*,*,#11639,.T.);
#16260=ORIENTED_EDGE('',*,*,#11640,.T.);
#16261=ORIENTED_EDGE('',*,*,#11641,.F.);
#16262=ORIENTED_EDGE('',*,*,#11642,.F.);
#16263=ORIENTED_EDGE('',*,*,#11643,.F.);
#16264=ORIENTED_EDGE('',*,*,#11636,.T.);
#16265=ORIENTED_EDGE('',*,*,#11644,.T.);
#16266=ORIENTED_EDGE('',*,*,#11645,.F.);
#16267=ORIENTED_EDGE('',*,*,#11646,.F.);
#16268=ORIENTED_EDGE('',*,*,#11647,.F.);
#16269=ORIENTED_EDGE('',*,*,#11641,.T.);
#16270=ORIENTED_EDGE('',*,*,#11648,.T.);
#16271=ORIENTED_EDGE('',*,*,#11649,.T.);
#16272=ORIENTED_EDGE('',*,*,#11650,.F.);
#16273=ORIENTED_EDGE('',*,*,#11651,.F.);
#16274=ORIENTED_EDGE('',*,*,#11652,.F.);
#16275=ORIENTED_EDGE('',*,*,#11645,.T.);
#16276=ORIENTED_EDGE('',*,*,#11653,.T.);
#16277=ORIENTED_EDGE('',*,*,#11654,.F.);
#16278=ORIENTED_EDGE('',*,*,#11655,.F.);
#16279=ORIENTED_EDGE('',*,*,#11656,.F.);
#16280=ORIENTED_EDGE('',*,*,#11650,.T.);
#16281=ORIENTED_EDGE('',*,*,#11657,.T.);
#16282=ORIENTED_EDGE('',*,*,#11658,.T.);
#16283=ORIENTED_EDGE('',*,*,#11659,.F.);
#16284=ORIENTED_EDGE('',*,*,#11660,.F.);
#16285=ORIENTED_EDGE('',*,*,#11661,.F.);
#16286=ORIENTED_EDGE('',*,*,#11654,.T.);
#16287=ORIENTED_EDGE('',*,*,#11662,.T.);
#16288=ORIENTED_EDGE('',*,*,#11663,.T.);
#16289=ORIENTED_EDGE('',*,*,#11664,.F.);
#16290=ORIENTED_EDGE('',*,*,#11665,.F.);
#16291=ORIENTED_EDGE('',*,*,#11666,.F.);
#16292=ORIENTED_EDGE('',*,*,#11659,.T.);
#16293=ORIENTED_EDGE('',*,*,#11667,.T.);
#16294=ORIENTED_EDGE('',*,*,#11668,.F.);
#16295=ORIENTED_EDGE('',*,*,#11669,.F.);
#16296=ORIENTED_EDGE('',*,*,#11670,.F.);
#16297=ORIENTED_EDGE('',*,*,#11664,.T.);
#16298=ORIENTED_EDGE('',*,*,#11671,.T.);
#16299=ORIENTED_EDGE('',*,*,#11672,.T.);
#16300=ORIENTED_EDGE('',*,*,#11673,.F.);
#16301=ORIENTED_EDGE('',*,*,#11674,.F.);
#16302=ORIENTED_EDGE('',*,*,#11675,.F.);
#16303=ORIENTED_EDGE('',*,*,#11668,.T.);
#16304=ORIENTED_EDGE('',*,*,#11676,.T.);
#16305=ORIENTED_EDGE('',*,*,#11677,.F.);
#16306=ORIENTED_EDGE('',*,*,#11678,.F.);
#16307=ORIENTED_EDGE('',*,*,#11679,.F.);
#16308=ORIENTED_EDGE('',*,*,#11673,.T.);
#16309=ORIENTED_EDGE('',*,*,#11680,.T.);
#16310=ORIENTED_EDGE('',*,*,#11681,.T.);
#16311=ORIENTED_EDGE('',*,*,#11682,.F.);
#16312=ORIENTED_EDGE('',*,*,#11683,.F.);
#16313=ORIENTED_EDGE('',*,*,#11684,.F.);
#16314=ORIENTED_EDGE('',*,*,#11677,.T.);
#16315=ORIENTED_EDGE('',*,*,#11685,.T.);
#16316=ORIENTED_EDGE('',*,*,#11686,.F.);
#16317=ORIENTED_EDGE('',*,*,#11687,.F.);
#16318=ORIENTED_EDGE('',*,*,#11688,.F.);
#16319=ORIENTED_EDGE('',*,*,#11682,.T.);
#16320=ORIENTED_EDGE('',*,*,#11689,.T.);
#16321=ORIENTED_EDGE('',*,*,#11690,.T.);
#16322=ORIENTED_EDGE('',*,*,#11691,.F.);
#16323=ORIENTED_EDGE('',*,*,#11692,.F.);
#16324=ORIENTED_EDGE('',*,*,#11693,.F.);
#16325=ORIENTED_EDGE('',*,*,#11686,.T.);
#16326=ORIENTED_EDGE('',*,*,#11694,.T.);
#16327=ORIENTED_EDGE('',*,*,#11695,.T.);
#16328=ORIENTED_EDGE('',*,*,#11696,.F.);
#16329=ORIENTED_EDGE('',*,*,#11697,.F.);
#16330=ORIENTED_EDGE('',*,*,#11698,.F.);
#16331=ORIENTED_EDGE('',*,*,#11691,.T.);
#16332=ORIENTED_EDGE('',*,*,#11699,.T.);
#16333=ORIENTED_EDGE('',*,*,#11700,.F.);
#16334=ORIENTED_EDGE('',*,*,#11701,.F.);
#16335=ORIENTED_EDGE('',*,*,#11702,.F.);
#16336=ORIENTED_EDGE('',*,*,#11696,.T.);
#16337=ORIENTED_EDGE('',*,*,#11703,.T.);
#16338=ORIENTED_EDGE('',*,*,#11704,.T.);
#16339=ORIENTED_EDGE('',*,*,#11705,.F.);
#16340=ORIENTED_EDGE('',*,*,#11706,.F.);
#16341=ORIENTED_EDGE('',*,*,#11707,.F.);
#16342=ORIENTED_EDGE('',*,*,#11700,.T.);
#16343=ORIENTED_EDGE('',*,*,#11708,.T.);
#16344=ORIENTED_EDGE('',*,*,#11709,.F.);
#16345=ORIENTED_EDGE('',*,*,#11710,.F.);
#16346=ORIENTED_EDGE('',*,*,#11711,.F.);
#16347=ORIENTED_EDGE('',*,*,#11705,.T.);
#16348=ORIENTED_EDGE('',*,*,#11712,.T.);
#16349=ORIENTED_EDGE('',*,*,#11713,.T.);
#16350=ORIENTED_EDGE('',*,*,#11714,.F.);
#16351=ORIENTED_EDGE('',*,*,#11715,.F.);
#16352=ORIENTED_EDGE('',*,*,#11716,.F.);
#16353=ORIENTED_EDGE('',*,*,#11709,.T.);
#16354=ORIENTED_EDGE('',*,*,#11717,.T.);
#16355=ORIENTED_EDGE('',*,*,#11718,.T.);
#16356=ORIENTED_EDGE('',*,*,#11719,.F.);
#16357=ORIENTED_EDGE('',*,*,#11720,.F.);
#16358=ORIENTED_EDGE('',*,*,#11721,.F.);
#16359=ORIENTED_EDGE('',*,*,#11714,.T.);
#16360=ORIENTED_EDGE('',*,*,#11722,.T.);
#16361=ORIENTED_EDGE('',*,*,#11723,.T.);
#16362=ORIENTED_EDGE('',*,*,#11724,.F.);
#16363=ORIENTED_EDGE('',*,*,#11725,.F.);
#16364=ORIENTED_EDGE('',*,*,#11726,.F.);
#16365=ORIENTED_EDGE('',*,*,#11719,.T.);
#16366=ORIENTED_EDGE('',*,*,#11727,.T.);
#16367=ORIENTED_EDGE('',*,*,#11728,.T.);
#16368=ORIENTED_EDGE('',*,*,#11729,.T.);
#16369=ORIENTED_EDGE('',*,*,#11730,.T.);
#16370=ORIENTED_EDGE('',*,*,#11731,.T.);
#16371=ORIENTED_EDGE('',*,*,#11732,.T.);
#16372=ORIENTED_EDGE('',*,*,#11733,.T.);
#16373=ORIENTED_EDGE('',*,*,#11734,.T.);
#16374=ORIENTED_EDGE('',*,*,#11735,.T.);
#16375=ORIENTED_EDGE('',*,*,#11736,.T.);
#16376=ORIENTED_EDGE('',*,*,#11737,.T.);
#16377=ORIENTED_EDGE('',*,*,#11738,.T.);
#16378=ORIENTED_EDGE('',*,*,#11739,.T.);
#16379=ORIENTED_EDGE('',*,*,#11740,.T.);
#16380=ORIENTED_EDGE('',*,*,#11741,.T.);
#16381=ORIENTED_EDGE('',*,*,#11742,.T.);
#16382=ORIENTED_EDGE('',*,*,#11743,.T.);
#16383=ORIENTED_EDGE('',*,*,#11744,.T.);
#16384=ORIENTED_EDGE('',*,*,#11745,.T.);
#16385=ORIENTED_EDGE('',*,*,#11746,.T.);
#16386=ORIENTED_EDGE('',*,*,#11747,.T.);
#16387=ORIENTED_EDGE('',*,*,#11748,.T.);
#16388=ORIENTED_EDGE('',*,*,#11749,.T.);
#16389=ORIENTED_EDGE('',*,*,#11750,.T.);
#16390=ORIENTED_EDGE('',*,*,#11751,.T.);
#16391=ORIENTED_EDGE('',*,*,#11752,.T.);
#16392=ORIENTED_EDGE('',*,*,#11753,.T.);
#16393=ORIENTED_EDGE('',*,*,#11754,.T.);
#16394=ORIENTED_EDGE('',*,*,#11755,.T.);
#16395=ORIENTED_EDGE('',*,*,#11756,.T.);
#16396=ORIENTED_EDGE('',*,*,#11757,.T.);
#16397=ORIENTED_EDGE('',*,*,#11758,.T.);
#16398=ORIENTED_EDGE('',*,*,#11759,.T.);
#16399=ORIENTED_EDGE('',*,*,#11760,.T.);
#16400=ORIENTED_EDGE('',*,*,#11761,.T.);
#16401=ORIENTED_EDGE('',*,*,#11762,.T.);
#16402=ORIENTED_EDGE('',*,*,#11763,.T.);
#16403=ORIENTED_EDGE('',*,*,#11764,.T.);
#16404=ORIENTED_EDGE('',*,*,#11765,.T.);
#16405=ORIENTED_EDGE('',*,*,#11766,.T.);
#16406=ORIENTED_EDGE('',*,*,#11767,.T.);
#16407=ORIENTED_EDGE('',*,*,#11768,.T.);
#16408=ORIENTED_EDGE('',*,*,#11769,.T.);
#16409=ORIENTED_EDGE('',*,*,#11770,.T.);
#16410=ORIENTED_EDGE('',*,*,#11771,.F.);
#16411=ORIENTED_EDGE('',*,*,#11772,.T.);
#16412=ORIENTED_EDGE('',*,*,#11773,.T.);
#16413=ORIENTED_EDGE('',*,*,#11774,.T.);
#16414=ORIENTED_EDGE('',*,*,#11775,.T.);
#16415=ORIENTED_EDGE('',*,*,#11776,.T.);
#16416=ORIENTED_EDGE('',*,*,#11777,.T.);
#16417=ORIENTED_EDGE('',*,*,#11778,.T.);
#16418=ORIENTED_EDGE('',*,*,#11779,.T.);
#16419=ORIENTED_EDGE('',*,*,#11780,.T.);
#16420=ORIENTED_EDGE('',*,*,#11781,.T.);
#16421=ORIENTED_EDGE('',*,*,#11782,.T.);
#16422=ORIENTED_EDGE('',*,*,#11783,.T.);
#16423=ORIENTED_EDGE('',*,*,#11784,.T.);
#16424=ORIENTED_EDGE('',*,*,#11785,.T.);
#16425=ORIENTED_EDGE('',*,*,#11786,.T.);
#16426=ORIENTED_EDGE('',*,*,#11787,.T.);
#16427=ORIENTED_EDGE('',*,*,#11788,.T.);
#16428=ORIENTED_EDGE('',*,*,#11789,.T.);
#16429=ORIENTED_EDGE('',*,*,#11790,.T.);
#16430=ORIENTED_EDGE('',*,*,#11791,.T.);
#16431=ORIENTED_EDGE('',*,*,#11792,.T.);
#16432=ORIENTED_EDGE('',*,*,#11793,.T.);
#16433=ORIENTED_EDGE('',*,*,#11794,.T.);
#16434=ORIENTED_EDGE('',*,*,#11795,.T.);
#16435=ORIENTED_EDGE('',*,*,#11796,.T.);
#16436=ORIENTED_EDGE('',*,*,#11797,.T.);
#16437=ORIENTED_EDGE('',*,*,#11798,.T.);
#16438=ORIENTED_EDGE('',*,*,#11799,.T.);
#16439=ORIENTED_EDGE('',*,*,#11800,.T.);
#16440=ORIENTED_EDGE('',*,*,#11801,.T.);
#16441=ORIENTED_EDGE('',*,*,#11802,.T.);
#16442=ORIENTED_EDGE('',*,*,#11803,.T.);
#16443=ORIENTED_EDGE('',*,*,#11804,.T.);
#16444=ORIENTED_EDGE('',*,*,#11805,.T.);
#16445=ORIENTED_EDGE('',*,*,#11806,.T.);
#16446=ORIENTED_EDGE('',*,*,#11807,.T.);
#16447=ORIENTED_EDGE('',*,*,#11808,.T.);
#16448=ORIENTED_EDGE('',*,*,#11809,.T.);
#16449=ORIENTED_EDGE('',*,*,#11810,.T.);
#16450=ORIENTED_EDGE('',*,*,#11724,.T.);
#16451=ORIENTED_EDGE('',*,*,#11811,.T.);
#16452=ORIENTED_EDGE('',*,*,#11812,.T.);
#16453=ORIENTED_EDGE('',*,*,#11813,.F.);
#16454=ORIENTED_EDGE('',*,*,#11814,.F.);
#16455=ORIENTED_EDGE('',*,*,#11815,.F.);
#16456=ORIENTED_EDGE('',*,*,#11816,.F.);
#16457=ORIENTED_EDGE('',*,*,#11817,.T.);
#16458=ORIENTED_EDGE('',*,*,#11818,.T.);
#16459=ORIENTED_EDGE('',*,*,#11817,.F.);
#16460=ORIENTED_EDGE('',*,*,#11818,.F.);
#16461=ORIENTED_EDGE('',*,*,#11819,.F.);
#16462=ORIENTED_EDGE('',*,*,#11820,.T.);
#16463=ORIENTED_EDGE('',*,*,#11813,.T.);
#16464=ORIENTED_EDGE('',*,*,#11821,.T.);
#16465=ORIENTED_EDGE('',*,*,#11822,.F.);
#16466=ORIENTED_EDGE('',*,*,#11820,.F.);
#16467=ORIENTED_EDGE('',*,*,#11823,.F.);
#16468=ORIENTED_EDGE('',*,*,#11770,.F.);
#16469=ORIENTED_EDGE('',*,*,#11769,.F.);
#16470=ORIENTED_EDGE('',*,*,#11768,.F.);
#16471=ORIENTED_EDGE('',*,*,#11767,.F.);
#16472=ORIENTED_EDGE('',*,*,#11766,.F.);
#16473=ORIENTED_EDGE('',*,*,#11765,.F.);
#16474=ORIENTED_EDGE('',*,*,#11764,.F.);
#16475=ORIENTED_EDGE('',*,*,#11763,.F.);
#16476=ORIENTED_EDGE('',*,*,#11762,.F.);
#16477=ORIENTED_EDGE('',*,*,#11761,.F.);
#16478=ORIENTED_EDGE('',*,*,#11760,.F.);
#16479=ORIENTED_EDGE('',*,*,#11759,.F.);
#16480=ORIENTED_EDGE('',*,*,#11758,.F.);
#16481=ORIENTED_EDGE('',*,*,#11757,.F.);
#16482=ORIENTED_EDGE('',*,*,#11756,.F.);
#16483=ORIENTED_EDGE('',*,*,#11755,.F.);
#16484=ORIENTED_EDGE('',*,*,#11754,.F.);
#16485=ORIENTED_EDGE('',*,*,#11753,.F.);
#16486=ORIENTED_EDGE('',*,*,#11752,.F.);
#16487=ORIENTED_EDGE('',*,*,#11751,.F.);
#16488=ORIENTED_EDGE('',*,*,#11750,.F.);
#16489=ORIENTED_EDGE('',*,*,#11749,.F.);
#16490=ORIENTED_EDGE('',*,*,#11748,.F.);
#16491=ORIENTED_EDGE('',*,*,#11747,.F.);
#16492=ORIENTED_EDGE('',*,*,#11746,.F.);
#16493=ORIENTED_EDGE('',*,*,#11745,.F.);
#16494=ORIENTED_EDGE('',*,*,#11744,.F.);
#16495=ORIENTED_EDGE('',*,*,#11743,.F.);
#16496=ORIENTED_EDGE('',*,*,#11742,.F.);
#16497=ORIENTED_EDGE('',*,*,#11741,.F.);
#16498=ORIENTED_EDGE('',*,*,#11740,.F.);
#16499=ORIENTED_EDGE('',*,*,#11739,.F.);
#16500=ORIENTED_EDGE('',*,*,#11738,.F.);
#16501=ORIENTED_EDGE('',*,*,#11737,.F.);
#16502=ORIENTED_EDGE('',*,*,#11736,.F.);
#16503=ORIENTED_EDGE('',*,*,#11735,.F.);
#16504=ORIENTED_EDGE('',*,*,#11734,.F.);
#16505=ORIENTED_EDGE('',*,*,#11733,.F.);
#16506=ORIENTED_EDGE('',*,*,#11732,.F.);
#16507=ORIENTED_EDGE('',*,*,#11731,.F.);
#16508=ORIENTED_EDGE('',*,*,#11824,.F.);
#16509=ORIENTED_EDGE('',*,*,#11551,.T.);
#16510=ORIENTED_EDGE('',*,*,#11556,.T.);
#16511=ORIENTED_EDGE('',*,*,#11555,.T.);
#16512=ORIENTED_EDGE('',*,*,#11561,.T.);
#16513=ORIENTED_EDGE('',*,*,#11560,.T.);
#16514=ORIENTED_EDGE('',*,*,#11566,.T.);
#16515=ORIENTED_EDGE('',*,*,#11565,.T.);
#16516=ORIENTED_EDGE('',*,*,#11571,.T.);
#16517=ORIENTED_EDGE('',*,*,#11570,.T.);
#16518=ORIENTED_EDGE('',*,*,#11575,.T.);
#16519=ORIENTED_EDGE('',*,*,#11574,.T.);
#16520=ORIENTED_EDGE('',*,*,#11580,.T.);
#16521=ORIENTED_EDGE('',*,*,#11579,.T.);
#16522=ORIENTED_EDGE('',*,*,#11584,.T.);
#16523=ORIENTED_EDGE('',*,*,#11583,.T.);
#16524=ORIENTED_EDGE('',*,*,#11589,.T.);
#16525=ORIENTED_EDGE('',*,*,#11588,.T.);
#16526=ORIENTED_EDGE('',*,*,#11593,.T.);
#16527=ORIENTED_EDGE('',*,*,#11592,.T.);
#16528=ORIENTED_EDGE('',*,*,#11598,.T.);
#16529=ORIENTED_EDGE('',*,*,#11597,.T.);
#16530=ORIENTED_EDGE('',*,*,#11602,.T.);
#16531=ORIENTED_EDGE('',*,*,#11601,.T.);
#16532=ORIENTED_EDGE('',*,*,#11607,.T.);
#16533=ORIENTED_EDGE('',*,*,#11606,.T.);
#16534=ORIENTED_EDGE('',*,*,#11611,.T.);
#16535=ORIENTED_EDGE('',*,*,#11610,.T.);
#16536=ORIENTED_EDGE('',*,*,#11616,.T.);
#16537=ORIENTED_EDGE('',*,*,#11615,.T.);
#16538=ORIENTED_EDGE('',*,*,#11620,.T.);
#16539=ORIENTED_EDGE('',*,*,#11619,.T.);
#16540=ORIENTED_EDGE('',*,*,#11625,.T.);
#16541=ORIENTED_EDGE('',*,*,#11624,.T.);
#16542=ORIENTED_EDGE('',*,*,#11629,.T.);
#16543=ORIENTED_EDGE('',*,*,#11628,.T.);
#16544=ORIENTED_EDGE('',*,*,#11634,.T.);
#16545=ORIENTED_EDGE('',*,*,#11633,.T.);
#16546=ORIENTED_EDGE('',*,*,#11638,.T.);
#16547=ORIENTED_EDGE('',*,*,#11637,.T.);
#16548=ORIENTED_EDGE('',*,*,#11643,.T.);
#16549=ORIENTED_EDGE('',*,*,#11642,.T.);
#16550=ORIENTED_EDGE('',*,*,#11647,.T.);
#16551=ORIENTED_EDGE('',*,*,#11646,.T.);
#16552=ORIENTED_EDGE('',*,*,#11652,.T.);
#16553=ORIENTED_EDGE('',*,*,#11651,.T.);
#16554=ORIENTED_EDGE('',*,*,#11656,.T.);
#16555=ORIENTED_EDGE('',*,*,#11655,.T.);
#16556=ORIENTED_EDGE('',*,*,#11661,.T.);
#16557=ORIENTED_EDGE('',*,*,#11660,.T.);
#16558=ORIENTED_EDGE('',*,*,#11666,.T.);
#16559=ORIENTED_EDGE('',*,*,#11665,.T.);
#16560=ORIENTED_EDGE('',*,*,#11670,.T.);
#16561=ORIENTED_EDGE('',*,*,#11669,.T.);
#16562=ORIENTED_EDGE('',*,*,#11675,.T.);
#16563=ORIENTED_EDGE('',*,*,#11674,.T.);
#16564=ORIENTED_EDGE('',*,*,#11679,.T.);
#16565=ORIENTED_EDGE('',*,*,#11678,.T.);
#16566=ORIENTED_EDGE('',*,*,#11684,.T.);
#16567=ORIENTED_EDGE('',*,*,#11683,.T.);
#16568=ORIENTED_EDGE('',*,*,#11688,.T.);
#16569=ORIENTED_EDGE('',*,*,#11687,.T.);
#16570=ORIENTED_EDGE('',*,*,#11693,.T.);
#16571=ORIENTED_EDGE('',*,*,#11692,.T.);
#16572=ORIENTED_EDGE('',*,*,#11698,.T.);
#16573=ORIENTED_EDGE('',*,*,#11697,.T.);
#16574=ORIENTED_EDGE('',*,*,#11702,.T.);
#16575=ORIENTED_EDGE('',*,*,#11701,.T.);
#16576=ORIENTED_EDGE('',*,*,#11707,.T.);
#16577=ORIENTED_EDGE('',*,*,#11706,.T.);
#16578=ORIENTED_EDGE('',*,*,#11711,.T.);
#16579=ORIENTED_EDGE('',*,*,#11710,.T.);
#16580=ORIENTED_EDGE('',*,*,#11716,.T.);
#16581=ORIENTED_EDGE('',*,*,#11715,.T.);
#16582=ORIENTED_EDGE('',*,*,#11721,.T.);
#16583=ORIENTED_EDGE('',*,*,#11720,.T.);
#16584=ORIENTED_EDGE('',*,*,#11726,.T.);
#16585=ORIENTED_EDGE('',*,*,#11725,.T.);
#16586=ORIENTED_EDGE('',*,*,#11815,.T.);
#16587=ORIENTED_EDGE('',*,*,#11814,.T.);
#16588=ORIENTED_EDGE('',*,*,#11825,.T.);
#16589=ORIENTED_EDGE('',*,*,#11826,.T.);
#16590=ORIENTED_EDGE('',*,*,#11827,.T.);
#16591=ORIENTED_EDGE('',*,*,#11552,.T.);
#16592=ORIENTED_EDGE('',*,*,#11824,.T.);
#16593=ORIENTED_EDGE('',*,*,#11821,.F.);
#16594=ORIENTED_EDGE('',*,*,#11812,.F.);
#16595=ORIENTED_EDGE('',*,*,#11811,.F.);
#16596=ORIENTED_EDGE('',*,*,#11728,.F.);
#16597=ORIENTED_EDGE('',*,*,#11727,.F.);
#16598=ORIENTED_EDGE('',*,*,#11723,.F.);
#16599=ORIENTED_EDGE('',*,*,#11722,.F.);
#16600=ORIENTED_EDGE('',*,*,#11718,.F.);
#16601=ORIENTED_EDGE('',*,*,#11717,.F.);
#16602=ORIENTED_EDGE('',*,*,#11713,.F.);
#16603=ORIENTED_EDGE('',*,*,#11712,.F.);
#16604=ORIENTED_EDGE('',*,*,#11708,.F.);
#16605=ORIENTED_EDGE('',*,*,#11704,.F.);
#16606=ORIENTED_EDGE('',*,*,#11703,.F.);
#16607=ORIENTED_EDGE('',*,*,#11699,.F.);
#16608=ORIENTED_EDGE('',*,*,#11695,.F.);
#16609=ORIENTED_EDGE('',*,*,#11694,.F.);
#16610=ORIENTED_EDGE('',*,*,#11690,.F.);
#16611=ORIENTED_EDGE('',*,*,#11689,.F.);
#16612=ORIENTED_EDGE('',*,*,#11685,.F.);
#16613=ORIENTED_EDGE('',*,*,#11681,.F.);
#16614=ORIENTED_EDGE('',*,*,#11680,.F.);
#16615=ORIENTED_EDGE('',*,*,#11676,.F.);
#16616=ORIENTED_EDGE('',*,*,#11672,.F.);
#16617=ORIENTED_EDGE('',*,*,#11671,.F.);
#16618=ORIENTED_EDGE('',*,*,#11667,.F.);
#16619=ORIENTED_EDGE('',*,*,#11663,.F.);
#16620=ORIENTED_EDGE('',*,*,#11662,.F.);
#16621=ORIENTED_EDGE('',*,*,#11658,.F.);
#16622=ORIENTED_EDGE('',*,*,#11657,.F.);
#16623=ORIENTED_EDGE('',*,*,#11653,.F.);
#16624=ORIENTED_EDGE('',*,*,#11649,.F.);
#16625=ORIENTED_EDGE('',*,*,#11648,.F.);
#16626=ORIENTED_EDGE('',*,*,#11644,.F.);
#16627=ORIENTED_EDGE('',*,*,#11640,.F.);
#16628=ORIENTED_EDGE('',*,*,#11639,.F.);
#16629=ORIENTED_EDGE('',*,*,#11635,.F.);
#16630=ORIENTED_EDGE('',*,*,#11631,.F.);
#16631=ORIENTED_EDGE('',*,*,#11630,.F.);
#16632=ORIENTED_EDGE('',*,*,#11626,.F.);
#16633=ORIENTED_EDGE('',*,*,#11622,.F.);
#16634=ORIENTED_EDGE('',*,*,#11621,.F.);
#16635=ORIENTED_EDGE('',*,*,#11617,.F.);
#16636=ORIENTED_EDGE('',*,*,#11613,.F.);
#16637=ORIENTED_EDGE('',*,*,#11612,.F.);
#16638=ORIENTED_EDGE('',*,*,#11608,.F.);
#16639=ORIENTED_EDGE('',*,*,#11604,.F.);
#16640=ORIENTED_EDGE('',*,*,#11603,.F.);
#16641=ORIENTED_EDGE('',*,*,#11599,.F.);
#16642=ORIENTED_EDGE('',*,*,#11595,.F.);
#16643=ORIENTED_EDGE('',*,*,#11594,.F.);
#16644=ORIENTED_EDGE('',*,*,#11590,.F.);
#16645=ORIENTED_EDGE('',*,*,#11586,.F.);
#16646=ORIENTED_EDGE('',*,*,#11585,.F.);
#16647=ORIENTED_EDGE('',*,*,#11581,.F.);
#16648=ORIENTED_EDGE('',*,*,#11577,.F.);
#16649=ORIENTED_EDGE('',*,*,#11576,.F.);
#16650=ORIENTED_EDGE('',*,*,#11572,.F.);
#16651=ORIENTED_EDGE('',*,*,#11568,.F.);
#16652=ORIENTED_EDGE('',*,*,#11567,.F.);
#16653=ORIENTED_EDGE('',*,*,#11563,.F.);
#16654=ORIENTED_EDGE('',*,*,#11562,.F.);
#16655=ORIENTED_EDGE('',*,*,#11558,.F.);
#16656=ORIENTED_EDGE('',*,*,#11557,.F.);
#16657=ORIENTED_EDGE('',*,*,#11553,.F.);
#16658=ORIENTED_EDGE('',*,*,#11827,.F.);
#16659=ORIENTED_EDGE('',*,*,#11828,.T.);
#16660=ORIENTED_EDGE('',*,*,#11729,.F.);
#16661=ORIENTED_EDGE('',*,*,#11810,.F.);
#16662=ORIENTED_EDGE('',*,*,#11809,.F.);
#16663=ORIENTED_EDGE('',*,*,#11808,.F.);
#16664=ORIENTED_EDGE('',*,*,#11807,.F.);
#16665=ORIENTED_EDGE('',*,*,#11806,.F.);
#16666=ORIENTED_EDGE('',*,*,#11805,.F.);
#16667=ORIENTED_EDGE('',*,*,#11804,.F.);
#16668=ORIENTED_EDGE('',*,*,#11803,.F.);
#16669=ORIENTED_EDGE('',*,*,#11802,.F.);
#16670=ORIENTED_EDGE('',*,*,#11801,.F.);
#16671=ORIENTED_EDGE('',*,*,#11800,.F.);
#16672=ORIENTED_EDGE('',*,*,#11799,.F.);
#16673=ORIENTED_EDGE('',*,*,#11798,.F.);
#16674=ORIENTED_EDGE('',*,*,#11797,.F.);
#16675=ORIENTED_EDGE('',*,*,#11796,.F.);
#16676=ORIENTED_EDGE('',*,*,#11795,.F.);
#16677=ORIENTED_EDGE('',*,*,#11794,.F.);
#16678=ORIENTED_EDGE('',*,*,#11793,.F.);
#16679=ORIENTED_EDGE('',*,*,#11792,.F.);
#16680=ORIENTED_EDGE('',*,*,#11791,.F.);
#16681=ORIENTED_EDGE('',*,*,#11790,.F.);
#16682=ORIENTED_EDGE('',*,*,#11789,.F.);
#16683=ORIENTED_EDGE('',*,*,#11788,.F.);
#16684=ORIENTED_EDGE('',*,*,#11787,.F.);
#16685=ORIENTED_EDGE('',*,*,#11786,.F.);
#16686=ORIENTED_EDGE('',*,*,#11785,.F.);
#16687=ORIENTED_EDGE('',*,*,#11784,.F.);
#16688=ORIENTED_EDGE('',*,*,#11783,.F.);
#16689=ORIENTED_EDGE('',*,*,#11782,.F.);
#16690=ORIENTED_EDGE('',*,*,#11781,.F.);
#16691=ORIENTED_EDGE('',*,*,#11780,.F.);
#16692=ORIENTED_EDGE('',*,*,#11779,.F.);
#16693=ORIENTED_EDGE('',*,*,#11778,.F.);
#16694=ORIENTED_EDGE('',*,*,#11777,.F.);
#16695=ORIENTED_EDGE('',*,*,#11776,.F.);
#16696=ORIENTED_EDGE('',*,*,#11775,.F.);
#16697=ORIENTED_EDGE('',*,*,#11774,.F.);
#16698=ORIENTED_EDGE('',*,*,#11773,.F.);
#16699=ORIENTED_EDGE('',*,*,#11772,.F.);
#16700=ORIENTED_EDGE('',*,*,#11829,.F.);
#16701=ORIENTED_EDGE('',*,*,#11816,.T.);
#16702=ORIENTED_EDGE('',*,*,#11828,.F.);
#16703=ORIENTED_EDGE('',*,*,#11826,.F.);
#16704=ORIENTED_EDGE('',*,*,#11830,.T.);
#16705=ORIENTED_EDGE('',*,*,#11829,.T.);
#16706=ORIENTED_EDGE('',*,*,#11830,.F.);
#16707=ORIENTED_EDGE('',*,*,#11825,.F.);
#16708=ORIENTED_EDGE('',*,*,#11730,.F.);
#16709=ORIENTED_EDGE('',*,*,#11819,.T.);
#16710=ORIENTED_EDGE('',*,*,#11831,.T.);
#16711=ORIENTED_EDGE('',*,*,#11832,.F.);
#16712=ORIENTED_EDGE('',*,*,#11831,.F.);
#16713=ORIENTED_EDGE('',*,*,#11822,.T.);
#16714=ORIENTED_EDGE('',*,*,#11771,.T.);
#16715=ORIENTED_EDGE('',*,*,#11823,.T.);
#16716=ORIENTED_EDGE('',*,*,#11833,.F.);
#16717=ORIENTED_EDGE('',*,*,#11834,.T.);
#16718=ORIENTED_EDGE('',*,*,#11832,.T.);
#16719=ORIENTED_EDGE('',*,*,#11834,.F.);
#16720=ORIENTED_EDGE('',*,*,#11835,.F.);
#16721=ORIENTED_EDGE('',*,*,#11833,.T.);
#16722=ORIENTED_EDGE('',*,*,#11836,.F.);
#16723=ORIENTED_EDGE('',*,*,#11837,.T.);
#16724=ORIENTED_EDGE('',*,*,#11835,.T.);
#16725=ORIENTED_EDGE('',*,*,#11837,.F.);
#16726=ORIENTED_EDGE('',*,*,#11836,.T.);
#16727=ORIENTED_EDGE('',*,*,#11838,.F.);
#16728=ORIENTED_EDGE('',*,*,#11839,.F.);
#16729=ORIENTED_EDGE('',*,*,#11840,.T.);
#16730=ORIENTED_EDGE('',*,*,#11838,.T.);
#16731=ORIENTED_EDGE('',*,*,#11840,.F.);
#16732=ORIENTED_EDGE('',*,*,#11839,.T.);
#16733=ORIENTED_EDGE('',*,*,#11841,.T.);
#16734=ORIENTED_EDGE('',*,*,#11842,.F.);
#16735=ORIENTED_EDGE('',*,*,#11841,.F.);
#16736=ORIENTED_EDGE('',*,*,#11842,.T.);
#18933=B_SPLINE_SURFACE_WITH_KNOTS('',3,3,((#88758,#88759,#88760,#88761,
#88762,#88763,#88764,#88765,#88766,#88767,#88768,#88769,#88770,#88771,#88772,
#88773,#88774,#88775,#88776,#88777,#88778,#88779,#88780,#88781,#88782,#88783,
#88784,#88785,#88786,#88787,#88788,#88789,#88790,#88791,#88792,#88793,#88794,
#88795,#88796,#88797,#88798,#88799,#88800,#88801,#88802,#88803,#88804,#88805,
#88806,#88807,#88808,#88809,#88810,#88811,#88812,#88813,#88814,#88815,#88816,
#88817,#88818,#88819,#88820,#88821,#88822,#88823,#88824,#88825,#88826,#88827,
#88828,#88829,#88830,#88831,#88832,#88833,#88834,#88835,#88836,#88837,#88838,
#88839,#88840,#88841,#88842,#88843,#88844,#88845,#88846,#88847,#88848,#88849,
#88850,#88851,#88852,#88853,#88854,#88855,#88856,#88857,#88858,#88859,#88860,
#88861,#88862,#88863,#88864,#88865,#88866,#88867,#88868,#88869,#88870,#88871,
#88872,#88873,#88874,#88875,#88876,#88877,#88878,#88879,#88880,#88881,#88882,
#88883,#88884,#88885,#88886,#88887,#88888,#88889,#88890,#88891,#88892,#88893,
#88894,#88895,#88896,#88897,#88898,#88899,#88900,#88901,#88902,#88903,#88904,
#88905,#88906,#88907,#88908,#88909,#88910,#88911,#88912,#88913,#88914,#88915,
#88916,#88917,#88918,#88919,#88920,#88921,#88922,#88923,#88924,#88925,#88926,
#88927,#88928,#88929,#88930,#88931,#88932,#88933,#88934,#88935,#88936,#88937,
#88938,#88939,#88940,#88941,#88942,#88943,#88944,#88945,#88946,#88947,#88948,
#88949,#88950,#88951,#88952,#88953,#88954,#88955,#88956,#88957,#88958,#88959,
#88960,#88961,#88962,#88963,#88964,#88965,#88966,#88967,#88968,#88969,#88970,
#88971,#88972,#88973,#88974,#88975,#88976,#88977,#88978,#88979,#88980,#88981,
#88982,#88983,#88984,#88985,#88986,#88987,#88988,#88989,#88990,#88991,#88992,
#88993,#88994,#88995,#88996,#88997,#88998,#88999,#89000,#89001,#89002,#89003,
#89004,#89005,#89006,#89007),(#89008,#89009,#89010,#89011,#89012,#89013,
#89014,#89015,#89016,#89017,#89018,#89019,#89020,#89021,#89022,#89023,#89024,
#89025,#89026,#89027,#89028,#89029,#89030,#89031,#89032,#89033,#89034,#89035,
#89036,#89037,#89038,#89039,#89040,#89041,#89042,#89043,#89044,#89045,#89046,
#89047,#89048,#89049,#89050,#89051,#89052,#89053,#89054,#89055,#89056,#89057,
#89058,#89059,#89060,#89061,#89062,#89063,#89064,#89065,#89066,#89067,#89068,
#89069,#89070,#89071,#89072,#89073,#89074,#89075,#89076,#89077,#89078,#89079,
#89080,#89081,#89082,#89083,#89084,#89085,#89086,#89087,#89088,#89089,#89090,
#89091,#89092,#89093,#89094,#89095,#89096,#89097,#89098,#89099,#89100,#89101,
#89102,#89103,#89104,#89105,#89106,#89107,#89108,#89109,#89110,#89111,#89112,
#89113,#89114,#89115,#89116,#89117,#89118,#89119,#89120,#89121,#89122,#89123,
#89124,#89125,#89126,#89127,#89128,#89129,#89130,#89131,#89132,#89133,#89134,
#89135,#89136,#89137,#89138,#89139,#89140,#89141,#89142,#89143,#89144,#89145,
#89146,#89147,#89148,#89149,#89150,#89151,#89152,#89153,#89154,#89155,#89156,
#89157,#89158,#89159,#89160,#89161,#89162,#89163,#89164,#89165,#89166,#89167,
#89168,#89169,#89170,#89171,#89172,#89173,#89174,#89175,#89176,#89177,#89178,
#89179,#89180,#89181,#89182,#89183,#89184,#89185,#89186,#89187,#89188,#89189,
#89190,#89191,#89192,#89193,#89194,#89195,#89196,#89197,#89198,#89199,#89200,
#89201,#89202,#89203,#89204,#89205,#89206,#89207,#89208,#89209,#89210,#89211,
#89212,#89213,#89214,#89215,#89216,#89217,#89218,#89219,#89220,#89221,#89222,
#89223,#89224,#89225,#89226,#89227,#89228,#89229,#89230,#89231,#89232,#89233,
#89234,#89235,#89236,#89237,#89238,#89239,#89240,#89241,#89242,#89243,#89244,
#89245,#89246,#89247,#89248,#89249,#89250,#89251,#89252,#89253,#89254,#89255,
#89256,#89257),(#89258,#89259,#89260,#89261,#89262,#89263,#89264,#89265,
#89266,#89267,#89268,#89269,#89270,#89271,#89272,#89273,#89274,#89275,#89276,
#89277,#89278,#89279,#89280,#89281,#89282,#89283,#89284,#89285,#89286,#89287,
#89288,#89289,#89290,#89291,#89292,#89293,#89294,#89295,#89296,#89297,#89298,
#89299,#89300,#89301,#89302,#89303,#89304,#89305,#89306,#89307,#89308,#89309,
#89310,#89311,#89312,#89313,#89314,#89315,#89316,#89317,#89318,#89319,#89320,
#89321,#89322,#89323,#89324,#89325,#89326,#89327,#89328,#89329,#89330,#89331,
#89332,#89333,#89334,#89335,#89336,#89337,#89338,#89339,#89340,#89341,#89342,
#89343,#89344,#89345,#89346,#89347,#89348,#89349,#89350,#89351,#89352,#89353,
#89354,#89355,#89356,#89357,#89358,#89359,#89360,#89361,#89362,#89363,#89364,
#89365,#89366,#89367,#89368,#89369,#89370,#89371,#89372,#89373,#89374,#89375,
#89376,#89377,#89378,#89379,#89380,#89381,#89382,#89383,#89384,#89385,#89386,
#89387,#89388,#89389,#89390,#89391,#89392,#89393,#89394,#89395,#89396,#89397,
#89398,#89399,#89400,#89401,#89402,#89403,#89404,#89405,#89406,#89407,#89408,
#89409,#89410,#89411,#89412,#89413,#89414,#89415,#89416,#89417,#89418,#89419,
#89420,#89421,#89422,#89423,#89424,#89425,#89426,#89427,#89428,#89429,#89430,
#89431,#89432,#89433,#89434,#89435,#89436,#89437,#89438,#89439,#89440,#89441,
#89442,#89443,#89444,#89445,#89446,#89447,#89448,#89449,#89450,#89451,#89452,
#89453,#89454,#89455,#89456,#89457,#89458,#89459,#89460,#89461,#89462,#89463,
#89464,#89465,#89466,#89467,#89468,#89469,#89470,#89471,#89472,#89473,#89474,
#89475,#89476,#89477,#89478,#89479,#89480,#89481,#89482,#89483,#89484,#89485,
#89486,#89487,#89488,#89489,#89490,#89491,#89492,#89493,#89494,#89495,#89496,
#89497,#89498,#89499,#89500,#89501,#89502,#89503,#89504,#89505,#89506,#89507),
(#89508,#89509,#89510,#89511,#89512,#89513,#89514,#89515,#89516,#89517,
#89518,#89519,#89520,#89521,#89522,#89523,#89524,#89525,#89526,#89527,#89528,
#89529,#89530,#89531,#89532,#89533,#89534,#89535,#89536,#89537,#89538,#89539,
#89540,#89541,#89542,#89543,#89544,#89545,#89546,#89547,#89548,#89549,#89550,
#89551,#89552,#89553,#89554,#89555,#89556,#89557,#89558,#89559,#89560,#89561,
#89562,#89563,#89564,#89565,#89566,#89567,#89568,#89569,#89570,#89571,#89572,
#89573,#89574,#89575,#89576,#89577,#89578,#89579,#89580,#89581,#89582,#89583,
#89584,#89585,#89586,#89587,#89588,#89589,#89590,#89591,#89592,#89593,#89594,
#89595,#89596,#89597,#89598,#89599,#89600,#89601,#89602,#89603,#89604,#89605,
#89606,#89607,#89608,#89609,#89610,#89611,#89612,#89613,#89614,#89615,#89616,
#89617,#89618,#89619,#89620,#89621,#89622,#89623,#89624,#89625,#89626,#89627,
#89628,#89629,#89630,#89631,#89632,#89633,#89634,#89635,#89636,#89637,#89638,
#89639,#89640,#89641,#89642,#89643,#89644,#89645,#89646,#89647,#89648,#89649,
#89650,#89651,#89652,#89653,#89654,#89655,#89656,#89657,#89658,#89659,#89660,
#89661,#89662,#89663,#89664,#89665,#89666,#89667,#89668,#89669,#89670,#89671,
#89672,#89673,#89674,#89675,#89676,#89677,#89678,#89679,#89680,#89681,#89682,
#89683,#89684,#89685,#89686,#89687,#89688,#89689,#89690,#89691,#89692,#89693,
#89694,#89695,#89696,#89697,#89698,#89699,#89700,#89701,#89702,#89703,#89704,
#89705,#89706,#89707,#89708,#89709,#89710,#89711,#89712,#89713,#89714,#89715,
#89716,#89717,#89718,#89719,#89720,#89721,#89722,#89723,#89724,#89725,#89726,
#89727,#89728,#89729,#89730,#89731,#89732,#89733,#89734,#89735,#89736,#89737,
#89738,#89739,#89740,#89741,#89742,#89743,#89744,#89745,#89746,#89747,#89748,
#89749,#89750,#89751,#89752,#89753,#89754,#89755,#89756,#89757)),
 .UNSPECIFIED.,.F.,.F.,.F.,(4,4),(4,1,1,1,1,1,1,1,1,1,1,1,1,1,1,1,1,1,1,
1,1,1,1,1,1,1,1,1,1,1,1,1,1,1,1,1,1,1,1,1,1,1,1,1,1,1,1,1,1,1,1,1,1,1,1,
1,1,1,1,1,1,1,1,1,1,1,1,1,1,1,1,1,1,1,1,1,1,1,1,1,1,1,1,1,1,1,1,1,1,1,1,
1,1,1,1,1,1,1,1,1,1,1,1,1,1,1,1,1,1,1,1,1,1,1,1,1,1,1,1,1,1,1,1,1,1,1,1,
1,1,1,1,1,1,1,1,1,1,1,1,1,1,1,1,1,1,1,1,1,1,1,1,1,1,1,1,1,1,1,1,1,1,1,1,
1,1,1,1,1,1,1,1,1,1,1,1,1,1,1,1,1,1,1,1,1,1,1,1,1,1,1,1,1,1,1,1,1,1,1,1,
1,1,1,1,1,1,1,1,1,1,1,1,1,1,1,1,1,1,1,1,1,1,1,1,1,1,1,1,1,1,1,1,1,1,1,1,
1,1,1,1,1,1,1,1,1,1,1,1,4),(-0.000536156821677024,0.0823575402511902),(8.31473274985828,
9.31424788838504,10.3137630269118,11.3132781654386,12.3127933039653,13.3123084424921,
14.3118235810189,15.3113387195456,16.3108538580724,17.3103689965991,18.3098841351259,
19.3093992736527,20.3089144121794,21.3084295507062,22.307944689233,23.3074598277597,
24.3069749662865,25.3064901048132,26.30600524334,27.3055203818668,28.3050355203935,
29.3045506589203,30.3040657974471,31.3035809359738,32.3030960745006,33.3026112130273,
34.3021263515541,35.3016414900809,36.3011566286076,37.3006717671344,38.3001869056612,
39.2997020441879,40.2992171827147,41.2987323212414,42.2982474597682,43.297762598295,
44.2972777368217,45.2967928753485,46.2963080138753,47.295823152402,48.2953382909288,
49.2948534294556,50.2943685679823,51.2938837065091,52.2933988450358,53.2929139835626,
54.2924291220894,55.2919442606161,56.2914593991429,57.2909745376696,58.2904896761964,
59.2900048147232,60.2895199532499,61.2890350917767,62.2885502303035,63.2880653688302,
64.287580507357,65.2870956458838,66.2866107844105,67.2861259229373,68.285641061464,
69.2851561999908,70.2846713385176,71.2841864770443,72.2837016155711,73.2832167540979,
74.2827318926246,75.2822470311514,76.2817621696781,77.2812773082049,78.2807924467317,
79.2803075852584,80.2798227237852,81.2793378623119,82.2788530008387,83.2783681393655,
84.2778832778922,85.277398416419,86.2769135549458,87.2764286934725,88.2759438319993,
89.2754589705261,90.2749741090528,91.2744892475796,92.2740043861063,93.2735195246331,
94.2730346631599,95.2725498016866,96.2720649402134,97.2715800787402,98.2710952172669,
99.2706103557937,100.27012549432,101.269640632847,102.269155771374,103.268670909901,
104.268186048427,105.267701186954,106.267216325481,107.266731464008,108.266246602535,
109.265761741061,110.265276879588,111.264792018115,112.264307156642,113.263822295168,
114.263337433695,115.262852572222,116.262367710749,117.261882849275,118.261397987802,
119.260913126329,120.260428264856,121.259943403382,122.259458541909,123.258973680436,
124.258488818963,125.25800395749,126.257519096016,127.257034234543,128.25654937307,
129.256064511597,130.255579650123,131.25509478865,132.254609927177,133.254125065704,
134.25364020423,135.253155342757,136.252670481284,137.252185619811,138.251700758337,
139.251215896864,140.250731035391,141.250246173918,142.249761312444,143.249276450971,
144.248791589498,145.248306728025,146.247821866552,147.247337005078,148.246852143605,
149.246367282132,150.245882420659,151.245397559185,152.244912697712,153.244427836239,
154.243942974766,155.243458113292,156.242973251819,157.242488390346,158.242003528873,
159.241518667399,160.241033805926,161.240548944453,162.24006408298,163.239579221506,
164.239094360033,165.23860949856,166.238124637087,167.237639775614,168.23715491414,
169.236670052667,170.236185191194,171.235700329721,172.235215468247,173.234730606774,
174.234245745301,175.233760883828,176.233276022354,177.232791160881,178.232306299408,
179.231821437935,180.231336576461,181.230851714988,182.230366853515,183.229881992042,
184.229397130569,185.228912269095,186.228427407622,187.227942546149,188.227457684676,
189.226972823202,190.226487961729,191.226003100256,192.225518238783,193.225033377309,
194.224548515836,195.224063654363,196.22357879289,197.223093931416,198.222609069943,
199.22212420847,200.221639346997,201.221154485523,202.22066962405,203.220184762577,
204.219699901104,205.219215039631,206.218730178157,207.218245316684,208.217760455211,
209.217275593738,210.216790732264,211.216305870791,212.215821009318,213.215336147845,
214.214851286371,215.214366424898,216.213881563425,217.213396701952,218.212911840478,
219.212426979005,220.211942117532,221.211457256059,222.210972394585,223.210487533112,
224.210002671639,225.209517810166,226.209032948693,227.208548087219,228.208063225746,
229.207578364273,230.2070935028,231.206608641326,232.206123779853,233.20563891838,
234.205154056907,235.204669195433,236.20418433396,237.203699472487,238.203214611014,
239.20272974954,240.202244888067,241.201760026594,242.201275165121,243.200790303647,
244.200305442174,245.199820580701,246.199335719228,247.198850857755,248.198365996281,
249.197881134808,250.197396273335,251.196911411862,252.196426550388,253.195941688915,
254.195456827442,255.194971965969),.UNSPECIFIED.);
#18934=B_SPLINE_SURFACE_WITH_KNOTS('',3,3,((#89946,#89947,#89948,#89949,
#89950,#89951,#89952,#89953,#89954,#89955,#89956,#89957,#89958,#89959,#89960,
#89961,#89962,#89963,#89964,#89965,#89966,#89967,#89968,#89969,#89970,#89971,
#89972,#89973,#89974,#89975,#89976,#89977,#89978,#89979,#89980,#89981,#89982,
#89983,#89984,#89985,#89986,#89987,#89988,#89989,#89990,#89991,#89992,#89993,
#89994,#89995,#89996,#89997,#89998,#89999,#90000,#90001,#90002,#90003,#90004,
#90005,#90006,#90007,#90008,#90009,#90010,#90011,#90012,#90013,#90014,#90015,
#90016,#90017,#90018,#90019,#90020,#90021,#90022,#90023,#90024,#90025,#90026,
#90027,#90028,#90029,#90030,#90031,#90032,#90033,#90034,#90035,#90036,#90037,
#90038,#90039,#90040,#90041,#90042,#90043,#90044,#90045,#90046,#90047,#90048,
#90049,#90050,#90051,#90052,#90053,#90054,#90055,#90056,#90057,#90058,#90059,
#90060,#90061,#90062,#90063,#90064,#90065,#90066,#90067,#90068,#90069,#90070,
#90071,#90072,#90073,#90074,#90075,#90076,#90077,#90078,#90079,#90080,#90081,
#90082,#90083,#90084,#90085,#90086,#90087,#90088,#90089,#90090,#90091,#90092,
#90093,#90094,#90095,#90096,#90097,#90098,#90099,#90100,#90101,#90102,#90103,
#90104,#90105,#90106,#90107,#90108,#90109,#90110,#90111,#90112,#90113,#90114,
#90115,#90116,#90117,#90118,#90119,#90120,#90121,#90122,#90123,#90124,#90125,
#90126,#90127,#90128,#90129,#90130,#90131,#90132,#90133,#90134,#90135,#90136,
#90137,#90138,#90139,#90140,#90141,#90142,#90143,#90144,#90145,#90146,#90147,
#90148,#90149,#90150,#90151,#90152,#90153,#90154,#90155,#90156,#90157,#90158,
#90159,#90160,#90161,#90162,#90163,#90164,#90165,#90166,#90167,#90168,#90169,
#90170,#90171,#90172,#90173,#90174,#90175,#90176,#90177,#90178,#90179,#90180,
#90181,#90182,#90183,#90184,#90185,#90186,#90187,#90188,#90189,#90190,#90191,
#90192,#90193,#90194,#90195),(#90196,#90197,#90198,#90199,#90200,#90201,
#90202,#90203,#90204,#90205,#90206,#90207,#90208,#90209,#90210,#90211,#90212,
#90213,#90214,#90215,#90216,#90217,#90218,#90219,#90220,#90221,#90222,#90223,
#90224,#90225,#90226,#90227,#90228,#90229,#90230,#90231,#90232,#90233,#90234,
#90235,#90236,#90237,#90238,#90239,#90240,#90241,#90242,#90243,#90244,#90245,
#90246,#90247,#90248,#90249,#90250,#90251,#90252,#90253,#90254,#90255,#90256,
#90257,#90258,#90259,#90260,#90261,#90262,#90263,#90264,#90265,#90266,#90267,
#90268,#90269,#90270,#90271,#90272,#90273,#90274,#90275,#90276,#90277,#90278,
#90279,#90280,#90281,#90282,#90283,#90284,#90285,#90286,#90287,#90288,#90289,
#90290,#90291,#90292,#90293,#90294,#90295,#90296,#90297,#90298,#90299,#90300,
#90301,#90302,#90303,#90304,#90305,#90306,#90307,#90308,#90309,#90310,#90311,
#90312,#90313,#90314,#90315,#90316,#90317,#90318,#90319,#90320,#90321,#90322,
#90323,#90324,#90325,#90326,#90327,#90328,#90329,#90330,#90331,#90332,#90333,
#90334,#90335,#90336,#90337,#90338,#90339,#90340,#90341,#90342,#90343,#90344,
#90345,#90346,#90347,#90348,#90349,#90350,#90351,#90352,#90353,#90354,#90355,
#90356,#90357,#90358,#90359,#90360,#90361,#90362,#90363,#90364,#90365,#90366,
#90367,#90368,#90369,#90370,#90371,#90372,#90373,#90374,#90375,#90376,#90377,
#90378,#90379,#90380,#90381,#90382,#90383,#90384,#90385,#90386,#90387,#90388,
#90389,#90390,#90391,#90392,#90393,#90394,#90395,#90396,#90397,#90398,#90399,
#90400,#90401,#90402,#90403,#90404,#90405,#90406,#90407,#90408,#90409,#90410,
#90411,#90412,#90413,#90414,#90415,#90416,#90417,#90418,#90419,#90420,#90421,
#90422,#90423,#90424,#90425,#90426,#90427,#90428,#90429,#90430,#90431,#90432,
#90433,#90434,#90435,#90436,#90437,#90438,#90439,#90440,#90441,#90442,#90443,
#90444,#90445),(#90446,#90447,#90448,#90449,#90450,#90451,#90452,#90453,
#90454,#90455,#90456,#90457,#90458,#90459,#90460,#90461,#90462,#90463,#90464,
#90465,#90466,#90467,#90468,#90469,#90470,#90471,#90472,#90473,#90474,#90475,
#90476,#90477,#90478,#90479,#90480,#90481,#90482,#90483,#90484,#90485,#90486,
#90487,#90488,#90489,#90490,#90491,#90492,#90493,#90494,#90495,#90496,#90497,
#90498,#90499,#90500,#90501,#90502,#90503,#90504,#90505,#90506,#90507,#90508,
#90509,#90510,#90511,#90512,#90513,#90514,#90515,#90516,#90517,#90518,#90519,
#90520,#90521,#90522,#90523,#90524,#90525,#90526,#90527,#90528,#90529,#90530,
#90531,#90532,#90533,#90534,#90535,#90536,#90537,#90538,#90539,#90540,#90541,
#90542,#90543,#90544,#90545,#90546,#90547,#90548,#90549,#90550,#90551,#90552,
#90553,#90554,#90555,#90556,#90557,#90558,#90559,#90560,#90561,#90562,#90563,
#90564,#90565,#90566,#90567,#90568,#90569,#90570,#90571,#90572,#90573,#90574,
#90575,#90576,#90577,#90578,#90579,#90580,#90581,#90582,#90583,#90584,#90585,
#90586,#90587,#90588,#90589,#90590,#90591,#90592,#90593,#90594,#90595,#90596,
#90597,#90598,#90599,#90600,#90601,#90602,#90603,#90604,#90605,#90606,#90607,
#90608,#90609,#90610,#90611,#90612,#90613,#90614,#90615,#90616,#90617,#90618,
#90619,#90620,#90621,#90622,#90623,#90624,#90625,#90626,#90627,#90628,#90629,
#90630,#90631,#90632,#90633,#90634,#90635,#90636,#90637,#90638,#90639,#90640,
#90641,#90642,#90643,#90644,#90645,#90646,#90647,#90648,#90649,#90650,#90651,
#90652,#90653,#90654,#90655,#90656,#90657,#90658,#90659,#90660,#90661,#90662,
#90663,#90664,#90665,#90666,#90667,#90668,#90669,#90670,#90671,#90672,#90673,
#90674,#90675,#90676,#90677,#90678,#90679,#90680,#90681,#90682,#90683,#90684,
#90685,#90686,#90687,#90688,#90689,#90690,#90691,#90692,#90693,#90694,#90695),
(#90696,#90697,#90698,#90699,#90700,#90701,#90702,#90703,#90704,#90705,
#90706,#90707,#90708,#90709,#90710,#90711,#90712,#90713,#90714,#90715,#90716,
#90717,#90718,#90719,#90720,#90721,#90722,#90723,#90724,#90725,#90726,#90727,
#90728,#90729,#90730,#90731,#90732,#90733,#90734,#90735,#90736,#90737,#90738,
#90739,#90740,#90741,#90742,#90743,#90744,#90745,#90746,#90747,#90748,#90749,
#90750,#90751,#90752,#90753,#90754,#90755,#90756,#90757,#90758,#90759,#90760,
#90761,#90762,#90763,#90764,#90765,#90766,#90767,#90768,#90769,#90770,#90771,
#90772,#90773,#90774,#90775,#90776,#90777,#90778,#90779,#90780,#90781,#90782,
#90783,#90784,#90785,#90786,#90787,#90788,#90789,#90790,#90791,#90792,#90793,
#90794,#90795,#90796,#90797,#90798,#90799,#90800,#90801,#90802,#90803,#90804,
#90805,#90806,#90807,#90808,#90809,#90810,#90811,#90812,#90813,#90814,#90815,
#90816,#90817,#90818,#90819,#90820,#90821,#90822,#90823,#90824,#90825,#90826,
#90827,#90828,#90829,#90830,#90831,#90832,#90833,#90834,#90835,#90836,#90837,
#90838,#90839,#90840,#90841,#90842,#90843,#90844,#90845,#90846,#90847,#90848,
#90849,#90850,#90851,#90852,#90853,#90854,#90855,#90856,#90857,#90858,#90859,
#90860,#90861,#90862,#90863,#90864,#90865,#90866,#90867,#90868,#90869,#90870,
#90871,#90872,#90873,#90874,#90875,#90876,#90877,#90878,#90879,#90880,#90881,
#90882,#90883,#90884,#90885,#90886,#90887,#90888,#90889,#90890,#90891,#90892,
#90893,#90894,#90895,#90896,#90897,#90898,#90899,#90900,#90901,#90902,#90903,
#90904,#90905,#90906,#90907,#90908,#90909,#90910,#90911,#90912,#90913,#90914,
#90915,#90916,#90917,#90918,#90919,#90920,#90921,#90922,#90923,#90924,#90925,
#90926,#90927,#90928,#90929,#90930,#90931,#90932,#90933,#90934,#90935,#90936,
#90937,#90938,#90939,#90940,#90941,#90942,#90943,#90944,#90945)),
 .UNSPECIFIED.,.F.,.F.,.F.,(4,4),(4,1,1,1,1,1,1,1,1,1,1,1,1,1,1,1,1,1,1,
1,1,1,1,1,1,1,1,1,1,1,1,1,1,1,1,1,1,1,1,1,1,1,1,1,1,1,1,1,1,1,1,1,1,1,1,
1,1,1,1,1,1,1,1,1,1,1,1,1,1,1,1,1,1,1,1,1,1,1,1,1,1,1,1,1,1,1,1,1,1,1,1,
1,1,1,1,1,1,1,1,1,1,1,1,1,1,1,1,1,1,1,1,1,1,1,1,1,1,1,1,1,1,1,1,1,1,1,1,
1,1,1,1,1,1,1,1,1,1,1,1,1,1,1,1,1,1,1,1,1,1,1,1,1,1,1,1,1,1,1,1,1,1,1,1,
1,1,1,1,1,1,1,1,1,1,1,1,1,1,1,1,1,1,1,1,1,1,1,1,1,1,1,1,1,1,1,1,1,1,1,1,
1,1,1,1,1,1,1,1,1,1,1,1,1,1,1,1,1,1,1,1,1,1,1,1,1,1,1,1,1,1,1,1,1,1,1,1,
1,1,1,1,1,1,1,1,1,1,1,1,4),(-0.000330323912087073,0.0826817882439028),(11.6145450452496,
12.6147293662818,13.6142445048086,14.6137596433353,15.6132747818621,16.6127899203889,
17.6123050589156,18.6118201974424,19.6113353359692,20.6108504744959,21.6103656130227,
22.6098807515494,23.6093958900762,24.608911028603,25.6084261671297,26.6079413056565,
27.6074564441833,28.60697158271,29.6064867212368,30.6060018597635,31.6055169982903,
32.6050321368171,33.6045472753438,34.6040624138706,35.6035775523974,36.6030926909241,
37.6026078294509,38.6021229679776,39.6016381065044,40.6011532450312,41.6006683835579,
42.6001835220847,43.5996986606115,44.5992137991382,45.598728937665,46.5982440761917,
47.5977592147185,48.5972743532453,49.596789491772,50.5963046302988,51.5958197688256,
52.5953349073523,53.5948500458791,54.5943651844058,55.5938803229326,56.5933954614594,
57.5929105999861,58.5924257385129,59.5919408770397,60.5914560155664,61.5909711540932,
62.5904862926199,63.5900014311467,64.5895165696735,65.5890317082002,66.588546846727,
67.5880619852538,68.5875771237805,69.5870922623073,70.5866074008341,71.5861225393608,
72.5856376778876,73.5851528164143,74.5846679549411,75.5841830934679,76.5836982319946,
77.5832133705214,78.5827285090482,79.5822436475749,80.5817587861017,81.5812739246284,
82.5807890631552,83.580304201682,84.5798193402087,85.5793344787355,86.5788496172623,
87.578364755789,88.5778798943158,89.5773950328425,90.5769101713693,91.5764253098961,
92.5759404484228,93.5754555869496,94.5749707254764,95.5744858640031,96.5740010025299,
97.5735161410566,98.5730312795834,99.5725464181102,100.572061556637,101.571576695164,
102.57109183369,103.570606972217,104.570122110744,105.569637249271,106.569152387798,
107.568667526324,108.568182664851,109.567697803378,110.567212941905,111.566728080431,
112.566243218958,113.565758357485,114.565273496012,115.564788634538,116.564303773065,
117.563818911592,118.563334050119,119.562849188645,120.562364327172,121.561879465699,
122.561394604226,123.560909742752,124.560424881279,125.559940019806,126.559455158333,
127.55897029686,128.558485435386,129.558000573913,130.55751571244,131.557030850967,
132.556545989493,133.55606112802,134.555576266547,135.555091405074,136.5546065436,
137.554121682127,138.553636820654,139.553151959181,140.552667097707,141.552182236234,
142.551697374761,143.551212513288,144.550727651814,145.550242790341,146.549757928868,
147.549273067395,148.548788205922,149.548303344448,150.547818482975,151.547333621502,
152.546848760029,153.546363898555,154.545879037082,155.545394175609,156.544909314136,
157.544424452662,158.543939591189,159.543454729716,160.542969868243,161.542485006769,
162.542000145296,163.541515283823,164.54103042235,165.540545560876,166.540060699403,
167.53957583793,168.539090976457,169.538606114984,170.53812125351,171.537636392037,
172.537151530564,173.536666669091,174.536181807617,175.535696946144,176.535212084671,
177.534727223198,178.534242361724,179.533757500251,180.533272638778,181.532787777305,
182.532302915831,183.531818054358,184.531333192885,185.530848331412,186.530363469939,
187.529878608465,188.529393746992,189.528908885519,190.528424024046,191.527939162572,
192.527454301099,193.526969439626,194.526484578153,195.525999716679,196.525514855206,
197.525029993733,198.52454513226,199.524060270786,200.523575409313,201.52309054784,
202.522605686367,203.522120824893,204.52163596342,205.521151101947,206.520666240474,
207.520181379001,208.519696517527,209.519211656054,210.518726794581,211.518241933108,
212.517757071634,213.517272210161,214.516787348688,215.516302487215,216.515817625741,
217.515332764268,218.514847902795,219.514363041322,220.513878179848,221.513393318375,
222.512908456902,223.512423595429,224.511938733956,225.511453872482,226.510969011009,
227.510484149536,228.509999288063,229.509514426589,230.509029565116,231.508544703643,
232.50805984217,233.507574980696,234.507090119223,235.50660525775,236.506120396277,
237.505635534803,238.50515067333,239.504665811857,240.504180950384,241.50369608891,
242.503211227437,243.502726365964,244.502241504491,245.501756643018,246.501271781544,
247.500786920071,248.500302058598,249.499817197125,250.499332335651,251.498847474178,
252.498362612705,253.497877751232,254.497392889758,255.496908028285,256.496423166812,
257.495938305339,258.495453443865),.UNSPECIFIED.);
#19617=ADVANCED_FACE('',(#5683),#4817,.T.);
#19618=ADVANCED_FACE('',(#5684),#4818,.T.);
#19619=ADVANCED_FACE('',(#5685),#4819,.T.);
#19620=ADVANCED_FACE('',(#5686),#4820,.T.);
#19621=ADVANCED_FACE('',(#5687),#4821,.T.);
#19622=ADVANCED_FACE('',(#5688),#4822,.T.);
#19623=ADVANCED_FACE('',(#5689),#4823,.T.);
#19624=ADVANCED_FACE('',(#5690),#4824,.T.);
#19625=ADVANCED_FACE('',(#5691),#4825,.T.);
#19626=ADVANCED_FACE('',(#5692),#4826,.T.);
#19627=ADVANCED_FACE('',(#5693),#4827,.T.);
#19628=ADVANCED_FACE('',(#5694),#4828,.T.);
#19629=ADVANCED_FACE('',(#5695),#4829,.T.);
#19630=ADVANCED_FACE('',(#5696),#4830,.T.);
#19631=ADVANCED_FACE('',(#5697),#4831,.T.);
#19632=ADVANCED_FACE('',(#5698),#4832,.T.);
#19633=ADVANCED_FACE('',(#5699),#4833,.T.);
#19634=ADVANCED_FACE('',(#5700),#4834,.T.);
#19635=ADVANCED_FACE('',(#5701),#4835,.T.);
#19636=ADVANCED_FACE('',(#5702),#4836,.T.);
#19637=ADVANCED_FACE('',(#5703),#4837,.T.);
#19638=ADVANCED_FACE('',(#5704),#4838,.T.);
#19639=ADVANCED_FACE('',(#5705),#4839,.T.);
#19640=ADVANCED_FACE('',(#5706),#4840,.T.);
#19641=ADVANCED_FACE('',(#5707),#4841,.T.);
#19642=ADVANCED_FACE('',(#5708),#4842,.T.);
#19643=ADVANCED_FACE('',(#5709),#4843,.T.);
#19644=ADVANCED_FACE('',(#5710),#4844,.T.);
#19645=ADVANCED_FACE('',(#5711),#4845,.T.);
#19646=ADVANCED_FACE('',(#5712),#4846,.T.);
#19647=ADVANCED_FACE('',(#5713),#4847,.T.);
#19648=ADVANCED_FACE('',(#5714),#4848,.T.);
#19649=ADVANCED_FACE('',(#5715),#4849,.T.);
#19650=ADVANCED_FACE('',(#5716),#4850,.T.);
#19651=ADVANCED_FACE('',(#5717),#4851,.T.);
#19652=ADVANCED_FACE('',(#5718),#4852,.T.);
#19653=ADVANCED_FACE('',(#5719),#4853,.T.);
#19654=ADVANCED_FACE('',(#5720),#4854,.T.);
#19655=ADVANCED_FACE('',(#5721),#4855,.T.);
#19656=ADVANCED_FACE('',(#5722),#4856,.T.);
#19657=ADVANCED_FACE('',(#5723),#4857,.T.);
#19658=ADVANCED_FACE('',(#5724),#4858,.F.);
#19659=ADVANCED_FACE('',(#5725),#1522,.F.);
#19660=ADVANCED_FACE('',(#5726),#1523,.F.);
#19661=ADVANCED_FACE('',(#5727),#18933,.F.);
#19662=ADVANCED_FACE('',(#5728),#1524,.T.);
#19663=ADVANCED_FACE('',(#5729),#18934,.F.);
#19664=ADVANCED_FACE('',(#5730,#1757),#1525,.T.);
#19665=ADVANCED_FACE('',(#5731),#232,.T.);
#19666=ADVANCED_FACE('',(#5732),#233,.T.);
#19667=ADVANCED_FACE('',(#5733),#4859,.T.);
#19668=ADVANCED_FACE('',(#5734,#1758),#1526,.T.);
#19669=ADVANCED_FACE('',(#5735),#4860,.T.);
#19670=ADVANCED_FACE('',(#5736,#1759),#1527,.T.);
#19671=ADVANCED_FACE('',(#5737),#4861,.T.);
#19672=ADVANCED_FACE('',(#5738),#234,.T.);
#19673=ADVANCED_FACE('',(#5739),#1528,.T.);
#20122=CLOSED_SHELL('',(#19617,#19618,#19619,#19620,#19621,#19622,#19623,
#19624,#19625,#19626,#19627,#19628,#19629,#19630,#19631,#19632,#19633,#19634,
#19635,#19636,#19637,#19638,#19639,#19640,#19641,#19642,#19643,#19644,#19645,
#19646,#19647,#19648,#19649,#19650,#19651,#19652,#19653,#19654,#19655,#19656,
#19657,#19658,#19659,#19660,#19661,#19662,#19663,#19664,#19665,#19666,#19667,
#19668,#19669,#19670,#19671,#19672,#19673));
#21537=AXIS2_PLACEMENT_3D('',#61990,#25691,#25692);
#21538=AXIS2_PLACEMENT_3D('',#61991,#25693,#25694);
#21539=AXIS2_PLACEMENT_3D('',#62106,#25696,#25697);
#21540=AXIS2_PLACEMENT_3D('',#62174,#25698,#25699);
#21541=AXIS2_PLACEMENT_3D('',#62604,#25701,#25702);
#21542=AXIS2_PLACEMENT_3D('',#63031,#25704,#25705);
#21543=AXIS2_PLACEMENT_3D('',#63487,#25707,#25708);
#21544=AXIS2_PLACEMENT_3D('',#63951,#25710,#25711);
#21545=AXIS2_PLACEMENT_3D('',#64294,#25713,#25714);
#21546=AXIS2_PLACEMENT_3D('',#64692,#25716,#25717);
#21547=AXIS2_PLACEMENT_3D('',#65025,#25719,#25720);
#21548=AXIS2_PLACEMENT_3D('',#65417,#25722,#25723);
#21549=AXIS2_PLACEMENT_3D('',#65800,#25725,#25726);
#21550=AXIS2_PLACEMENT_3D('',#66199,#25728,#25729);
#21551=AXIS2_PLACEMENT_3D('',#66755,#25731,#25732);
#21552=AXIS2_PLACEMENT_3D('',#67216,#25734,#25735);
#21553=AXIS2_PLACEMENT_3D('',#67746,#25737,#25738);
#21554=AXIS2_PLACEMENT_3D('',#68199,#25740,#25741);
#21555=AXIS2_PLACEMENT_3D('',#68738,#25743,#25744);
#21556=AXIS2_PLACEMENT_3D('',#69200,#25746,#25747);
#21557=AXIS2_PLACEMENT_3D('',#69711,#25749,#25750);
#21558=AXIS2_PLACEMENT_3D('',#70194,#25752,#25753);
#21559=AXIS2_PLACEMENT_3D('',#70658,#25755,#25756);
#21560=AXIS2_PLACEMENT_3D('',#71125,#25758,#25759);
#21561=AXIS2_PLACEMENT_3D('',#71589,#25761,#25762);
#21562=AXIS2_PLACEMENT_3D('',#72041,#25764,#25765);
#21563=AXIS2_PLACEMENT_3D('',#72527,#25767,#25768);
#21564=AXIS2_PLACEMENT_3D('',#72980,#25770,#25771);
#21565=AXIS2_PLACEMENT_3D('',#73453,#25773,#25774);
#21566=AXIS2_PLACEMENT_3D('',#73921,#25776,#25777);
#21567=AXIS2_PLACEMENT_3D('',#74393,#25779,#25780);
#21568=AXIS2_PLACEMENT_3D('',#74855,#25782,#25783);
#21569=AXIS2_PLACEMENT_3D('',#75315,#25785,#25786);
#21570=AXIS2_PLACEMENT_3D('',#75801,#25788,#25789);
#21571=AXIS2_PLACEMENT_3D('',#76258,#25791,#25792);
#21572=AXIS2_PLACEMENT_3D('',#76729,#25794,#25795);
#21573=AXIS2_PLACEMENT_3D('',#77191,#25797,#25798);
#21574=AXIS2_PLACEMENT_3D('',#77652,#25800,#25801);
#21575=AXIS2_PLACEMENT_3D('',#78089,#25803,#25804);
#21576=AXIS2_PLACEMENT_3D('',#78385,#25806,#25807);
#21577=AXIS2_PLACEMENT_3D('',#78745,#25809,#25810);
#21578=AXIS2_PLACEMENT_3D('',#79047,#25812,#25813);
#21579=AXIS2_PLACEMENT_3D('',#79124,#25814,#25815);
#21580=AXIS2_PLACEMENT_3D('',#84052,#25816,#25817);
#21581=AXIS2_PLACEMENT_3D('',#88373,#25818,#25819);
#21582=AXIS2_PLACEMENT_3D('',#88453,#25820,#25821);
#21583=AXIS2_PLACEMENT_3D('',#88558,#25822,#25823);
#21584=AXIS2_PLACEMENT_3D('',#88560,#25824,#25825);
#21585=AXIS2_PLACEMENT_3D('',#88563,#25827,#25828);
#21586=AXIS2_PLACEMENT_3D('',#88564,#25829,#25830);
#21587=AXIS2_PLACEMENT_3D('',#88565,#25831,#25832);
#21588=AXIS2_PLACEMENT_3D('',#88568,#25833,#25834);
#21589=AXIS2_PLACEMENT_3D('',#88757,#25835,#25836);
#21590=AXIS2_PLACEMENT_3D('',#89856,#25837,#25838);
#21591=AXIS2_PLACEMENT_3D('',#89858,#25839,#25840);
#21592=AXIS2_PLACEMENT_3D('',#89860,#25841,#25842);
#21593=AXIS2_PLACEMENT_3D('',#90950,#25843,#25844);
#21594=AXIS2_PLACEMENT_3D('',#90952,#25845,#25846);
#21595=AXIS2_PLACEMENT_3D('',#90953,#25847,#25848);
#21596=AXIS2_PLACEMENT_3D('',#90955,#25850,#25851);
#21597=AXIS2_PLACEMENT_3D('',#90958,#25853,#25854);
#21598=AXIS2_PLACEMENT_3D('',#90959,#25855,#25856);
#21599=AXIS2_PLACEMENT_3D('',#90961,#25857,#25858);
#21600=AXIS2_PLACEMENT_3D('',#90963,#25860,#25861);
#21601=AXIS2_PLACEMENT_3D('',#90965,#25862,#25863);
#21602=AXIS2_PLACEMENT_3D('',#90966,#25864,#25865);
#21603=AXIS2_PLACEMENT_3D('',#90968,#25866,#25867);
#21604=AXIS2_PLACEMENT_3D('',#90970,#25869,#25870);
#21605=AXIS2_PLACEMENT_3D('',#90972,#25871,#25872);
#21606=AXIS2_PLACEMENT_3D('',#90973,#25873,#25874);
#21607=AXIS2_PLACEMENT_3D('',#90975,#25875,#25876);
#21608=AXIS2_PLACEMENT_3D('',#90977,#25878,#25879);
#21609=AXIS2_PLACEMENT_3D('',#90980,#25881,#25882);
#21610=AXIS2_PLACEMENT_3D('',#90981,#25883,#25884);
#25691=DIRECTION('axis',(0.,0.,1.));
#25692=DIRECTION('refdir',(1.,0.,0.));
#25693=DIRECTION('center_axis',(1.,0.,0.));
#25694=DIRECTION('ref_axis',(0.,-0.555251325848433,-0.831682610821915));
#25695=DIRECTION('',(-1.,0.,0.));
#25696=DIRECTION('center_axis',(-1.,0.,0.));
#25697=DIRECTION('ref_axis',(0.,1.,-3.76905526341366E-13));
#25698=DIRECTION('center_axis',(1.,0.,0.));
#25699=DIRECTION('ref_axis',(0.,-0.555251325848433,-0.831682610821915));
#25700=DIRECTION('',(-1.,0.,0.));
#25701=DIRECTION('center_axis',(1.,0.,0.));
#25702=DIRECTION('ref_axis',(0.,-0.555251325848433,-0.831682610821915));
#25703=DIRECTION('',(-1.,0.,0.));
#25704=DIRECTION('center_axis',(1.,0.,0.));
#25705=DIRECTION('ref_axis',(0.,-0.555251325848433,-0.831682610821915));
#25706=DIRECTION('',(-1.,0.,0.));
#25707=DIRECTION('center_axis',(1.,0.,0.));
#25708=DIRECTION('ref_axis',(0.,-0.555251325848433,-0.831682610821915));
#25709=DIRECTION('',(-1.,0.,0.));
#25710=DIRECTION('center_axis',(1.,0.,0.));
#25711=DIRECTION('ref_axis',(0.,-0.555251325848433,-0.831682610821915));
#25712=DIRECTION('',(-1.,0.,0.));
#25713=DIRECTION('center_axis',(1.,0.,0.));
#25714=DIRECTION('ref_axis',(0.,-0.555251325848433,-0.831682610821915));
#25715=DIRECTION('',(-1.,0.,0.));
#25716=DIRECTION('center_axis',(1.,0.,0.));
#25717=DIRECTION('ref_axis',(0.,-0.555251325848433,-0.831682610821915));
#25718=DIRECTION('',(-1.,0.,0.));
#25719=DIRECTION('center_axis',(1.,0.,0.));
#25720=DIRECTION('ref_axis',(0.,-0.555251325848433,-0.831682610821915));
#25721=DIRECTION('',(-1.,0.,0.));
#25722=DIRECTION('center_axis',(1.,0.,0.));
#25723=DIRECTION('ref_axis',(0.,-0.555251325848433,-0.831682610821915));
#25724=DIRECTION('',(-1.,0.,0.));
#25725=DIRECTION('center_axis',(1.,0.,0.));
#25726=DIRECTION('ref_axis',(0.,-0.555251325848433,-0.831682610821915));
#25727=DIRECTION('',(-1.,0.,0.));
#25728=DIRECTION('center_axis',(1.,0.,0.));
#25729=DIRECTION('ref_axis',(0.,-0.555251325848433,-0.831682610821915));
#25730=DIRECTION('',(-1.,0.,0.));
#25731=DIRECTION('center_axis',(1.,0.,0.));
#25732=DIRECTION('ref_axis',(0.,-0.555251325848433,-0.831682610821915));
#25733=DIRECTION('',(-1.,0.,0.));
#25734=DIRECTION('center_axis',(1.,0.,0.));
#25735=DIRECTION('ref_axis',(0.,-0.555251325848433,-0.831682610821915));
#25736=DIRECTION('',(-1.,0.,0.));
#25737=DIRECTION('center_axis',(1.,0.,0.));
#25738=DIRECTION('ref_axis',(0.,-0.555251325848433,-0.831682610821915));
#25739=DIRECTION('',(-1.,0.,0.));
#25740=DIRECTION('center_axis',(1.,0.,0.));
#25741=DIRECTION('ref_axis',(0.,-0.555251325848433,-0.831682610821915));
#25742=DIRECTION('',(-1.,0.,0.));
#25743=DIRECTION('center_axis',(1.,0.,0.));
#25744=DIRECTION('ref_axis',(0.,-0.555251325848433,-0.831682610821915));
#25745=DIRECTION('',(-1.,0.,0.));
#25746=DIRECTION('center_axis',(1.,0.,0.));
#25747=DIRECTION('ref_axis',(0.,-0.555251325848433,-0.831682610821915));
#25748=DIRECTION('',(-1.,0.,0.));
#25749=DIRECTION('center_axis',(1.,0.,0.));
#25750=DIRECTION('ref_axis',(0.,-0.555251325848433,-0.831682610821915));
#25751=DIRECTION('',(-1.,0.,0.));
#25752=DIRECTION('center_axis',(1.,0.,0.));
#25753=DIRECTION('ref_axis',(0.,-0.555251325848433,-0.831682610821915));
#25754=DIRECTION('',(-1.,0.,0.));
#25755=DIRECTION('center_axis',(1.,0.,0.));
#25756=DIRECTION('ref_axis',(0.,-0.555251325848433,-0.831682610821915));
#25757=DIRECTION('',(-1.,0.,0.));
#25758=DIRECTION('center_axis',(1.,0.,0.));
#25759=DIRECTION('ref_axis',(0.,-0.555251325848433,-0.831682610821915));
#25760=DIRECTION('',(-1.,0.,0.));
#25761=DIRECTION('center_axis',(1.,0.,0.));
#25762=DIRECTION('ref_axis',(0.,-0.555251325848433,-0.831682610821915));
#25763=DIRECTION('',(-1.,0.,0.));
#25764=DIRECTION('center_axis',(1.,0.,0.));
#25765=DIRECTION('ref_axis',(0.,-0.555251325848433,-0.831682610821915));
#25766=DIRECTION('',(-1.,0.,0.));
#25767=DIRECTION('center_axis',(1.,0.,0.));
#25768=DIRECTION('ref_axis',(0.,-0.555251325848433,-0.831682610821915));
#25769=DIRECTION('',(-1.,0.,0.));
#25770=DIRECTION('center_axis',(1.,0.,0.));
#25771=DIRECTION('ref_axis',(0.,-0.555251325848433,-0.831682610821915));
#25772=DIRECTION('',(-1.,0.,0.));
#25773=DIRECTION('center_axis',(1.,0.,0.));
#25774=DIRECTION('ref_axis',(0.,-0.555251325848433,-0.831682610821915));
#25775=DIRECTION('',(-1.,0.,0.));
#25776=DIRECTION('center_axis',(1.,0.,0.));
#25777=DIRECTION('ref_axis',(0.,-0.555251325848433,-0.831682610821915));
#25778=DIRECTION('',(-1.,0.,0.));
#25779=DIRECTION('center_axis',(1.,0.,0.));
#25780=DIRECTION('ref_axis',(0.,-0.555251325848433,-0.831682610821915));
#25781=DIRECTION('',(-1.,0.,0.));
#25782=DIRECTION('center_axis',(1.,0.,0.));
#25783=DIRECTION('ref_axis',(0.,-0.555251325848433,-0.831682610821915));
#25784=DIRECTION('',(-1.,0.,0.));
#25785=DIRECTION('center_axis',(1.,0.,0.));
#25786=DIRECTION('ref_axis',(0.,-0.555251325848433,-0.831682610821915));
#25787=DIRECTION('',(-1.,0.,0.));
#25788=DIRECTION('center_axis',(1.,0.,0.));
#25789=DIRECTION('ref_axis',(0.,-0.555251325848433,-0.831682610821915));
#25790=DIRECTION('',(-1.,0.,0.));
#25791=DIRECTION('center_axis',(1.,0.,0.));
#25792=DIRECTION('ref_axis',(0.,-0.555251325848433,-0.831682610821915));
#25793=DIRECTION('',(-1.,0.,0.));
#25794=DIRECTION('center_axis',(1.,0.,0.));
#25795=DIRECTION('ref_axis',(0.,-0.555251325848433,-0.831682610821915));
#25796=DIRECTION('',(-1.,0.,0.));
#25797=DIRECTION('center_axis',(1.,0.,0.));
#25798=DIRECTION('ref_axis',(0.,-0.555251325848433,-0.831682610821915));
#25799=DIRECTION('',(-1.,0.,0.));
#25800=DIRECTION('center_axis',(1.,0.,0.));
#25801=DIRECTION('ref_axis',(0.,-0.555251325848433,-0.831682610821915));
#25802=DIRECTION('',(-1.,0.,0.));
#25803=DIRECTION('center_axis',(1.,0.,0.));
#25804=DIRECTION('ref_axis',(0.,-0.555251325848433,-0.831682610821915));
#25805=DIRECTION('',(-1.,0.,0.));
#25806=DIRECTION('center_axis',(1.,0.,0.));
#25807=DIRECTION('ref_axis',(0.,-0.555251325848433,-0.831682610821915));
#25808=DIRECTION('',(-1.,0.,0.));
#25809=DIRECTION('center_axis',(1.,0.,0.));
#25810=DIRECTION('ref_axis',(0.,-0.555251325848433,-0.831682610821915));
#25811=DIRECTION('',(-1.,0.,0.));
#25812=DIRECTION('center_axis',(1.,0.,0.));
#25813=DIRECTION('ref_axis',(0.,1.,0.));
#25814=DIRECTION('center_axis',(1.,0.,0.));
#25815=DIRECTION('ref_axis',(0.,1.,0.));
#25816=DIRECTION('center_axis',(-1.,0.,0.));
#25817=DIRECTION('ref_axis',(0.,1.,0.));
#25818=DIRECTION('center_axis',(1.,0.,0.));
#25819=DIRECTION('ref_axis',(0.,-0.555251325848433,-0.831682610821915));
#25820=DIRECTION('center_axis',(1.,0.,0.));
#25821=DIRECTION('ref_axis',(0.,1.,-3.76905526341366E-13));
#25822=DIRECTION('center_axis',(1.,0.,0.));
#25823=DIRECTION('ref_axis',(0.,0.,-1.));
#25824=DIRECTION('center_axis',(1.,0.,0.));
#25825=DIRECTION('ref_axis',(0.,0.,-1.));
#25826=DIRECTION('',(1.,0.,0.));
#25827=DIRECTION('center_axis',(1.,0.,0.));
#25828=DIRECTION('ref_axis',(0.,0.,-1.));
#25829=DIRECTION('center_axis',(1.,0.,0.));
#25830=DIRECTION('ref_axis',(0.,0.,-1.));
#25831=DIRECTION('center_axis',(1.,0.,0.));
#25832=DIRECTION('ref_axis',(0.,0.,-1.));
#25833=DIRECTION('center_axis',(-1.,0.,0.));
#25834=DIRECTION('ref_axis',(0.,1.,0.));
#25835=DIRECTION('center_axis',(-1.,0.,0.));
#25836=DIRECTION('ref_axis',(0.,1.,0.));
#25837=DIRECTION('center_axis',(1.,0.,0.));
#25838=DIRECTION('ref_axis',(0.,0.,-1.));
#25839=DIRECTION('center_axis',(1.,0.,0.));
#25840=DIRECTION('ref_axis',(0.,1.,0.));
#25841=DIRECTION('center_axis',(1.,0.,0.));
#25842=DIRECTION('ref_axis',(0.,1.,0.));
#25843=DIRECTION('center_axis',(-1.,0.,0.));
#25844=DIRECTION('ref_axis',(0.,0.,1.));
#25845=DIRECTION('center_axis',(1.,0.,0.));
#25846=DIRECTION('ref_axis',(0.,0.,-1.));
#25847=DIRECTION('center_axis',(1.,0.,0.));
#25848=DIRECTION('ref_axis',(0.,1.,0.));
#25849=DIRECTION('',(-0.707106781186548,0.707106781186547,8.65956056235493E-17));
#25850=DIRECTION('center_axis',(-1.,0.,0.));
#25851=DIRECTION('ref_axis',(0.,1.,0.));
#25852=DIRECTION('',(0.707106781186546,0.707106781186549,-8.65956056235495E-17));
#25853=DIRECTION('center_axis',(1.,0.,0.));
#25854=DIRECTION('ref_axis',(0.,0.,-1.));
#25855=DIRECTION('center_axis',(1.,0.,0.));
#25856=DIRECTION('ref_axis',(0.,1.,0.));
#25857=DIRECTION('center_axis',(1.,0.,0.));
#25858=DIRECTION('ref_axis',(0.,0.,-1.));
#25859=DIRECTION('',(-1.,0.,0.));
#25860=DIRECTION('center_axis',(-1.,0.,0.));
#25861=DIRECTION('ref_axis',(0.,0.,1.));
#25862=DIRECTION('center_axis',(1.,0.,0.));
#25863=DIRECTION('ref_axis',(0.,0.,-1.));
#25864=DIRECTION('center_axis',(1.,0.,0.));
#25865=DIRECTION('ref_axis',(0.,1.,0.));
#25866=DIRECTION('center_axis',(1.,0.,0.));
#25867=DIRECTION('ref_axis',(0.,0.,-1.));
#25868=DIRECTION('',(-1.,0.,0.));
#25869=DIRECTION('center_axis',(1.,0.,0.));
#25870=DIRECTION('ref_axis',(0.,0.,-1.));
#25871=DIRECTION('center_axis',(1.,0.,0.));
#25872=DIRECTION('ref_axis',(0.,0.,-1.));
#25873=DIRECTION('center_axis',(1.,0.,0.));
#25874=DIRECTION('ref_axis',(0.,1.,0.));
#25875=DIRECTION('center_axis',(1.,0.,0.));
#25876=DIRECTION('ref_axis',(0.,0.,-1.));
#25877=DIRECTION('',(-1.,0.,0.));
#25878=DIRECTION('center_axis',(-1.,0.,0.));
#25879=DIRECTION('ref_axis',(0.,1.,0.));
#25880=DIRECTION('',(0.707106781186547,0.707106781186548,-8.65956056235494E-17));
#25881=DIRECTION('center_axis',(1.,0.,0.));
#25882=DIRECTION('ref_axis',(0.,0.,-1.));
#25883=DIRECTION('center_axis',(1.,0.,0.));
#25884=DIRECTION('ref_axis',(0.,0.,-1.));
#61990=CARTESIAN_POINT('',(0.,0.,0.));
#61991=CARTESIAN_POINT('Origin',(-1.72497344927317,0.,0.));
#61992=CARTESIAN_POINT('',(1.21707771886868,1.78943621037804,2.68030513402633));
#61993=CARTESIAN_POINT('',(0.970338898719273,1.78943621037804,2.68030513402633));
#61994=CARTESIAN_POINT('',(-1.72497344927317,1.78943621037804,2.68030513402633));
#61995=CARTESIAN_POINT('',(0.58586766091457,-1.87152408986075,-2.62364539211588));
#61996=CARTESIAN_POINT('Ctrl Pts',(0.58586766091457,-1.87152408986075,-2.62364539211588));
#61997=CARTESIAN_POINT('Ctrl Pts',(0.59198764571749,-1.79127517131912,-2.68088932633323));
#61998=CARTESIAN_POINT('Ctrl Pts',(0.59810763052041,-1.70824895664009,-2.73455380169506));
#61999=CARTESIAN_POINT('Ctrl Pts',(0.60422761532333,-1.62280149583887,-2.78435501824088));
#62000=CARTESIAN_POINT('Ctrl Pts',(0.61033956178225,-1.53746626670259,-2.83409082297227));
#62001=CARTESIAN_POINT('Ctrl Pts',(0.616451508241169,-1.44971648895612,
-2.87997323007931));
#62002=CARTESIAN_POINT('Ctrl Pts',(0.622563454700089,-1.35993908319214,
-2.92176030031667));
#62003=CARTESIAN_POINT('Ctrl Pts',(0.62880158690121,-1.2683081552065,-2.9644100961207));
#62004=CARTESIAN_POINT('Ctrl Pts',(0.635039719102331,-1.17456531372328,
-3.00279328572004));
#62005=CARTESIAN_POINT('Ctrl Pts',(0.641277851303452,-1.07915085300422,
-3.03670067655017));
#62006=CARTESIAN_POINT('Ctrl Pts',(0.647379645712096,-0.985821727530616,
-3.06986700280113));
#62007=CARTESIAN_POINT('Ctrl Pts',(0.65348144012074,-0.89089374539159,-3.09875102118765));
#62008=CARTESIAN_POINT('Ctrl Pts',(0.659583234529385,-0.794800091963228,
-3.12320514476959));
#62009=CARTESIAN_POINT('Ctrl Pts',(0.665683183521829,-0.698735500934035,
-3.14765187248848));
#62010=CARTESIAN_POINT('Ctrl Pts',(0.671783132514273,-0.601506367318778,
-3.16767125788266));
#62011=CARTESIAN_POINT('Ctrl Pts',(0.677883081506717,-0.503560139985367,
-3.18316583732578));
#62012=CARTESIAN_POINT('Ctrl Pts',(0.683982884505863,-0.405616256850698,
-3.19866004592895));
#62013=CARTESIAN_POINT('Ctrl Pts',(0.690082687505009,-0.30695575120951,
-3.20962959565981));
#62014=CARTESIAN_POINT('Ctrl Pts',(0.696182490504155,-0.208034236627888,
-3.21602850094502));
#62015=CARTESIAN_POINT('Ctrl Pts',(0.702523835256058,-0.105195599473501,
-3.22268079192129));
#62016=CARTESIAN_POINT('Ctrl Pts',(0.708865180007961,-0.00207536863801527,
-3.22439290423859));
#62017=CARTESIAN_POINT('Ctrl Pts',(0.715206524759864,0.100812806682847,
-3.22117282065224));
#62018=CARTESIAN_POINT('Ctrl Pts',(0.721314650644506,0.19991701115185,-3.21807116372079));
#62019=CARTESIAN_POINT('Ctrl Pts',(0.727422776529149,0.29880548247049,-3.21039382167964));
#62020=CARTESIAN_POINT('Ctrl Pts',(0.733530902413792,0.397024509110286,
-3.19820091640062));
#62021=CARTESIAN_POINT('Ctrl Pts',(0.739643164081569,0.495310039388279,
-3.18599975536312));
#62022=CARTESIAN_POINT('Ctrl Pts',(0.745755425749347,0.59292478846357,-3.16927702307148));
#62023=CARTESIAN_POINT('Ctrl Pts',(0.751867687417125,0.689425970731327,
-3.14814380125514));
#62024=CARTESIAN_POINT('Ctrl Pts',(0.757988843515511,0.786067579426479,
-3.12697982683278));
#62025=CARTESIAN_POINT('Ctrl Pts',(0.764109999613896,0.881591964901016,
-3.10139267837718));
#62026=CARTESIAN_POINT('Ctrl Pts',(0.770231155712282,0.975572625816714,
-3.07154287195492));
#62027=CARTESIAN_POINT('Ctrl Pts',(0.770913646317185,0.986051188540249,
-3.06821470777909));
#62028=CARTESIAN_POINT('Ctrl Pts',(0.771596136922087,0.99651058265728,-3.06483360044361));
#62029=CARTESIAN_POINT('Ctrl Pts',(0.77227862752699,1.00695023444242,-3.06139980856084));
#62030=CARTESIAN_POINT('Ctrl Pts',(0.778461682484641,1.10152873891206,-3.03029121340689));
#62031=CARTESIAN_POINT('Ctrl Pts',(0.784644737442292,1.19482414783666,-2.99474310349924));
#62032=CARTESIAN_POINT('Ctrl Pts',(0.790827792399944,1.2863904560637,-2.95488022719166));
#62033=CARTESIAN_POINT('Ctrl Pts',(0.797002694600637,1.3778360282045,-2.91506991265887));
#62034=CARTESIAN_POINT('Ctrl Pts',(0.80317759680133,1.4675566384062,-2.87095631233905));
#62035=CARTESIAN_POINT('Ctrl Pts',(0.809352499002023,1.55512216672304,-2.82271369590801));
#62036=CARTESIAN_POINT('Ctrl Pts',(0.815521064788214,1.64259783912549,-2.77452058393946));
#62037=CARTESIAN_POINT('Ctrl Pts',(0.821689630574404,1.72792244976038,-2.72220708804443));
#62038=CARTESIAN_POINT('Ctrl Pts',(0.827858196360595,1.81068744465614,-2.66599485000715));
#62039=CARTESIAN_POINT('Ctrl Pts',(0.834022504977734,1.8933953201846,-2.6098214062388));
#62040=CARTESIAN_POINT('Ctrl Pts',(0.840186813594873,1.97354673523881,-2.54975481228269));
#62041=CARTESIAN_POINT('Ctrl Pts',(0.846351122212013,2.05076003749252,-2.48606130880227));
#62042=CARTESIAN_POINT('Ctrl Pts',(0.852513243557509,2.12794594227525,-2.42239040558453));
#62043=CARTESIAN_POINT('Ctrl Pts',(0.858675364903006,2.20219547258825,-2.35509542523953));
#62044=CARTESIAN_POINT('Ctrl Pts',(0.864837486248502,2.27315885622364,-2.28448383160662));
#62045=CARTESIAN_POINT('Ctrl Pts',(0.870999052686446,2.34411584950814,-2.21387859664541));
#62046=CARTESIAN_POINT('Ctrl Pts',(0.87716061912439,2.4117869778883,-2.13995764742067));
#62047=CARTESIAN_POINT('Ctrl Pts',(0.883322185562333,2.4758589676832,-2.06306566416164));
#62048=CARTESIAN_POINT('Ctrl Pts',(0.889484828557319,2.53994215222094,-1.98616024623353));
#62049=CARTESIAN_POINT('Ctrl Pts',(0.895647471552306,2.60042467190617,-1.90628309533125));
#62050=CARTESIAN_POINT('Ctrl Pts',(0.901810114547291,2.65703385441066,-1.82381157442748));
#62051=CARTESIAN_POINT('Ctrl Pts',(0.907979443228864,2.71370445070343,-1.7412505823761));
#62052=CARTESIAN_POINT('Ctrl Pts',(0.914148771910437,2.76649307349234,-1.6560899573173));
#62053=CARTESIAN_POINT('Ctrl Pts',(0.92031810059201,2.81517075098734,-1.56873554345064));
#62054=CARTESIAN_POINT('Ctrl Pts',(0.926490943813296,2.86387615915443,-1.48133136557036));
#62055=CARTESIAN_POINT('Ctrl Pts',(0.932663787034581,2.90846576506642,-1.39173129711002));
#62056=CARTESIAN_POINT('Ctrl Pts',(0.938836630255866,2.9487578174585,-1.30036337093806));
#62057=CARTESIAN_POINT('Ctrl Pts',(0.945019777252445,2.98911712577124,-1.20884293245587));
#62058=CARTESIAN_POINT('Ctrl Pts',(0.951202924249024,3.02516439562367,-1.11554914552634));
#62059=CARTESIAN_POINT('Ctrl Pts',(0.957386071245603,3.05676697446734,-1.02092763029796));
#62060=CARTESIAN_POINT('Ctrl Pts',(0.961965996252608,3.08017535230666,-0.950840432947641));
#62061=CARTESIAN_POINT('Ctrl Pts',(0.966545921259613,3.10114617417517,-0.880025126616937));
#62062=CARTESIAN_POINT('Ctrl Pts',(0.971125846266619,3.11964365813319,-0.808666191187291));
#62063=CARTESIAN_POINT('Ctrl Pts',(0.9772898628455,3.14453899978408,-0.712625828000808));
#62064=CARTESIAN_POINT('Ctrl Pts',(0.983453879424382,3.16504011821803,-0.615261367917324));
#62065=CARTESIAN_POINT('Ctrl Pts',(0.989617896003263,3.18100867365013,-0.517011973422887));
#62066=CARTESIAN_POINT('Ctrl Pts',(0.995773445998527,3.19695529547643,-0.418897529362669));
#62067=CARTESIAN_POINT('Ctrl Pts',(1.00192899599379,3.20838165831193,-0.319900992765871));
#62068=CARTESIAN_POINT('Ctrl Pts',(1.00808454598905,3.21519955765861,-0.220475320459806));
#62069=CARTESIAN_POINT('Ctrl Pts',(1.01423347326855,3.22201012167221,-0.121156619580885));
#62070=CARTESIAN_POINT('Ctrl Pts',(1.02038240054804,3.22422204917994,-0.0214101330237101));
#62071=CARTESIAN_POINT('Ctrl Pts',(1.02653132782754,3.22179858874209,0.0783033593116213));
#62072=CARTESIAN_POINT('Ctrl Pts',(1.0326756475632,3.21937694426329,0.177942133852175));
#62073=CARTESIAN_POINT('Ctrl Pts',(1.03881996729886,3.21232682783494,0.277547529115844));
#62074=CARTESIAN_POINT('Ctrl Pts',(1.04496428703453,3.20066353678552,0.376656988242065));
#62075=CARTESIAN_POINT('Ctrl Pts',(1.05110621065712,3.18900479409382,0.475727797447691));
#62076=CARTESIAN_POINT('Ctrl Pts',(1.05724813427972,3.1727365019672,0.574302622559335));
#62077=CARTESIAN_POINT('Ctrl Pts',(1.06339005790232,3.15192589226522,0.671923159422321));
#62078=CARTESIAN_POINT('Ctrl Pts',(1.06953124130622,3.13111779063779,0.769531931152668));
#62079=CARTESIAN_POINT('Ctrl Pts',(1.07567242471013,3.1057685505429,0.866186217138891));
#62080=CARTESIAN_POINT('Ctrl Pts',(1.08181360811403,3.07599649092961,0.96143806367792));
#62081=CARTESIAN_POINT('Ctrl Pts',(1.08795570614685,3.04621999725459,1.05670409642284));
#62082=CARTESIAN_POINT('Ctrl Pts',(1.09409780417966,3.01201950586568,1.15056685899043));
#62083=CARTESIAN_POINT('Ctrl Pts',(1.10023990221247,2.97356284238373,1.24259469856217));
#62084=CARTESIAN_POINT('Ctrl Pts',(1.10638856068393,2.93506510294043,1.33472083402439));
#62085=CARTESIAN_POINT('Ctrl Pts',(1.11253721915539,2.89230228172724,1.42500772996328));
#62086=CARTESIAN_POINT('Ctrl Pts',(1.11868587762685,2.84548985531016,1.51304495829667));
#62087=CARTESIAN_POINT('Ctrl Pts',(1.12483794886281,2.79865144602419,1.60113105100084));
#62088=CARTESIAN_POINT('Ctrl Pts',(1.13099002009876,2.74775917783632,1.68696461480813));
#62089=CARTESIAN_POINT('Ctrl Pts',(1.13714209133472,2.69307278616028,1.77016285435632));
#62090=CARTESIAN_POINT('Ctrl Pts',(1.14330451496477,2.63829437099227,1.85350109569095));
#62091=CARTESIAN_POINT('Ctrl Pts',(1.14946693859481,2.57970933561407,1.93419480215496));
#62092=CARTESIAN_POINT('Ctrl Pts',(1.15562936222486,2.51761882014655,2.01189289947151));
#62093=CARTESIAN_POINT('Ctrl Pts',(1.16041059648533,2.46944470593019,2.07217645463832));
#62094=CARTESIAN_POINT('Ctrl Pts',(1.1651918307458,2.41916124120921,2.13065737238373));
#62095=CARTESIAN_POINT('Ctrl Pts',(1.16997306500627,2.36692389664468,2.18718742452318));
#62096=CARTESIAN_POINT('Ctrl Pts',(1.17614724738719,2.29946790623175,2.26018674497009));
#62097=CARTESIAN_POINT('Ctrl Pts',(1.1823214297681,2.22851335131468,2.33019050162449));
#62098=CARTESIAN_POINT('Ctrl Pts',(1.18849561214902,2.1543568113567,2.39684465325998));
#62099=CARTESIAN_POINT('Ctrl Pts',(1.19466057704773,2.08031098024166,2.46339929642315));
#62100=CARTESIAN_POINT('Ctrl Pts',(1.20082554194645,2.00307299067149,2.5266139917632));
#62101=CARTESIAN_POINT('Ctrl Pts',(1.20699050684516,1.92297788170925,2.58616968293981));
#62102=CARTESIAN_POINT('Ctrl Pts',(1.210352910853,1.87929359156197,2.61865166750778));
#62103=CARTESIAN_POINT('Ctrl Pts',(1.21371531486084,1.83476007336656,2.65004583235345));
#62104=CARTESIAN_POINT('Ctrl Pts',(1.21707771886868,1.78943621037804,2.68030513402633));
#62105=CARTESIAN_POINT('',(0.585799999999996,1.87158653173902,-2.62360084935058));
#62106=CARTESIAN_POINT('Origin',(0.585799999999996,0.,0.));
#62107=CARTESIAN_POINT('Ctrl Pts',(0.585799999999996,1.87158653173884,-2.62360084935071));
#62108=CARTESIAN_POINT('Ctrl Pts',(0.592116907679877,1.95489173876411,-2.56417378233677));
#62109=CARTESIAN_POINT('Ctrl Pts',(0.598433815359758,2.03541956961639,-2.5007358573198));
#62110=CARTESIAN_POINT('Ctrl Pts',(0.604750723039639,2.11277861187854,-2.43357434644775));
#62111=CARTESIAN_POINT('Ctrl Pts',(0.611063991591541,2.19009308811734,-2.36645152686989));
#62112=CARTESIAN_POINT('Ctrl Pts',(0.617377260143442,2.26424210505644,-2.29560965736233));
#62113=CARTESIAN_POINT('Ctrl Pts',(0.623690528695344,2.3348670426893,-2.22137647765149));
#62114=CARTESIAN_POINT('Ctrl Pts',(0.630001626341581,2.40546769494986,-2.14716882405743));
#62115=CARTESIAN_POINT('Ctrl Pts',(0.636312723987817,2.4725464023986,-2.06957247583033));
#62116=CARTESIAN_POINT('Ctrl Pts',(0.642623821634054,2.53578159308669,-1.98895180300145));
#62117=CARTESIAN_POINT('Ctrl Pts',(0.648935997183835,2.59902758402538,-1.9083173605696));
#62118=CARTESIAN_POINT('Ctrl Pts',(0.655248172733616,2.65842849049503,-1.8246578754955));
#62119=CARTESIAN_POINT('Ctrl Pts',(0.661560348283396,2.71370335737527,-1.73837040088416));
#62120=CARTESIAN_POINT('Ctrl Pts',(0.667873475567062,2.76898655846033,-1.65206991606536));
#62121=CARTESIAN_POINT('Ctrl Pts',(0.674186602850728,2.8201422624078,-1.5631409939926));
#62122=CARTESIAN_POINT('Ctrl Pts',(0.680499730134394,2.86693369117845,-1.47200841467904));
#62123=CARTESIAN_POINT('Ctrl Pts',(0.686815142455302,2.91374205611284,-1.38084284991654));
#62124=CARTESIAN_POINT('Ctrl Pts',(0.693130554776209,2.95618281591122,-1.28747240051333));
#62125=CARTESIAN_POINT('Ctrl Pts',(0.699445967097116,2.9940661496825,-1.19234451976995));
#62126=CARTESIAN_POINT('Ctrl Pts',(0.705764999607745,3.03197119935269,-1.09716210878236));
#62127=CARTESIAN_POINT('Ctrl Pts',(0.712084032118375,3.06531347215733,-1.0002206370582));
#62128=CARTESIAN_POINT('Ctrl Pts',(0.718403064629004,3.09395229576761,-0.901984896777288));
#62129=CARTESIAN_POINT('Ctrl Pts',(0.724731470229132,3.12263359965576,-0.803603442356719));
#62130=CARTESIAN_POINT('Ctrl Pts',(0.731059875829262,3.14659740761162,-0.703924274890147));
#62131=CARTESIAN_POINT('Ctrl Pts',(0.737388281429391,3.16575359991218,-0.603424980542821));
#62132=CARTESIAN_POINT('Ctrl Pts',(0.74372187585346,3.1849254988718,-0.50284328421663));
#62133=CARTESIAN_POINT('Ctrl Pts',(0.75005547027753,3.1992818684031,-0.40144052147717));
#62134=CARTESIAN_POINT('Ctrl Pts',(0.756389064701599,3.20878440969236,-0.299700141166575));
#62135=CARTESIAN_POINT('Ctrl Pts',(0.762733850894677,3.21830374243367,-0.19777998066182));
#62136=CARTESIAN_POINT('Ctrl Pts',(0.769078637087755,3.22295209404247,-0.0955214153485939));
#62137=CARTESIAN_POINT('Ctrl Pts',(0.775423423280833,3.22274326031057,0.00659095007003059));
#62138=CARTESIAN_POINT('Ctrl Pts',(0.7784980217671,3.2226420622786,0.0560732359329862));
#62139=CARTESIAN_POINT('Ctrl Pts',(0.781572620253367,3.22140106071772,0.105521249986489));
#62140=CARTESIAN_POINT('Ctrl Pts',(0.784647218739633,3.21902619190892,0.154880400000556));
#62141=CARTESIAN_POINT('Ctrl Pts',(0.790757168417377,3.21430676952652,0.252968629754527));
#62142=CARTESIAN_POINT('Ctrl Pts',(0.796867118095121,3.20508966068731,0.351050336190424));
#62143=CARTESIAN_POINT('Ctrl Pts',(0.802977067772864,3.19136495852951,0.448672780509321));
#62144=CARTESIAN_POINT('Ctrl Pts',(0.80907773518726,3.17766110700166,0.546146916366667));
#62145=CARTESIAN_POINT('Ctrl Pts',(0.815178402601655,3.15946332634572,0.643162741113106));
#62146=CARTESIAN_POINT('Ctrl Pts',(0.82127907001605,3.13681369133633,0.739268170791191));
#62147=CARTESIAN_POINT('Ctrl Pts',(0.827489896212018,3.11375507546858,0.837108960933415));
#62148=CARTESIAN_POINT('Ctrl Pts',(0.833700722407985,3.08608224683887,0.934005690625308));
#62149=CARTESIAN_POINT('Ctrl Pts',(0.839911548603953,3.05389490892766,1.02948698278597));
#62150=CARTESIAN_POINT('Ctrl Pts',(0.845999056097287,3.02234666485472,1.12307245163689));
#62151=CARTESIAN_POINT('Ctrl Pts',(0.852086563590622,2.9864616711278,1.21529772588378));
#62152=CARTESIAN_POINT('Ctrl Pts',(0.858174071083956,2.9463849432905,1.30573095561493));
#62153=CARTESIAN_POINT('Ctrl Pts',(0.864258621066954,2.90632768603896,1.39612024992391));
#62154=CARTESIAN_POINT('Ctrl Pts',(0.870343171049953,2.86208291936874,1.48471882347684));
#62155=CARTESIAN_POINT('Ctrl Pts',(0.876427721032951,2.81384418973302,1.57111375730904));
#62156=CARTESIAN_POINT('Ctrl Pts',(0.882511025615258,2.76561533371941,1.65749100761318));
#62157=CARTESIAN_POINT('Ctrl Pts',(0.888594330197564,2.71339435643726,1.7416651269668));
#62158=CARTESIAN_POINT('Ctrl Pts',(0.89467763477987,2.65742072344934,1.82324783314885));
#62159=CARTESIAN_POINT('Ctrl Pts',(0.900982740108154,2.59940625995823,1.90780509121223));
#62160=CARTESIAN_POINT('Ctrl Pts',(0.907287845436437,2.53736051465106,1.98957791235419));
#62161=CARTESIAN_POINT('Ctrl Pts',(0.913592950764721,2.47159830858911,2.06816811779881));
#62162=CARTESIAN_POINT('Ctrl Pts',(0.919681880675533,2.40809081067382,2.14406379720673));
#62163=CARTESIAN_POINT('Ctrl Pts',(0.925770810586345,2.34111788180747,2.21699122991317));
#62164=CARTESIAN_POINT('Ctrl Pts',(0.931859740497157,2.27100209004627,2.2866278817301));
#62165=CARTESIAN_POINT('Ctrl Pts',(0.937951885881013,2.20084927118152,2.35630130762393));
#62166=CARTESIAN_POINT('Ctrl Pts',(0.944044031264868,2.1275506154588,2.42268019643455));
#62167=CARTESIAN_POINT('Ctrl Pts',(0.950136176648724,2.05146263451116,2.48548156736366));
#62168=CARTESIAN_POINT('Ctrl Pts',(0.956235946814951,1.97527942367991,2.54836153897543));
#62169=CARTESIAN_POINT('Ctrl Pts',(0.962335716981179,1.89630027968192,2.60765479757206));
#62170=CARTESIAN_POINT('Ctrl Pts',(0.968435487147407,1.81491111748615,2.663121326212));
#62171=CARTESIAN_POINT('Ctrl Pts',(0.969069957671363,1.80644538468387,2.66889070383266));
#62172=CARTESIAN_POINT('Ctrl Pts',(0.969704428195318,1.79795359929468,2.67461872021029));
#62173=CARTESIAN_POINT('Ctrl Pts',(0.970338898719273,1.78943621037804,2.68030513402633));
#62174=CARTESIAN_POINT('Origin',(-1.72497344927317,0.,0.));
#62175=CARTESIAN_POINT('',(2.46694827513675,1.78943621037803,2.68030513402633));
#62176=CARTESIAN_POINT('',(2.22053406624882,1.78943621037804,2.68030513402633));
#62177=CARTESIAN_POINT('',(-1.72497344927317,1.78943621037804,2.68030513402633));
#62178=CARTESIAN_POINT('',(1.64657344923657,-3.22274952152685,0.00175613167923087));
#62179=CARTESIAN_POINT('Ctrl Pts',(1.6465734492731,-3.22274952152717,0.00175613108471597));
#62180=CARTESIAN_POINT('Ctrl Pts',(1.65280034903924,-3.22280473869681,-0.0995752037854233));
#62181=CARTESIAN_POINT('Ctrl Pts',(1.65902724880537,-3.2180764441791,-0.200906486064027));
#62182=CARTESIAN_POINT('Ctrl Pts',(1.66525414857151,-3.20859114138214,-0.301762240752683));
#62183=CARTESIAN_POINT('Ctrl Pts',(1.67148276993094,-3.19910321611906,-0.402645879717201));
#62184=CARTESIAN_POINT('Ctrl Pts',(1.67771139129037,-3.18485570519006,-0.50305331217472));
#62185=CARTESIAN_POINT('Ctrl Pts',(1.6839400126498,-3.16592690778675,-0.602515043008761));
#62186=CARTESIAN_POINT('Ctrl Pts',(1.69017185848045,-3.14698831120654,-0.702028263806664));
#62187=CARTESIAN_POINT('Ctrl Pts',(1.6964037043111,-3.12336368506292,-0.800594397529432));
#62188=CARTESIAN_POINT('Ctrl Pts',(1.70263555014175,-3.0951820835199,-0.897755775452007));
#62189=CARTESIAN_POINT('Ctrl Pts',(1.70887643902191,-3.06695958757336,-0.995058144531123));
#62190=CARTESIAN_POINT('Ctrl Pts',(1.71511732790207,-3.03416703117107,-1.09095128516009));
#62191=CARTESIAN_POINT('Ctrl Pts',(1.72135821678223,-2.99698289431817,-1.18499413233327));
#62192=CARTESIAN_POINT('Ctrl Pts',(1.72760426415207,-2.95976802242259,-1.27911471187209));
#62193=CARTESIAN_POINT('Ctrl Pts',(1.73385031152191,-2.91815451181887,-1.3713815703785));
#62194=CARTESIAN_POINT('Ctrl Pts',(1.74009635889175,-2.87236752200162,-1.46137687851227));
#62195=CARTESIAN_POINT('Ctrl Pts',(1.74635354898619,-2.82649884983587,-1.55153273504968));
#62196=CARTESIAN_POINT('Ctrl Pts',(1.75261073908064,-2.77644203880034,-1.63940858621195));
#62197=CARTESIAN_POINT('Ctrl Pts',(1.75886792917508,-2.72246647293615,-1.72461412096696));
#62198=CARTESIAN_POINT('Ctrl Pts',(1.76141685985845,-2.70047897153262,-1.7593234711149));
#62199=CARTESIAN_POINT('Ctrl Pts',(1.76396579054183,-2.67784165713318,-1.79359007414299));
#62200=CARTESIAN_POINT('Ctrl Pts',(1.7665147212252,-2.65457462769775,-1.82738915080596));
#62201=CARTESIAN_POINT('Ctrl Pts',(1.77268729314374,-2.59823044640725,-1.90923807390272));
#62202=CARTESIAN_POINT('Ctrl Pts',(1.77885986506227,-2.53799813444767,-1.988622600153));
#62203=CARTESIAN_POINT('Ctrl Pts',(1.78503243698081,-2.47412053420035,-2.06515015065447));
#62204=CARTESIAN_POINT('Ctrl Pts',(1.79119665166003,-2.41032941984574,-2.14157408809759));
#62205=CARTESIAN_POINT('Ctrl Pts',(1.79736086633924,-2.34290310289145,-2.21514840768785));
#62206=CARTESIAN_POINT('Ctrl Pts',(1.80352508101845,-2.27212760626152,-2.28550950629489));
#62207=CARTESIAN_POINT('Ctrl Pts',(1.809682770457,-2.20142703031047,-2.35579612289155));
#62208=CARTESIAN_POINT('Ctrl Pts',(1.81584045989556,-2.12738462948071,-2.4228759763318));
#62209=CARTESIAN_POINT('Ctrl Pts',(1.82199814933411,-2.05032595519718,-2.48641932102065));
#62210=CARTESIAN_POINT('Ctrl Pts',(1.82815134253488,-1.97332354781798,-2.54991626746387));
#62211=CARTESIAN_POINT('Ctrl Pts',(1.83430453573565,-1.89330957988632,-2.60988156373336));
#62212=CARTESIAN_POINT('Ctrl Pts',(1.84045772893642,-1.81064495922136,-2.66602370472325));
#62213=CARTESIAN_POINT('Ctrl Pts',(1.84660859180534,-1.7280116452279,-2.72214458361151));
#62214=CARTESIAN_POINT('Ctrl Pts',(1.85275945467427,-1.64273003205378,-2.77444494045738));
#62215=CARTESIAN_POINT('Ctrl Pts',(1.85891031754319,-1.55519175338522,-2.82267535729892));
#62216=CARTESIAN_POINT('Ctrl Pts',(1.86506049577754,-1.46766321834669,-2.87090040575369));
#62217=CARTESIAN_POINT('Ctrl Pts',(1.87121067401189,-1.37787889760995,-2.91505620527407));
#62218=CARTESIAN_POINT('Ctrl Pts',(1.87736085224624,-1.28625599776136,-2.95493875921701));
#62219=CARTESIAN_POINT('Ctrl Pts',(1.88351199054027,-1.19461879532692,-2.99482753893595));
#62220=CARTESIAN_POINT('Ctrl Pts',(1.8896631288343,-1.10114284197652,-3.0304415747476));
#62221=CARTESIAN_POINT('Ctrl Pts',(1.89581426712834,-1.00626539882668,-3.061624978606));
#62222=CARTESIAN_POINT('Ctrl Pts',(1.90197198119414,-0.911286528529178,
-3.09284171856203));
#62223=CARTESIAN_POINT('Ctrl Pts',(1.90812969525993,-0.814903590014241,
-3.11961823239626));
#62224=CARTESIAN_POINT('Ctrl Pts',(1.91428740932573,-0.717568975034798,
-3.14184855277391));
#62225=CARTESIAN_POINT('Ctrl Pts',(1.9204485590456,-0.620180052878697,-3.16409127640538));
#62226=CARTESIAN_POINT('Ctrl Pts',(1.92660970876546,-0.521838824287656,
-3.18178267821856));
#62227=CARTESIAN_POINT('Ctrl Pts',(1.93277085848533,-0.423005768012119,
-3.19486833574225));
#62228=CARTESIAN_POINT('Ctrl Pts',(1.93894230378675,-0.324007556881048,
-3.20797586003765));
#62229=CARTESIAN_POINT('Ctrl Pts',(1.94511374908818,-0.224516309361872,
-3.21646222973386));
#62230=CARTESIAN_POINT('Ctrl Pts',(1.9512851943896,-0.124995636520338,-3.22032508504202));
#62231=CARTESIAN_POINT('Ctrl Pts',(1.95597744291468,-0.0493284779298773,
-3.22326207568797));
#62232=CARTESIAN_POINT('Ctrl Pts',(1.96066969143976,0.0263556273248075,
-3.22352738288182));
#62233=CARTESIAN_POINT('Ctrl Pts',(1.96536193996483,0.101854934327927,-3.22114003651705));
#62234=CARTESIAN_POINT('Ctrl Pts',(1.97153433126488,0.201170062931038,-3.21799961549003));
#62235=CARTESIAN_POINT('Ctrl Pts',(1.97770672256493,0.300514518760375,-3.2102561973682));
#62236=CARTESIAN_POINT('Ctrl Pts',(1.98387911386498,0.399426776188079,-3.19790178288265));
#62237=CARTESIAN_POINT('Ctrl Pts',(1.99004314898721,0.498205126290214,-3.18556409379236));
#62238=CARTESIAN_POINT('Ctrl Pts',(1.99620718410944,0.596552013751196,-3.1686278691003));
#62239=CARTESIAN_POINT('Ctrl Pts',(2.00237121923168,0.694006938371615,-3.14713710092078));
#62240=CARTESIAN_POINT('Ctrl Pts',(2.00852873041156,0.791358717844935,-3.12566907831778));
#62241=CARTESIAN_POINT('Ctrl Pts',(2.01468624159145,0.887819989502827,-3.09965618882277));
#62242=CARTESIAN_POINT('Ctrl Pts',(2.02084375277134,0.982937360234891,-3.0691939835003));
#62243=CARTESIAN_POINT('Ctrl Pts',(2.02699677043197,1.07798531789979,-3.03875400834556));
#62244=CARTESIAN_POINT('Ctrl Pts',(2.0331497880926,1.17169091208353,-3.00387130491829));
#62245=CARTESIAN_POINT('Ctrl Pts',(2.03930280575323,1.26361379977512,-2.96469184360161));
#62246=CARTESIAN_POINT('Ctrl Pts',(2.04545349480919,1.35550189932253,-2.92552720972109));
#62247=CARTESIAN_POINT('Ctrl Pts',(2.05160418386515,1.44560823380423,-2.88206921913371));
#62248=CARTESIAN_POINT('Ctrl Pts',(2.05775487292111,1.53351125056552,-2.83451244606352));
#62249=CARTESIAN_POINT('Ctrl Pts',(2.06390487928364,1.62140451056433,-2.78696095153957));
#62250=CARTESIAN_POINT('Ctrl Pts',(2.07005488564617,1.7070945570307,-2.7353117857095));
#62251=CARTESIAN_POINT('Ctrl Pts',(2.0762048920087,1.79018421900486,-2.67980559453964));
#62252=CARTESIAN_POINT('Ctrl Pts',(2.08235586058764,1.87328688100408,-2.62429071899366));
#62253=CARTESIAN_POINT('Ctrl Pts',(2.08850682916659,1.95378798918882,-2.56491786077052));
#62254=CARTESIAN_POINT('Ctrl Pts',(2.09465779774553,2.03131999898255,-2.50197054823464));
#62255=CARTESIAN_POINT('Ctrl Pts',(2.10081534652916,2.10893495124091,-2.43895589570257));
#62256=CARTESIAN_POINT('Ctrl Pts',(2.10697289531279,2.18357412451723,-2.3723594272501));
#62257=CARTESIAN_POINT('Ctrl Pts',(2.11313044409641,2.25490378730162,-2.30250439142096));
#62258=CARTESIAN_POINT('Ctrl Pts',(2.11929143073562,2.32627327454985,-2.23261035443522));
#62259=CARTESIAN_POINT('Ctrl Pts',(2.12545241737482,2.39432927567538,-2.15945444496975));
#62260=CARTESIAN_POINT('Ctrl Pts',(2.13161340401402,2.45877704760324,-2.08339458400935));
#62261=CARTESIAN_POINT('Ctrl Pts',(2.13778469158107,2.52333257367623,-2.00720755394673));
#62262=CARTESIAN_POINT('Ctrl Pts',(2.14395597914812,2.58426755499085,-1.92810721834254));
#62263=CARTESIAN_POINT('Ctrl Pts',(2.15012726671517,2.64132935127803,-1.84648228276828));
#62264=CARTESIAN_POINT('Ctrl Pts',(2.15482123071161,2.68473131795583,-1.78439726329146));
#62265=CARTESIAN_POINT('Ctrl Pts',(2.15951519470805,2.72589339377815,-1.72085231729032));
#62266=CARTESIAN_POINT('Ctrl Pts',(2.16420915870449,2.76472240631613,-1.65602765028654));
#62267=CARTESIAN_POINT('Ctrl Pts',(2.1703812373919,2.81577855436516,-1.57078989687891));
#62268=CARTESIAN_POINT('Ctrl Pts',(2.17655331607932,2.86297903973375,-1.48303869173317));
#62269=CARTESIAN_POINT('Ctrl Pts',(2.18272539476673,2.90606756231055,-1.393157882577));
#62270=CARTESIAN_POINT('Ctrl Pts',(2.1888891115705,2.94909770889593,-1.30339884323399));
#62271=CARTESIAN_POINT('Ctrl Pts',(2.19505282837426,2.98802677922563,-1.21151632272987));
#62272=CARTESIAN_POINT('Ctrl Pts',(2.20121654517802,3.02264275951866,-1.11792142426442));
#62273=CARTESIAN_POINT('Ctrl Pts',(2.20737373278518,3.05722207126441,-1.02442567044058));
#62274=CARTESIAN_POINT('Ctrl Pts',(2.21353092039234,3.08749722638055,-0.929221550063133));
#62275=CARTESIAN_POINT('Ctrl Pts',(2.21968810799949,3.11330342310276,-0.832742071830553));
#62276=CARTESIAN_POINT('Ctrl Pts',(2.22584079549085,3.13909075879927,-0.73633310774381));
#62277=CARTESIAN_POINT('Ctrl Pts',(2.2319934829822,3.16041551802508,-0.638651057405087));
#62278=CARTESIAN_POINT('Ctrl Pts',(2.23814617047355,3.17716236682762,-0.540145218727602));
#62279=CARTESIAN_POINT('Ctrl Pts',(2.24429652541123,3.19390286670967,-0.44167672473183));
#62280=CARTESIAN_POINT('Ctrl Pts',(2.2504468803489,3.20606883194019,-0.342385490731476));
#62281=CARTESIAN_POINT('Ctrl Pts',(2.25659723528658,3.21359597362361,-0.242731293429856));
#62282=CARTESIAN_POINT('Ctrl Pts',(2.26274690396581,3.2211222754263,-0.143088215573441));
#62283=CARTESIAN_POINT('Ctrl Pts',(2.26889657264504,3.22401075002825,-0.0430826881038844));
#62284=CARTESIAN_POINT('Ctrl Pts',(2.27504624132427,3.22224904753393,0.0568211067005552));
#62285=CARTESIAN_POINT('Ctrl Pts',(2.28119686903602,3.22048707030448,0.156740481366882));
#62286=CARTESIAN_POINT('Ctrl Pts',(2.28734749674778,3.21407348323025,0.256557657479677));
#62287=CARTESIAN_POINT('Ctrl Pts',(2.29349812445953,3.20304802887491,0.355810184256337));
#62288=CARTESIAN_POINT('Ctrl Pts',(2.29965532950994,3.19201078415435,0.455168849383647));
#62289=CARTESIAN_POINT('Ctrl Pts',(2.30581253456035,3.17635187186371,0.553961226813639));
#62290=CARTESIAN_POINT('Ctrl Pts',(2.31196973961076,3.15616273100808,0.651731829739503));
#62291=CARTESIAN_POINT('Ctrl Pts',(2.31813038038822,3.13596232459011,0.749556988767112));
#62292=CARTESIAN_POINT('Ctrl Pts',(2.32429102116568,3.11122676294175,0.846358816950549));
#62293=CARTESIAN_POINT('Ctrl Pts',(2.33045166194313,3.08209773392253,0.941695875030569));
#62294=CARTESIAN_POINT('Ctrl Pts',(2.33662260373307,3.05291999917572,1.03719234318832));
#62295=CARTESIAN_POINT('Ctrl Pts',(2.34279354552301,3.01933426948965,1.13121873977146));
#62296=CARTESIAN_POINT('Ctrl Pts',(2.34896448731295,2.98153089518619,1.22335239548964));
#62297=CARTESIAN_POINT('Ctrl Pts',(2.35366178402335,2.95275511479446,1.29348417320747));
#62298=CARTESIAN_POINT('Ctrl Pts',(2.35835908073374,2.92153655702733,1.36251964955495));
#62299=CARTESIAN_POINT('Ctrl Pts',(2.36305637744414,2.88797665975281,1.43028262075123));
#62300=CARTESIAN_POINT('Ctrl Pts',(2.36922850018484,2.84387984877527,1.51932135968647));
#62301=CARTESIAN_POINT('Ctrl Pts',(2.37540062292555,2.79558387048185,1.60647556528312));
#62302=CARTESIAN_POINT('Ctrl Pts',(2.38157274566625,2.74327306222189,1.6913221066928));
#62303=CARTESIAN_POINT('Ctrl Pts',(2.38773684236677,2.6910302773417,1.77605831624753));
#62304=CARTESIAN_POINT('Ctrl Pts',(2.39390093906729,2.63478326276098,1.85849245816756));
#62305=CARTESIAN_POINT('Ctrl Pts',(2.40006503576781,2.57476326090943,1.93822385517541));
#62306=CARTESIAN_POINT('Ctrl Pts',(2.40622186982413,2.51481397565102,2.0178613112871));
#62307=CARTESIAN_POINT('Ctrl Pts',(2.41237870388045,2.45110080597488,2.09480201206285));
#62308=CARTESIAN_POINT('Ctrl Pts',(2.41853553793677,2.38389885062525,2.168673288554));
#62309=CARTESIAN_POINT('Ctrl Pts',(2.42468813289258,2.31674316513447,2.24249370322843));
#62310=CARTESIAN_POINT('Ctrl Pts',(2.4308407278484,2.24610375926931,2.31324857355045));
#62311=CARTESIAN_POINT('Ctrl Pts',(2.43699332280421,2.17229620568289,2.38059798312855));
#62312=CARTESIAN_POINT('Ctrl Pts',(2.44314380416744,2.09851400710507,2.44792425625549));
#62313=CARTESIAN_POINT('Ctrl Pts',(2.44929428553067,2.02156614221978,2.51184709906017));
#62314=CARTESIAN_POINT('Ctrl Pts',(2.4554447668939,1.94180462797299,2.57206383071701));
#62315=CARTESIAN_POINT('Ctrl Pts',(2.45927926964151,1.89207750460312,2.60960580659732));
#62316=CARTESIAN_POINT('Ctrl Pts',(2.46311377238913,1.84125746650579,2.64570801633063));
#62317=CARTESIAN_POINT('Ctrl Pts',(2.46694827513675,1.78943621037803,2.68030513402633));
#62318=CARTESIAN_POINT('Ctrl Pts',(1.21707771886868,1.78943621037804,2.68030513402633));
#62319=CARTESIAN_POINT('Ctrl Pts',(1.22340032573857,1.70420999519611,2.73720420629387));
#62320=CARTESIAN_POINT('Ctrl Pts',(1.22972293260845,1.61618729446822,2.79008771147135));
#62321=CARTESIAN_POINT('Ctrl Pts',(1.23604553947834,1.52578684091609,2.83867787510089));
#62322=CARTESIAN_POINT('Ctrl Pts',(1.24219858989544,1.43781070071279,2.88596497245497));
#62323=CARTESIAN_POINT('Ctrl Pts',(1.24835164031254,1.34758313548586,2.92918587595363));
#62324=CARTESIAN_POINT('Ctrl Pts',(1.25450469072965,1.25551775368136,2.96812950066046));
#62325=CARTESIAN_POINT('Ctrl Pts',(1.26065635079051,1.16347317516455,3.00706432558379));
#62326=CARTESIAN_POINT('Ctrl Pts',(1.26680801085137,1.06959200506838,3.04172362352167));
#62327=CARTESIAN_POINT('Ctrl Pts',(1.27295967091224,0.974309102690366,3.07194390165489));
#62328=CARTESIAN_POINT('Ctrl Pts',(1.27911158389948,0.879022282742172,3.10216542229918));
#62329=CARTESIAN_POINT('Ctrl Pts',(1.28526349688673,0.7823340300486,3.12794742984124));
#62330=CARTESIAN_POINT('Ctrl Pts',(1.29141540987398,0.684694716996577,3.14917619497814));
#62331=CARTESIAN_POINT('Ctrl Pts',(1.29786581602997,0.582317907167919,3.17143498791085));
#62332=CARTESIAN_POINT('Ctrl Pts',(1.30431622218597,0.478895929833729,3.18868741957029));
#62333=CARTESIAN_POINT('Ctrl Pts',(1.31076662834196,0.374958615110494,3.20086294605914));
#62334=CARTESIAN_POINT('Ctrl Pts',(1.31692766278283,0.275684032981056,3.21249226617007));
#62335=CARTESIAN_POINT('Ctrl Pts',(1.32308869722371,0.175939800375313,3.21949038117817));
#62336=CARTESIAN_POINT('Ctrl Pts',(1.32924973166458,0.076190108328905,3.22184925623357));
#62337=CARTESIAN_POINT('Ctrl Pts',(1.33541511191715,-0.023629944203698,
3.22420979516976));
#62338=CARTESIAN_POINT('Ctrl Pts',(1.34158049216972,-0.123455030898768,
3.22192459052998));
#62339=CARTESIAN_POINT('Ctrl Pts',(1.34774587242229,-0.222824135759187,
3.21503763073205));
#62340=CARTESIAN_POINT('Ctrl Pts',(1.35392043030039,-0.322341158898122,
3.20814041918395));
#62341=CARTESIAN_POINT('Ctrl Pts',(1.36009498817849,-0.421400416785637,
3.19662783719734));
#62342=CARTESIAN_POINT('Ctrl Pts',(1.36626954605659,-0.519549453305405,
3.1805952160044));
#62343=CARTESIAN_POINT('Ctrl Pts',(1.36711979195303,-0.533064723092881,
3.17838749997879));
#62344=CARTESIAN_POINT('Ctrl Pts',(1.36797003784947,-0.546562755769955,
3.17609415400508));
#62345=CARTESIAN_POINT('Ctrl Pts',(1.36882028374592,-0.56004239262392,3.17371550094902));
#62346=CARTESIAN_POINT('Ctrl Pts',(1.37499381742182,-0.657916422248695,
3.15644438584421));
#62347=CARTESIAN_POINT('Ctrl Pts',(1.38116735109773,-0.75516218775552,3.13461128406342));
#62348=CARTESIAN_POINT('Ctrl Pts',(1.38734088477363,-0.851321599816241,
3.10827429551935));
#62349=CARTESIAN_POINT('Ctrl Pts',(1.39350608513824,-0.947351211610776,
3.08197285781789));
#62350=CARTESIAN_POINT('Ctrl Pts',(1.39967128550285,-1.04229696956204,3.05117973097203));
#62351=CARTESIAN_POINT('Ctrl Pts',(1.40583648586747,-1.13570923744721,3.01600432534124));
#62352=CARTESIAN_POINT('Ctrl Pts',(1.4119951834889,-1.2290229787717,2.98086602095867));
#62353=CARTESIAN_POINT('Ctrl Pts',(1.41815388111033,-1.32080604162271,2.9413547794624));
#62354=CARTESIAN_POINT('Ctrl Pts',(1.42431257873176,-1.4106231976854,2.89763002411485));
#62355=CARTESIAN_POINT('Ctrl Pts',(1.43046680993421,-1.50037521642912,2.85393697889329));
#62356=CARTESIAN_POINT('Ctrl Pts',(1.43662104113665,-1.58816377375753,2.80603668460894));
#62357=CARTESIAN_POINT('Ctrl Pts',(1.4427752723391,-1.67357376430967,2.75413660117184));
#62358=CARTESIAN_POINT('Ctrl Pts',(1.44892719120158,-1.75895166361803,2.70225601824304));
#62359=CARTESIAN_POINT('Ctrl Pts',(1.45507911006407,-1.84195240132714,2.64637885756395));
#62360=CARTESIAN_POINT('Ctrl Pts',(1.46123102892656,-1.92218641645228,2.58675799851983));
#62361=CARTESIAN_POINT('Ctrl Pts',(1.46738227994742,-2.00241172151206,2.52714361181266));
#62362=CARTESIAN_POINT('Ctrl Pts',(1.47353353096828,-2.07987055265335,2.46378659371234));
#62363=CARTESIAN_POINT('Ctrl Pts',(1.47968478198914,-2.15420406316013,2.39698193918194));
#62364=CARTESIAN_POINT('Ctrl Pts',(1.48583700867722,-2.22854936391411,2.33016668857736));
#62365=CARTESIAN_POINT('Ctrl Pts',(1.49198923536531,-2.2997680364378,2.2599030055844));
#62366=CARTESIAN_POINT('Ctrl Pts',(1.4981414620534,-2.36753668152556,2.18652409639842));
#62367=CARTESIAN_POINT('Ctrl Pts',(1.50430028217181,-2.43537795525044,2.11306654597416));
#62368=CARTESIAN_POINT('Ctrl Pts',(1.51045910229022,-2.49976152299853,2.03648742203356));
#62369=CARTESIAN_POINT('Ctrl Pts',(1.51661792240863,-2.56040312316878,1.95715441633192));
#62370=CARTESIAN_POINT('Ctrl Pts',(1.52278018970818,-2.62107866532407,1.87777700679389));
#62371=CARTESIAN_POINT('Ctrl Pts',(1.52894245700773,-2.6780078215014,1.7956430026586));
#62372=CARTESIAN_POINT('Ctrl Pts',(1.53510472430728,-2.73094986828718,1.71114884782191));
#62373=CARTESIAN_POINT('Ctrl Pts',(1.54127729460607,-2.78398043149739,1.62651342303203));
#62374=CARTESIAN_POINT('Ctrl Pts',(1.54744986490486,-2.83301035644263,1.53951034383121));
#62375=CARTESIAN_POINT('Ctrl Pts',(1.55362243520364,-2.87784498461981,1.45056051476614));
#62376=CARTESIAN_POINT('Ctrl Pts',(1.55830412429761,-2.91185055759974,1.38309503045632));
#62377=CARTESIAN_POINT('Ctrl Pts',(1.56298581339158,-2.94344365280984,1.31451014118222));
#62378=CARTESIAN_POINT('Ctrl Pts',(1.56766750248555,-2.97255827287987,1.24499593446463));
#62379=CARTESIAN_POINT('Ctrl Pts',(1.57453989941227,-3.01529652855551,1.14295386994037));
#62380=CARTESIAN_POINT('Ctrl Pts',(1.58141229633898,-3.05282061275208,1.03860409475009));
#62381=CARTESIAN_POINT('Ctrl Pts',(1.5882846932657,-3.08490276173312,0.932465824119787));
#62382=CARTESIAN_POINT('Ctrl Pts',(1.59513648219888,-3.11688870720235,0.826645826257836));
#62383=CARTESIAN_POINT('Ctrl Pts',(1.60198827113206,-3.14346516490069,0.719048267582058));
#62384=CARTESIAN_POINT('Ctrl Pts',(1.60884006006525,-3.16445263402091,0.610210692743205));
#62385=CARTESIAN_POINT('Ctrl Pts',(1.61565487371116,-3.18532684546384,0.50196045365489));
#62386=CARTESIAN_POINT('Ctrl Pts',(1.62246968735706,-3.20067211544954,0.392483786661898));
#62387=CARTESIAN_POINT('Ctrl Pts',(1.62928450100298,-3.21035947712258,0.28232886878472));
#62388=CARTESIAN_POINT('Ctrl Pts',(1.63504748374751,-3.21855164510581,0.189175787286705));
#62389=CARTESIAN_POINT('Ctrl Pts',(1.64081046649204,-3.22269841813423,0.0955380707283682));
#62390=CARTESIAN_POINT('Ctrl Pts',(1.64657344923657,-3.22274952152685,0.00175613167923302));
#62391=CARTESIAN_POINT('',(1.40002655078068,-3.22274939283074,0.00197825911163994));
#62392=CARTESIAN_POINT('Ctrl Pts',(0.970338898719273,1.78943621037804,2.68030513402633));
#62393=CARTESIAN_POINT('Ctrl Pts',(0.974724078305945,1.73056778607964,2.71960711078642));
#62394=CARTESIAN_POINT('Ctrl Pts',(0.979109257892617,1.67047586253169,2.75692070227038));
#62395=CARTESIAN_POINT('Ctrl Pts',(0.983494437479289,1.6093118116581,2.79217353603921));
#62396=CARTESIAN_POINT('Ctrl Pts',(0.989675583431169,1.52309779966941,2.8418642970299));
#62397=CARTESIAN_POINT('Ctrl Pts',(0.995856729383049,1.43443090023847,2.88764431992224));
#62398=CARTESIAN_POINT('Ctrl Pts',(1.00203787533493,1.34370061336218,2.92926376827866));
#62399=CARTESIAN_POINT('Ctrl Pts',(1.00821066572557,1.25309297404582,2.97082695621794));
#62400=CARTESIAN_POINT('Ctrl Pts',(1.0143834561162,1.16042788175746,3.00824057022586));
#62401=CARTESIAN_POINT('Ctrl Pts',(1.02055624650684,1.06612126559161,3.04129955932548));
#62402=CARTESIAN_POINT('Ctrl Pts',(1.02672250133371,0.971914498418576,3.07432354656733));
#62403=CARTESIAN_POINT('Ctrl Pts',(1.03288875616058,0.876070069259749,3.10300193334037));
#62404=CARTESIAN_POINT('Ctrl Pts',(1.03905501098746,0.7790249504798,3.12717727176282));
#62405=CARTESIAN_POINT('Ctrl Pts',(1.04521671673993,0.682051425475667,3.15133477514337));
#62406=CARTESIAN_POINT('Ctrl Pts',(1.05137842249239,0.583879390990891,3.1709957314356));
#62407=CARTESIAN_POINT('Ctrl Pts',(1.05754012824486,0.484961218254331,3.18605244452901));
#62408=CARTESIAN_POINT('Ctrl Pts',(1.06369946807815,0.386081027273421,3.20110337627424));
#62409=CARTESIAN_POINT('Ctrl Pts',(1.06985880791144,0.286455694870284,3.21155351289783));
#62410=CARTESIAN_POINT('Ctrl Pts',(1.07601814774473,0.186547178965657,3.21734637745456));
#62411=CARTESIAN_POINT('Ctrl Pts',(1.08217675666867,0.0866505188881857,
3.22313855459039));
#62412=CARTESIAN_POINT('Ctrl Pts',(1.0883353655926,-0.013528825689528,3.22427453348602));
#62413=CARTESIAN_POINT('Ctrl Pts',(1.09449397451654,-0.113525377969389,
3.22074984298019));
#62414=CARTESIAN_POINT('Ctrl Pts',(1.10065348649824,-0.213536593083651,
3.21722463563701));
#62415=CARTESIAN_POINT('Ctrl Pts',(1.10681299847994,-0.313364529969851,
3.20903741670471));
#62416=CARTESIAN_POINT('Ctrl Pts',(1.11297251046164,-0.412546311658843,
3.19623577090876));
#62417=CARTESIAN_POINT('Ctrl Pts',(1.11913845611142,-0.511831689649731,
3.18342075367361));
#62418=CARTESIAN_POINT('Ctrl Pts',(1.1253044017612,-0.610469134487032,3.16598174018904));
#62419=CARTESIAN_POINT('Ctrl Pts',(1.13147034741098,-0.708003590241276,
3.14401788778395));
#62420=CARTESIAN_POINT('Ctrl Pts',(1.13763966237117,-0.805591342582289,
3.12204203348316));
#62421=CARTESIAN_POINT('Ctrl Pts',(1.14380897733136,-0.902074487851182,
3.09553653020164));
#62422=CARTESIAN_POINT('Ctrl Pts',(1.14997829229155,-0.997012811986731,
3.06465055352716));
#62423=CARTESIAN_POINT('Ctrl Pts',(1.15615770773974,-1.09210657046299,3.03371400990339));
#62424=CARTESIAN_POINT('Ctrl Pts',(1.16233712318792,-1.18565005041696,2.99838282009929));
#62425=CARTESIAN_POINT('Ctrl Pts',(1.16851653863611,-1.2772225817404,2.95885451470538));
#62426=CARTESIAN_POINT('Ctrl Pts',(1.17312491116372,-1.34551388553319,2.92937581106951));
#62427=CARTESIAN_POINT('Ctrl Pts',(1.17773328369132,-1.41270944558138,2.89756384378956));
#62428=CARTESIAN_POINT('Ctrl Pts',(1.18234165621892,-1.47864453547035,2.86351670157931));
#62429=CARTESIAN_POINT('Ctrl Pts',(1.18852471287063,-1.5671096918085,2.81783562700175));
#62430=CARTESIAN_POINT('Ctrl Pts',(1.19470776952234,-1.65360548738925,2.76797396991164));
#62431=CARTESIAN_POINT('Ctrl Pts',(1.20089082617404,-1.7377112728214,2.71412547514101));
#62432=CARTESIAN_POINT('Ctrl Pts',(1.20706573011307,-1.82170615998072,2.66034798268056));
#62433=CARTESIAN_POINT('Ctrl Pts',(1.21324063405209,-1.90331694006354,2.60259433364497));
#62434=CARTESIAN_POINT('Ctrl Pts',(1.21941553799112,-1.98214648415018,2.54110465700866));
#62435=CARTESIAN_POINT('Ctrl Pts',(1.22558410555742,-2.06089513736343,2.47967807795466));
#62436=CARTESIAN_POINT('Ctrl Pts',(1.23175267312373,-2.13686788981976,2.41452335863386));
#62437=CARTESIAN_POINT('Ctrl Pts',(1.23792124069003,-2.20969640222499,2.34592399120132));
#62438=CARTESIAN_POINT('Ctrl Pts',(1.24408555114311,-2.28247465349265,2.27737196624675));
#62439=CARTESIAN_POINT('Ctrl Pts',(1.2502498615962,-2.35211266494071,2.20538031540524));
#62440=CARTESIAN_POINT('Ctrl Pts',(1.25641417204928,-2.41827571657017,2.13027231150082));
#62441=CARTESIAN_POINT('Ctrl Pts',(1.26257629526443,-2.48441529203994,2.05519095762916));
#62442=CARTESIAN_POINT('Ctrl Pts',(1.26873841847957,-2.54708207223402,1.97699577233909));
#62443=CARTESIAN_POINT('Ctrl Pts',(1.27490054169472,-2.60597933810157,1.89604568823848));
#62444=CARTESIAN_POINT('Ctrl Pts',(1.28106211003392,-2.66487130049253,1.81510289338753));
#62445=CARTESIAN_POINT('Ctrl Pts',(1.28722367837312,-2.71999416898764,1.73140604281522));
#62446=CARTESIAN_POINT('Ctrl Pts',(1.29338524671231,-2.77109315175436,1.64534504186815));
#62447=CARTESIAN_POINT('Ctrl Pts',(1.29954789163807,-2.82220106284499,1.55926900382149));
#62448=CARTESIAN_POINT('Ctrl Pts',(1.30571053656383,-2.86928347053962,1.47082836672944));
#62449=CARTESIAN_POINT('Ctrl Pts',(1.31187318148959,-2.91213084404561,1.38043888298549));
#62450=CARTESIAN_POINT('Ctrl Pts',(1.31804251213623,-2.95502470174525,1.28995133763535));
#62451=CARTESIAN_POINT('Ctrl Pts',(1.32421184278288,-2.99367416495057,1.19751111535027));
#62452=CARTESIAN_POINT('Ctrl Pts',(1.33038117342953,-3.0279173592827,1.10355517662438));
#62453=CARTESIAN_POINT('Ctrl Pts',(1.33655401863793,-3.06218006137476,1.00954571281323));
#62454=CARTESIAN_POINT('Ctrl Pts',(1.34272686384633,-3.09203136623493,0.914019225727417));
#62455=CARTESIAN_POINT('Ctrl Pts',(1.34889970905473,-3.11735953592752,0.817427113730492));
#62456=CARTESIAN_POINT('Ctrl Pts',(1.35508285805436,-3.14272998372102,0.720673768959608));
#62457=CARTESIAN_POINT('Ctrl Pts',(1.36126600705399,-3.16356212508625,0.622851669525752));
#62458=CARTESIAN_POINT('Ctrl Pts',(1.36744915605362,-3.17979548502384,0.524421811066224));
#62459=CARTESIAN_POINT('Ctrl Pts',(1.37202906235527,-3.19181966032345,0.451514053375713));
#62460=CARTESIAN_POINT('Ctrl Pts',(1.37660896865692,-3.20132180253824,0.378273034406715));
#62461=CARTESIAN_POINT('Ctrl Pts',(1.38118887495857,-3.20829576914891,0.304886569335508));
#62462=CARTESIAN_POINT('Ctrl Pts',(1.38746810021468,-3.21785734189577,0.204270942163111));
#62463=CARTESIAN_POINT('Ctrl Pts',(1.39374732547078,-3.22268726269155,0.103193402978869));
#62464=CARTESIAN_POINT('Ctrl Pts',(1.40002655072689,-3.22274939283021,0.00197825997873392));
#62465=CARTESIAN_POINT('Ctrl Pts',(1.40002655078068,-3.22274939283074,0.00197825911163994));
#62466=CARTESIAN_POINT('Ctrl Pts',(1.40611289410352,-3.22280961446214,-0.096127810451189));
#62467=CARTESIAN_POINT('Ctrl Pts',(1.41219923742636,-3.21838586447631,-0.194419403685365));
#62468=CARTESIAN_POINT('Ctrl Pts',(1.41828558074921,-3.20945371439036,-0.292445580725625));
#62469=CARTESIAN_POINT('Ctrl Pts',(1.4243642957019,-3.20053275949065,-0.390348895823498));
#62470=CARTESIAN_POINT('Ctrl Pts',(1.43044301065459,-3.18711466954245,-0.48798701409589));
#62471=CARTESIAN_POINT('Ctrl Pts',(1.43652172560728,-3.16922703223334,-0.584908181393845));
#62472=CARTESIAN_POINT('Ctrl Pts',(1.44259457085173,-3.15135666752429,-0.681735760000863));
#62473=CARTESIAN_POINT('Ctrl Pts',(1.44866741609618,-3.12902541369874,-0.777847326044531));
#62474=CARTESIAN_POINT('Ctrl Pts',(1.45474026134062,-3.10231262737273,-0.872796611212326));
#62475=CARTESIAN_POINT('Ctrl Pts',(1.46080994861889,-3.07561373207676,-0.967696521397057));
#62476=CARTESIAN_POINT('Ctrl Pts',(1.46687963589716,-3.04453794865945,-1.06143492126537));
#62477=CARTESIAN_POINT('Ctrl Pts',(1.47294932317543,-3.00921544023296,-1.15357704413861));
#62478=CARTESIAN_POINT('Ctrl Pts',(1.47901757973629,-2.97390125785778,-1.24569744771508));
#62479=CARTESIAN_POINT('Ctrl Pts',(1.48508583629715,-2.93434249874623,-1.33622190438346));
#62480=CARTESIAN_POINT('Ctrl Pts',(1.49115409285801,-2.89071839202695,-1.42473321730671));
#62481=CARTESIAN_POINT('Ctrl Pts',(1.49722264422245,-2.84709216599334,-1.51324883022158));
#62482=CARTESIAN_POINT('Ctrl Pts',(1.50329119558689,-2.79940039902377,-1.59975070469585));
#62483=CARTESIAN_POINT('Ctrl Pts',(1.50935974695134,-2.74786890398481,-1.6838450192976));
#62484=CARTESIAN_POINT('Ctrl Pts',(1.51543427654096,-2.6962866444614,-1.76802217652837));
#62485=CARTESIAN_POINT('Ctrl Pts',(1.52150880613059,-2.64085733711762,-1.8497866555326));
#62486=CARTESIAN_POINT('Ctrl Pts',(1.52758333572022,-2.58185073403517,-1.92877275739317));
#62487=CARTESIAN_POINT('Ctrl Pts',(1.53366085369367,-2.52281510246989,-2.00779771671344));
#62488=CARTESIAN_POINT('Ctrl Pts',(1.53973837166712,-2.46019895644871,-2.08404123304722));
#62489=CARTESIAN_POINT('Ctrl Pts',(1.54581588964056,-2.39431159208105,-2.1571716581038));
#62490=CARTESIAN_POINT('Ctrl Pts',(1.55190370974851,-2.32831254059168,-2.23042604815372));
#62491=CARTESIAN_POINT('Ctrl Pts',(1.55799152985646,-2.25903151012212,-2.30055648906815));
#62492=CARTESIAN_POINT('Ctrl Pts',(1.56407934996441,-2.18681383281671,-2.36726906436541));
#62493=CARTESIAN_POINT('Ctrl Pts',(1.56939826454235,-2.12371741245714,-2.4255556896251));
#62494=CARTESIAN_POINT('Ctrl Pts',(1.57471717912028,-2.05837998910448,-2.48123379851504));
#62495=CARTESIAN_POINT('Ctrl Pts',(1.58003609369822,-1.99105012604439,-2.53413436069965));
#62496=CARTESIAN_POINT('Ctrl Pts',(1.58621005733018,-1.91289656298442,-2.59553902179205));
#62497=CARTESIAN_POINT('Ctrl Pts',(1.59238402096213,-1.83176267791174,-2.65343255355774));
#62498=CARTESIAN_POINT('Ctrl Pts',(1.59855798459408,-1.74799729359038,-2.70751233129245));
#62499=CARTESIAN_POINT('Ctrl Pts',(1.60472359529448,-1.6643452378476,-2.76151894295278));
#62500=CARTESIAN_POINT('Ctrl Pts',(1.61088920599487,-1.57806912081644,-2.81172182289254));
#62501=CARTESIAN_POINT('Ctrl Pts',(1.61705481669526,-1.48955036306467,-2.8578588625742));
#62502=CARTESIAN_POINT('Ctrl Pts',(1.62321390456034,-1.40112525269132,-2.90394709211749));
#62503=CARTESIAN_POINT('Ctrl Pts',(1.62937299242542,-1.3104626014072,-2.94597783359531));
#62504=CARTESIAN_POINT('Ctrl Pts',(1.63553208029051,-1.21797149036223,-2.98373306633901));
#62505=CARTESIAN_POINT('Ctrl Pts',(1.64168666964908,-1.1255479334542,-3.02146072322019));
#62506=CARTESIAN_POINT('Ctrl Pts',(1.64784125900765,-1.03129897269383,-3.05491891651411));
#62507=CARTESIAN_POINT('Ctrl Pts',(1.65399584836623,-0.935656064375376,
-3.08393665494244));
#62508=CARTESIAN_POINT('Ctrl Pts',(1.66014810554239,-0.840049398395078,
-3.11294339756662));
#62509=CARTESIAN_POINT('Ctrl Pts',(1.66630036271855,-0.743050249374499,
-3.13751290288959));
#62510=CARTESIAN_POINT('Ctrl Pts',(1.67245261989471,-0.645106886623676,
-3.15752350226102));
#62511=CARTESIAN_POINT('Ctrl Pts',(1.67860418890626,-0.547174479389529,
-3.17753186333423));
#62512=CARTESIAN_POINT('Ctrl Pts',(1.68475575791781,-0.448298493720705,
-3.19298224541561));
#62513=CARTESIAN_POINT('Ctrl Pts',(1.69090732692936,-0.348938103326894,
-3.20380395195253));
#62514=CARTESIAN_POINT('Ctrl Pts',(1.69705985078779,-0.249562290207691,
-3.21462733823534));
#62515=CARTESIAN_POINT('Ctrl Pts',(1.70321237464623,-0.149702354603581,
-3.22082057490184));
#62516=CARTESIAN_POINT('Ctrl Pts',(1.70936489850467,-0.0498223097291922,
-3.22236486139501));
#62517=CARTESIAN_POINT('Ctrl Pts',(1.71552398134482,0.050164213625006,-3.22391079419578));
#62518=CARTESIAN_POINT('Ctrl Pts',(1.72168306418496,0.150170454167541,-3.22079787329112));
#62519=CARTESIAN_POINT('Ctrl Pts',(1.72784214702511,0.249732798242018,-3.21305945976451));
#62520=CARTESIAN_POINT('Ctrl Pts',(1.73400465833322,0.349350563929725,-3.20531673863179));
#62521=CARTESIAN_POINT('Ctrl Pts',(1.74016716964133,0.448523510269242,-3.19294345083693));
#62522=CARTESIAN_POINT('Ctrl Pts',(1.74632968094944,0.546795625717764,-3.17602457581737));
#62523=CARTESIAN_POINT('Ctrl Pts',(1.75250246174458,0.645231506255649,-3.15907750642074));
#62524=CARTESIAN_POINT('Ctrl Pts',(1.75867524253972,0.742763133199492,-3.13756981248004));
#62525=CARTESIAN_POINT('Ctrl Pts',(1.76484802333487,0.838946982297594,-3.11163711306344));
#62526=CARTESIAN_POINT('Ctrl Pts',(1.76952645303586,0.911845954626379,-3.09198238771289));
#62527=CARTESIAN_POINT('Ctrl Pts',(1.77420488273686,0.983970983093657,-3.06978684944512));
#62528=CARTESIAN_POINT('Ctrl Pts',(1.77888331243785,1.05513677840373,-3.04512790229898));
#62529=CARTESIAN_POINT('Ctrl Pts',(1.78505684657086,1.14904531065251,-3.01258859710041));
#62530=CARTESIAN_POINT('Ctrl Pts',(1.79123038070387,1.24161168933727,-2.97564417336767));
#62531=CARTESIAN_POINT('Ctrl Pts',(1.79740391483688,1.33239278795469,-2.9344244786851));
#62532=CARTESIAN_POINT('Ctrl Pts',(1.80356911567004,1.42305134637076,-2.89326042410563));
#62533=CARTESIAN_POINT('Ctrl Pts',(1.8097343165032,1.51192902275237,-2.84783274704531));
#62534=CARTESIAN_POINT('Ctrl Pts',(1.81589951733636,1.59859915563183,-2.79832062175034));
#62535=CARTESIAN_POINT('Ctrl Pts',(1.82205821543712,1.68517787337393,-2.74886071926367));
#62536=CARTESIAN_POINT('Ctrl Pts',(1.82821691353788,1.76955330183398,-2.69532514767589));
#62537=CARTESIAN_POINT('Ctrl Pts',(1.83437561163864,1.85132091907383,-2.6379401845189));
#62538=CARTESIAN_POINT('Ctrl Pts',(1.84052984333481,1.93302923688781,-2.58059683802489));
#62539=CARTESIAN_POINT('Ctrl Pts',(1.84668407503097,2.01213314926246,-2.51940989890954));
#62540=CARTESIAN_POINT('Ctrl Pts',(1.85283830672713,2.08825560415908,-2.45464989238755));
#62541=CARTESIAN_POINT('Ctrl Pts',(1.85899022609203,2.16434945754348,-2.38991421816173));
#62542=CARTESIAN_POINT('Ctrl Pts',(1.86514214545692,2.23746374903061,-2.32160842514124));
#62543=CARTESIAN_POINT('Ctrl Pts',(1.87129406482181,2.30725383552129,-2.25004384423332));
#62544=CARTESIAN_POINT('Ctrl Pts',(1.8774453163532,2.37703634581417,-2.17848703215689));
#62545=CARTESIAN_POINT('Ctrl Pts',(1.88359656788458,2.44349506545273,-2.10367244637228));
#62546=CARTESIAN_POINT('Ctrl Pts',(1.88974781941597,2.50632234230045,-2.02594814321236));
#62547=CARTESIAN_POINT('Ctrl Pts',(1.89590004662217,2.56915958443593,-1.94821151188724));
#62548=CARTESIAN_POINT('Ctrl Pts',(1.90205227382837,2.62836396670925,-1.86756458413676));
#62549=CARTESIAN_POINT('Ctrl Pts',(1.90820450103458,2.68366888381557,-1.78438753765545));
#62550=CARTESIAN_POINT('Ctrl Pts',(1.91436332167981,2.73903307207479,-1.70112134902012));
#62551=CARTESIAN_POINT('Ctrl Pts',(1.92052214232505,2.79048920905492,-1.61531998918389));
#62552=CARTESIAN_POINT('Ctrl Pts',(1.92668096297029,2.83781479041402,-1.52739149461015));
#62553=CARTESIAN_POINT('Ctrl Pts',(1.93284323080231,2.88516686062997,-1.43941378510362));
#62554=CARTESIAN_POINT('Ctrl Pts',(1.93900549863433,2.92838358324439,-1.34930696127557));
#62555=CARTESIAN_POINT('Ctrl Pts',(1.94516776646635,2.96728999288113,-1.25750056089352));
#62556=CARTESIAN_POINT('Ctrl Pts',(1.95134033730146,3.00626145208564,-1.16554066480937));
#62557=CARTESIAN_POINT('Ctrl Pts',(1.95751290813657,3.04090805260098,-1.07187592353269));
#62558=CARTESIAN_POINT('Ctrl Pts',(1.96368547897169,3.07110418390735,-0.976952738921796));
#62559=CARTESIAN_POINT('Ctrl Pts',(1.96836716304029,3.09400691773524,-0.904956746813321));
#62560=CARTESIAN_POINT('Ctrl Pts',(1.9730488471089,3.11435045411151,-0.832237156790994));
#62561=CARTESIAN_POINT('Ctrl Pts',(1.9777305311775,3.13209970296924,-0.758992103489897));
#62562=CARTESIAN_POINT('Ctrl Pts',(1.98390158482016,3.15549546509521,-0.662445829466025));
#62563=CARTESIAN_POINT('Ctrl Pts',(1.99007263846282,3.17446435259434,-0.5646462106067));
#62564=CARTESIAN_POINT('Ctrl Pts',(1.99624369210548,3.18887569945224,-0.466035766806547));
#62565=CARTESIAN_POINT('Ctrl Pts',(2.00240636985073,3.20326748596116,-0.367559165784109));
#62566=CARTESIAN_POINT('Ctrl Pts',(2.00856904759598,3.21311396454698,-0.26827435339916));
#62567=CARTESIAN_POINT('Ctrl Pts',(2.01473172534123,3.21833485185556,-0.168636721481037));
#62568=CARTESIAN_POINT('Ctrl Pts',(2.02088786132567,3.22355019712586,-0.0691048561764178));
#62569=CARTESIAN_POINT('Ctrl Pts',(2.02704399731011,3.22414969018264,0.0307786525172366));
#62570=CARTESIAN_POINT('Ctrl Pts',(2.03320013329455,3.22010463541055,0.130551520509984));
#62571=CARTESIAN_POINT('Ctrl Pts',(2.03935175454817,3.21606254716382,0.230251217987271));
#62572=CARTESIAN_POINT('Ctrl Pts',(2.04550337580178,3.20738270066198,0.329840003189144));
#62573=CARTESIAN_POINT('Ctrl Pts',(2.05165499705539,3.19408847376308,0.42885473563181));
#62574=CARTESIAN_POINT('Ctrl Pts',(2.05780427710877,3.1807993064161,0.527831784786608));
#62575=CARTESIAN_POINT('Ctrl Pts',(2.06395355716215,3.16289930586048,0.626234785062532));
#62576=CARTESIAN_POINT('Ctrl Pts',(2.07010283721553,3.14046370306913,0.723605757443461));
#62577=CARTESIAN_POINT('Ctrl Pts',(2.07625142360946,3.11803063108917,0.820965746051489));
#62578=CARTESIAN_POINT('Ctrl Pts',(2.08240001000338,3.09106307162903,0.917293514740002));
#62579=CARTESIAN_POINT('Ctrl Pts',(2.08854859639731,3.05968715741981,1.01214231273091));
#62580=CARTESIAN_POINT('Ctrl Pts',(2.0946981356625,3.02830638075845,1.1070058098231));
#62581=CARTESIAN_POINT('Ctrl Pts',(2.10084767492769,2.99251602889572,1.20038946835059));
#62582=CARTESIAN_POINT('Ctrl Pts',(2.10699721419288,2.95249145840519,1.29186367335891));
#62583=CARTESIAN_POINT('Ctrl Pts',(2.1131533279081,2.91242409779212,1.38343567310666));
#62584=CARTESIAN_POINT('Ctrl Pts',(2.11930944162332,2.86811365356512,1.47309374398627));
#62585=CARTESIAN_POINT('Ctrl Pts',(2.12546555533855,2.81978277213684,1.56043028695944));
#62586=CARTESIAN_POINT('Ctrl Pts',(2.13162510146531,2.77142494327337,1.64781552542007));
#62587=CARTESIAN_POINT('Ctrl Pts',(2.13778464759208,2.71904244094299,1.73287628818928));
#62588=CARTESIAN_POINT('Ctrl Pts',(2.14394419371885,2.6629017123353,1.81523332741048));
#62589=CARTESIAN_POINT('Ctrl Pts',(2.15011404678936,2.60666704184946,1.89772817700813));
#62590=CARTESIAN_POINT('Ctrl Pts',(2.15628389985988,2.54666184486046,1.97750991862143));
#62591=CARTESIAN_POINT('Ctrl Pts',(2.16245375293039,2.48319345044674,2.05423169339742));
#62592=CARTESIAN_POINT('Ctrl Pts',(2.16716175192598,2.4347629394222,2.11277539524198));
#62593=CARTESIAN_POINT('Ctrl Pts',(2.17186975092156,2.38431676498116,2.16953804500934));
#62594=CARTESIAN_POINT('Ctrl Pts',(2.17657774991715,2.3320052453869,2.22438060996494));
#62595=CARTESIAN_POINT('Ctrl Pts',(2.18275082151698,2.26341501071306,2.29628952084339));
#62596=CARTESIAN_POINT('Ctrl Pts',(2.18892389311682,2.19137498214984,2.36514939853218));
#62597=CARTESIAN_POINT('Ctrl Pts',(2.19509696471665,2.11618713243843,2.43061094850698));
#62598=CARTESIAN_POINT('Ctrl Pts',(2.20126084637904,2.04111121592341,2.49597504496293));
#62599=CARTESIAN_POINT('Ctrl Pts',(2.20742472804142,1.96289712224357,2.55795059180821));
#62600=CARTESIAN_POINT('Ctrl Pts',(2.21358860970381,1.88188474811586,2.61622387369829));
#62601=CARTESIAN_POINT('Ctrl Pts',(2.21590376188548,1.85145652366623,2.63811130163582));
#62602=CARTESIAN_POINT('Ctrl Pts',(2.21821891406715,1.82063390650502,2.65947680130358));
#62603=CARTESIAN_POINT('Ctrl Pts',(2.22053406624882,1.78943621037804,2.68030513402633));
#62604=CARTESIAN_POINT('Origin',(-1.72497344927317,0.,0.));
#62605=CARTESIAN_POINT('',(3.71684364332268,1.78943621037804,2.68030513402633));
#62606=CARTESIAN_POINT('',(3.47041119666184,1.78943621037803,2.68030513402633));
#62607=CARTESIAN_POINT('',(-1.72497344927317,1.78943621037804,2.68030513402633));
#62608=CARTESIAN_POINT('',(2.89657344930667,-3.22274890153366,-0.00266085768222635));
#62609=CARTESIAN_POINT('Ctrl Pts',(2.89657344930667,-3.22274890153366,-0.0026608576822207));
#62610=CARTESIAN_POINT('Ctrl Pts',(2.90385415680925,-3.22265127549824,-0.120902506046961));
#62611=CARTESIAN_POINT('Ctrl Pts',(2.91113486431182,-3.21604242047407,-0.238865259363918));
#62612=CARTESIAN_POINT('Ctrl Pts',(2.91841557181439,-3.20303727403663,-0.355906987332332));
#62613=CARTESIAN_POINT('Ctrl Pts',(2.92578180427762,-3.18987935884191,-0.474323580198954));
#62614=CARTESIAN_POINT('Ctrl Pts',(2.93314803674085,-3.17017407925754,-0.591797313652501));
#62615=CARTESIAN_POINT('Ctrl Pts',(2.94051426920408,-3.14408976635058,-0.707684324843768));
#62616=CARTESIAN_POINT('Ctrl Pts',(2.94687552402374,-3.12156414527831,-0.807760831002979));
#62617=CARTESIAN_POINT('Ctrl Pts',(2.9532367788434,-3.09428217040264,-0.906654364654217));
#62618=CARTESIAN_POINT('Ctrl Pts',(2.95959803366306,-3.06238066868043,-1.00396324763031));
#62619=CARTESIAN_POINT('Ctrl Pts',(2.96577029116436,-3.03142698282921,-1.09838101580951));
#62620=CARTESIAN_POINT('Ctrl Pts',(2.97194254866565,-2.99604816420421,-1.19153210136813));
#62621=CARTESIAN_POINT('Ctrl Pts',(2.97811480616694,-2.95636635020544,-1.28297138154869));
#62622=CARTESIAN_POINT('Ctrl Pts',(2.98427870432196,-2.91673827894566,-1.37428682169089));
#62623=CARTESIAN_POINT('Ctrl Pts',(2.99044260247699,-2.87281896696189,-1.46389466950883));
#62624=CARTESIAN_POINT('Ctrl Pts',(2.99660650063201,-2.8247801555252,-1.55136541003435));
#62625=CARTESIAN_POINT('Ctrl Pts',(3.00276387187365,-2.77679221208686,-1.6387435283373));
#62626=CARTESIAN_POINT('Ctrl Pts',(3.00892124311529,-2.72469364943321,-1.72398865971088));
#62627=CARTESIAN_POINT('Ctrl Pts',(3.01507861435693,-2.66870368702595,-1.80669261175058));
#62628=CARTESIAN_POINT('Ctrl Pts',(3.02123148816823,-2.61275462047277,-1.88933615566336));
#62629=CARTESIAN_POINT('Ctrl Pts',(3.02738436197953,-2.55292004798889,-1.96944185189964));
#62630=CARTESIAN_POINT('Ctrl Pts',(3.03353723579083,-2.48946390168153,-2.04662821360515));
#62631=CARTESIAN_POINT('Ctrl Pts',(3.0396877786396,-2.42603179518119,-2.12378533393139));
#62632=CARTESIAN_POINT('Ctrl Pts',(3.04583832148837,-2.35898111656308,-2.19802498210599));
#62633=CARTESIAN_POINT('Ctrl Pts',(3.05198886433714,-2.28861715374865,-2.26899737462771));
#62634=CARTESIAN_POINT('Ctrl Pts',(3.05813872230041,-2.21826102621949,-2.33996186411328));
#62635=CARTESIAN_POINT('Ctrl Pts',(3.06428858026368,-2.14459265383724,-2.40765951280687));
#62636=CARTESIAN_POINT('Ctrl Pts',(3.07043843822696,-2.06795467750557,-2.47177689411541));
#62637=CARTESIAN_POINT('Ctrl Pts',(3.07658925637862,-1.99130473554876,-2.53590428618606));
#62638=CARTESIAN_POINT('Ctrl Pts',(3.08274007453028,-1.91168460190081,-2.59645002181334));
#62639=CARTESIAN_POINT('Ctrl Pts',(3.08889089268194,-1.82946973436362,-2.65314116728596));
#62640=CARTESIAN_POINT('Ctrl Pts',(3.09504828879816,-1.74716694250944,-2.70989294084684));
#62641=CARTESIAN_POINT('Ctrl Pts',(3.10120568491439,-1.66226423382163,-2.76278164543452));
#62642=CARTESIAN_POINT('Ctrl Pts',(3.10736308103061,-1.57516567043588,-2.81157796854014));
#62643=CARTESIAN_POINT('Ctrl Pts',(3.11352391352038,-1.48801849832103,-2.86040152432513));
#62644=CARTESIAN_POINT('Ctrl Pts',(3.11968474601016,-1.39867341941258,-2.90512795579674));
#62645=CARTESIAN_POINT('Ctrl Pts',(3.12584557849993,-1.30755680027941,-2.94557511812941));
#62646=CARTESIAN_POINT('Ctrl Pts',(3.13201671107229,-1.21628784642471,-2.9860899026727));
#62647=CARTESIAN_POINT('Ctrl Pts',(3.13818784364465,-1.12324184126048,-3.02231096981099));
#62648=CARTESIAN_POINT('Ctrl Pts',(3.14435897621701,-1.02886284865085,-3.0541052374085));
#62649=CARTESIAN_POINT('Ctrl Pts',(3.14905440161224,-0.957052769466965,
-3.07829651992425));
#62650=CARTESIAN_POINT('Ctrl Pts',(3.15374982700747,-0.884471360269048,
-3.09992604749025));
#62651=CARTESIAN_POINT('Ctrl Pts',(3.1584452524027,-0.811317954453893,-3.11895507169962));
#62652=CARTESIAN_POINT('Ctrl Pts',(3.16461750160968,-0.715156049402839,
-3.14396918004966));
#62653=CARTESIAN_POINT('Ctrl Pts',(3.17078975081665,-0.617666974353875,
-3.16457593251688));
#62654=CARTESIAN_POINT('Ctrl Pts',(3.17696200002363,-0.519291210154257,
-3.18063738919678));
#62655=CARTESIAN_POINT('Ctrl Pts',(3.18312588983436,-0.421048681338786,
-3.19667709301542));
#62656=CARTESIAN_POINT('Ctrl Pts',(3.18928977964509,-0.321922275196099,
-3.20818366725772));
#62657=CARTESIAN_POINT('Ctrl Pts',(3.19545366945582,-0.222366164594063,
-3.21506933849703));
#62658=CARTESIAN_POINT('Ctrl Pts',(3.2016110323146,-0.122915474103324,-3.22194771848898));
#62659=CARTESIAN_POINT('Ctrl Pts',(3.20776839517339,-0.0230364147158,-3.22421489357896));
#62660=CARTESIAN_POINT('Ctrl Pts',(3.21392575803217,0.0768091053907777,
-3.22183455873033));
#62661=CARTESIAN_POINT('Ctrl Pts',(3.22007862343751,0.176581696454737,-3.21945596252297));
#62662=CARTESIAN_POINT('Ctrl Pts',(3.22623148884285,0.276320364000828,-3.21243661580049));
#62663=CARTESIAN_POINT('Ctrl Pts',(3.23238435424819,0.375561488131964,-3.20079226616351));
#62664=CARTESIAN_POINT('Ctrl Pts',(3.23853488867949,0.474765015392593,-3.18915232791453));
#62665=CARTESIAN_POINT('Ctrl Pts',(3.24468542311079,0.573470942832583,-3.17289091883314));
#62666=CARTESIAN_POINT('Ctrl Pts',(3.25083595754209,0.671219958122833,-3.1520757177323));
#62667=CARTESIAN_POINT('Ctrl Pts',(3.25698580708638,0.76895808866282,-3.13126283448873));
#62668=CARTESIAN_POINT('Ctrl Pts',(3.26313565663066,0.865739094052329,-3.10589725785115));
#62669=CARTESIAN_POINT('Ctrl Pts',(3.26928550617495,0.961114048533461,-3.07609774685585));
#62670=CARTESIAN_POINT('Ctrl Pts',(3.2754363159161,1.05650389422965,-3.04629358316184));
#62671=CARTESIAN_POINT('Ctrl Pts',(3.28158712565725,1.15048683832345,-3.01205423960778));
#62672=CARTESIAN_POINT('Ctrl Pts',(3.2877379353984,1.24263027357175,-2.97354797602174));
#62673=CARTESIAN_POINT('Ctrl Pts',(3.2938953231697,1.33487225231609,-2.93500053161991));
#62674=CARTESIAN_POINT('Ctrl Pts',(3.300052710941,1.42527039219857,-2.89217722258056));
#62675=CARTESIAN_POINT('Ctrl Pts',(3.3062100987123,1.51341331384771,-2.84529395739149));
#62676=CARTESIAN_POINT('Ctrl Pts',(3.31237092288049,1.60160542747125,-2.79838452696602));
#62677=CARTESIAN_POINT('Ctrl Pts',(3.31853174704868,1.68753944272647,-2.74741084962619));
#62678=CARTESIAN_POINT('Ctrl Pts',(3.32469257121686,1.77083159789182,-2.69263310059278));
#62679=CARTESIAN_POINT('Ctrl Pts',(3.33086369559309,1.85426300821244,-2.63776376929774));
#62680=CARTESIAN_POINT('Ctrl Pts',(3.33703481996932,1.93504338424352,-2.57907791786674));
#62681=CARTESIAN_POINT('Ctrl Pts',(3.34320594434554,2.01282066713522,-2.51687713733772));
#62682=CARTESIAN_POINT('Ctrl Pts',(3.34790145327781,2.07200014631612,-2.46954956739062));
#62683=CARTESIAN_POINT('Ctrl Pts',(3.35259696221008,2.12944165980346,-2.42018790724988));
#62684=CARTESIAN_POINT('Ctrl Pts',(3.35729247114235,2.18500482297474,-2.36893889454269));
#62685=CARTESIAN_POINT('Ctrl Pts',(3.36346471603464,2.25804258203986,-2.30157208479331));
#62686=CARTESIAN_POINT('Ctrl Pts',(3.36963696092693,2.32809045580273,-2.23070574890648));
#62687=CARTESIAN_POINT('Ctrl Pts',(3.37580920581922,2.39479423544368,-2.15663583675727));
#62688=CARTESIAN_POINT('Ctrl Pts',(3.38197309122092,2.46140767362416,-2.08266624252222));
#62689=CARTESIAN_POINT('Ctrl Pts',(3.38813697662262,2.5246857317135,-2.00550201584714));
#62690=CARTESIAN_POINT('Ctrl Pts',(3.39430086202433,2.58430899788456,-1.92547775005397));
#62691=CARTESIAN_POINT('Ctrl Pts',(3.40045822038607,2.64386912799526,-1.8455382232763));
#62692=CARTESIAN_POINT('Ctrl Pts',(3.40661557874781,2.6997819022575,-1.76274502481236));
#62693=CARTESIAN_POINT('Ctrl Pts',(3.41277293710955,2.75176702188678,-1.67746708455229));
#62694=CARTESIAN_POINT('Ctrl Pts',(3.41892579790345,2.80371416961501,-1.59225143453088));
#62695=CARTESIAN_POINT('Ctrl Pts',(3.42507865869735,2.85173914117513,-1.50455502092003));
#62696=CARTESIAN_POINT('Ctrl Pts',(3.43123151949125,2.89560449933464,-1.41477635898151));
#62697=CARTESIAN_POINT('Ctrl Pts',(3.43738204924227,2.93945323887819,-1.32503171014963));
#62698=CARTESIAN_POINT('Ctrl Pts',(3.44353257899329,2.97914530582987,-1.23320677031985));
#62699=CARTESIAN_POINT('Ctrl Pts',(3.44968310874432,3.0144892770641,-1.13972451099621));
#62700=CARTESIAN_POINT('Ctrl Pts',(3.45583295354482,3.04982931223552,-1.04625266227533));
#62701=CARTESIAN_POINT('Ctrl Pts',(3.46198279834532,3.08082206077932,-0.951124267311737));
#62702=CARTESIAN_POINT('Ctrl Pts',(3.46813264314583,3.10732468480901,-0.854781179996733));
#62703=CARTESIAN_POINT('Ctrl Pts',(3.47428344808497,3.1338314465355,-0.758423051209431));
#62704=CARTESIAN_POINT('Ctrl Pts',(3.4804342530241,3.15584657612648,-0.660850272249102));
#62705=CARTESIAN_POINT('Ctrl Pts',(3.48658505796324,3.17327769977594,-0.562517735369062));
#62706=CARTESIAN_POINT('Ctrl Pts',(3.49274244087121,3.19072746511363,-0.464080036909504));
#62707=CARTESIAN_POINT('Ctrl Pts',(3.49889982377918,3.20358335904078,-0.364881386549443));
#62708=CARTESIAN_POINT('Ctrl Pts',(3.50505720668715,3.21180456834944,-0.265384583632243));
#62709=CARTESIAN_POINT('Ctrl Pts',(3.51121802595036,3.220030365808,-0.165832252844545));
#62710=CARTESIAN_POINT('Ctrl Pts',(3.51737884521358,3.22361631196527,-0.0659818722363817));
#62711=CARTESIAN_POINT('Ctrl Pts',(3.52353966447679,3.22257376432983,0.0337030555450616));
#62712=CARTESIAN_POINT('Ctrl Pts',(3.52971078393028,3.22152947367312,0.133554645206927));
#62713=CARTESIAN_POINT('Ctrl Pts',(3.53588190338377,3.21584125693355,0.233239795633299));
#62714=CARTESIAN_POINT('Ctrl Pts',(3.54205302283725,3.20557245304592,0.332299278923597));
#62715=CARTESIAN_POINT('Ctrl Pts',(3.54674857851883,3.19775900188832,0.407672851430785));
#62716=CARTESIAN_POINT('Ctrl Pts',(3.55144413420041,3.18729466636823,0.482684279285471));
#62717=CARTESIAN_POINT('Ctrl Pts',(3.55613968988199,3.1742269775727,0.557136121023987));
#62718=CARTESIAN_POINT('Ctrl Pts',(3.56231279094659,3.15704729340199,0.655015642568272));
#62719=CARTESIAN_POINT('Ctrl Pts',(3.56848589201118,3.13530584823963,0.752272099629848));
#62720=CARTESIAN_POINT('Ctrl Pts',(3.57465899307578,3.10906010156392,0.848447315608531));
#62721=CARTESIAN_POINT('Ctrl Pts',(3.58082173739428,3.08285838794904,0.944461176332702));
#62722=CARTESIAN_POINT('Ctrl Pts',(3.58698448171277,3.0521675228787,1.03939698999922));
#62723=CARTESIAN_POINT('Ctrl Pts',(3.59314722603127,3.01709620244243,1.1328053971038));
#62724=CARTESIAN_POINT('Ctrl Pts',(3.59930404400262,2.98205860802314,1.22612397886146));
#62725=CARTESIAN_POINT('Ctrl Pts',(3.60546086197397,2.94264907967364,1.31791766835387));
#62726=CARTESIAN_POINT('Ctrl Pts',(3.61161767994533,2.89902635809779,1.40775130529305));
#62727=CARTESIAN_POINT('Ctrl Pts',(3.61777022437955,2.85543391568907,1.49752258739491));
#62728=CARTESIAN_POINT('Ctrl Pts',(3.62392276881378,2.80763428156778,1.58533613155658));
#62729=CARTESIAN_POINT('Ctrl Pts',(3.630075313248,2.75583426623992,1.67077678327114));
#62730=CARTESIAN_POINT('Ctrl Pts',(3.6362252329377,2.70405634938012,1.75618098504453));
#62731=CARTESIAN_POINT('Ctrl Pts',(3.6423751526274,2.64828166987867,1.83921393652311));
#62732=CARTESIAN_POINT('Ctrl Pts',(3.6485250723171,2.58876244520109,1.91948601579081));
#62733=CARTESIAN_POINT('Ctrl Pts',(3.65467598423213,2.52923361771805,1.99977104612038));
#62734=CARTESIAN_POINT('Ctrl Pts',(3.66082689614716,2.46595928868833,2.0772939592081));
#62735=CARTESIAN_POINT('Ctrl Pts',(3.66697780806219,2.39923406070027,2.15169549064817));
#62736=CARTESIAN_POINT('Ctrl Pts',(3.67312908450406,2.332504878317,2.22610143141091));
#62737=CARTESIAN_POINT('Ctrl Pts',(3.67928036094594,2.26232468623143,2.29738530431221));
#62738=CARTESIAN_POINT('Ctrl Pts',(3.68543163738781,2.18902626992494,2.36522336198477));
#62739=CARTESIAN_POINT('Ctrl Pts',(3.69158813076747,2.11566568875208,2.43311895355781));
#62740=CARTESIAN_POINT('Ctrl Pts',(3.69774462414714,2.03918192636869,2.49756260392495));
#62741=CARTESIAN_POINT('Ctrl Pts',(3.7039011175268,1.95994206271907,2.55826985935506));
#62742=CARTESIAN_POINT('Ctrl Pts',(3.7082152927921,1.90441456700022,2.60081059214712));
#62743=CARTESIAN_POINT('Ctrl Pts',(3.71252946805739,1.84753438604866,2.64151739378657));
#62744=CARTESIAN_POINT('Ctrl Pts',(3.71684364332268,1.78943621037804,2.68030513402633));
#62745=CARTESIAN_POINT('Ctrl Pts',(2.46694827513675,1.78943621037803,2.68030513402633));
#62746=CARTESIAN_POINT('Ctrl Pts',(2.47309858708958,1.70631803001642,2.7357968315169));
#62747=CARTESIAN_POINT('Ctrl Pts',(2.47924889904241,1.62062286331172,2.78741412951648));
#62748=CARTESIAN_POINT('Ctrl Pts',(2.48539921099525,1.53275181053506,2.83492318234577));
#62749=CARTESIAN_POINT('Ctrl Pts',(2.49177457642762,1.44166536212804,2.88417069620453));
#62750=CARTESIAN_POINT('Ctrl Pts',(2.49814994186,1.34824116592263,2.92900328203538));
#62751=CARTESIAN_POINT('Ctrl Pts',(2.50452530729238,1.25295192047284,2.9692135402297));
#62752=CARTESIAN_POINT('Ctrl Pts',(2.51068485063132,1.16088845472983,3.00806258043689));
#62753=CARTESIAN_POINT('Ctrl Pts',(2.51684439397026,1.06708461404918,3.04259710715594));
#62754=CARTESIAN_POINT('Ctrl Pts',(2.5230039373092,0.971983818768544,3.07268042896623));
#62755=CARTESIAN_POINT('Ctrl Pts',(2.52948721378829,0.87188471803028,3.10434486932706));
#62756=CARTESIAN_POINT('Ctrl Pts',(2.53597049026739,0.770349159965806,3.13107732305021));
#62757=CARTESIAN_POINT('Ctrl Pts',(2.54245376674648,0.667906563794865,3.1527794696965));
#62758=CARTESIAN_POINT('Ctrl Pts',(2.54893704322558,0.565463967623921,3.17448161634279));
#62759=CARTESIAN_POINT('Ctrl Pts',(2.55542031970468,0.462114891302979,3.19115344258992));
#62760=CARTESIAN_POINT('Ctrl Pts',(2.56190359618377,0.358393190207404,3.20276004154432));
#62761=CARTESIAN_POINT('Ctrl Pts',(2.56807585854909,0.259647200551854,3.21380985164366));
#62762=CARTESIAN_POINT('Ctrl Pts',(2.57424812091441,0.160215915954576,3.2203080957865));
#62763=CARTESIAN_POINT('Ctrl Pts',(2.58042038327972,0.0605549853338471,
3.22218104026624));
#62764=CARTESIAN_POINT('Ctrl Pts',(2.58658428659543,-0.0389709752201438,
3.22405144823102));
#62765=CARTESIAN_POINT('Ctrl Pts',(2.59274818991113,-0.138725533162269,
3.22130899885287));
#62766=CARTESIAN_POINT('Ctrl Pts',(2.59891209322684,-0.238246639486325,
3.21393156449752));
#62767=CARTESIAN_POINT('Ctrl Pts',(2.60506946991764,-0.337662368276467,
3.20656194170966));
#62768=CARTESIAN_POINT('Ctrl Pts',(2.61122684660845,-0.436844706088377,
3.19456712292281));
#62769=CARTESIAN_POINT('Ctrl Pts',(2.61738422329925,-0.535331285272566,
3.17797702595667));
#62770=CARTESIAN_POINT('Ctrl Pts',(2.62353710297378,-0.633745935164174,
3.16139904550376));
#62771=CARTESIAN_POINT('Ctrl Pts',(2.62968998264831,-0.731465409659298,
3.1402325313951));
#62772=CARTESIAN_POINT('Ctrl Pts',(2.63584286232284,-0.828033067762345,
3.11455916642983));
#62773=CARTESIAN_POINT('Ctrl Pts',(2.64199341128746,-0.92456414605074,3.08889552653142));
#62774=CARTESIAN_POINT('Ctrl Pts',(2.64814396025207,-1.01994385556388,3.05872853944413));
#62775=CARTESIAN_POINT('Ctrl Pts',(2.65429450921669,-1.11372722245748,3.02419067461976));
#62776=CARTESIAN_POINT('Ctrl Pts',(2.66044437354207,-1.20750014999481,2.98965665432655));
#62777=CARTESIAN_POINT('Ctrl Pts',(2.66659423786746,-1.29967668058446,2.95075287371668));
#62778=CARTESIAN_POINT('Ctrl Pts',(2.67274410219285,-1.38982940309251,2.90766087995136));
#62779=CARTESIAN_POINT('Ctrl Pts',(2.67889492694671,-1.47999620481225,2.86456215648021));
#62780=CARTESIAN_POINT('Ctrl Pts',(2.68504575170057,-1.56813817873332,2.81727410803243));
#62781=CARTESIAN_POINT('Ctrl Pts',(2.69119657645443,-1.65385112258556,2.76602495050614));
#62782=CARTESIAN_POINT('Ctrl Pts',(2.69735397950775,-1.73965573632506,2.71472098206936));
#62783=CARTESIAN_POINT('Ctrl Pts',(2.70351138256106,-1.82302575882768,2.6594476682448));
#62784=CARTESIAN_POINT('Ctrl Pts',(2.70966878561438,-1.9035847918134,2.60047736057762));
#62785=CARTESIAN_POINT('Ctrl Pts',(2.71582962523795,-1.98418878641267,2.54147414039789));
#62786=CARTESIAN_POINT('Ctrl Pts',(2.72199046486152,-2.06197832891767,2.47877008981964));
#62787=CARTESIAN_POINT('Ctrl Pts',(2.72815130448509,-2.13661066740312,2.41267743771089));
#62788=CARTESIAN_POINT('Ctrl Pts',(2.73432244444248,-2.21136778401089,2.34647428501759));
#62789=CARTESIAN_POINT('Ctrl Pts',(2.74049358439987,-2.2829568412898,2.27687151723568));
#62790=CARTESIAN_POINT('Ctrl Pts',(2.74666472435726,-2.35107237070964,2.2042178363732));
#62791=CARTESIAN_POINT('Ctrl Pts',(2.75136008787931,-2.40289864176029,2.1489386747888));
#62792=CARTESIAN_POINT('Ctrl Pts',(2.75605545140136,-2.45271484194789,2.09189407818914));
#62793=CARTESIAN_POINT('Ctrl Pts',(2.76075081492341,-2.50040295090739,2.03324928269841));
#62794=CARTESIAN_POINT('Ctrl Pts',(2.76690134343908,-2.56287033445203,1.95642956783138));
#62795=CARTESIAN_POINT('Ctrl Pts',(2.77305187195475,-2.62191048814613,1.87658535584688));
#62796=CARTESIAN_POINT('Ctrl Pts',(2.77920240047041,-2.67721494782827,1.79405621027461));
#62797=CARTESIAN_POINT('Ctrl Pts',(2.78534493015722,-2.73244748346243,1.71163439474877));
#62798=CARTESIAN_POINT('Ctrl Pts',(2.79148745984403,-2.78395373460758,1.62653494104741));
#62799=CARTESIAN_POINT('Ctrl Pts',(2.79762998953084,-2.83146485192257,1.53913103887456));
#62800=CARTESIAN_POINT('Ctrl Pts',(2.80376620097837,-2.87892709904517,1.45181704082852));
#62801=CARTESIAN_POINT('Ctrl Pts',(2.80990241242589,-2.92240217001727,1.36220368580563));
#62802=CARTESIAN_POINT('Ctrl Pts',(2.81603862387342,-2.96166458789849,1.27069289416762));
#62803=CARTESIAN_POINT('Ctrl Pts',(2.82217019162361,-3.00089729318147,1.17925135510072));
#62804=CARTESIAN_POINT('Ctrl Pts',(2.8283017593738,-3.03592351039349,1.08591563407114));
#62805=CARTESIAN_POINT('Ctrl Pts',(2.834433327124,-3.06656427008512,0.991111063371452));
#62806=CARTESIAN_POINT('Ctrl Pts',(2.84056261682008,-3.09719364585161,0.896341715301602));
#62807=CARTESIAN_POINT('Ctrl Pts',(2.84669190651617,-3.12344066455406,0.800105016553149));
#62808=CARTESIAN_POINT('Ctrl Pts',(2.85282119621226,-3.14517528780142,0.702844201443844));
#62809=CARTESIAN_POINT('Ctrl Pts',(2.85894917939328,-3.16690527811184,0.605604118381222));
#62810=CARTESIAN_POINT('Ctrl Pts',(2.86507716257431,-3.18412469451779,0.507340780662209));
#62811=CARTESIAN_POINT('Ctrl Pts',(2.87120514575533,-3.19675425206134,0.408509258680556));
#62812=CARTESIAN_POINT('Ctrl Pts',(2.87733501507794,-3.20938769687629,0.30964731718919));
#62813=CARTESIAN_POINT('Ctrl Pts',(2.88346488440056,-3.21742840928701,0.210217276517037));
#62814=CARTESIAN_POINT('Ctrl Pts',(2.88959475372317,-3.22084886858185,0.110680297501366));
#62815=CARTESIAN_POINT('Ctrl Pts',(2.89192098557315,-3.22214690299898,0.0729068836403979));
#62816=CARTESIAN_POINT('Ctrl Pts',(2.89424721742312,-3.2227800936602,0.0351180933736112));
#62817=CARTESIAN_POINT('Ctrl Pts',(2.8965734492731,-3.22274890153411,-0.00266085713696655));
#62818=CARTESIAN_POINT('',(2.65002655068888,-3.22274940472809,0.00195878144663014));
#62819=CARTESIAN_POINT('Ctrl Pts',(2.22053406624882,1.78943621037804,2.68030513402633));
#62820=CARTESIAN_POINT('Ctrl Pts',(2.22698785384915,1.70246857774578,2.7383668184918));
#62821=CARTESIAN_POINT('Ctrl Pts',(2.23344164144948,1.61258358561053,2.79225052418815));
#62822=CARTESIAN_POINT('Ctrl Pts',(2.23989542904981,1.52022580284294,2.84165991471016));
#62823=CARTESIAN_POINT('Ctrl Pts',(2.24604743268732,1.43218673947039,2.88875888496492));
#62824=CARTESIAN_POINT('Ctrl Pts',(2.25219943632483,1.34190135858284,2.93179231733081));
#62825=CARTESIAN_POINT('Ctrl Pts',(2.25835143996234,1.24978285820519,2.97054883310079));
#62826=CARTESIAN_POINT('Ctrl Pts',(2.26450181180627,1.15768879187974,3.00929506886484));
#62827=CARTESIAN_POINT('Ctrl Pts',(2.27065218365019,1.06376297245931,3.04376647412016));
#62828=CARTESIAN_POINT('Ctrl Pts',(2.27680255549412,0.968439931846692,3.07379922260787));
#62829=CARTESIAN_POINT('Ctrl Pts',(2.28295294065452,0.873116684845393,3.10383203612099));
#62830=CARTESIAN_POINT('Ctrl Pts',(2.28910332581493,0.776396625153268,3.12942604385474));
#62831=CARTESIAN_POINT('Ctrl Pts',(2.29525371097533,0.67872988283739,3.15046715720757));
#62832=CARTESIAN_POINT('Ctrl Pts',(2.30140575411951,0.581036812109558,3.17151394269696));
#62833=CARTESIAN_POINT('Ctrl Pts',(2.30755779726369,0.482396976245193,3.18800530393077));
#62834=CARTESIAN_POINT('Ctrl Pts',(2.31370984040787,0.383270145989764,3.19987836607784));
#62835=CARTESIAN_POINT('Ctrl Pts',(2.31986883114248,0.284031370385205,3.21176483664404));
#62836=CARTESIAN_POINT('Ctrl Pts',(2.32602782187709,0.184304934504294,3.21902254740279));
#62837=CARTESIAN_POINT('Ctrl Pts',(2.3321868126117,0.0845549822087228,3.2216405785692));
#62838=CARTESIAN_POINT('Ctrl Pts',(2.33834986641296,-0.0152607748138019,
3.22426033684246));
#62839=CARTESIAN_POINT('Ctrl Pts',(2.34451292021421,-0.115099645594101,
3.2222343312196));
#62840=CARTESIAN_POINT('Ctrl Pts',(2.35067597401546,-0.214500279457155,
3.21560370577794));
#62841=CARTESIAN_POINT('Ctrl Pts',(2.35684856104054,-0.314054669643128,
3.20896282385654));
#62842=CARTESIAN_POINT('Ctrl Pts',(2.36302114806561,-0.413169039665234,
3.19770315608448));
#62843=CARTESIAN_POINT('Ctrl Pts',(2.36919373509068,-0.511390087318214,
3.18191730582249));
#62844=CARTESIAN_POINT('Ctrl Pts',(2.37127081294605,-0.544441506793105,
3.17660536127248));
#62845=CARTESIAN_POINT('Ctrl Pts',(2.37334789080142,-0.577391886665494,
3.17078132761479));
#62846=CARTESIAN_POINT('Ctrl Pts',(2.37542496865678,-0.610224342440297,
3.16445000187921));
#62847=CARTESIAN_POINT('Ctrl Pts',(2.38159736003055,-0.707791588790864,
3.14563538679203));
#62848=CARTESIAN_POINT('Ctrl Pts',(2.38776975140431,-0.804659501487889,
3.12227111501522));
#62849=CARTESIAN_POINT('Ctrl Pts',(2.39394214277808,-0.900371102754934,
3.09442231116308));
#62850=CARTESIAN_POINT('Ctrl Pts',(2.40010617797621,-0.995953129777267,
3.06661120898637));
#62851=CARTESIAN_POINT('Ctrl Pts',(2.40627021317434,-1.09038154341743,3.03432776212098));
#62852=CARTESIAN_POINT('Ctrl Pts',(2.41243424837247,-1.18320860454814,2.99768826942083));
#62853=CARTESIAN_POINT('Ctrl Pts',(2.41859175963029,-1.27593741863991,2.96108755551667));
#62854=CARTESIAN_POINT('Ctrl Pts',(2.42474927088812,-1.36706784796038,2.92014012026545));
#62855=CARTESIAN_POINT('Ctrl Pts',(2.43090678214594,-1.45616732866535,2.87501204752739));
#62856=CARTESIAN_POINT('Ctrl Pts',(2.43705979988732,-1.54520178797373,2.82991690753249));
#62857=CARTESIAN_POINT('Ctrl Pts',(2.44321281762869,-1.63220785903381,2.78064739136689));
#62858=CARTESIAN_POINT('Ctrl Pts',(2.44936583537007,-1.71677384112069,2.72741730231069));
#62859=CARTESIAN_POINT('Ctrl Pts',(2.45551652450848,-1.80130781930221,2.67420735812468));
#62860=CARTESIAN_POINT('Ctrl Pts',(2.46166721364688,-1.88340317621615,2.61704005043262));
#62861=CARTESIAN_POINT('Ctrl Pts',(2.46781790278529,-1.96267445496097,2.556174201095));
#62862=CARTESIAN_POINT('Ctrl Pts',(2.47396790923187,-2.04193693504074,2.49531510752353));
#62863=CARTESIAN_POINT('Ctrl Pts',(2.48011791567845,-2.11837561563714,2.43075855299986));
#62864=CARTESIAN_POINT('Ctrl Pts',(2.48626792212503,-2.1916364039487,2.36280499309334));
#62865=CARTESIAN_POINT('Ctrl Pts',(2.49241889078954,-2.26490865449929,2.29484080130632));
#62866=CARTESIAN_POINT('Ctrl Pts',(2.49856985945406,-2.33500170669935,2.22347884386782));
#62867=CARTESIAN_POINT('Ctrl Pts',(2.50472082811857,-2.40159750585018,2.14905723106534));
#62868=CARTESIAN_POINT('Ctrl Pts',(2.51087837698962,-2.46826454810708,2.07455600322823));
#62869=CARTESIAN_POINT('Ctrl Pts',(2.51703592586067,-2.53142657611034,1.9969889081573));
#62870=CARTESIAN_POINT('Ctrl Pts',(2.52319347473172,-2.59080520688077,1.91672792604988));
#62871=CARTESIAN_POINT('Ctrl Pts',(2.52935446145952,-2.65021698967818,1.83642213296905));
#62872=CARTESIAN_POINT('Ctrl Pts',(2.53551544818731,-2.7058409267516,1.75341981840851));
#62873=CARTESIAN_POINT('Ctrl Pts',(2.54167643491511,-2.7574426183601,1.6681210294674));
#62874=CARTESIAN_POINT('Ctrl Pts',(2.54784772257175,-2.80913058597878,1.5826796242873));
#62875=CARTESIAN_POINT('Ctrl Pts',(2.55401901022839,-2.85678266769303,1.49493445708755));
#62876=CARTESIAN_POINT('Ctrl Pts',(2.56019029788503,-2.9002109070008,1.40530931022803));
#62877=CARTESIAN_POINT('Ctrl Pts',(2.5648842610555,-2.93324300130765,1.33713923585895));
#62878=CARTESIAN_POINT('Ctrl Pts',(2.56957822422597,-2.96383242873378,1.26788202310293));
#62879=CARTESIAN_POINT('Ctrl Pts',(2.57427218739644,-2.99191570283412,1.19773034930013));
#62880=CARTESIAN_POINT('Ctrl Pts',(2.5812281548249,-3.03353220744489,1.09377283188832));
#62881=CARTESIAN_POINT('Ctrl Pts',(2.58818412225336,-3.06976700649434,0.987543649318438));
#62882=CARTESIAN_POINT('Ctrl Pts',(2.59514008968182,-3.10039628824057,0.879579682782686));
#62883=CARTESIAN_POINT('Ctrl Pts',(2.60207254730286,-3.13092204901395,0.77198061330658));
#62884=CARTESIAN_POINT('Ctrl Pts',(2.6090050049239,-3.15587999011657,0.662658666473282));
#62885=CARTESIAN_POINT('Ctrl Pts',(2.61593746254494,-3.17509501101313,0.552167758511445));
#62886=CARTESIAN_POINT('Ctrl Pts',(2.62282775611551,-3.19419316381541,0.442348869691205));
#62887=CARTESIAN_POINT('Ctrl Pts',(2.62971804968608,-3.20761793720828,0.331375411940045));
#62888=CARTESIAN_POINT('Ctrl Pts',(2.63660834325665,-3.21524508618567,0.219810368861196));
#62889=CARTESIAN_POINT('Ctrl Pts',(2.6410810790674,-3.22019614117566,0.147389512145142));
#62890=CARTESIAN_POINT('Ctrl Pts',(2.64555381487814,-3.22270518073489,0.074719756395053));
#62891=CARTESIAN_POINT('Ctrl Pts',(2.65002655068888,-3.22274940472809,0.00195878144664628));
#62892=CARTESIAN_POINT('Ctrl Pts',(2.65002655072688,-3.22274940472846,0.00195878082847808));
#62893=CARTESIAN_POINT('Ctrl Pts',(2.65623082264165,-3.22281074919503,-0.0989702461627191));
#62894=CARTESIAN_POINT('Ctrl Pts',(2.66243509455643,-3.21812646153104,-0.199913400276856));
#62895=CARTESIAN_POINT('Ctrl Pts',(2.6686393664712,-3.20871911843152,-0.30039837135389));
#62896=CARTESIAN_POINT('Ctrl Pts',(2.67484458885946,-3.19931033415883,-0.400898736388821));
#62897=CARTESIAN_POINT('Ctrl Pts',(2.68104981124771,-3.18517709478693,-0.500940356932082));
#62898=CARTESIAN_POINT('Ctrl Pts',(2.68725503363597,-3.16639382626989,-0.60005641356455));
#62899=CARTESIAN_POINT('Ctrl Pts',(2.69346275534655,-3.14760299227988,-0.699212391888294));
#62900=CARTESIAN_POINT('Ctrl Pts',(2.69967047705712,-3.12415848302303,-0.797441648834382));
#62901=CARTESIAN_POINT('Ctrl Pts',(2.7058781987677,-3.09618558234046,-0.894288768914743));
#62902=CARTESIAN_POINT('Ctrl Pts',(2.71209432393503,-3.06817481445441,-0.991266991938087));
#62903=CARTESIAN_POINT('Ctrl Pts',(2.71831044910236,-3.03562353304882,-1.08685893474145));
#62904=CARTESIAN_POINT('Ctrl Pts',(2.72452657426969,-2.99870658257103,-1.18062542499523));
#62905=CARTESIAN_POINT('Ctrl Pts',(2.73074730314363,-2.96176229113661,-1.27446135937998));
#62906=CARTESIAN_POINT('Ctrl Pts',(2.73696803201756,-2.92044606429033,-1.36646876259605));
#62907=CARTESIAN_POINT('Ctrl Pts',(2.74318876089149,-2.87497959467187,-1.45623140081525));
#62908=CARTESIAN_POINT('Ctrl Pts',(2.74942070735249,-2.82943113722022,-1.54615590434469));
#62909=CARTESIAN_POINT('Ctrl Pts',(2.75565265381348,-2.77971769847653,-1.63382719011838));
#62910=CARTESIAN_POINT('Ctrl Pts',(2.76188460027447,-2.72610544442492,-1.71885620933713));
#62911=CARTESIAN_POINT('Ctrl Pts',(2.76562953556167,-2.69388847605383,-1.76995231173488));
#62912=CARTESIAN_POINT('Ctrl Pts',(2.76937447084887,-2.66026441834211,-1.82009485367877));
#62913=CARTESIAN_POINT('Ctrl Pts',(2.77311940613607,-2.62529792475211,-1.86920527732838));
#62914=CARTESIAN_POINT('Ctrl Pts',(2.77929171094779,-2.56766706064283,-1.95014779861423));
#62915=CARTESIAN_POINT('Ctrl Pts',(2.78546401575951,-2.50618786891869,-2.02856497857034));
#62916=CARTESIAN_POINT('Ctrl Pts',(2.79163632057123,-2.44110933590487,-2.10406814829228));
#62917=CARTESIAN_POINT('Ctrl Pts',(2.7978002664343,-2.3761189366,-2.1794690665639));
#62918=CARTESIAN_POINT('Ctrl Pts',(2.80396421229737,-2.30753916564686,-2.25196349228689));
#62919=CARTESIAN_POINT('Ctrl Pts',(2.81012815816044,-2.23566172760433,-2.32119240956566));
#62920=CARTESIAN_POINT('Ctrl Pts',(2.81628557744201,-2.16386039567438,-2.39034802506969));
#62921=CARTESIAN_POINT('Ctrl Pts',(2.82244299672357,-2.08876864956578,-2.45624470655207));
#62922=CARTESIAN_POINT('Ctrl Pts',(2.82860041600513,-2.01071718314817,-2.5185579151357));
#62923=CARTESIAN_POINT('Ctrl Pts',(2.8347533381567,-1.93272272236467,-2.58082561267217));
#62924=CARTESIAN_POINT('Ctrl Pts',(2.84090626030827,-1.85177317745502,-2.63951477061048));
#62925=CARTESIAN_POINT('Ctrl Pts',(2.84705918245984,-1.7682339904531,-2.69433964405126));
#62926=CARTESIAN_POINT('Ctrl Pts',(2.85320977381804,-1.68472644899764,-2.74914374923776));
#62927=CARTESIAN_POINT('Ctrl Pts',(2.85936036517623,-1.59863157740502,-2.80008624049596));
#62928=CARTESIAN_POINT('Ctrl Pts',(2.86551095653443,-1.51034487473563,-2.84692394030115));
#62929=CARTESIAN_POINT('Ctrl Pts',(2.87166086311904,-1.4220680014303,-2.89375642545012));
#62930=CARTESIAN_POINT('Ctrl Pts',(2.87781076970365,-1.33160016592131,-2.93648482417372));
#62931=CARTESIAN_POINT('Ctrl Pts',(2.88396067628826,-1.23936171878009,-2.97491177894782));
#62932=CARTESIAN_POINT('Ctrl Pts',(2.89011154311597,-1.14710886957738,-3.01334473368594));
#62933=CARTESIAN_POINT('Ctrl Pts',(2.89626240994369,-1.05308526061636,-3.0474747433944));
#62934=CARTESIAN_POINT('Ctrl Pts',(2.90241327677141,-0.957730533264694,
-3.0771528704555));
#62935=CARTESIAN_POINT('Ctrl Pts',(2.9085707213467,-0.862273833403293,-3.10686273535682));
#62936=CARTESIAN_POINT('Ctrl Pts',(2.914728165922,-0.765483588118864,-3.13211108134687));
#62937=CARTESIAN_POINT('Ctrl Pts',(2.9208856104973,-0.667813777359608,-3.15279912478875));
#62938=CARTESIAN_POINT('Ctrl Pts',(2.9270464914016,-0.570089459312684,-3.17349871375453));
#62939=CARTESIAN_POINT('Ctrl Pts',(2.93320737230589,-0.471485026918437,
-3.1896328616928));
#62940=CARTESIAN_POINT('Ctrl Pts',(2.93936825321019,-0.372461729326465,
-3.20115445155137));
#62941=CARTESIAN_POINT('Ctrl Pts',(2.94553943361812,-0.273272888717306,
-3.21269530272313));
#62942=CARTESIAN_POINT('Ctrl Pts',(2.95171061402605,-0.173664217725312,
-3.21960816307786));
#62943=CARTESIAN_POINT('Ctrl Pts',(2.95788179443398,-0.0740992724655996,
-3.22189802140292));
#62944=CARTESIAN_POINT('Ctrl Pts',(2.96257673791456,0.0016482765836582,
-3.22364011200862));
#62945=CARTESIAN_POINT('Ctrl Pts',(2.96727168139514,0.0773704706349393,
-3.22270751540126));
#62946=CARTESIAN_POINT('Ctrl Pts',(2.97196662487572,0.152865534961373,-3.21912250321745));
#62947=CARTESIAN_POINT('Ctrl Pts',(2.97813888724918,0.252116004504065,-3.21440942500851));
#62948=CARTESIAN_POINT('Ctrl Pts',(2.98431114962264,0.3513229829132,-3.20509368556077));
#62949=CARTESIAN_POINT('Ctrl Pts',(2.9904834119961,0.450024894527647,-3.19117457322619));
#62950=CARTESIAN_POINT('Ctrl Pts',(2.99664731532029,0.548593134873285,-3.1772743114425));
#62951=CARTESIAN_POINT('Ctrl Pts',(3.00281121864447,0.646657241635713,-3.15878312828077));
#62952=CARTESIAN_POINT('Ctrl Pts',(3.00897512196866,0.743757484854407,-3.13575228074908));
#62953=CARTESIAN_POINT('Ctrl Pts',(3.01513249866829,0.840754913866283,-3.11274581933881));
#62954=CARTESIAN_POINT('Ctrl Pts',(3.02128987536792,0.936790088033487,-3.08520934963691));
#62955=CARTESIAN_POINT('Ctrl Pts',(3.02744725206756,1.03141119745655,-3.05324556894156));
#62956=CARTESIAN_POINT('Ctrl Pts',(3.03360013175136,1.12596320072481,-3.02130513286761));
#62957=CARTESIAN_POINT('Ctrl Pts',(3.03975301143516,1.21910278225954,-2.98494395308761));
#62958=CARTESIAN_POINT('Ctrl Pts',(3.04590589111896,1.31039197699404,-2.94431493375448));
#62959=CARTESIAN_POINT('Ctrl Pts',(3.05205644009313,1.4016465913993,-2.90370130468598));
#62960=CARTESIAN_POINT('Ctrl Pts',(3.0582069890673,1.49105181533694,-2.85882322477603));
#62961=CARTESIAN_POINT('Ctrl Pts',(3.06435753804148,1.57818923945029,-2.80988189911663));
#62962=CARTESIAN_POINT('Ctrl Pts',(3.07050740237668,1.66531696399429,-2.7609460212862));
#62963=CARTESIAN_POINT('Ctrl Pts',(3.07665726671188,1.75017701186951,-2.7079480096469));
#62964=CARTESIAN_POINT('Ctrl Pts',(3.08280713104708,1.8323760803352,-2.65113475001091));
#62965=CARTESIAN_POINT('Ctrl Pts',(3.08895795581103,1.91458798588874,-2.59431261780716));
#62966=CARTESIAN_POINT('Ctrl Pts',(3.09510878057498,1.9941377292465,-2.5336743011308));
#62967=CARTESIAN_POINT('Ctrl Pts',(3.10125960533894,2.07066230816602,-2.46950909454503));
#62968=CARTESIAN_POINT('Ctrl Pts',(3.10741700840269,2.14726873003199,-2.40527526334686));
#62969=CARTESIAN_POINT('Ctrl Pts',(3.11357441146643,2.22084319318331,-2.33750728957088));
#62970=CARTESIAN_POINT('Ctrl Pts',(3.11973181453018,2.29105713233226,-2.26653364830295));
#62971=CARTESIAN_POINT('Ctrl Pts',(3.12589265416439,2.36131025929246,-2.19552039521874));
#62972=CARTESIAN_POINT('Ctrl Pts',(3.13205349379859,2.42819883626417,-2.12129823426576));
#62973=CARTESIAN_POINT('Ctrl Pts',(3.1382143334328,2.49143382992998,-2.04422969198191));
#62974=CARTESIAN_POINT('Ctrl Pts',(3.14438547340107,2.55477454645137,-1.96703229847354));
#62975=CARTESIAN_POINT('Ctrl Pts',(3.15055661336933,2.6144492185164,-1.88697936634528));
#62976=CARTESIAN_POINT('Ctrl Pts',(3.1567277533376,2.67021139739144,-1.80446353682773));
#62977=CARTESIAN_POINT('Ctrl Pts',(3.16142311676352,2.71263851727304,-1.74168067823614));
#62978=CARTESIAN_POINT('Ctrl Pts',(3.16611848018944,2.75280155671635,-1.67747265830885));
#62979=CARTESIAN_POINT('Ctrl Pts',(3.17081384361537,2.79061012582739,-1.61202130511033));
#62980=CARTESIAN_POINT('Ctrl Pts',(3.1769860681354,2.84031085315475,-1.52598314140801));
#62981=CARTESIAN_POINT('Ctrl Pts',(3.18315829265544,2.88611633399345,-1.43749286806601));
#62982=CARTESIAN_POINT('Ctrl Pts',(3.18933051717548,2.92777638832986,-1.34693837366012));
#62983=CARTESIAN_POINT('Ctrl Pts',(3.19549438190015,2.96938001738102,-1.25650652823439));
#62984=CARTESIAN_POINT('Ctrl Pts',(3.20165824662482,3.00684919972532,-1.16401640990137));
#62985=CARTESIAN_POINT('Ctrl Pts',(3.20782211134949,3.0399784693731,-1.06988245534169));
#62986=CARTESIAN_POINT('Ctrl Pts',(3.21397944875849,3.07307265629101,-0.975848185324895));
#62987=CARTESIAN_POINT('Ctrl Pts',(3.22013678616748,3.10183592401484,-0.880173947369748));
#62988=CARTESIAN_POINT('Ctrl Pts',(3.22629412357647,3.12611036071096,-0.78329533073776));
#62989=CARTESIAN_POINT('Ctrl Pts',(3.23244696308815,3.15036706507955,-0.68648748334266));
#62990=CARTESIAN_POINT('Ctrl Pts',(3.23859980259983,3.17014135250086,-0.588477426529155));
#62991=CARTESIAN_POINT('Ctrl Pts',(3.24475264211151,3.18532503143249,-0.489716251138973));
#62992=CARTESIAN_POINT('Ctrl Pts',(3.25090315038462,3.20050295744665,-0.39099249519726));
#62993=CARTESIAN_POINT('Ctrl Pts',(3.25705365865773,3.21109366507162,-0.291518615015593));
#62994=CARTESIAN_POINT('Ctrl Pts',(3.26320416693084,3.21704016779057,-0.191755368430845));
#62995=CARTESIAN_POINT('Ctrl Pts',(3.26935399008264,3.22298600811291,-0.0920032347368021));
#62996=CARTESIAN_POINT('Ctrl Pts',(3.27550381323444,3.22428864621116,0.00803776766592394));
#62997=CARTESIAN_POINT('Ctrl Pts',(3.28165363638624,3.2209430979592,0.107903300269344));
#62998=CARTESIAN_POINT('Ctrl Pts',(3.28780441953062,3.21759702746432,0.207784421966731));
#62999=CARTESIAN_POINT('Ctrl Pts',(3.29395520267501,3.20960134396411,0.307489585282811));
#63000=CARTESIAN_POINT('Ctrl Pts',(3.3001059858194,3.19700312176381,0.406557009449417));
#63001=CARTESIAN_POINT('Ctrl Pts',(3.30626334683947,3.18439142655731,0.505730379994744));
#63002=CARTESIAN_POINT('Ctrl Pts',(3.31242070785954,3.16716741857891,0.604264217714333));
#63003=CARTESIAN_POINT('Ctrl Pts',(3.31857806887961,3.14542975161115,0.701704524838918));
#63004=CARTESIAN_POINT('Ctrl Pts',(3.32473886616897,3.12367995339477,0.799199210963468));
#63005=CARTESIAN_POINT('Ctrl Pts',(3.33089966345832,3.09741159392134,0.895598732033169));
#63006=CARTESIAN_POINT('Ctrl Pts',(3.33706046074768,3.06677334679193,0.990463932663182));
#63007=CARTESIAN_POINT('Ctrl Pts',(3.34323155831427,3.03608387537701,1.08548773904182));
#63008=CARTESIAN_POINT('Ctrl Pts',(3.34940265588086,3.00101007536719,1.178971694106));
#63009=CARTESIAN_POINT('Ctrl Pts',(3.35557375344745,2.96174897914172,1.27049618143975));
#63010=CARTESIAN_POINT('Ctrl Pts',(3.3602695230833,2.93187405632025,1.34013985566801));
#63011=CARTESIAN_POINT('Ctrl Pts',(3.36496529271915,2.8995756340568,1.40864937726985));
#63012=CARTESIAN_POINT('Ctrl Pts',(3.369661062355,2.86495782129977,1.47585034629982));
#63013=CARTESIAN_POINT('Ctrl Pts',(3.37583326514642,2.8194555549831,1.56418049040802));
#63014=CARTESIAN_POINT('Ctrl Pts',(3.38200546793785,2.76978438610278,1.65055979252062));
#63015=CARTESIAN_POINT('Ctrl Pts',(3.38817767072928,2.71613533611053,1.73456807258515));
#63016=CARTESIAN_POINT('Ctrl Pts',(3.3943418226725,2.66255626443436,1.81846677460538));
#63017=CARTESIAN_POINT('Ctrl Pts',(3.40050597461572,2.60500985405945,1.90000023739665));
#63018=CARTESIAN_POINT('Ctrl Pts',(3.40667012655894,2.54373367116966,1.97877148065605));
#63019=CARTESIAN_POINT('Ctrl Pts',(3.41282693327524,2.48253050521263,2.05744885980216));
#63020=CARTESIAN_POINT('Ctrl Pts',(3.41898373999155,2.41760667358952,2.13337022645203));
#63021=CARTESIAN_POINT('Ctrl Pts',(3.42514054670785,2.34924314121892,2.20616731594316));
#63022=CARTESIAN_POINT('Ctrl Pts',(3.43129310438258,2.28092678906758,2.27891416545218));
#63023=CARTESIAN_POINT('Ctrl Pts',(3.43744566205732,2.20917575047399,2.34854070754722));
#63024=CARTESIAN_POINT('Ctrl Pts',(3.44359821973205,2.1343109395226,2.41471206895028));
#63025=CARTESIAN_POINT('Ctrl Pts',(3.44974841764773,2.05947484230707,2.48085805091315));
#63026=CARTESIAN_POINT('Ctrl Pts',(3.4558986155634,1.98152767094381,2.54355119831489));
#63027=CARTESIAN_POINT('Ctrl Pts',(3.46204881347908,1.90082614629056,2.60249448108506));
#63028=CARTESIAN_POINT('Ctrl Pts',(3.46483627454,1.86424970426183,2.62920941087715));
#63029=CARTESIAN_POINT('Ctrl Pts',(3.46762373560092,1.82710793091848,2.65515458680447));
#63030=CARTESIAN_POINT('Ctrl Pts',(3.47041119666184,1.78943621037803,2.68030513402633));
#63031=CARTESIAN_POINT('Origin',(-1.72497344927317,0.,0.));
#63032=CARTESIAN_POINT('',(4.96704894786217,1.78943621037804,2.68030513402633));
#63033=CARTESIAN_POINT('',(4.7207101123806,1.78943616882057,2.68030516177109));
#63034=CARTESIAN_POINT('',(-1.72497344927317,1.78943621037804,2.68030513402633));
#63035=CARTESIAN_POINT('',(4.14657344921911,-3.22274994184251,-0.000612253281709201));
#63036=CARTESIAN_POINT('Ctrl Pts',(4.1465734492731,-3.22274994184235,-0.000612254151029935));
#63037=CARTESIAN_POINT('Ctrl Pts',(4.14860941488238,-3.22274371421397,-0.0333929040906794));
#63038=CARTESIAN_POINT('Ctrl Pts',(4.15064538049165,-3.22223735157171,-0.066168248405641));
#63039=CARTESIAN_POINT('Ctrl Pts',(4.15268134610092,-3.22123125223858,-0.0989281663706331));
#63040=CARTESIAN_POINT('Ctrl Pts',(4.15885359442719,-3.21818115409513,-0.198243374794371));
#63041=CARTESIAN_POINT('Ctrl Pts',(4.16502584275346,-3.21052833720515,-0.297592198081419));
#63042=CARTESIAN_POINT('Ctrl Pts',(4.17119809107972,-3.19826435630236,-0.396513139386145));
#63043=CARTESIAN_POINT('Ctrl Pts',(4.17736197996862,-3.18601698522712,-0.49530010626698));
#63044=CARTESIAN_POINT('Ctrl Pts',(4.18352586885752,-3.16917091607389,-0.593659915717286));
#63045=CARTESIAN_POINT('Ctrl Pts',(4.18968975774641,-3.14776969585369,-0.691132045534844));
#63046=CARTESIAN_POINT('Ctrl Pts',(4.19584711964366,-3.12639113755816,-0.788500961328129));
#63047=CARTESIAN_POINT('Ctrl Pts',(4.20200448154091,-3.10046711038163,-0.884983644310407));
#63048=CARTESIAN_POINT('Ctrl Pts',(4.20816184343815,-3.07009272710254,-0.980126629314843));
#63049=CARTESIAN_POINT('Ctrl Pts',(4.21431470782583,-3.03974053012367,-1.07520011921845));
#63050=CARTESIAN_POINT('Ctrl Pts',(4.2204675722135,-3.00494457162692,-1.16893544412282));
#63051=CARTESIAN_POINT('Ctrl Pts',(4.22662043660117,-2.96585039615279,-1.2608921405657));
#63052=CARTESIAN_POINT('Ctrl Pts',(4.23277096998064,-2.92677103147865,-1.3528139992809));
#63053=CARTESIAN_POINT('Ctrl Pts',(4.23892150336011,-2.88339685516167,-1.44295816912987));
#63054=CARTESIAN_POINT('Ctrl Pts',(4.24507203673957,-2.83592203354208,-1.53090293035533));
#63055=CARTESIAN_POINT('Ctrl Pts',(4.251221885199,-2.78845249869272,-1.61883789810019));
#63056=CARTESIAN_POINT('Ctrl Pts',(4.25737173365843,-2.73688343276047,-1.70457356193074));
#63057=CARTESIAN_POINT('Ctrl Pts',(4.26352158211785,-2.68145509702484,-1.78771253985072));
#63058=CARTESIAN_POINT('Ctrl Pts',(4.26967239074222,-2.62601810736143,-1.87086449811191));
#63059=CARTESIAN_POINT('Ctrl Pts',(4.27582319936658,-2.56672089207044,-1.95141860375034));
#63060=CARTESIAN_POINT('Ctrl Pts',(4.28197400799094,-2.50384662286267,-2.02900706052966));
#63061=CARTESIAN_POINT('Ctrl Pts',(4.28813139460239,-2.44090511271866,-2.10667849434459));
#63062=CARTESIAN_POINT('Ctrl Pts',(4.29428878121383,-2.37437918357418,-2.18137760777539));
#63063=CARTESIAN_POINT('Ctrl Pts',(4.30044616782528,-2.30459175906569,-2.25277038034206));
#63064=CARTESIAN_POINT('Ctrl Pts',(4.3066069908079,-2.2347653869469,-2.32420299644649));
#63065=CARTESIAN_POINT('Ctrl Pts',(4.31276781379052,-2.16167421232127,-2.39232530076201));
#63066=CARTESIAN_POINT('Ctrl Pts',(4.31892863677314,-2.08567586774788,-2.45684222879576));
#63067=CARTESIAN_POINT('Ctrl Pts',(4.32509975993361,-2.00955046280174,-2.52146702161224));
#63068=CARTESIAN_POINT('Ctrl Pts',(4.33127088309407,-1.93050852333384,-2.58247413233613));
#63069=CARTESIAN_POINT('Ctrl Pts',(4.33744200625453,-1.84893850573749,-2.63961057061477));
#63070=CARTESIAN_POINT('Ctrl Pts',(4.34213752578321,-1.78687304364591,-2.68308487095854));
#63071=CARTESIAN_POINT('Ctrl Pts',(4.34683304531188,-1.72334459615962,-2.72431912931856));
#63072=CARTESIAN_POINT('Ctrl Pts',(4.35152856484056,-1.65853347065144,-2.76321991329479));
#63073=CARTESIAN_POINT('Ctrl Pts',(4.35770081291735,-1.57333941654742,-2.81435489156858));
#63074=CARTESIAN_POINT('Ctrl Pts',(4.36387306099414,-1.48562834827015,-2.86163619811208));
#63075=CARTESIAN_POINT('Ctrl Pts',(4.37004530907093,-1.3957839145922,-2.90480719261463));
#63076=CARTESIAN_POINT('Ctrl Pts',(4.37620919770796,-1.30606116253211,-2.94791971809199));
#63077=CARTESIAN_POINT('Ctrl Pts',(4.38237308634498,-1.21421117603225,-2.98693280975896));
#63078=CARTESIAN_POINT('Ctrl Pts',(4.38853697498201,-1.1206448967466,-3.02163409066945));
#63079=CARTESIAN_POINT('Ctrl Pts',(4.39469433662532,-1.02717769558391,-3.05629862610066));
#63080=CARTESIAN_POINT('Ctrl Pts',(4.40085169826864,-0.931998219814458,
-3.08666027783024));
#63081=CARTESIAN_POINT('Ctrl Pts',(4.40700905991195,-0.835539356792753,
-3.11255386230509));
#63082=CARTESIAN_POINT('Ctrl Pts',(4.41316192404367,-0.739150950060656,
-3.13842853337137));
#63083=CARTESIAN_POINT('Ctrl Pts',(4.41931478817538,-0.64148543228148,-3.15984151350616));
#63084=CARTESIAN_POINT('Ctrl Pts',(4.4254676523071,-0.542992022632832,-3.17667707295802));
#63085=CARTESIAN_POINT('Ctrl Pts',(4.43161818542945,-0.444535927161101,
-3.19350625426694));
#63086=CARTESIAN_POINT('Ctrl Pts',(4.4377687185518,-0.345252990723664,-3.20576138754103));
#63087=CARTESIAN_POINT('Ctrl Pts',(4.44391925167414,-0.245602955433838,
-3.21337777903286));
#63088=CARTESIAN_POINT('Ctrl Pts',(4.45006909987557,-0.145964017132235,
-3.22099332236637));
#63089=CARTESIAN_POINT('Ctrl Pts',(4.456218948077,-0.0459584943661108,-3.22397111782779));
#63090=CARTESIAN_POINT('Ctrl Pts',(4.46236879627843,0.0539494198851558,
-3.2222984068199));
#63091=CARTESIAN_POINT('Ctrl Pts',(4.46851960464423,0.15387293257334,-3.22062543465475));
#63092=CARTESIAN_POINT('Ctrl Pts',(4.47467041301002,0.253698372121929,-3.21430052112014));
#63093=CARTESIAN_POINT('Ctrl Pts',(4.48082122137582,0.352963231245526,-3.20336300157955));
#63094=CARTESIAN_POINT('Ctrl Pts',(4.48697860772943,0.452334249266459,-3.19241378489835));
#63095=CARTESIAN_POINT('Ctrl Pts',(4.49313599408304,0.55114305709235,-3.17684215927443));
#63096=CARTESIAN_POINT('Ctrl Pts',(4.49929338043665,0.648934065630894,-3.15673916264296));
#63097=CARTESIAN_POINT('Ctrl Pts',(4.50545420316144,0.746779650280764,-3.13662494674502));
#63098=CARTESIAN_POINT('Ctrl Pts',(4.51161502588623,0.84360588347207,-3.11197443072196));
#63099=CARTESIAN_POINT('Ctrl Pts',(4.51777584861102,0.938971178766004,-3.08292891386532));
#63100=CARTESIAN_POINT('Ctrl Pts',(4.52394697151633,1.03449591376486,-3.05383483627573));
#63101=CARTESIAN_POINT('Ctrl Pts',(4.53011809442164,1.12855442262882,-3.02033122640812));
#63102=CARTESIAN_POINT('Ctrl Pts',(4.53628921732695,1.2207238452979,-2.98260806275667));
#63103=CARTESIAN_POINT('Ctrl Pts',(4.54098473941138,1.29085428448887,-2.95390502916985));
#63104=CARTESIAN_POINT('Ctrl Pts',(4.5456802614958,1.35989143043535,-2.9227601029014));
#63105=CARTESIAN_POINT('Ctrl Pts',(4.55037578358022,1.42765919263351,-2.88927444044159));
#63106=CARTESIAN_POINT('Ctrl Pts',(4.55654803161821,1.51673968884811,-2.84525764940055));
#63107=CARTESIAN_POINT('Ctrl Pts',(4.56272027965621,1.60393941745078,-2.7970398038875));
#63108=CARTESIAN_POINT('Ctrl Pts',(4.5688925276942,1.68883504750651,-2.74480486461491));
#63109=CARTESIAN_POINT('Ctrl Pts',(4.57505641629111,1.77361569838222,-2.69264067021437));
#63110=CARTESIAN_POINT('Ctrl Pts',(4.58122030488801,1.85609808650302,-2.63647042144559));
#63111=CARTESIAN_POINT('Ctrl Pts',(4.58738419348492,1.9358813581292,-2.57652497169111));
#63112=CARTESIAN_POINT('Ctrl Pts',(4.59354155508686,2.01558014655881,-2.51664299869198));
#63113=CARTESIAN_POINT('Ctrl Pts',(4.5996989166888,2.09258515534237,-2.45299403178666));
#63114=CARTESIAN_POINT('Ctrl Pts',(4.60585627829074,2.16652336397703,-2.38585290322804));
#63115=CARTESIAN_POINT('Ctrl Pts',(4.61200914237935,2.24040756602563,-2.31876081647343));
#63116=CARTESIAN_POINT('Ctrl Pts',(4.61816200646796,2.31122910097951,-2.24818193057484));
#63117=CARTESIAN_POINT('Ctrl Pts',(4.62431487055656,2.37864771852987,-2.17443155643784));
#63118=CARTESIAN_POINT('Ctrl Pts',(4.63046540363475,2.44604079456037,-2.10070912260447));
#63119=CARTESIAN_POINT('Ctrl Pts',(4.63661593671293,2.5100332220557,-2.02381790818875));
#63120=CARTESIAN_POINT('Ctrl Pts',(4.64276646979111,2.5703219927888,-1.94410967177425));
#63121=CARTESIAN_POINT('Ctrl Pts',(4.64891631794738,2.63060404977859,-1.8644103116502));
#63122=CARTESIAN_POINT('Ctrl Pts',(4.65506616610365,2.68718300795863,-1.78189489965333));
#63123=CARTESIAN_POINT('Ctrl Pts',(4.66121601425992,2.73979714078375,-1.69694702034364));
#63124=CARTESIAN_POINT('Ctrl Pts',(4.6673668225796,2.79241948814749,-1.61198587829261));
#63125=CARTESIAN_POINT('Ctrl Pts',(4.67351763089927,2.84107555187938,-1.52459188391078));
#63126=CARTESIAN_POINT('Ctrl Pts',(4.67966843921895,2.88554833880993,-1.43517537147599));
#63127=CARTESIAN_POINT('Ctrl Pts',(4.68582582552524,2.93006868719609,-1.34566323248436));
#63128=CARTESIAN_POINT('Ctrl Pts',(4.69198321183152,2.97039663123149,-1.25412464586935));
#63129=CARTESIAN_POINT('Ctrl Pts',(4.69814059813781,3.00636241114835,-1.16099208237363));
#63130=CARTESIAN_POINT('Ctrl Pts',(4.70430142081453,3.04234826317642,-1.06780754260558));
#63131=CARTESIAN_POINT('Ctrl Pts',(4.71046224349125,3.07396696539453,-0.973027666433112));
#63132=CARTESIAN_POINT('Ctrl Pts',(4.71662306616797,3.10109860971386,-0.877100322272653));
#63133=CARTESIAN_POINT('Ctrl Pts',(4.72279418902449,3.12827561499052,-0.781012598736921));
#63134=CARTESIAN_POINT('Ctrl Pts',(4.728965311881,3.15095047898476,-0.683773998425126));
#63135=CARTESIAN_POINT('Ctrl Pts',(4.73513643473751,3.16905436853162,-0.585842958300801));
#63136=CARTESIAN_POINT('Ctrl Pts',(4.73983195726496,3.18282936915601,-0.511328576440075));
#63137=CARTESIAN_POINT('Ctrl Pts',(4.7445274797924,3.19395907252953,-0.436413526130888));
#63138=CARTESIAN_POINT('Ctrl Pts',(4.74922300231984,3.20243335845127,-0.361300632684886));
#63139=CARTESIAN_POINT('Ctrl Pts',(4.75539525044793,3.21357277799652,-0.262564993944416));
#63140=CARTESIAN_POINT('Ctrl Pts',(4.76156749857602,3.22016128260903,-0.163139920551488));
#63141=CARTESIAN_POINT('Ctrl Pts',(4.76773974670411,3.22212472232074,-0.0634809917178259));
#63142=CARTESIAN_POINT('Ctrl Pts',(4.77390363539251,3.22408550283025,0.0360429631504318));
#63143=CARTESIAN_POINT('Ctrl Pts',(4.7800675240809,3.22143366034395,0.135799713468046));
#63144=CARTESIAN_POINT('Ctrl Pts',(4.7862314127693,3.21414664507579,0.235327232695285));
#63145=CARTESIAN_POINT('Ctrl Pts',(4.792388774464,3.20686734608953,0.33474936139342));
#63146=CARTESIAN_POINT('Ctrl Pts',(4.79854613615871,3.19496266387674,0.433942310753885));
#63147=CARTESIAN_POINT('Ctrl Pts',(4.80470349785342,3.17846209378533,0.532443687980034));
#63148=CARTESIAN_POINT('Ctrl Pts',(4.81085636203633,3.16197357617878,0.630873117003702));
#63149=CARTESIAN_POINT('Ctrl Pts',(4.81700922621924,3.14089591646675,0.728611551091125));
#63150=CARTESIAN_POINT('Ctrl Pts',(4.82316209040215,3.11531038017994,0.825202276804377));
#63151=CARTESIAN_POINT('Ctrl Pts',(4.82931262357554,3.08973453696072,0.921756409169636));
#63152=CARTESIAN_POINT('Ctrl Pts',(4.83546315674894,3.05965432167019,1.01716327769536));
#63153=CARTESIAN_POINT('Ctrl Pts',(4.84161368992234,3.02520179712534,1.11097778968331));
#63154=CARTESIAN_POINT('Ctrl Pts',(4.84776353817463,2.99075310920095,1.2047818545217));
#63155=CARTESIAN_POINT('Ctrl Pts',(4.85391338642692,2.95193322979036,1.29699350761948));
#63156=CARTESIAN_POINT('Ctrl Pts',(4.8600632346792,2.90892331543334,1.38718517416685));
#63157=CARTESIAN_POINT('Ctrl Pts',(4.86621404309559,2.86590668602025,1.47739092216747));
#63158=CARTESIAN_POINT('Ctrl Pts',(4.87236485151199,2.81869890927398,1.56557566508484));
#63159=CARTESIAN_POINT('Ctrl Pts',(4.87851565992838,2.76752783162929,1.65133499437797));
#63160=CARTESIAN_POINT('Ctrl Pts',(4.88467304633186,2.71630202903372,1.73718603905602));
#63161=CARTESIAN_POINT('Ctrl Pts',(4.89083043273534,2.66110468458998,1.82060611669234));
#63162=CARTESIAN_POINT('Ctrl Pts',(4.89698781913883,2.60220780570796,1.90121858249191));
#63163=CARTESIAN_POINT('Ctrl Pts',(4.90314864191316,2.54327805711392,1.98187603723803));
#63164=CARTESIAN_POINT('Ctrl Pts',(4.9093094646875,2.48064493462321,2.05972242124727));
#63165=CARTESIAN_POINT('Ctrl Pts',(4.91547028746184,2.41462035361907,2.1344146997218));
#63166=CARTESIAN_POINT('Ctrl Pts',(4.92164141041565,2.34848538719095,2.20923185500286));
#63167=CARTESIAN_POINT('Ctrl Pts',(4.92781253336947,2.27894793900684,2.28088405963915));
#63168=CARTESIAN_POINT('Ctrl Pts',(4.93398365632328,2.20635643154003,2.34906552899274));
#63169=CARTESIAN_POINT('Ctrl Pts',(4.93867917790202,2.15112256368568,2.40094386021644));
#63170=CARTESIAN_POINT('Ctrl Pts',(4.94337469948076,2.09412131139111,2.45081359014625));
#63171=CARTESIAN_POINT('Ctrl Pts',(4.9480702210595,2.0355178209157,2.49855653592922));
#63172=CARTESIAN_POINT('Ctrl Pts',(4.95439646332706,1.95656176198702,2.56288026153138));
#63173=CARTESIAN_POINT('Ctrl Pts',(4.96072270559462,1.87441123637086,2.62357376170643));
#63174=CARTESIAN_POINT('Ctrl Pts',(4.96704894786217,1.78943621037804,2.68030513402633));
#63175=CARTESIAN_POINT('Ctrl Pts',(3.71684364332268,1.78943621037804,2.68030513402633));
#63176=CARTESIAN_POINT('Ctrl Pts',(3.72320085420584,1.70382486360772,2.73746132941066));
#63177=CARTESIAN_POINT('Ctrl Pts',(3.729558065089,1.61556784701393,2.79044800209424));
#63178=CARTESIAN_POINT('Ctrl Pts',(3.73591527597216,1.52511857513192,2.83903696599526));
#63179=CARTESIAN_POINT('Ctrl Pts',(3.74227248685532,1.43466930324992,2.88762592989628));
#63180=CARTESIAN_POINT('Ctrl Pts',(3.74862969773848,1.34202825831221,2.93181703204401));
#63181=CARTESIAN_POINT('Ctrl Pts',(3.75498690862164,1.24766919048137,2.97143722020566));
#63182=CARTESIAN_POINT('Ctrl Pts',(3.76115915673829,1.15605549551158,3.00990466076362));
#63183=CARTESIAN_POINT('Ctrl Pts',(3.76733140485495,1.06249987373899,3.04419896492224));
#63184=CARTESIAN_POINT('Ctrl Pts',(3.77350365297161,0.967418642046842,3.07412080659174));
#63185=CARTESIAN_POINT('Ctrl Pts',(3.77966754165257,0.872466184413464,3.10400212336554));
#63186=CARTESIAN_POINT('Ctrl Pts',(3.78583143033354,0.775992634399417,3.12952261879608));
#63187=CARTESIAN_POINT('Ctrl Pts',(3.79199531901451,0.67843501282167,3.15053066893145));
#63188=CARTESIAN_POINT('Ctrl Pts',(3.79815268070577,0.580980695768812,3.17151647347901));
#63189=CARTESIAN_POINT('Ctrl Pts',(3.80431004239703,0.482445011648844,3.18799924143239));
#63190=CARTESIAN_POINT('Ctrl Pts',(3.81046740408829,0.383279974942234,3.19987718878526));
#63191=CARTESIAN_POINT('Ctrl Pts',(3.81662026827382,0.284187371096189,3.21174646015986));
#63192=CARTESIAN_POINT('Ctrl Pts',(3.82277313245936,0.184466758610693,3.21901754661746));
#63193=CARTESIAN_POINT('Ctrl Pts',(3.82892599664489,0.0845792668482427,
3.22163994110444));
#63194=CARTESIAN_POINT('Ctrl Pts',(3.83507652982463,-0.0152703826485386,
3.22426134210017));
#63195=CARTESIAN_POINT('Ctrl Pts',(3.84122706300438,-0.115286352056842,
3.22223753913711));
#63196=CARTESIAN_POINT('Ctrl Pts',(3.84737759618413,-0.215004372247607,
3.2155700400418));
#63197=CARTESIAN_POINT('Ctrl Pts',(3.85352744444649,-0.314711287936841,
3.20890328343269));
#63198=CARTESIAN_POINT('Ctrl Pts',(3.85967729270886,-0.41411988696594,3.19759388777563));
#63199=CARTESIAN_POINT('Ctrl Pts',(3.86582714097123,-0.512768898671985,
3.18169540010585));
#63200=CARTESIAN_POINT('Ctrl Pts',(3.87197794940145,-0.611433312320612,
3.16579443022575));
#63201=CARTESIAN_POINT('Ctrl Pts',(3.87812875783167,-0.709337474206959,
3.14530301432027));
#63202=CARTESIAN_POINT('Ctrl Pts',(3.88427956626189,-0.80602920865643,3.12032602099407));
#63203=CARTESIAN_POINT('Ctrl Pts',(3.89043695268496,-0.902824350250759,
3.09532231597859));
#63204=CARTESIAN_POINT('Ctrl Pts',(3.89659433910804,-0.998404053776648,
3.06582356306365));
#63205=CARTESIAN_POINT('Ctrl Pts',(3.90275172553111,-1.09233036180624,3.03198481908737));
#63206=CARTESIAN_POINT('Ctrl Pts',(3.90891254832827,-1.18630908914307,2.99812719005583));
#63207=CARTESIAN_POINT('Ctrl Pts',(3.91507337112543,-1.27863218196992,2.95992491246381));
#63208=CARTESIAN_POINT('Ctrl Pts',(3.92123419392259,-1.36888270774741,2.91758079492756));
#63209=CARTESIAN_POINT('Ctrl Pts',(3.92740531690434,-1.45928412198666,2.87516588291444));
#63210=CARTESIAN_POINT('Ctrl Pts',(3.93357643988609,-1.54760566334814,2.82859550181945));
#63211=CARTESIAN_POINT('Ctrl Pts',(3.93974756286785,-1.63345587410689,2.77811797262926));
#63212=CARTESIAN_POINT('Ctrl Pts',(3.94444308436566,-1.6987781033675,2.73971032394524));
#63213=CARTESIAN_POINT('Ctrl Pts',(3.94913860586347,-1.76267009048399,2.69904158402108));
#63214=CARTESIAN_POINT('Ctrl Pts',(3.95383412736128,-1.82497196443557,2.65623697954911));
#63215=CARTESIAN_POINT('Ctrl Pts',(3.9599753003298,-1.90645526386844,2.60025374530473));
#63216=CARTESIAN_POINT('Ctrl Pts',(3.96611647329832,-1.98551067995544,2.54041410671207));
#63217=CARTESIAN_POINT('Ctrl Pts',(3.97225764626685,-2.06174767113923,2.47695662114862));
#63218=CARTESIAN_POINT('Ctrl Pts',(3.97839048445549,-2.1378811937278,2.41358525987713));
#63219=CARTESIAN_POINT('Ctrl Pts',(3.98452332264413,-2.21120355799046,2.3466060871575));
#63220=CARTESIAN_POINT('Ctrl Pts',(3.99065616083278,-2.28135294761985,2.27630101060607));
#63221=CARTESIAN_POINT('Ctrl Pts',(3.99678253559132,-2.35142840644222,2.20607002894093));
#63222=CARTESIAN_POINT('Ctrl Pts',(4.00290891034986,-2.41833722883924,2.13252041972971));
#63223=CARTESIAN_POINT('Ctrl Pts',(4.0090352851084,-2.48175127719434,2.05597377430848));
#63224=CARTESIAN_POINT('Ctrl Pts',(4.01515727946341,-2.54511998403313,1.97948186030816));
#63225=CARTESIAN_POINT('Ctrl Pts',(4.02127927381843,-2.60499860428731,1.89999750682691));
#63226=CARTESIAN_POINT('Ctrl Pts',(4.02740126817344,-2.66109712391762,1.81787779005558));
#63227=CARTESIAN_POINT('Ctrl Pts',(4.03352105751895,-2.71717543807858,1.73578765102412));
#63228=CARTESIAN_POINT('Ctrl Pts',(4.03964084686445,-2.76947610886918,1.65106439674511));
#63229=CARTESIAN_POINT('Ctrl Pts',(4.04576063620995,-2.81775115050717,1.56409591020357));
#63230=CARTESIAN_POINT('Ctrl Pts',(4.05187990105706,-2.86602205471813,1.47713487732244));
#63231=CARTESIAN_POINT('Ctrl Pts',(4.05799916590417,-2.91026780271043,1.38792937895106));
#63232=CARTESIAN_POINT('Ctrl Pts',(4.06411843075128,-2.95028581219471,1.2968928979922));
#63233=CARTESIAN_POINT('Ctrl Pts',(4.07023885074343,-2.99031137595325,1.2058392319071));
#63234=CARTESIAN_POINT('Ctrl Pts',(4.07635927073557,-3.0261074398551,1.11295429910164));
#63235=CARTESIAN_POINT('Ctrl Pts',(4.08247969072771,-3.05751953874999,1.01867160197094));
#63236=CARTESIAN_POINT('Ctrl Pts',(4.08860663556407,-3.08896512538787,0.924288392144779));
#63237=CARTESIAN_POINT('Ctrl Pts',(4.09473358040043,-3.1160172793467,0.828504861050562));
#63238=CARTESIAN_POINT('Ctrl Pts',(4.10086052523678,-3.13857149017669,0.731769474322391));
#63239=CARTESIAN_POINT('Ctrl Pts',(4.10699115011104,-3.16113924778292,0.634975985244822));
#63240=CARTESIAN_POINT('Ctrl Pts',(4.1131217749853,-3.17920360524386,0.537229934087183));
#63241=CARTESIAN_POINT('Ctrl Pts',(4.11925239985956,-3.19271160062645,0.438987696553426));
#63242=CARTESIAN_POINT('Ctrl Pts',(4.12539264638702,-3.20624079600899,0.340591273637435));
#63243=CARTESIAN_POINT('Ctrl Pts',(4.13153289291448,-3.21519931595962,0.241697546589613));
#63244=CARTESIAN_POINT('Ctrl Pts',(4.13767313944194,-3.21958624004559,0.1427655610052));
#63245=CARTESIAN_POINT('Ctrl Pts',(4.14063990936766,-3.22170586087619,0.0949648028090939));
#63246=CARTESIAN_POINT('Ctrl Pts',(4.14360667929339,-3.22275901660992,0.0471550793021853));
#63247=CARTESIAN_POINT('Ctrl Pts',(4.14657344921911,-3.22274994184251,-0.000612253281710953));
#63248=CARTESIAN_POINT('',(3.90002655072689,-3.222749015224,-0.00251939927735915));
#63249=CARTESIAN_POINT('Ctrl Pts',(3.47041119666184,1.78943621037803,2.68030513402633));
#63250=CARTESIAN_POINT('Ctrl Pts',(3.47656128588147,1.70631955428236,2.73579581388027));
#63251=CARTESIAN_POINT('Ctrl Pts',(3.4827113751011,1.62062143679504,2.78741528527276));
#63252=CARTESIAN_POINT('Ctrl Pts',(3.48886146432073,1.5327422123689,2.8349283717446));
#63253=CARTESIAN_POINT('Ctrl Pts',(3.4950132591234,1.4448386167004,2.88245463485692));
#63254=CARTESIAN_POINT('Ctrl Pts',(3.50116505392607,1.35475309436674,2.92587204395454));
#63255=CARTESIAN_POINT('Ctrl Pts',(3.50731684872874,1.26290954461645,2.96499191307779));
#63256=CARTESIAN_POINT('Ctrl Pts',(3.51347561751752,1.17096187636731,3.00415613046566));
#63257=CARTESIAN_POINT('Ctrl Pts',(3.5196343863063,1.07725260334655,3.03901291458188));
#63258=CARTESIAN_POINT('Ctrl Pts',(3.52579315509507,0.982224312330869,3.06942225227585));
#63259=CARTESIAN_POINT('Ctrl Pts',(3.5319560303526,0.88713265951016,3.09985186593717));
#63260=CARTESIAN_POINT('Ctrl Pts',(3.53811890561013,0.790720656657336,3.12582801726841));
#63261=CARTESIAN_POINT('Ctrl Pts',(3.54428178086766,0.693442729433876,3.1472614672911));
#63262=CARTESIAN_POINT('Ctrl Pts',(3.55045414406345,0.596015039813806,3.16872791477718));
#63263=CARTESIAN_POINT('Ctrl Pts',(3.55662650725925,0.49771919223111,3.18563763084689));
#63264=CARTESIAN_POINT('Ctrl Pts',(3.56279887045505,0.39901621521905,3.19795303631749));
#63265=CARTESIAN_POINT('Ctrl Pts',(3.56470200733491,0.368582932253415,3.20175026950001));
#63266=CARTESIAN_POINT('Ctrl Pts',(3.56660514421478,0.338110950773104,3.20511110214546));
#63267=CARTESIAN_POINT('Ctrl Pts',(3.56850828109465,0.307613771781163,3.20803543152356));
#63268=CARTESIAN_POINT('Ctrl Pts',(3.57468053030192,0.208705390125472,3.21751960992225));
#63269=CARTESIAN_POINT('Ctrl Pts',(3.58085277950919,0.109183892706614,3.22244196246382));
#63270=CARTESIAN_POINT('Ctrl Pts',(3.58702502871646,0.00950603695194093,
3.22273598015126));
#63271=CARTESIAN_POINT('Ctrl Pts',(3.59318891852752,-0.0900368199293453,
3.22302959963533));
#63272=CARTESIAN_POINT('Ctrl Pts',(3.59935280833858,-0.189735183693171,
3.21870734211687));
#63273=CARTESIAN_POINT('Ctrl Pts',(3.60551669814965,-0.289126714756948,
3.20975439953182));
#63274=CARTESIAN_POINT('Ctrl Pts',(3.61167406100881,-0.388412999983746,
3.2008109372307));
#63275=CARTESIAN_POINT('Ctrl Pts',(3.61783142386798,-0.487392668215522,
3.18724657711801));
#63276=CARTESIAN_POINT('Ctrl Pts',(3.62398878672715,-0.585603885382707,
3.16909855509807));
#63277=CARTESIAN_POINT('Ctrl Pts',(3.63014165213293,-0.683743367233776,
3.150963788734));
#63278=CARTESIAN_POINT('Ctrl Pts',(3.63629451753871,-0.781115088106869,
3.12825209553679));
#63279=CARTESIAN_POINT('Ctrl Pts',(3.64244738294449,-0.877263759601254,
3.10105237920779));
#63280=CARTESIAN_POINT('Ctrl Pts',(3.64859791737628,-0.973376005781941,
3.07386296731861));
#63281=CARTESIAN_POINT('Ctrl Pts',(3.65474845180807,-1.06826570573873,3.04218902881309));
#63282=CARTESIAN_POINT('Ctrl Pts',(3.66089898623986,-1.16149004099436,3.00617006291575));
#63283=CARTESIAN_POINT('Ctrl Pts',(3.66704883578467,-1.25470399534181,2.9701551078765));
#63284=CARTESIAN_POINT('Ctrl Pts',(3.67319868532948,-1.34625254849613,2.92979624393343));
#63285=CARTESIAN_POINT('Ctrl Pts',(3.67934853487429,-1.4357112196894,2.88528176373781));
#63286=CARTESIAN_POINT('Ctrl Pts',(3.68549934461603,-1.52518385836927,2.840760333345));
#63287=CARTESIAN_POINT('Ctrl Pts',(3.69165015435776,-1.61256557804487,2.79208219148369));
#63288=CARTESIAN_POINT('Ctrl Pts',(3.6978009640995,-1.69745584298123,2.73948192613656));
#63289=CARTESIAN_POINT('Ctrl Pts',(3.70395835187143,-1.78243689445615,2.68682540703617));
#63290=CARTESIAN_POINT('Ctrl Pts',(3.71011573964336,-1.86492080049206,2.63023861761331));
#63291=CARTESIAN_POINT('Ctrl Pts',(3.71627312741529,-1.9445355248577,2.56999983561603));
#63292=CARTESIAN_POINT('Ctrl Pts',(3.72243395158413,-2.02419468166819,2.50972743475765));
#63293=CARTESIAN_POINT('Ctrl Pts',(3.72859477575297,-2.10098113406282,2.4457992603061));
#63294=CARTESIAN_POINT('Ctrl Pts',(3.73475559992181,-2.17455711951252,2.37853292944988));
#63295=CARTESIAN_POINT('Ctrl Pts',(3.74092672429874,-2.2482561157705,2.31115413682127));
#63296=CARTESIAN_POINT('Ctrl Pts',(3.74709784867567,-2.3187336168382,2.240426347702));
#63297=CARTESIAN_POINT('Ctrl Pts',(3.7532689730526,-2.38568971657671,2.16670305734776));
#63298=CARTESIAN_POINT('Ctrl Pts',(3.75796448197983,-2.43663553209621,2.11060819572134));
#63299=CARTESIAN_POINT('Ctrl Pts',(3.76265999090706,-2.48554343781636,2.05277984879521));
#63300=CARTESIAN_POINT('Ctrl Pts',(3.7673554998343,-2.53229803443386,1.99338511765851));
#63301=CARTESIAN_POINT('Ctrl Pts',(3.77352308979459,-2.59371058527001,1.91536964518692));
#63302=CARTESIAN_POINT('Ctrl Pts',(3.77969067975488,-2.65162685585028,1.83437075499305));
#63303=CARTESIAN_POINT('Ctrl Pts',(3.78585826971516,-2.70574288779974,1.75073498497664));
#63304=CARTESIAN_POINT('Ctrl Pts',(3.79201770503995,-2.75978736886495,1.6672097961149));
#63305=CARTESIAN_POINT('Ctrl Pts',(3.79817714036473,-2.81004136009811,1.58105501493636));
#63306=CARTESIAN_POINT('Ctrl Pts',(3.80433657568952,-2.85624109874265,1.49265010915264));
#63307=CARTESIAN_POINT('Ctrl Pts',(3.81048951699238,-2.90239212803315,1.40433841051642));
#63308=CARTESIAN_POINT('Ctrl Pts',(3.81664245829524,-2.94449719937154,1.31378168439207));
#63309=CARTESIAN_POINT('Ctrl Pts',(3.8227953995981,-2.98233639688537,1.22138739894956));
#63310=CARTESIAN_POINT('Ctrl Pts',(3.82923132885883,-3.0219159063419,1.12474368727824));
#63311=CARTESIAN_POINT('Ctrl Pts',(3.83566725811956,-3.05682748145951,1.02608974805838));
#63312=CARTESIAN_POINT('Ctrl Pts',(3.84210318738029,-3.08687391680823,0.925919534424568));
#63313=CARTESIAN_POINT('Ctrl Pts',(3.84824844188452,-3.11556332352516,0.830273446410853));
#63314=CARTESIAN_POINT('Ctrl Pts',(3.85439369638874,-3.1398173607693,0.733245531105524));
#63315=CARTESIAN_POINT('Ctrl Pts',(3.86053895089296,-3.15951455436372,0.635283671491602));
#63316=CARTESIAN_POINT('Ctrl Pts',(3.86668277880153,-3.17920717533534,0.537344553322039));
#63317=CARTESIAN_POINT('Ctrl Pts',(3.87282660671009,-3.19434497486423,0.438472348615513));
#63318=CARTESIAN_POINT('Ctrl Pts',(3.87897043461866,-3.20485745082501,0.339125761910541));
#63319=CARTESIAN_POINT('Ctrl Pts',(3.88511547167601,-3.21537199571542,0.239759623094642));
#63320=CARTESIAN_POINT('Ctrl Pts',(3.89126050873337,-3.2212593575108,0.13991934830266));
#63321=CARTESIAN_POINT('Ctrl Pts',(3.89740554579072,-3.22250090277616,0.0400686174806361));
#63322=CARTESIAN_POINT('Ctrl Pts',(3.89827921410278,-3.2226774190032,0.0258723777117459));
#63323=CARTESIAN_POINT('Ctrl Pts',(3.89915288241483,-3.22276011248822,0.0116759280118308));
#63324=CARTESIAN_POINT('Ctrl Pts',(3.90002655072689,-3.222749015224,-0.00251939927735915));
#63325=CARTESIAN_POINT('Ctrl Pts',(3.89829624432446,-3.2227489236479,-0.00263393741439584));
#63326=CARTESIAN_POINT('Ctrl Pts',(3.91595129500457,-3.22253094053598,-0.269346743677202));
#63327=CARTESIAN_POINT('Ctrl Pts',(3.93437946122793,-3.18920692885496,-0.534984637514666));
#63328=CARTESIAN_POINT('Ctrl Pts',(3.95516903211871,-3.11145621610261,-0.841051025868991));
#63329=CARTESIAN_POINT('Ctrl Pts',(3.95836463507959,-3.09828573428671,-0.88834265120157));
#63330=CARTESIAN_POINT('Ctrl Pts',(3.96329871450964,-3.07593784755422,-0.962030744259893));
#63331=CARTESIAN_POINT('Ctrl Pts',(3.9650709584551,-3.06748927056815,-0.988638708584469));
#63332=CARTESIAN_POINT('Ctrl Pts',(3.96729513049513,-3.05633221135099,-1.0222559740767));
#63333=CARTESIAN_POINT('Ctrl Pts',(3.96776489670188,-3.0539438401511,-1.02936916922689));
#63334=CARTESIAN_POINT('Ctrl Pts',(3.96851370572064,-3.05008524048497,-1.04072944893667));
#63335=CARTESIAN_POINT('Ctrl Pts',(3.96879367818867,-3.04863095098841,-1.04498185887322));
#63336=CARTESIAN_POINT('Ctrl Pts',(3.96932484246404,-3.04584968754368,-1.05305917867508));
#63337=CARTESIAN_POINT('Ctrl Pts',(3.969576127422,-3.0445244175548,-1.05688458403497));
#63338=CARTESIAN_POINT('Ctrl Pts',(3.97015138851569,-3.0414687597898,-1.065651329487));
#63339=CARTESIAN_POINT('Ctrl Pts',(3.97047507361979,-3.03973353906192,-1.07059095140779));
#63340=CARTESIAN_POINT('Ctrl Pts',(3.97149612218472,-3.03420991239585,-1.08619326721662));
#63341=CARTESIAN_POINT('Ctrl Pts',(3.97219090358894,-3.03037733126317,-1.09684039188465));
#63342=CARTESIAN_POINT('Ctrl Pts',(3.9786022981665,-2.99433214620401,-1.19534474085333));
#63343=CARTESIAN_POINT('Ctrl Pts',(3.9841068925916,-2.95835994717107,-1.28178943134916));
#63344=CARTESIAN_POINT('Ctrl Pts',(3.99110972518947,-2.9067957229066,-1.39191977411194));
#63345=CARTESIAN_POINT('Ctrl Pts',(3.99271202593447,-2.89458882724424,-1.41713006231336));
#63346=CARTESIAN_POINT('Ctrl Pts',(4.00428852625473,-2.80357307851722,-1.59901625877954));
#63347=CARTESIAN_POINT('Ctrl Pts',(4.01395094561155,-2.71241849951249,-1.74918976159062));
#63348=CARTESIAN_POINT('Ctrl Pts',(4.03042749383148,-2.54072946932644,-1.98608731183182));
#63349=CARTESIAN_POINT('Ctrl Pts',(4.03710638507521,-2.46684469302928,-2.077142998892));
#63350=CARTESIAN_POINT('Ctrl Pts',(4.04688930567678,-2.35462230345866,-2.2009924256654));
#63351=CARTESIAN_POINT('Ctrl Pts',(4.04984446173679,-2.32021887943467,-2.23722994215407));
#63352=CARTESIAN_POINT('Ctrl Pts',(4.05481852288709,-2.26161748433221,-2.29614944032516));
#63353=CARTESIAN_POINT('Ctrl Pts',(4.05681737097479,-2.23788630487701,-2.31928451462677));
#63354=CARTESIAN_POINT('Ctrl Pts',(4.05953126288423,-2.20544780410219,-2.34994675160794));
#63355=CARTESIAN_POINT('Ctrl Pts',(4.06023220235083,-2.19705027461547,-2.35779978739771));
#63356=CARTESIAN_POINT('Ctrl Pts',(4.06134673295185,-2.18366818196363,-2.3701806211883));
#63357=CARTESIAN_POINT('Ctrl Pts',(4.06175905420739,-2.17871108628348,-2.37473807132339));
#63358=CARTESIAN_POINT('Ctrl Pts',(4.06261551701357,-2.16840137748681,-2.3841571496871));
#63359=CARTESIAN_POINT('Ctrl Pts',(4.06305975755903,-2.16304661734325,-2.38901636204808));
#63360=CARTESIAN_POINT('Ctrl Pts',(4.06407683804947,-2.15077090230105,-2.4000809349523));
#63361=CARTESIAN_POINT('Ctrl Pts',(4.06465017307326,-2.14383938624236,-2.40627443397515));
#63362=CARTESIAN_POINT('Ctrl Pts',(4.06614639141237,-2.12572092676786,-2.42232334344498));
#63363=CARTESIAN_POINT('Ctrl Pts',(4.06707125096456,-2.11449231445283,-2.43213118042316));
#63364=CARTESIAN_POINT('Ctrl Pts',(4.07304170814661,-2.04182604505612,-2.49471928250622));
#63365=CARTESIAN_POINT('Ctrl Pts',(4.07817919892415,-1.97848995924225,-2.54524133945071));
#63366=CARTESIAN_POINT('Ctrl Pts',(4.09479480746094,-1.77132421879356,-2.69808585921478));
#63367=CARTESIAN_POINT('Ctrl Pts',(4.10659923276721,-1.62097840437645,-2.79099829066499));
#63368=CARTESIAN_POINT('Ctrl Pts',(4.12776499001686,-1.34209428532099,-2.93318331527292));
#63369=CARTESIAN_POINT('Ctrl Pts',(4.13704889169592,-1.21655833503412,-2.98743525391738));
#63370=CARTESIAN_POINT('Ctrl Pts',(4.15046970054646,-1.02646704459472,-3.05560960579081));
#63371=CARTESIAN_POINT('Ctrl Pts',(4.15475995277674,-0.96431830660466,-3.07578867983054));
#63372=CARTESIAN_POINT('Ctrl Pts',(4.16116457666881,-0.868801600061347,
-3.10362176838711));
#63373=CARTESIAN_POINT('Ctrl Pts',(4.16333993794741,-0.835856478455067,
-3.11265617682662));
#63374=CARTESIAN_POINT('Ctrl Pts',(4.16599120262217,-0.794997073074134,
-3.12316532883506));
#63375=CARTESIAN_POINT('Ctrl Pts',(4.16649413383713,-0.787214208670261,
-3.12513612669384));
#63376=CARTESIAN_POINT('Ctrl Pts',(4.16728330530509,-0.774949785126235,
-3.12819303351709));
#63377=CARTESIAN_POINT('Ctrl Pts',(4.16757065511968,-0.770473185579285,
-3.1292986267456));
#63378=CARTESIAN_POINT('Ctrl Pts',(4.16810781299591,-0.762084023043602,
-3.13135141899449));
#63379=CARTESIAN_POINT('Ctrl Pts',(4.16835774720863,-0.7581721014789,-3.1323008846829));
#63380=CARTESIAN_POINT('Ctrl Pts',(4.16892494087611,-0.749275239999326,
-3.1344426055548));
#63381=CARTESIAN_POINT('Ctrl Pts',(4.16924193404962,-0.744289240698065,
-3.13563029705974));
#63382=CARTESIAN_POINT('Ctrl Pts',(4.17018281216945,-0.729450130204712,
-3.13912766342682));
#63383=CARTESIAN_POINT('Ctrl Pts',(4.17080473928084,-0.719588837954609,
-3.14140285388979));
#63384=CARTESIAN_POINT('Ctrl Pts',(4.17525598443436,-0.648647645853428,
-3.15741877596831));
#63385=CARTESIAN_POINT('Ctrl Pts',(4.17899106165022,-0.587184829443091,
-3.16942459992701));
#63386=CARTESIAN_POINT('Ctrl Pts',(4.18916173011016,-0.415915283632065,
-3.19772539964168));
#63387=CARTESIAN_POINT('Ctrl Pts',(4.19544934182919,-0.305554179850657,
-3.21015162654846));
#63388=CARTESIAN_POINT('Ctrl Pts',(4.21755431393519,0.0874498216113729,
-3.23394607130042));
#63389=CARTESIAN_POINT('Ctrl Pts',(4.23308729682306,0.370654043767491,-3.21382288440688));
#63390=CARTESIAN_POINT('Ctrl Pts',(4.25155477586855,0.674258455400089,-3.15154467992324));
#63391=CARTESIAN_POINT('Ctrl Pts',(4.25318660356209,0.700849430980891,-3.14573812355095));
#63392=CARTESIAN_POINT('Ctrl Pts',(4.25606612717574,0.747333206683158,-3.13496903519134));
#63393=CARTESIAN_POINT('Ctrl Pts',(4.25730916102787,0.767258366310866,-3.13015212773323));
#63394=CARTESIAN_POINT('Ctrl Pts',(4.25913808920433,0.79636166062724,-3.12282183015479));
#63395=CARTESIAN_POINT('Ctrl Pts',(4.25971917100869,0.80557703922378,-3.12045729152429));
#63396=CARTESIAN_POINT('Ctrl Pts',(4.26072098326376,0.82141035321995,-3.11631987013151));
#63397=CARTESIAN_POINT('Ctrl Pts',(4.26114107475744,0.828033389607171,-3.11456661606368));
#63398=CARTESIAN_POINT('Ctrl Pts',(4.26197727760211,0.841183904282025,-3.11104049355862));
#63399=CARTESIAN_POINT('Ctrl Pts',(4.26239336944931,0.84771149261833,-3.10926816752015));
#63400=CARTESIAN_POINT('Ctrl Pts',(4.26337473982638,0.863068973691513,-3.10504645305774));
#63401=CARTESIAN_POINT('Ctrl Pts',(4.26394057395368,0.8718940603346,-3.10257993833628));
#63402=CARTESIAN_POINT('Ctrl Pts',(4.26561682598403,0.897949418412696,-3.0951778053476));
#63403=CARTESIAN_POINT('Ctrl Pts',(4.26673069783869,0.915148953000686,-3.09013610988973));
#63404=CARTESIAN_POINT('Ctrl Pts',(4.28126486133419,1.13806839036644,-3.02276747256088));
#63405=CARTESIAN_POINT('Ctrl Pts',(4.29537687310971,1.33705338690073,-2.94016644205476));
#63406=CARTESIAN_POINT('Ctrl Pts',(4.32639973344547,1.74301069113347,-2.72186915882474));
#63407=CARTESIAN_POINT('Ctrl Pts',(4.3433250456539,1.94566558426213,-2.58090206230544));
#63408=CARTESIAN_POINT('Ctrl Pts',(4.36091782157502,2.15160899024179,-2.39947951108252));
#63409=CARTESIAN_POINT('Ctrl Pts',(4.36272024665419,2.17265890588032,-2.38043621678441));
#63410=CARTESIAN_POINT('Ctrl Pts',(4.36497671263521,2.1989843404895,-2.35598013265586));
#63411=CARTESIAN_POINT('Ctrl Pts',(4.36544921676442,2.20449536471763,-2.35082426073199));
#63412=CARTESIAN_POINT('Ctrl Pts',(4.36620136122019,2.21326639038375,-2.34256050775859));
#63413=CARTESIAN_POINT('Ctrl Pts',(4.36648194556313,2.21653803426503,-2.33946510778919));
#63414=CARTESIAN_POINT('Ctrl Pts',(4.36701357296606,2.2227364224219,-2.33357595321866));
#63415=CARTESIAN_POINT('Ctrl Pts',(4.36726471197749,2.22566435921892,-2.33078357924211));
#63416=CARTESIAN_POINT('Ctrl Pts',(4.36783872799068,2.23235606072812,-2.32437759496224));
#63417=CARTESIAN_POINT('Ctrl Pts',(4.36816131830814,2.236116308802,-2.32076035821279));
#63418=CARTESIAN_POINT('Ctrl Pts',(4.36917547428718,2.24793568927166,-2.30933510190075));
#63419=CARTESIAN_POINT('Ctrl Pts',(4.36986450719853,2.25596294352708,-2.30149401086866));
#63420=CARTESIAN_POINT('Ctrl Pts',(4.37604781438054,2.32795000107118,-2.23043791581065));
#63421=CARTESIAN_POINT('Ctrl Pts',(4.38134639890174,2.38928527954381,-2.16460704429943));
#63422=CARTESIAN_POINT('Ctrl Pts',(4.40288769430563,2.63216283490052,-1.88100424711725));
#63423=CARTESIAN_POINT('Ctrl Pts',(4.41816305212166,2.78733281025583,-1.64233218336919));
#63424=CARTESIAN_POINT('Ctrl Pts',(4.43885838217843,2.94193992404305,-1.31790304328928));
#63425=CARTESIAN_POINT('Ctrl Pts',(4.44328939140737,2.97216077692852,-1.24825399633594));
#63426=CARTESIAN_POINT('Ctrl Pts',(4.45051345702558,3.01657237848328,-1.1351176767666));
#63427=CARTESIAN_POINT('Ctrl Pts',(4.45325439504823,3.03234611333544,-1.09228100074657));
#63428=CARTESIAN_POINT('Ctrl Pts',(4.45681548597968,3.05143810003533,-1.03682796817928));
#63429=CARTESIAN_POINT('Ctrl Pts',(4.45760763056258,3.05559745101562,-1.02450520913099));
#63430=CARTESIAN_POINT('Ctrl Pts',(4.4588891876824,3.06218513172882,-1.00459111132922));
#63431=CARTESIAN_POINT('Ctrl Pts',(4.45937705490786,3.06466011764314,-0.997015267418113));
#63432=CARTESIAN_POINT('Ctrl Pts',(4.46030931507377,3.06932687629583,-0.982548915553051));
#63433=CARTESIAN_POINT('Ctrl Pts',(4.46075354100511,3.07152361369001,-0.975660050526738));
#63434=CARTESIAN_POINT('Ctrl Pts',(4.46177050000567,3.07649085479769,-0.959899972315114));
#63435=CARTESIAN_POINT('Ctrl Pts',(4.46234372773577,3.07924619518045,-0.951024081226524));
#63436=CARTESIAN_POINT('Ctrl Pts',(4.46383948733479,3.08631989785583,-0.927884237699482));
#63437=CARTESIAN_POINT('Ctrl Pts',(4.46476399346217,3.09057773973611,-0.913602152527389));
#63438=CARTESIAN_POINT('Ctrl Pts',(4.47072877998744,3.11731407203665,-0.82159425254196));
#63439=CARTESIAN_POINT('Ctrl Pts',(4.47586075644791,3.13695602921426,-0.743080826215379));
#63440=CARTESIAN_POINT('Ctrl Pts',(4.48165066748825,3.15543798602923,-0.655291066412104));
#63441=CARTESIAN_POINT('Ctrl Pts',(4.48222057837829,3.15721853205701,-0.646657872358586));
#63442=CARTESIAN_POINT('Ctrl Pts',(4.48567380185249,3.16777390325158,-0.594395934104295));
#63443=CARTESIAN_POINT('Ctrl Pts',(4.48858136530917,3.17567936920568,-0.550598125370181));
#63444=CARTESIAN_POINT('Ctrl Pts',(4.49187560835493,3.18354548803674,-0.501184932064398));
#63445=CARTESIAN_POINT('Ctrl Pts',(4.49224042986894,3.18440172683359,-0.495715495199595));
#63446=CARTESIAN_POINT('Ctrl Pts',(4.49280733337037,3.18570916257407,-0.487220740518793));
#63447=CARTESIAN_POINT('Ctrl Pts',(4.493009186346,3.18617015481057,-0.484196925819996));
#63448=CARTESIAN_POINT('Ctrl Pts',(4.50975732666851,3.22404370250798,-0.233374463300362));
#63449=CARTESIAN_POINT('Ctrl Pts',(4.52700603721973,3.23242676764566,0.0179129766843247));
#63450=CARTESIAN_POINT('Ctrl Pts',(4.54804329181867,3.20614746278597,0.333283250996289));
#63451=CARTESIAN_POINT('Ctrl Pts',(4.55237211309135,3.19866283930282,0.398768713610387));
#63452=CARTESIAN_POINT('Ctrl Pts',(4.55882751035107,3.18422781735199,0.497987521690504));
#63453=CARTESIAN_POINT('Ctrl Pts',(4.56101615934486,3.17873677105047,0.531912713801335));
#63454=CARTESIAN_POINT('Ctrl Pts',(4.56368135787895,3.1712918014787,0.573664167029947));
#63455=CARTESIAN_POINT('Ctrl Pts',(4.56418526891043,3.16985005671571,0.581577929329981));
#63456=CARTESIAN_POINT('Ctrl Pts',(4.56497563082301,3.16753462372559,0.594022948643385));
#63457=CARTESIAN_POINT('Ctrl Pts',(4.56526319678306,3.16668081961353,0.598557802843704));
#63458=CARTESIAN_POINT('Ctrl Pts',(4.56580054184501,3.16506404260327,0.607044783962373));
#63459=CARTESIAN_POINT('Ctrl Pts',(4.56605044804377,3.16430341426244,0.61099727187183));
#63460=CARTESIAN_POINT('Ctrl Pts',(4.56661729652616,3.16255834201078,0.619974606973294));
#63461=CARTESIAN_POINT('Ctrl Pts',(4.56693397380988,3.1615693289951,0.624998526984795));
#63462=CARTESIAN_POINT('Ctrl Pts',(4.56789410013189,3.15852799447007,0.640255731409609));
#63463=CARTESIAN_POINT('Ctrl Pts',(4.56853542235707,3.15643790680179,0.650481545441991));
#63464=CARTESIAN_POINT('Ctrl Pts',(4.57327594307221,3.14055540117806,0.726307746699716));
#63465=CARTESIAN_POINT('Ctrl Pts',(4.57726698820174,3.12476776345976,0.791479041925194));
#63466=CARTESIAN_POINT('Ctrl Pts',(4.59921349909911,3.02498801926229,1.15359302946905));
#63467=CARTESIAN_POINT('Ctrl Pts',(4.61571281244848,2.90071888045702,1.4377754474775));
#63468=CARTESIAN_POINT('Ctrl Pts',(4.63782943042713,2.69819458869133,1.76395446119005));
#63469=CARTESIAN_POINT('Ctrl Pts',(4.64222709895316,2.65624028263549,1.82652011784748));
#63470=CARTESIAN_POINT('Ctrl Pts',(4.64940142303995,2.5855543073107,1.92434044217195));
#63471=CARTESIAN_POINT('Ctrl Pts',(4.65212687825173,2.55820042827832,1.96055794824799));
#63472=CARTESIAN_POINT('Ctrl Pts',(4.65567055075485,2.52205243337528,2.00637422989547));
#63473=CARTESIAN_POINT('Ctrl Pts',(4.65646110003356,2.5139515553092,2.01651521118285));
#63474=CARTESIAN_POINT('Ctrl Pts',(4.65774069804726,2.50078160397146,2.03279914339153));
#63475=CARTESIAN_POINT('Ctrl Pts',(4.6582282101251,2.49575057705763,2.03897279124818));
#63476=CARTESIAN_POINT('Ctrl Pts',(4.65916020544569,2.4861073345068,2.05071699338566));
#63477=CARTESIAN_POINT('Ctrl Pts',(4.65960452335164,2.48149914416054,2.05629080186186));
#63478=CARTESIAN_POINT('Ctrl Pts',(4.6606222765999,2.47091906603581,2.06900051136248));
#63479=CARTESIAN_POINT('Ctrl Pts',(4.66119620937051,2.46493497673199,2.07612612923487));
#63480=CARTESIAN_POINT('Ctrl Pts',(4.66296453911603,2.44644381899632,2.0979520318141));
#63481=CARTESIAN_POINT('Ctrl Pts',(4.66416309851909,2.4338356597759,2.11256574865444));
#63482=CARTESIAN_POINT('Ctrl Pts',(4.68114258440495,2.25419393527325,2.31704001804854));
#63483=CARTESIAN_POINT('Ctrl Pts',(4.69790376698204,2.06554702547489,2.4866702066965));
#63484=CARTESIAN_POINT('Ctrl Pts',(4.71689863682896,1.83606345053158,2.64873209885375));
#63485=CARTESIAN_POINT('Ctrl Pts',(4.71880447807139,1.81285064742445,2.66467309289869));
#63486=CARTESIAN_POINT('Ctrl Pts',(4.7207101123806,1.78943616882057,2.68030516177109));
#63487=CARTESIAN_POINT('Origin',(-1.72497344927317,0.,0.));
#63488=CARTESIAN_POINT('',(6.21703160867442,1.78943621037803,2.68030513402633));
#63489=CARTESIAN_POINT('',(5.97308385260372,1.78943621012791,2.68030513419332));
#63490=CARTESIAN_POINT('',(-1.72497344927317,1.78943621037804,2.68030513402633));
#63491=CARTESIAN_POINT('',(5.3965734492289,-3.22274863470805,0.00296647727227422));
#63492=CARTESIAN_POINT('Ctrl Pts',(5.3965734492731,-3.22274863470871,0.00296647655588668));
#63493=CARTESIAN_POINT('Ctrl Pts',(5.40274171710666,-3.22284065656237,-0.0970050882467916));
#63494=CARTESIAN_POINT('Ctrl Pts',(5.40890998494021,-3.21827644653641,-0.197093019516699));
#63495=CARTESIAN_POINT('Ctrl Pts',(5.41507825277377,-3.20905173235025,-0.29682409201389));
#63496=CARTESIAN_POINT('Ctrl Pts',(5.42116256464214,-3.1999525752579,-0.395197730191385));
#63497=CARTESIAN_POINT('Ctrl Pts',(5.42724687651051,-3.18631903927338,-0.493223706962624));
#63498=CARTESIAN_POINT('Ctrl Pts',(5.43333118837888,-3.16819941223115,-0.590449021371175));
#63499=CARTESIAN_POINT('Ctrl Pts',(5.43941381045283,-3.15008481754844,-0.687647333417328));
#63500=CARTESIAN_POINT('Ctrl Pts',(5.44549643252677,-3.12748668799687,-0.784044987656764));
#63501=CARTESIAN_POINT('Ctrl Pts',(5.45157905460072,-3.10050477759769,-0.879197182999313));
#63502=CARTESIAN_POINT('Ctrl Pts',(5.45766170092831,-3.07352275961178,-0.974349757748389));
#63503=CARTESIAN_POINT('Ctrl Pts',(5.46374434725589,-3.04215704853434,-1.06825643594335));
#63504=CARTESIAN_POINT('Ctrl Pts',(5.46982699358348,-3.00655750993043,-1.16048675217812));
#63505=CARTESIAN_POINT('Ctrl Pts',(5.47605906722472,-2.97008342706819,-1.25498281388799));
#63506=CARTESIAN_POINT('Ctrl Pts',(5.48229114086597,-2.92916493292472,-1.34771860642642));
#63507=CARTESIAN_POINT('Ctrl Pts',(5.48852321450722,-2.88401526439077,-1.43825363453774));
#63508=CARTESIAN_POINT('Ctrl Pts',(5.49461453428551,-2.83988531908591,-1.52674389301489));
#63509=CARTESIAN_POINT('Ctrl Pts',(5.50070585406379,-2.79171358696322,-1.61313138708066));
#63510=CARTESIAN_POINT('Ctrl Pts',(5.50679717384208,-2.73974460436993,-1.6970318398091));
#63511=CARTESIAN_POINT('Ctrl Pts',(5.51309962441481,-2.6859743286283,-1.78384036006361));
#63512=CARTESIAN_POINT('Ctrl Pts',(5.51940207498753,-2.62813907424609,-1.86798585899725));
#63513=CARTESIAN_POINT('Ctrl Pts',(5.52570452556026,-2.56655578273067,-1.94907900728312));
#63514=CARTESIAN_POINT('Ctrl Pts',(5.53200697613298,-2.50497249121526,-2.03017215556899));
#63515=CARTESIAN_POINT('Ctrl Pts',(5.53830942670571,-2.43964155430169,-2.10821260448766));
#63516=CARTESIAN_POINT('Ctrl Pts',(5.54461187727843,-2.3709213396552,-2.18285353692538));
#63517=CARTESIAN_POINT('Ctrl Pts',(5.55078412537011,-2.30362081760956,-2.25595246050808));
#63518=CARTESIAN_POINT('Ctrl Pts',(5.55695637346178,-2.23281805406449,-2.32606467171766));
#63519=CARTESIAN_POINT('Ctrl Pts',(5.56312862155345,-2.15880867791026,-2.39283569320573));
#63520=CARTESIAN_POINT('Ctrl Pts',(5.56929251020499,-2.08489953702532,-2.45951628275576));
#63521=CARTESIAN_POINT('Ctrl Pts',(5.57545639885653,-2.00779273520899,-2.5228643884479));
#63522=CARTESIAN_POINT('Ctrl Pts',(5.58162028750807,-1.92782257632733,-2.58256029488232));
#63523=CARTESIAN_POINT('Ctrl Pts',(5.58777764916552,-1.84793709852667,-2.64219298881399));
#63524=CARTESIAN_POINT('Ctrl Pts',(5.59393501082297,-1.7651946377974,-2.69818091372776));
#63525=CARTESIAN_POINT('Ctrl Pts',(5.60009237248042,-1.67996387002175,-2.75024343612007));
#63526=CARTESIAN_POINT('Ctrl Pts',(5.60624523662563,-1.59479535722517,-2.80226793056395));
#63527=CARTESIAN_POINT('Ctrl Pts',(5.61239810077084,-1.50714252051476,-2.85037249727189));
#63528=CARTESIAN_POINT('Ctrl Pts',(5.61855096491605,-1.41740366000132,-2.89431933744618));
#63529=CARTESIAN_POINT('Ctrl Pts',(5.62470149805149,-1.3276987970142,-2.93824952838014));
#63530=CARTESIAN_POINT('Ctrl Pts',(5.63085203118693,-1.23590987019932,-2.97802493176923));
#63531=CARTESIAN_POINT('Ctrl Pts',(5.63700256432237,-1.14245967763006,-3.01345374072499));
#63532=CARTESIAN_POINT('Ctrl Pts',(5.64315241253649,-1.04901989164323,-3.04887860434033));
#63533=CARTESIAN_POINT('Ctrl Pts',(5.6493022607506,-0.953919613870974,-3.07995768186979));
#63534=CARTESIAN_POINT('Ctrl Pts',(5.65545210896471,-0.85760056883472,-3.10654773451727));
#63535=CARTESIAN_POINT('Ctrl Pts',(5.66160291734275,-0.761266485691932,
-3.13314193861832));
#63536=CARTESIAN_POINT('Ctrl Pts',(5.66775372572079,-0.663713676084884,
-3.15524561014111));
#63537=CARTESIAN_POINT('Ctrl Pts',(5.67390453409883,-0.565396948671176,
-3.17276596252124));
#63538=CARTESIAN_POINT('Ctrl Pts',(5.68006192046393,-0.46697507635262,-3.1903050520566));
#63539=CARTESIAN_POINT('Ctrl Pts',(5.68621930682905,-0.367788083289609,
-3.20325095803661));
#63540=CARTESIAN_POINT('Ctrl Pts',(5.69237669319415,-0.268298732007348,
-3.21156244729933));
#63541=CARTESIAN_POINT('Ctrl Pts',(5.69853751593004,-0.168753856793466,
-3.21987857511437));
#63542=CARTESIAN_POINT('Ctrl Pts',(5.70469833866593,-0.0689067214065487,
-3.22355511941268));
#63543=CARTESIAN_POINT('Ctrl Pts',(5.71085916140181,0.0307791609832923,
-3.2226030170887));
#63544=CARTESIAN_POINT('Ctrl Pts',(5.71703028431745,0.130631706585357,-3.22164932296026));
#63545=CARTESIAN_POINT('Ctrl Pts',(5.72320140723309,0.230322026786169,-3.21605154903976));
#63546=CARTESIAN_POINT('Ctrl Pts',(5.72937253014873,0.329390835988332,-3.20587261750477));
#63547=CARTESIAN_POINT('Ctrl Pts',(5.73406805210517,0.404770920807088,-3.19812760947802));
#63548=CARTESIAN_POINT('Ctrl Pts',(5.73876357406162,0.47979127179733,-3.18773142797412));
#63549=CARTESIAN_POINT('Ctrl Pts',(5.74345909601806,0.554254408827507,-3.17473142372631));
#63550=CARTESIAN_POINT('Ctrl Pts',(5.74963134411001,0.65213595633563,-3.15764296111061));
#63551=CARTESIAN_POINT('Ctrl Pts',(5.75580359220197,0.749398752610503,-3.13599343576414));
#63552=CARTESIAN_POINT('Ctrl Pts',(5.76197584029392,0.845584758578796,-3.1098398638128));
#63553=CARTESIAN_POINT('Ctrl Pts',(5.76813972894573,0.941640494158123,-3.08372171318868));
#63554=CARTESIAN_POINT('Ctrl Pts',(5.77430361759753,1.03662192261712,-3.05311175354045));
#63555=CARTESIAN_POINT('Ctrl Pts',(5.78046750624934,1.13007933498806,-3.01811833086991));
#63556=CARTESIAN_POINT('Ctrl Pts',(5.78662486790704,1.22343778451035,-2.98316196303218));
#63557=CARTESIAN_POINT('Ctrl Pts',(5.79278222956474,1.31527502176757,-2.94383151175955));
#63558=CARTESIAN_POINT('Ctrl Pts',(5.79893959122244,1.40515562853039,-2.9002853690817));
#63559=CARTESIAN_POINT('Ctrl Pts',(5.80509245536788,1.49497058393905,-2.85677103374626));
#63560=CARTESIAN_POINT('Ctrl Pts',(5.81124531951332,1.58283136057116,-2.80904731792483));
#63561=CARTESIAN_POINT('Ctrl Pts',(5.81739818365876,1.6683225550101,-2.7573206949763));
#63562=CARTESIAN_POINT('Ctrl Pts',(5.82354871679442,1.75378136114909,-2.70561366863523));
#63563=CARTESIAN_POINT('Ctrl Pts',(5.82969924993009,1.83687199761976,-2.64990697305706));
#63564=CARTESIAN_POINT('Ctrl Pts',(5.83584978306576,1.91720450351031,-2.5904525578014));
#63565=CARTESIAN_POINT('Ctrl Pts',(5.84199963128007,1.99752806359925,-2.53100476336998));
#63566=CARTESIAN_POINT('Ctrl Pts',(5.84814947949438,2.07509375460424,-2.46781033741245));
#63567=CARTESIAN_POINT('Ctrl Pts',(5.85429932770869,2.14954223780144,-2.40116341185009));
#63568=CARTESIAN_POINT('Ctrl Pts',(5.86045013608695,2.2240023444969,-2.33450608083164));
#63569=CARTESIAN_POINT('Ctrl Pts',(5.86660094446522,2.29534395303616,-2.26439546930261));
#63570=CARTESIAN_POINT('Ctrl Pts',(5.87275175284348,2.36324309083601,-2.19116399571457));
#63571=CARTESIAN_POINT('Ctrl Pts',(5.87890913920876,2.43121484342397,-2.11785420466759));
#63572=CARTESIAN_POINT('Ctrl Pts',(5.88506652557405,2.49573647768147,-2.04141720585072));
#63573=CARTESIAN_POINT('Ctrl Pts',(5.89122391193933,2.55652308746937,-1.9622199840324));
#63574=CARTESIAN_POINT('Ctrl Pts',(5.89738473467538,2.61734362160708,-1.88297856310071));
#63575=CARTESIAN_POINT('Ctrl Pts',(5.90354555741143,2.67442473190287,-1.80097420790359));
#63576=CARTESIAN_POINT('Ctrl Pts',(5.90970638014748,2.72752499225266,-1.71660274354235));
#63577=CARTESIAN_POINT('Ctrl Pts',(5.91587750306326,2.7807140300675,-1.63209021989668));
#63578=CARTESIAN_POINT('Ctrl Pts',(5.92204862597904,2.82990870962749,-1.54520306020906));
#63579=CARTESIAN_POINT('Ctrl Pts',(5.92821974889481,2.87491362120401,-1.45636164228383));
#63580=CARTESIAN_POINT('Ctrl Pts',(5.93291527084911,2.90915723508805,-1.38876343787074));
#63581=CARTESIAN_POINT('Ctrl Pts',(5.93761079280341,2.94097614644785,-1.3200343281168));
#63582=CARTESIAN_POINT('Ctrl Pts',(5.94230631475771,2.97030340761317,-1.25036603809507));
#63583=CARTESIAN_POINT('Ctrl Pts',(5.94847856285123,3.00885399550898,-1.15878730106632));
#63584=CARTESIAN_POINT('Ctrl Pts',(5.95465081094475,3.04323321164755,-1.06526284977028));
#63585=CARTESIAN_POINT('Ctrl Pts',(5.96082305903828,3.07324135208549,-0.970208819961856));
#63586=CARTESIAN_POINT('Ctrl Pts',(5.96698694769168,3.1032088507266,-0.875283527439711));
#63587=CARTESIAN_POINT('Ctrl Pts',(5.97315083634509,3.12881691071329,-0.778833184511968));
#63588=CARTESIAN_POINT('Ctrl Pts',(5.9793147249985,3.14991351142471,-0.681294674163874));
#63589=CARTESIAN_POINT('Ctrl Pts',(5.98547208665783,3.17098777276636,-0.58385944817328));
#63590=CARTESIAN_POINT('Ctrl Pts',(5.99162944831715,3.18755998108103,-0.485338767800381));
#63591=CARTESIAN_POINT('Ctrl Pts',(5.99778680997648,3.19952794206126,-0.386184554933584));
#63592=CARTESIAN_POINT('Ctrl Pts',(6.00393967412358,3.21148716130211,-0.287102767126425));
#63593=CARTESIAN_POINT('Ctrl Pts',(6.01009253827068,3.21884876767893,-0.187388796797091));
#63594=CARTESIAN_POINT('Ctrl Pts',(6.01624540241778,3.22156183554115,-0.08750372726211));
#63595=CARTESIAN_POINT('Ctrl Pts',(6.02239593555511,3.22427387555884,0.0123435008600179));
#63596=CARTESIAN_POINT('Ctrl Pts',(6.02854646869244,3.22234086457052,0.112361265656007));
#63597=CARTESIAN_POINT('Ctrl Pts',(6.03469700182977,3.21576388893388,0.212085296823836));
#63598=CARTESIAN_POINT('Ctrl Pts',(6.04084685004577,3.20918764570707,0.311798222756611));
#63599=CARTESIAN_POINT('Ctrl Pts',(6.04699669826177,3.1979684945882,0.411217046659547));
#63600=CARTESIAN_POINT('Ctrl Pts',(6.05314654647777,3.18215956384424,0.509880449453238));
#63601=CARTESIAN_POINT('Ctrl Pts',(6.05929735485773,3.16634816488239,0.608559256373909));
#63602=CARTESIAN_POINT('Ctrl Pts',(6.06544816323768,3.14594563168597,0.706481978976487));
#63603=CARTESIAN_POINT('Ctrl Pts',(6.07159897161763,3.12105642232688,0.803196346575431));
#63604=CARTESIAN_POINT('Ctrl Pts',(6.07775635798462,3.09614059518254,0.900014145433683));
#63605=CARTESIAN_POINT('Ctrl Pts',(6.08391374435162,3.06672861867615,0.995620587257379));
#63606=CARTESIAN_POINT('Ctrl Pts',(6.09007113071861,3.03297515199977,1.08957757404048));
#63607=CARTESIAN_POINT('Ctrl Pts',(6.09623195345638,2.9992028478785,1.18358699720231));
#63608=CARTESIAN_POINT('Ctrl Pts',(6.10239277619414,2.96108439406214,1.27594473054054));
#63609=CARTESIAN_POINT('Ctrl Pts',(6.10855359893191,2.91882222058803,1.36623365757895));
#63610=CARTESIAN_POINT('Ctrl Pts',(6.1147247218494,2.87648938967076,1.45667353721176));
#63611=CARTESIAN_POINT('Ctrl Pts',(6.1208958447669,2.82999920333809,1.54503731709485));
#63612=CARTESIAN_POINT('Ctrl Pts',(6.1270669676844,2.7795996271054,1.63093331423929));
#63613=CARTESIAN_POINT('Ctrl Pts',(6.13176248962205,2.74125128774916,1.69629038852556));
#63614=CARTESIAN_POINT('Ctrl Pts',(6.1364580115597,2.70064055927373,1.7602192735415));
#63615=CARTESIAN_POINT('Ctrl Pts',(6.14115353349736,2.65789252322745,1.82255998460178));
#63616=CARTESIAN_POINT('Ctrl Pts',(6.14747670642878,2.60032635103439,1.90651041693621));
#63617=CARTESIAN_POINT('Ctrl Pts',(6.1537998793602,2.53867505022404,1.98788218939877));
#63618=CARTESIAN_POINT('Ctrl Pts',(6.16012305229163,2.47319949154006,2.06625309135788));
#63619=CARTESIAN_POINT('Ctrl Pts',(6.16628612829986,2.4093817137839,2.14263971415732));
#63620=CARTESIAN_POINT('Ctrl Pts',(6.1724492043081,2.34193129278647,2.21617522801198));
#63621=CARTESIAN_POINT('Ctrl Pts',(6.17861228031634,2.2711344639199,2.28649640482885));
#63622=CARTESIAN_POINT('Ctrl Pts',(6.18501550170935,2.19757902365759,2.35955765917228));
#63623=CARTESIAN_POINT('Ctrl Pts',(6.19141872310237,2.12041131911197,2.42914856902415));
#63624=CARTESIAN_POINT('Ctrl Pts',(6.19782194449538,2.03999865167889,2.49489940952503));
#63625=CARTESIAN_POINT('Ctrl Pts',(6.20422516588839,1.9595859842458,2.5606502500259));
#63626=CARTESIAN_POINT('Ctrl Pts',(6.21062838728141,1.87592872881404,2.62256064723214));
#63627=CARTESIAN_POINT('Ctrl Pts',(6.21703160867442,1.78943621037803,2.68030513402633));
#63628=CARTESIAN_POINT('Ctrl Pts',(4.96704894786217,1.78943621037804,2.68030513402633));
#63629=CARTESIAN_POINT('Ctrl Pts',(4.97321265127211,1.7066444304683,2.73557891872023));
#63630=CARTESIAN_POINT('Ctrl Pts',(4.97937635468204,1.62117190020534,2.78709141305354));
#63631=CARTESIAN_POINT('Ctrl Pts',(4.98554005809198,1.53339585901294,2.83457487148637));
#63632=CARTESIAN_POINT('Ctrl Pts',(4.99169728016169,1.44571211726273,2.88200839947501));
#63633=CARTESIAN_POINT('Ctrl Pts',(4.9978545022314,1.3557300601906,2.92542110895884));
#63634=CARTESIAN_POINT('Ctrl Pts',(5.00401172430111,1.26385524948627,2.96458892105567));
#63635=CARTESIAN_POINT('Ctrl Pts',(5.0101645101877,1.17204663315991,3.00372851335058));
#63636=CARTESIAN_POINT('Ctrl Pts',(5.01631729607428,1.07834837282433,3.03862911890848));
#63637=CARTESIAN_POINT('Ctrl Pts',(5.02247008196086,0.983189112428774,3.06911334618022));
#63638=CARTESIAN_POINT('Ctrl Pts',(5.02862057796086,0.888065267521128,3.09958622811596));
#63639=CARTESIAN_POINT('Ctrl Pts',(5.03477107396086,0.791481916196883,3.12564586532792));
#63640=CARTESIAN_POINT('Ctrl Pts',(5.04092156996085,0.693885249456781,3.14716393330349));
#63641=CARTESIAN_POINT('Ctrl Pts',(5.04707142212159,0.596298799220411,3.16867974874905));
#63642=CARTESIAN_POINT('Ctrl Pts',(5.05322127428233,0.497699668663595,3.18565484666855));
#63643=CARTESIAN_POINT('Ctrl Pts',(5.05937112644307,0.398545708663082,3.19801170739043));
#63644=CARTESIAN_POINT('Ctrl Pts',(5.06552197984165,0.299375605722082,3.21037057989345));
#63645=CARTESIAN_POINT('Ctrl Pts',(5.07167283324024,0.199650924991649,3.2181096680155));
#63646=CARTESIAN_POINT('Ctrl Pts',(5.07782368663882,0.0998351228974701,
3.22120327063289));
#63647=CARTESIAN_POINT('Ctrl Pts',(5.08398114074791,-8.77952618458383E-5,
3.22430019311079));
#63648=CARTESIAN_POINT('Ctrl Pts',(5.090138594857,-0.100101595050854,3.22274166192651));
#63649=CARTESIAN_POINT('Ctrl Pts',(5.09629604896609,-0.199742454542215,
3.21655413670491));
#63650=CARTESIAN_POINT('Ctrl Pts',(5.10245697636141,-0.299439519279874,
3.21036312123462));
#63651=CARTESIAN_POINT('Ctrl Pts',(5.10861790375672,-0.398762792994233,
3.19953795893322));
#63652=CARTESIAN_POINT('Ctrl Pts',(5.11477883115204,-0.497255301095885,
3.18415683156971));
#63653=CARTESIAN_POINT('Ctrl Pts',(5.12095001215027,-0.595911729822317,
3.16875010546721));
#63654=CARTESIAN_POINT('Ctrl Pts',(5.12712119314849,-0.69373420557751,3.14877235621637));
#63655=CARTESIAN_POINT('Ctrl Pts',(5.13329237414672,-0.790277517156108,
3.1243525742748));
#63656=CARTESIAN_POINT('Ctrl Pts',(5.13783406269752,-0.861328690825979,
3.10638080451323));
#63657=CARTESIAN_POINT('Ctrl Pts',(5.14237575124833,-0.931687305210557,
3.0860041857128));
#63658=CARTESIAN_POINT('Ctrl Pts',(5.14691743979913,-1.00118270264739,3.06329083803998));
#63659=CARTESIAN_POINT('Ctrl Pts',(5.15308968788507,-1.09562837610406,3.03242293172482));
#63660=CARTESIAN_POINT('Ctrl Pts',(5.15926193597101,-1.18881139356646,2.99712875767385));
#63661=CARTESIAN_POINT('Ctrl Pts',(5.16543418405695,-1.28028652250361,2.95753004765727));
#63662=CARTESIAN_POINT('Ctrl Pts',(5.17159807270263,-1.37163776126896,2.9179849685133));
#63663=CARTESIAN_POINT('Ctrl Pts',(5.17776196134831,-1.46128531392066,2.87414711198939));
#63664=CARTESIAN_POINT('Ctrl Pts',(5.18392584999398,-1.54879951053223,2.82618782791858));
#63665=CARTESIAN_POINT('Ctrl Pts',(5.19008321164546,-1.63622103761536,2.77827932834229));
#63666=CARTESIAN_POINT('Ctrl Pts',(5.19624057329693,-1.72151332099658,2.72625828529251));
#63667=CARTESIAN_POINT('Ctrl Pts',(5.20239793494841,-1.80426797008067,2.67034354618296));
#63668=CARTESIAN_POINT('Ctrl Pts',(5.20855079908749,-1.88696217281123,2.61446964879198));
#63669=CARTESIAN_POINT('Ctrl Pts',(5.21470366322658,-1.96712206760512,2.55470795228538));
#63670=CARTESIAN_POINT('Ctrl Pts',(5.22085652736567,-2.04436592872084,2.49132204100261));
#63671=CARTESIAN_POINT('Ctrl Pts',(5.2270070604949,-2.12158052603394,2.42796014344428));
#63672=CARTESIAN_POINT('Ctrl Pts',(5.23315759362414,-2.19588094935975,2.36097703455927));
#63673=CARTESIAN_POINT('Ctrl Pts',(5.23930812675337,-2.26691713867827,2.29067768332141));
#63674=CARTESIAN_POINT('Ctrl Pts',(5.24545797496119,-2.3379454174294,2.22038616059688));
#63675=CARTESIAN_POINT('Ctrl Pts',(5.25160782316901,-2.40570987612532,2.14677943527788));
#63676=CARTESIAN_POINT('Ctrl Pts',(5.25775767137683,-2.46989677767706,2.07019986236123));
#63677=CARTESIAN_POINT('Ctrl Pts',(5.26390847974851,-2.534093700605,1.9936083332247));
#63678=CARTESIAN_POINT('Ctrl Pts',(5.27005928812018,-2.59471167789402,1.91404336751283));
#63679=CARTESIAN_POINT('Ctrl Pts',(5.27621009649185,-2.65147743549569,1.831880173908));
#63680=CARTESIAN_POINT('Ctrl Pts',(5.28236748285051,-2.70830390128277,1.74962911080928));
#63681=CARTESIAN_POINT('Ctrl Pts',(5.28852486920918,-2.7612696732588,1.66477462916039));
#63682=CARTESIAN_POINT('Ctrl Pts',(5.29468225556784,-2.81014507257187,1.57772058159867));
#63683=CARTESIAN_POINT('Ctrl Pts',(5.30084307829723,-2.8590477487166,1.49061795011468));
#63684=CARTESIAN_POINT('Ctrl Pts',(5.30700390102661,-2.90385531124304,1.40131369632026));
#63685=CARTESIAN_POINT('Ctrl Pts',(5.313164723756,-2.94438522871155,1.3102340201068));
#63686=CARTESIAN_POINT('Ctrl Pts',(5.31933584666511,-2.98498290749258,1.21900206925798));
#63687=CARTESIAN_POINT('Ctrl Pts',(5.32550696957422,-3.02128849784746,1.12598917173341));
#63688=CARTESIAN_POINT('Ctrl Pts',(5.33167809248334,-3.05316851493949,1.0316392692614));
#63689=CARTESIAN_POINT('Ctrl Pts',(5.33637361450182,-3.07742557875266,0.959849734192361));
#63690=CARTESIAN_POINT('Ctrl Pts',(5.34106913652031,-3.09912148371401,0.887286509939943));
#63691=CARTESIAN_POINT('Ctrl Pts',(5.34576465853879,-3.11821729824784,0.814148907392219));
#63692=CARTESIAN_POINT('Ctrl Pts',(5.35378219689036,-3.15082313520839,0.689267471194136));
#63693=CARTESIAN_POINT('Ctrl Pts',(5.36179973524192,-3.17594116881185,0.562355834688537));
#63694=CARTESIAN_POINT('Ctrl Pts',(5.36981727359349,-3.19336690303654,0.434195100261212));
#63695=CARTESIAN_POINT('Ctrl Pts',(5.37766287724397,-3.21041894545287,0.308782750262963));
#63696=CARTESIAN_POINT('Ctrl Pts',(5.38550848089445,-3.22010509332094,0.182174046725123));
#63697=CARTESIAN_POINT('Ctrl Pts',(5.39335408454493,-3.22227854034219,0.0551232342140707));
#63698=CARTESIAN_POINT('Ctrl Pts',(5.39442720610625,-3.22257582439639,0.0377452257951675));
#63699=CARTESIAN_POINT('Ctrl Pts',(5.39550032766758,-3.22273262524449,0.0203589843103794));
#63700=CARTESIAN_POINT('Ctrl Pts',(5.3965734492289,-3.22274863470805,0.00296647727227207));
#63701=CARTESIAN_POINT('Ctrl Pts',(4.7207101123806,1.78943616882057,2.68030516177109));
#63702=CARTESIAN_POINT('Ctrl Pts',(4.72889755303781,1.68883730094667,2.74746738467149));
#63703=CARTESIAN_POINT('Ctrl Pts',(4.73708536016951,1.58451588245051,2.80892691062836));
#63704=CARTESIAN_POINT('Ctrl Pts',(4.74884783452162,1.42647606285484,2.89041694398679));
#63705=CARTESIAN_POINT('Ctrl Pts',(4.75256209441039,1.37530740771152,2.91511138750835));
#63706=CARTESIAN_POINT('Ctrl Pts',(4.75820039870415,1.29526386001628,2.951163970324));
#63707=CARTESIAN_POINT('Ctrl Pts',(4.76017023922003,1.26683476155088,2.96347888543182));
#63708=CARTESIAN_POINT('Ctrl Pts',(4.76260486192707,1.23105341746289,2.97836960271926));
#63709=CARTESIAN_POINT('Ctrl Pts',(4.76309176059549,1.22386468696764,2.98133078305861));
#63710=CARTESIAN_POINT('Ctrl Pts',(4.76386143184421,1.21244756476756,2.98598546723698));
#63711=CARTESIAN_POINT('Ctrl Pts',(4.76414522539568,1.2082262345078,2.98769604791423));
#63712=CARTESIAN_POINT('Ctrl Pts',(4.7646793889452,1.20025852239082,2.99090510085465));
#63713=CARTESIAN_POINT('Ctrl Pts',(4.76492986938302,1.19651299707394,2.9924054690019));
#63714=CARTESIAN_POINT('Ctrl Pts',(4.76550313818908,1.18791953235429,2.99582909188413));
#63715=CARTESIAN_POINT('Ctrl Pts',(4.7658256379411,1.183069744287,2.99774761182303));
#63716=CARTESIAN_POINT('Ctrl Pts',(4.76682112480404,1.16805262906288,3.00364608959917));
#63717=CARTESIAN_POINT('Ctrl Pts',(4.76749174880313,1.15786958805199,3.00758620838922));
#63718=CARTESIAN_POINT('Ctrl Pts',(4.77304955350832,1.07294473958257,3.03995088744119));
#63719=CARTESIAN_POINT('Ctrl Pts',(4.77778229359266,0.99718178801852,3.06563903517259));
#63720=CARTESIAN_POINT('Ctrl Pts',(4.78422070594391,0.890788434429024,3.09734999329969));
#63721=CARTESIAN_POINT('Ctrl Pts',(4.78600620843527,0.860914799047926,3.10578602234764));
#63722=CARTESIAN_POINT('Ctrl Pts',(4.79521992937685,0.70518558911452,3.14734279102525));
#63723=CARTESIAN_POINT('Ctrl Pts',(4.80246024979137,0.577525821225902,3.17325071235259));
#63724=CARTESIAN_POINT('Ctrl Pts',(4.81791077308689,0.303824174325026,3.21172787220646));
#63725=CARTESIAN_POINT('Ctrl Pts',(4.82611557127025,0.157792829201598,3.22220458553662));
#63726=CARTESIAN_POINT('Ctrl Pts',(4.84044737504432,-0.0897860164447993,
3.22309289531064));
#63727=CARTESIAN_POINT('Ctrl Pts',(4.84642857739393,-0.191086800961918,
3.21867550892016));
#63728=CARTESIAN_POINT('Ctrl Pts',(4.85356406895485,-0.308472370281793,
3.20799560519337));
#63729=CARTESIAN_POINT('Ctrl Pts',(4.85456901366792,-0.324928464367025,
3.20637060917226));
#63730=CARTESIAN_POINT('Ctrl Pts',(4.85611132938527,-0.350063723618893,
3.20369308318399));
#63731=CARTESIAN_POINT('Ctrl Pts',(4.85664582190098,-0.358752486085077,
3.20273174543012));
#63732=CARTESIAN_POINT('Ctrl Pts',(4.85757885129767,-0.373881165912992,
3.20099554956769));
#63733=CARTESIAN_POINT('Ctrl Pts',(4.85797688410912,-0.380322884056235,
3.20023657523345));
#63734=CARTESIAN_POINT('Ctrl Pts',(4.85887257845724,-0.394790977802582,
3.19848761903127));
#63735=CARTESIAN_POINT('Ctrl Pts',(4.85937057827695,-0.402815984910783,
3.19748686403015));
#63736=CARTESIAN_POINT('Ctrl Pts',(4.86070444850037,-0.424258832628833,
3.1947308376034));
#63737=CARTESIAN_POINT('Ctrl Pts',(4.86154203241878,-0.437669416811398,
3.19292125715712));
#63738=CARTESIAN_POINT('Ctrl Pts',(4.86413108754685,-0.478953414903274,
3.18708555267426));
#63739=CARTESIAN_POINT('Ctrl Pts',(4.86589141249331,-0.506785175817478,
3.18277856566573));
#63740=CARTESIAN_POINT('Ctrl Pts',(4.88588015665175,-0.820078004787635,
3.13008285547919));
#63741=CARTESIAN_POINT('Ctrl Pts',(4.90540610792843,-1.0977720546638,3.0438087459221));
#63742=CARTESIAN_POINT('Ctrl Pts',(4.93008522002194,-1.42863846504036,2.88977820878815));
#63743=CARTESIAN_POINT('Ctrl Pts',(4.93517866564755,-1.49599355223374,2.85549119888724));
#63744=CARTESIAN_POINT('Ctrl Pts',(4.94487292969805,-1.62329795077774,2.78494511671459));
#63745=CARTESIAN_POINT('Ctrl Pts',(4.94947982821201,-1.68339593601877,2.74903528895032));
#63746=CARTESIAN_POINT('Ctrl Pts',(4.95629943418041,-1.77241189675349,2.69183143069109));
#63747=CARTESIAN_POINT('Ctrl Pts',(4.95858225983423,-1.80221980310142,2.67196639642683));
#63748=CARTESIAN_POINT('Ctrl Pts',(4.96134598561325,-1.8383982849353,2.64697482946214));
#63749=CARTESIAN_POINT('Ctrl Pts',(4.96185666719518,-1.84508726255124,2.64231659701204));
#63750=CARTESIAN_POINT('Ctrl Pts',(4.96265525495301,-1.85555464825873,2.63496793574492));
#63751=CARTESIAN_POINT('Ctrl Pts',(4.96294431461668,-1.85934498715676,2.63229468229927));
#63752=CARTESIAN_POINT('Ctrl Pts',(4.9634829712892,-1.86641132885161,2.62728804862885));
#63753=CARTESIAN_POINT('Ctrl Pts',(4.96373270189526,-1.86968870011267,2.62495674323502));
#63754=CARTESIAN_POINT('Ctrl Pts',(4.96429724730185,-1.87710039171547,2.6196636322268));
#63755=CARTESIAN_POINT('Ctrl Pts',(4.9646118057091,-1.8812320594972,2.61669818010314));
#63756=CARTESIAN_POINT('Ctrl Pts',(4.96553886718725,-1.89341389838191,2.60791105445327));
#63757=CARTESIAN_POINT('Ctrl Pts',(4.96614949669855,-1.9014442792053,2.60206185892142));
#63758=CARTESIAN_POINT('Ctrl Pts',(4.97034096077725,-1.95659864984875,2.56149665843523));
#63759=CARTESIAN_POINT('Ctrl Pts',(4.97383957269568,-2.00279973559225,2.52553709947713));
#63760=CARTESIAN_POINT('Ctrl Pts',(4.97807834840705,-2.0585144629996,2.47968168293472));
#63761=CARTESIAN_POINT('Ctrl Pts',(4.97887508315419,-2.06897518071685,2.47096028997393));
#63762=CARTESIAN_POINT('Ctrl Pts',(4.99744292493297,-2.31237927941527,2.26539805839744));
#63763=CARTESIAN_POINT('Ctrl Pts',(5.01377036702038,-2.51628163786418,2.03653832142762));
#63764=CARTESIAN_POINT('Ctrl Pts',(5.03565214846368,-2.72629913496094,1.72017166620206));
#63765=CARTESIAN_POINT('Ctrl Pts',(5.04001533731903,-2.76543433339587,1.65652325924747));
#63766=CARTESIAN_POINT('Ctrl Pts',(5.0471381840054,-2.82459988479309,1.55234922817117));
#63767=CARTESIAN_POINT('Ctrl Pts',(5.04984758127164,-2.84605163645033,1.51266070543106));
#63768=CARTESIAN_POINT('Ctrl Pts',(5.05337318101048,-2.87258045047479,1.46101569725888));
#63769=CARTESIAN_POINT('Ctrl Pts',(5.05416206613419,-2.87842881188627,1.44945951282848));
#63770=CARTESIAN_POINT('Ctrl Pts',(5.05543962031527,-2.88775779067507,1.43074659975042));
#63771=CARTESIAN_POINT('Ctrl Pts',(5.05592676172055,-2.89128187600284,1.42361160503911));
#63772=CARTESIAN_POINT('Ctrl Pts',(5.05685848179972,-2.89795878723938,1.40996622475054));
#63773=CARTESIAN_POINT('Ctrl Pts',(5.05730289688509,-2.90111619504801,1.40345812511326));
#63774=CARTESIAN_POINT('Ctrl Pts',(5.05832148536821,-2.90829019451131,1.38854330607284));
#63775=CARTESIAN_POINT('Ctrl Pts',(5.05889615910528,-2.91229228069936,1.38012971752261));
#63776=CARTESIAN_POINT('Ctrl Pts',(5.0606690047254,-2.92449867193768,1.35417870018272));
#63777=CARTESIAN_POINT('Ctrl Pts',(5.06187136995943,-2.93258134722859,1.33658484568682));
#63778=CARTESIAN_POINT('Ctrl Pts',(5.07246486218908,-3.00207419271817,1.18165192915195));
#63779=CARTESIAN_POINT('Ctrl Pts',(5.08218257105554,-3.05394721594373,1.0402622234695));
#63780=CARTESIAN_POINT('Ctrl Pts',(5.10765835347028,-3.16079546099927,0.671004030380826));
#63781=CARTESIAN_POINT('Ctrl Pts',(5.12373565919984,-3.20115791289747,0.439829622649969));
#63782=CARTESIAN_POINT('Ctrl Pts',(5.14391216714926,-3.22056034376836,0.137403283518766));
#63783=CARTESIAN_POINT('Ctrl Pts',(5.14845698894086,-3.2227657577853,0.0683430641451825));
#63784=CARTESIAN_POINT('Ctrl Pts',(5.15327882890425,-3.22274859674846,-0.00648848231940785));
#63785=CARTESIAN_POINT('Ctrl Pts',(5.15364864015279,-3.22273189273413,-0.012237924310271));
#63786=CARTESIAN_POINT('Ctrl Pts',(5.15593699760881,-3.22253295606829,-0.0478804029247589));
#63787=CARTESIAN_POINT('Ctrl Pts',(5.15783771205345,-3.2219501873581,-0.0777710069350208));
#63788=CARTESIAN_POINT('Ctrl Pts',(5.16021625910801,-3.2206859222111,-0.115598417512247));
#63789=CARTESIAN_POINT('Ctrl Pts',(5.160714460794,-3.22039086388161,-0.123545500365449));
#63790=CARTESIAN_POINT('Ctrl Pts',(5.16150081984549,-3.21987703759093,-0.136128478418687));
#63791=CARTESIAN_POINT('Ctrl Pts',(5.16179004787196,-3.21967766956908,-0.140765068709603));
#63792=CARTESIAN_POINT('Ctrl Pts',(5.1623288540976,-3.21928683871364,-0.14941882904711));
#63793=CARTESIAN_POINT('Ctrl Pts',(5.16257856662343,-3.21909787388023,-0.153436029083458));
#63794=CARTESIAN_POINT('Ctrl Pts',(5.1631428602973,-3.2186531029101,-0.16252873917902));
#63795=CARTESIAN_POINT('Ctrl Pts',(5.16345718599811,-3.21839281182433,-0.167603990324072));
#63796=CARTESIAN_POINT('Ctrl Pts',(5.1644032282774,-3.21757153438086,-0.182909703286286));
#63797=CARTESIAN_POINT('Ctrl Pts',(5.16503290865684,-3.21697375851345,-0.193138246030363));
#63798=CARTESIAN_POINT('Ctrl Pts',(5.1710497340141,-3.21077041105784,-0.291248051758102));
#63799=CARTESIAN_POINT('Ctrl Pts',(5.17624751060617,-3.20161329406831,-0.378876658762356));
#63800=CARTESIAN_POINT('Ctrl Pts',(5.19051055988408,-3.16592145925169,-0.623103970351996));
#63801=CARTESIAN_POINT('Ctrl Pts',(5.19932033984886,-3.13139041662638,-0.778278640275637));
#63802=CARTESIAN_POINT('Ctrl Pts',(5.22151862429023,-3.01679153699887,-1.15837951672596));
#63803=CARTESIAN_POINT('Ctrl Pts',(5.23497187064074,-2.92295486118273,-1.37810986937873));
#63804=CARTESIAN_POINT('Ctrl Pts',(5.2505422799499,-2.79612047061904,-1.60256447391179));
#63805=CARTESIAN_POINT('Ctrl Pts',(5.25173279219761,-2.78631155790587,-1.61955872236515));
#63806=CARTESIAN_POINT('Ctrl Pts',(5.25349384726213,-2.77164251610682,-1.64444556176316));
#63807=CARTESIAN_POINT('Ctrl Pts',(5.25406002257949,-2.76690242461355,-1.65240866995258));
#63808=CARTESIAN_POINT('Ctrl Pts',(5.25507124026892,-2.75839407345961,-1.66656299846736));
#63809=CARTESIAN_POINT('Ctrl Pts',(5.25551579258902,-2.75463913523243,-1.67276218442448));
#63810=CARTESIAN_POINT('Ctrl Pts',(5.25644683101464,-2.74674503778029,-1.68569622132734));
#63811=CARTESIAN_POINT('Ctrl Pts',(5.25693345971092,-2.74260195079536,-1.69242860732217));
#63812=CARTESIAN_POINT('Ctrl Pts',(5.25820519658536,-2.73173049087484,-1.709949634755));
#63813=CARTESIAN_POINT('Ctrl Pts',(5.25899174813754,-2.72496301622357,-1.72071374171957));
#63814=CARTESIAN_POINT('Ctrl Pts',(5.26243886861109,-2.6951160670158,-1.76756957999835));
#63815=CARTESIAN_POINT('Ctrl Pts',(5.26512373764345,-2.67138281874331,-1.80323775056653));
#63816=CARTESIAN_POINT('Ctrl Pts',(5.27224390785945,-2.6072114551608,-1.89563126465691));
#63817=CARTESIAN_POINT('Ctrl Pts',(5.27672122105514,-2.56563463777498,-1.95153457568684));
#63818=CARTESIAN_POINT('Ctrl Pts',(5.2974457883047,-2.36767535309622,-2.20043695879772));
#63819=CARTESIAN_POINT('Ctrl Pts',(5.31443132934196,-2.19112515066032,-2.37628934424008));
#63820=CARTESIAN_POINT('Ctrl Pts',(5.33490508172688,-1.95200347036751,-2.56494945488731));
#63821=CARTESIAN_POINT('Ctrl Pts',(5.33866429867843,-1.90692482542808,-2.5986383834123));
#63822=CARTESIAN_POINT('Ctrl Pts',(5.34758456467734,-1.79666181233802,-2.67662685626281));
#63823=CARTESIAN_POINT('Ctrl Pts',(5.3527019746806,-1.7306849062489,-2.71975313086025));
#63824=CARTESIAN_POINT('Ctrl Pts',(5.35835849975618,-1.65386987484029,-2.76603512924918));
#63825=CARTESIAN_POINT('Ctrl Pts',(5.3590417944759,-1.64452365985475,-2.77160203480083));
#63826=CARTESIAN_POINT('Ctrl Pts',(5.36004772851081,-1.63066179579676,-2.77976380092835));
#63827=CARTESIAN_POINT('Ctrl Pts',(5.36037268704531,-1.62616787663143,-2.7823951407277));
#63828=CARTESIAN_POINT('Ctrl Pts',(5.36094810680071,-1.6181815122442,-2.78704546587128));
#63829=CARTESIAN_POINT('Ctrl Pts',(5.36119884950261,-1.61469164134779,-2.78906879431733));
#63830=CARTESIAN_POINT('Ctrl Pts',(5.36173207231841,-1.60724924467579,-2.79336503448279));
#63831=CARTESIAN_POINT('Ctrl Pts',(5.36201443259025,-1.60329570529989,-2.79563610514005));
#63832=CARTESIAN_POINT('Ctrl Pts',(5.36277810595028,-1.59256944029108,-2.80176746202727));
#63833=CARTESIAN_POINT('Ctrl Pts',(5.36325838249179,-1.58578745278571,-2.80561160729328));
#63834=CARTESIAN_POINT('Ctrl Pts',(5.36565503026636,-1.55176734975486,-2.82473200947441));
#63835=CARTESIAN_POINT('Ctrl Pts',(5.3675484636385,-1.52432103483468,-2.83963701674303));
#63836=CARTESIAN_POINT('Ctrl Pts',(5.37286635493834,-1.44577798590673,-2.88082360150712));
#63837=CARTESIAN_POINT('Ctrl Pts',(5.37624055838102,-1.39418716725492,-2.9061420397093));
#63838=CARTESIAN_POINT('Ctrl Pts',(5.38838782095632,-1.20341077218617,-2.99351583033522));
#63839=CARTESIAN_POINT('Ctrl Pts',(5.39686388171164,-1.06054321444173,-3.04706230016531));
#63840=CARTESIAN_POINT('Ctrl Pts',(5.4192689498355,-0.676129051834861,-3.16080983430566));
#63841=CARTESIAN_POINT('Ctrl Pts',(5.43325256142525,-0.430526723808855,
-3.20351254883275));
#63842=CARTESIAN_POINT('Ctrl Pts',(5.4494331686977,-0.16308008567044,-3.21867981603252));
#63843=CARTESIAN_POINT('Ctrl Pts',(5.45061182313246,-0.143677569434873,
-3.21960426185394));
#63844=CARTESIAN_POINT('Ctrl Pts',(5.45236472346193,-0.114945883282471,
-3.22071297098948));
#63845=CARTESIAN_POINT('Ctrl Pts',(5.45293473085194,-0.105622122146385,
-3.22103221995875));
#63846=CARTESIAN_POINT('Ctrl Pts',(5.4539490639417,-0.0890652365479059,
-3.22152716796304));
#63847=CARTESIAN_POINT('Ctrl Pts',(5.45439288001523,-0.0818326300813433,
-3.2217190022693));
#63848=CARTESIAN_POINT('Ctrl Pts',(5.45532607225916,-0.0666500331294796,
-3.2220705397702));
#63849=CARTESIAN_POINT('Ctrl Pts',(5.45581560443624,-0.0586999843869909,
-3.22222517838115));
#63850=CARTESIAN_POINT('Ctrl Pts',(5.45710321026734,-0.03782753653005,-3.22255390312858));
#63851=CARTESIAN_POINT('Ctrl Pts',(5.45790279455177,-0.0249046186859661,
-3.22267968207177));
#63852=CARTESIAN_POINT('Ctrl Pts',(5.46148736685304,0.0328534524901184,
-3.22289441478089));
#63853=CARTESIAN_POINT('Ctrl Pts',(5.46429911226672,0.0776850015226813,
-3.22212545869696));
#63854=CARTESIAN_POINT('Ctrl Pts',(5.47183364470494,0.196508924898696,-3.2176061592622));
#63855=CARTESIAN_POINT('Ctrl Pts',(5.47660473649848,0.270409438435103,-3.21223948265726));
#63856=CARTESIAN_POINT('Ctrl Pts',(5.50113489293887,0.643728589395928,-3.17215552209636));
#63857=CARTESIAN_POINT('Ctrl Pts',(5.52201745608186,0.937351417354883,-3.09811035649627));
#63858=CARTESIAN_POINT('Ctrl Pts',(5.54316047746374,1.23420901119516,-2.97711536924643));
#63859=CARTESIAN_POINT('Ctrl Pts',(5.54442429546548,1.25196243184823,-2.96969323383597));
#63860=CARTESIAN_POINT('Ctrl Pts',(5.5494447111496,1.32256125468897,-2.93943249825612));
#63861=CARTESIAN_POINT('Ctrl Pts',(5.55315196123961,1.37486073885267,-2.91533713726405));
#63862=CARTESIAN_POINT('Ctrl Pts',(5.55740256890582,1.43535388935104,-2.8854764739557));
#63863=CARTESIAN_POINT('Ctrl Pts',(5.5580230141851,1.44419748027931,-2.88106038003475));
#63864=CARTESIAN_POINT('Ctrl Pts',(5.55895822408513,1.45755058417665,-2.87431550318754));
#63865=CARTESIAN_POINT('Ctrl Pts',(5.55927482193106,1.46207504634677,-2.87201669162833));
#63866=CARTESIAN_POINT('Ctrl Pts',(5.55984106051881,1.47017467851059,-2.86787728925892));
#63867=CARTESIAN_POINT('Ctrl Pts',(5.56009094908147,1.47375183625143,-2.86604069359192));
#63868=CARTESIAN_POINT('Ctrl Pts',(5.56062862265659,1.48145448869857,-2.86206773913658));
#63869=CARTESIAN_POINT('Ctrl Pts',(5.56091626397239,1.48557878881347,-2.85992916142469));
#63870=CARTESIAN_POINT('Ctrl Pts',(5.56170915873222,1.4969569285186,-2.85399798841326));
#63871=CARTESIAN_POINT('Ctrl Pts',(5.56221323642519,1.50420102729836,-2.85018663189046));
#63872=CARTESIAN_POINT('Ctrl Pts',(5.56494347213424,1.54348843436372,-2.82932474259023));
#63873=CARTESIAN_POINT('Ctrl Pts',(5.56713834889372,1.57525798469487,-2.81176058566938));
#63874=CARTESIAN_POINT('Ctrl Pts',(5.57356807147927,1.66858876870023,-2.75808303758214));
#63875=CARTESIAN_POINT('Ctrl Pts',(5.57772378592383,1.72925749493823,-2.72045592663381));
#63876=CARTESIAN_POINT('Ctrl Pts',(5.59160704639625,1.93061550028086,-2.58611194428732));
#63877=CARTESIAN_POINT('Ctrl Pts',(5.60103092599434,2.06485659210997,-2.48024679972452));
#63878=CARTESIAN_POINT('Ctrl Pts',(5.62235895618099,2.34385979448734,-2.22179574286274));
#63879=CARTESIAN_POINT('Ctrl Pts',(5.63430901274956,2.48334679359652,-2.06470952215054));
#63880=CARTESIAN_POINT('Ctrl Pts',(5.64804667526959,2.61714378049107,-1.88069087504285));
#63881=CARTESIAN_POINT('Ctrl Pts',(5.6491350233813,2.62757754494847,-1.86608573232329));
#63882=CARTESIAN_POINT('Ctrl Pts',(5.65078648714904,2.64315652529494,-1.84388861739465));
#63883=CARTESIAN_POINT('Ctrl Pts',(5.65134613264727,2.64839234682038,-1.83636042898387));
#63884=CARTESIAN_POINT('Ctrl Pts',(5.65232082451493,2.65743520192789,-1.82323928315217));
#63885=CARTESIAN_POINT('Ctrl Pts',(5.65273530943965,2.66125690321684,-1.81765646645598));
#63886=CARTESIAN_POINT('Ctrl Pts',(5.65360088360612,2.66918818435974,-1.80599166058628));
#63887=CARTESIAN_POINT('Ctrl Pts',(5.65405208879384,2.67329461774508,-1.79990758844639));
#63888=CARTESIAN_POINT('Ctrl Pts',(5.6551203284501,2.68295044730295,-1.78549562009286));
#63889=CARTESIAN_POINT('Ctrl Pts',(5.65573803518012,2.68848188463367,-1.77715583571859));
#63890=CARTESIAN_POINT('Ctrl Pts',(5.65778528712872,2.70664219023806,-1.74949659775619));
#63891=CARTESIAN_POINT('Ctrl Pts',(5.65922112716679,2.7191021310095,-1.73006758480355));
#63892=CARTESIAN_POINT('Ctrl Pts',(5.67516639794492,2.85440497721602,-1.51401483145189));
#63893=CARTESIAN_POINT('Ctrl Pts',(5.69048380481867,2.95587114539125,-1.30485813474027));
#63894=CARTESIAN_POINT('Ctrl Pts',(5.71492101471144,3.07792294450576,-0.96408667233382));
#63895=CARTESIAN_POINT('Ctrl Pts',(5.72377684203181,3.11435944439208,-0.838951000405578));
#63896=CARTESIAN_POINT('Ctrl Pts',(5.73504785141941,3.15156641821013,-0.674689902675033));
#63897=CARTESIAN_POINT('Ctrl Pts',(5.73759119740044,3.15934387811338,-0.637278417531664));
#63898=CARTESIAN_POINT('Ctrl Pts',(5.74530553644627,3.18108114465367,-0.52251123320743));
#63899=CARTESIAN_POINT('Ctrl Pts',(5.75041028835494,3.19287925535904,-0.444769182042483));
#63900=CARTESIAN_POINT('Ctrl Pts',(5.75605443042392,3.2030603355405,-0.355865486786565));
#63901=CARTESIAN_POINT('Ctrl Pts',(5.75673731320433,3.20424262222793,-0.345057942485485));
#63902=CARTESIAN_POINT('Ctrl Pts',(5.75774275838028,3.20591018079604,-0.32906622532779));
#63903=CARTESIAN_POINT('Ctrl Pts',(5.75806763678374,3.2064376022514,-0.323886664994365));
#63904=CARTESIAN_POINT('Ctrl Pts',(5.75864296738437,3.20735138934002,-0.314691753231164));
#63905=CARTESIAN_POINT('Ctrl Pts',(5.75889370074057,3.20774276931626,-0.310676939637066));
#63906=CARTESIAN_POINT('Ctrl Pts',(5.75942696083544,3.20856053681283,-0.302121894131053));
#63907=CARTESIAN_POINT('Ctrl Pts',(5.7597093675177,3.20898482486157,-0.297581504344874));
#63908=CARTESIAN_POINT('Ctrl Pts',(5.76047329679431,3.21010862814966,-0.285273521559014));
#63909=CARTESIAN_POINT('Ctrl Pts',(5.76095378165595,3.21078959236411,-0.277504203862379));
#63910=CARTESIAN_POINT('Ctrl Pts',(5.76335314240504,3.21405956354168,-0.238571824618321));
#63911=CARTESIAN_POINT('Ctrl Pts',(5.76524901810381,3.21622322327722,-0.207373438937877));
#63912=CARTESIAN_POINT('Ctrl Pts',(5.77057560098595,3.22107869908176,-0.118671502974028));
#63913=CARTESIAN_POINT('Ctrl Pts',(5.7739558555122,3.22268463764689,-0.0611182975021338));
#63914=CARTESIAN_POINT('Ctrl Pts',(5.78613207429108,3.22291632152688,0.149231078375076));
#63915=CARTESIAN_POINT('Ctrl Pts',(5.79462973340814,3.21222010033394,0.301840421944264));
#63916=CARTESIAN_POINT('Ctrl Pts',(5.81702568812176,3.1558783932238,0.698579115131917));
#63917=CARTESIAN_POINT('Ctrl Pts',(5.83097945610616,3.09282206715676,0.939153625007292));
#63918=CARTESIAN_POINT('Ctrl Pts',(5.84712547503115,2.99576923190468,1.18821797460142));
#63919=CARTESIAN_POINT('Ctrl Pts',(5.84830470697859,2.9885496161645,1.20626133657158));
#63920=CARTESIAN_POINT('Ctrl Pts',(5.85005830329574,2.97762271635811,1.23286965720333));
#63921=CARTESIAN_POINT('Ctrl Pts',(5.85062842422423,2.97404062098887,1.24148580920065));
#63922=CARTESIAN_POINT('Ctrl Pts',(5.8516428854621,2.96761460890325,1.2567551260341));
#63923=CARTESIAN_POINT('Ctrl Pts',(5.85208671568457,2.96478559910676,1.26341452570482));
#63924=CARTESIAN_POINT('Ctrl Pts',(5.85301986263168,2.9588009165535,1.27737148518713));
#63925=CARTESIAN_POINT('Ctrl Pts',(5.85350933508997,2.95564062033671,1.28466699832001));
#63926=CARTESIAN_POINT('Ctrl Pts',(5.85479661463763,2.94727424481757,1.30378640735182));
#63927=CARTESIAN_POINT('Ctrl Pts',(5.85559593096266,2.94202404568027,1.31559073308843));
#63928=CARTESIAN_POINT('Ctrl Pts',(5.85917762242479,2.91825392711395,1.36818055093342));
#63929=CARTESIAN_POINT('Ctrl Pts',(5.86198670215332,2.8989565989596,1.40860722495973));
#63930=CARTESIAN_POINT('Ctrl Pts',(5.86951245628708,2.84556802897912,1.51470585722151));
#63931=CARTESIAN_POINT('Ctrl Pts',(5.8742772969735,2.81004869436329,1.57962533104583));
#63932=CARTESIAN_POINT('Ctrl Pts',(5.89867019027559,2.61966248410134,1.9008239562834));
#63933=CARTESIAN_POINT('Ctrl Pts',(5.91940508677537,2.43187999099283,2.13580939587745));
#63934=CARTESIAN_POINT('Ctrl Pts',(5.94428996814489,2.1579990584637,2.39482412440752));
#63935=CARTESIAN_POINT('Ctrl Pts',(5.94932930149055,2.09968983458391,2.44610861811486));
#63936=CARTESIAN_POINT('Ctrl Pts',(5.9549094112946,2.03118878406254,2.50210054715396));
#63937=CARTESIAN_POINT('Ctrl Pts',(5.95559015323106,2.02276268848518,2.50891732397592));
#63938=CARTESIAN_POINT('Ctrl Pts',(5.95659305738822,2.01024333330193,2.51894151184184));
#63939=CARTESIAN_POINT('Ctrl Pts',(5.9569175189599,2.00617654931791,2.52218164552797));
#63940=CARTESIAN_POINT('Ctrl Pts',(5.95749238614854,1.99894149602068,2.52791746776035));
#63941=CARTESIAN_POINT('Ctrl Pts',(5.95774307124977,1.99577637252504,2.53041706045841));
#63942=CARTESIAN_POINT('Ctrl Pts',(5.95827652688141,1.98901936935805,2.53573270315456));
#63943=CARTESIAN_POINT('Ctrl Pts',(5.95855917623622,1.98542620965538,2.53854705691229));
#63944=CARTESIAN_POINT('Ctrl Pts',(5.95931474457315,1.97578671202714,2.54606423822666));
#63945=CARTESIAN_POINT('Ctrl Pts',(5.9597866825447,1.96972952012782,2.55075319404933));
#63946=CARTESIAN_POINT('Ctrl Pts',(5.9620926199515,1.9399593527002,2.57362941123228));
#63947=CARTESIAN_POINT('Ctrl Pts',(5.96390568285206,1.91600998027129,2.59150854571359));
#63948=CARTESIAN_POINT('Ctrl Pts',(5.96819555235161,1.85815175216488,2.63346133104188));
#63949=CARTESIAN_POINT('Ctrl Pts',(5.97065400470327,1.82401930717595,2.65721662634895));
#63950=CARTESIAN_POINT('Ctrl Pts',(5.97308385260372,1.78943621012791,2.68030513419332));
#63951=CARTESIAN_POINT('Origin',(-1.72497344927317,0.,0.));
#63952=CARTESIAN_POINT('',(7.46680874532645,1.78773599488616,2.67780888195836));
#63953=CARTESIAN_POINT('',(7.21834907457188,1.78943621037019,2.68030513403157));
#63954=CARTESIAN_POINT('',(-1.72497344927317,1.78943621037804,2.68030513402633));
#63955=CARTESIAN_POINT('',(6.64657350830208,-3.22229727948493,-0.000739368720723987));
#63956=CARTESIAN_POINT('Ctrl Pts',(6.6465741241696,-3.21757478926457,-0.000748300723235639));
#63957=CARTESIAN_POINT('Ctrl Pts',(6.67694781268516,-3.21857998498449,-0.494633764188327));
#63958=CARTESIAN_POINT('Ctrl Pts',(6.77360390744728,-2.87916867694032,-2.06497840680236));
#63959=CARTESIAN_POINT('Ctrl Pts',(6.93654240845592,-0.430758100710129,
-3.78721504552185));
#63960=CARTESIAN_POINT('Ctrl Pts',(7.13538962719558,2.95292374036488,-2.41014350732934));
#63961=CARTESIAN_POINT('Ctrl Pts',(7.31214507281908,3.54954199346338,0.78188138285321));
#63962=CARTESIAN_POINT('Ctrl Pts',(7.42261811219602,2.381146258819,2.27471913214447));
#63963=CARTESIAN_POINT('Ctrl Pts',(7.46680874532643,1.78773599488645,2.67780888195817));
#63964=CARTESIAN_POINT('Ctrl Pts',(6.21703160867442,1.78943621037803,2.68030513402633));
#63965=CARTESIAN_POINT('Ctrl Pts',(6.22318199248066,1.70635893534742,2.73576952213351));
#63966=CARTESIAN_POINT('Ctrl Pts',(6.22933237628689,1.6206664666419,2.78739051154453));
#63967=CARTESIAN_POINT('Ctrl Pts',(6.23548276009313,1.53275288481828,2.83492260151512));
#63968=CARTESIAN_POINT('Ctrl Pts',(6.24163263185455,1.44484662216293,2.88245073424318));
#63969=CARTESIAN_POINT('Ctrl Pts',(6.24778250361596,1.35471999623927,2.92589043788173));
#63970=CARTESIAN_POINT('Ctrl Pts',(6.25393237537738,1.26279218109299,2.96504190018799));
#63971=CARTESIAN_POINT('Ctrl Pts',(6.26008338015052,1.1708474297737,3.00420057550087));
#63972=CARTESIAN_POINT('Ctrl Pts',(6.26623438492366,1.07710122971745,3.03906926992255));
#63973=CARTESIAN_POINT('Ctrl Pts',(6.2723853896968,0.981992300571668,3.06949648706721));
#63974=CARTESIAN_POINT('Ctrl Pts',(6.27854306737219,0.886780192740341,3.09995671310282));
#63975=CARTESIAN_POINT('Ctrl Pts',(6.28470074504757,0.790202818575205,3.12596570894925));
#63976=CARTESIAN_POINT('Ctrl Pts',(6.29085842272296,0.692713482170955,3.14742205528883));
#63977=CARTESIAN_POINT('Ctrl Pts',(6.29701969212446,0.59516728098533,3.16889091695049));
#63978=CARTESIAN_POINT('Ctrl Pts',(6.30318096152596,0.496708486284033,3.18580176775673));
#63979=CARTESIAN_POINT('Ctrl Pts',(6.30934223092745,0.397797938362765,3.19810480796586));
#63980=CARTESIAN_POINT('Ctrl Pts',(6.31551360593972,0.298725159019201,3.21042802741526));
#63981=CARTESIAN_POINT('Ctrl Pts',(6.32168498095198,0.199199579665378,3.21812830966896));
#63982=CARTESIAN_POINT('Ctrl Pts',(6.32785635596424,0.0996845383678606,
3.22120793419338));
#63983=CARTESIAN_POINT('Ctrl Pts',(6.33190448805516,0.0344073462664452,
3.22322802320766));
#63984=CARTESIAN_POINT('Ctrl Pts',(6.33595262014608,-0.0308653211708774,
3.22326103675657));
#63985=CARTESIAN_POINT('Ctrl Pts',(6.340000752237,-0.0960040035847728,3.22131972858884));
#63986=CARTESIAN_POINT('Ctrl Pts',(6.34617300032967,-0.195321935722083,
3.21835978672765));
#63987=CARTESIAN_POINT('Ctrl Pts',(6.35234524842235,-0.294677661022926,
3.21079715891031));
#63988=CARTESIAN_POINT('Ctrl Pts',(6.35851749651503,-0.393609690530847,
3.19862298091229));
#63989=CARTESIAN_POINT('Ctrl Pts',(6.36468138516757,-0.492407730548108,
3.18646529112255));
#63990=CARTESIAN_POINT('Ctrl Pts',(6.37084527382011,-0.590782788007754,
3.16970851774315));
#63991=CARTESIAN_POINT('Ctrl Pts',(6.37700916247265,-0.688274301395501,
3.14839578969013));
#63992=CARTESIAN_POINT('Ctrl Pts',(6.38316652413105,-0.785662580190206,
3.12710562986619));
#63993=CARTESIAN_POINT('Ctrl Pts',(6.38932388578945,-0.882168752945351,
3.10126919886733));
#63994=CARTESIAN_POINT('Ctrl Pts',(6.39548124744785,-0.977339268365972,
3.07098119776235));
#63995=CARTESIAN_POINT('Ctrl Pts',(6.40163411159406,-1.07244026853358,3.04071531987537));
#63996=CARTESIAN_POINT('Ctrl Pts',(6.40778697574027,-1.16620713835917,3.0060044678594));
#63997=CARTESIAN_POINT('Ctrl Pts',(6.41393983988647,-1.25819928246394,2.96699378632771));
#63998=CARTESIAN_POINT('Ctrl Pts',(6.42009037302291,-1.35015657538704,2.92799788397485));
#63999=CARTESIAN_POINT('Ctrl Pts',(6.42624090615936,-1.44034007909369,2.88470555829441));
#64000=CARTESIAN_POINT('Ctrl Pts',(6.4323914392958,-1.5283278977627,2.83731059269517));
#64001=CARTESIAN_POINT('Ctrl Pts',(6.43854128751092,-1.61630591813751,2.78992090498353));
#64002=CARTESIAN_POINT('Ctrl Pts',(6.44469113572604,-1.70208835717323,2.7384296916691));
#64003=CARTESIAN_POINT('Ctrl Pts',(6.45084098394116,-1.78527761495446,2.68307685317482));
#64004=CARTESIAN_POINT('Ctrl Pts',(6.45699179232021,-1.86847986091403,2.62771537254866));
#64005=CARTESIAN_POINT('Ctrl Pts',(6.46314260069927,-1.94908775977593,2.56849130986104));
#64006=CARTESIAN_POINT('Ctrl Pts',(6.46929340907832,-2.02673325841858,2.50568750280637));
#64007=CARTESIAN_POINT('Ctrl Pts',(6.47545079544441,-2.104461795103,2.44281653016908));
#64008=CARTESIAN_POINT('Ctrl Pts',(6.4816081818105,-2.17922126673205,2.3763584420281));
#64009=CARTESIAN_POINT('Ctrl Pts',(6.48776556817658,-2.25067735984032,2.3066358586483));
#64010=CARTESIAN_POINT('Ctrl Pts',(6.49392639091343,-2.32217333182166,2.23687436384849));
#64011=CARTESIAN_POINT('Ctrl Pts',(6.50008721365028,-2.39036195736178,2.16384506306423));
#64012=CARTESIAN_POINT('Ctrl Pts',(6.50624803638714,-2.45494784745847,2.08790532083211));
#64013=CARTESIAN_POINT('Ctrl Pts',(6.51241915930372,-2.51964171765855,2.01183861617514));
#64014=CARTESIAN_POINT('Ctrl Pts',(6.5185902822203,-2.58072055510864,1.93285209432769));
#64015=CARTESIAN_POINT('Ctrl Pts',(6.52476140513689,-2.63793101694836,1.85133398184169));
#64016=CARTESIAN_POINT('Ctrl Pts',(6.52945692708347,-2.68146166489912,1.78930797921684));
#64017=CARTESIAN_POINT('Ctrl Pts',(6.53415244903006,-2.72275359754839,1.72581695680638));
#64018=CARTESIAN_POINT('Ctrl Pts',(6.53884797097664,-2.76171321871341,1.66104113738451));
#64019=CARTESIAN_POINT('Ctrl Pts',(6.54522897047855,-2.814657561446,1.5730137623305));
#64020=CARTESIAN_POINT('Ctrl Pts',(6.55160996998045,-2.86346905836085,1.48232057530728));
#64021=CARTESIAN_POINT('Ctrl Pts',(6.55799096948236,-2.90787957691214,1.38937177482388));
#64022=CARTESIAN_POINT('Ctrl Pts',(6.56436131346836,-2.95221593514005,1.29657818786482));
#64023=CARTESIAN_POINT('Ctrl Pts',(6.57073165745436,-2.99216577134845,1.20153683592625));
#64024=CARTESIAN_POINT('Ctrl Pts',(6.57710200144036,-3.0275054200815,1.10468479390148));
#64025=CARTESIAN_POINT('Ctrl Pts',(6.58345995029587,-3.06277630650617,1.00802120224957));
#64026=CARTESIAN_POINT('Ctrl Pts',(6.58981789915138,-3.09345474225247,0.909554307574703));
#64027=CARTESIAN_POINT('Ctrl Pts',(6.59617584800689,-3.11936447139286,0.809742463448692));
#64028=CARTESIAN_POINT('Ctrl Pts',(6.60252648263553,-3.14524439380762,0.710045443535499));
#64029=CARTESIAN_POINT('Ctrl Pts',(6.60887711726416,-3.1663664260796,0.609006931994015));
#64030=CARTESIAN_POINT('Ctrl Pts',(6.6152277518928,-3.18260348814076,0.50710215911025));
#64031=CARTESIAN_POINT('Ctrl Pts',(6.62157054481824,-3.19882050083223,0.405323217270099));
#64032=CARTESIAN_POINT('Ctrl Pts',(6.62791333774369,-3.21016449675425,0.302680532611692));
#64033=CARTESIAN_POINT('Ctrl Pts',(6.63425613066913,-3.21655923055724,0.199660408737013));
#64034=CARTESIAN_POINT('Ctrl Pts',(6.63836190353712,-3.22069862543501,0.132974134341265));
#64035=CARTESIAN_POINT('Ctrl Pts',(6.64246767640511,-3.22276523869596,0.0661299544462664));
#64036=CARTESIAN_POINT('Ctrl Pts',(6.6465734492731,-3.22274991538269,-0.000738512616256426));
#64037=CARTESIAN_POINT('',(6.3999017287312,-3.22274859466306,0.0029702797283874));
#64038=CARTESIAN_POINT('Ctrl Pts',(5.97308385260372,1.78943621012791,2.68030513419332));
#64039=CARTESIAN_POINT('Ctrl Pts',(5.97382137809763,1.77893929148273,2.6873131296931));
#64040=CARTESIAN_POINT('Ctrl Pts',(5.97455626689363,1.76840085472424,2.69425969489273));
#64041=CARTESIAN_POINT('Ctrl Pts',(5.98318330575682,1.64380063053863,2.77534567482014));
#64042=CARTESIAN_POINT('Ctrl Pts',(5.99079261356728,1.52518809352019,2.84225796292038));
#64043=CARTESIAN_POINT('Ctrl Pts',(6.01229269678686,1.1788490015796,3.00969270911703));
#64044=CARTESIAN_POINT('Ctrl Pts',(6.02616469092226,0.943264145075388,3.09162894070542));
#64045=CARTESIAN_POINT('Ctrl Pts',(6.04149556839256,0.693084938689063,3.14734973413928));
#64046=CARTESIAN_POINT('Ctrl Pts',(6.04195784563979,0.685548664864803,3.14899985833507));
#64047=CARTESIAN_POINT('Ctrl Pts',(6.04410465739919,0.650586473199476,3.15652363919426));
#64048=CARTESIAN_POINT('Ctrl Pts',(6.04579931469567,0.62309118595241,3.1620660242917));
#64049=CARTESIAN_POINT('Ctrl Pts',(6.04818425143307,0.58456082007855,3.16931076653259));
#64050=CARTESIAN_POINT('Ctrl Pts',(6.04886486996055,0.573583407319249,3.17131584002005));
#64051=CARTESIAN_POINT('Ctrl Pts',(6.04996374001142,0.555891145472322,3.17445254552118));
#64052=CARTESIAN_POINT('Ctrl Pts',(6.05038084803096,0.549182671943636,3.17561999003182));
#64053=CARTESIAN_POINT('Ctrl Pts',(6.05124712165015,0.535265257883513,3.17799655394394));
#64054=CARTESIAN_POINT('Ctrl Pts',(6.05169638797248,0.528055808980083,3.17920242425297));
#64055=CARTESIAN_POINT('Ctrl Pts',(6.05275158514046,0.511142986195283,3.1819721889565));
#64056=CARTESIAN_POINT('Ctrl Pts',(6.05335814304593,0.501436476991041,3.18351623519368));
#64057=CARTESIAN_POINT('Ctrl Pts',(6.05528345677849,0.470676666321469,3.18826513174473));
#64058=CARTESIAN_POINT('Ctrl Pts',(6.05660740683802,0.44959892094112,3.19130566535268));
#64059=CARTESIAN_POINT('Ctrl Pts',(6.064666679993,0.321762238951724,3.20845493654918));
#64060=CARTESIAN_POINT('Ctrl Pts',(6.07156351342504,0.214392382068316,3.2174128660244));
#64061=CARTESIAN_POINT('Ctrl Pts',(6.09225405842035,-0.101761957662599,
3.22789431233396));
#64062=CARTESIAN_POINT('Ctrl Pts',(6.10643511298629,-0.310470080563394,
3.21453701411536));
#64063=CARTESIAN_POINT('Ctrl Pts',(6.13153438876407,-0.677276735840849,
3.15499269748844));
#64064=CARTESIAN_POINT('Ctrl Pts',(6.14243818045279,-0.835967764825255,
3.11670566790433));
#64065=CARTESIAN_POINT('Ctrl Pts',(6.15349346429487,-1.00252927274747,3.06287397228893));
#64066=CARTESIAN_POINT('Ctrl Pts',(6.15424883353228,-1.01394107149312,3.05911513792747));
#64067=CARTESIAN_POINT('Ctrl Pts',(6.15533620328506,-1.03041809104095,3.05358558160261));
#64068=CARTESIAN_POINT('Ctrl Pts',(6.15567113257438,-1.03550016349634,3.05186594707372));
#64069=CARTESIAN_POINT('Ctrl Pts',(6.15625868381738,-1.04442794500729,3.04882016159024));
#64070=CARTESIAN_POINT('Ctrl Pts',(6.15651162437462,-1.04827546782294,3.04749941006308));
#64071=CARTESIAN_POINT('Ctrl Pts',(6.15703909915638,-1.05630776115386,3.04472512727521));
#64072=CARTESIAN_POINT('Ctrl Pts',(6.15731355172057,-1.0604920297935,3.04327025455244));
#64073=CARTESIAN_POINT('Ctrl Pts',(6.15803372556163,-1.07148425274696,3.03942282852475));
#64074=CARTESIAN_POINT('Ctrl Pts',(6.158478603651,-1.07828724146511,3.03701601275));
#64075=CARTESIAN_POINT('Ctrl Pts',(6.16021892737412,-1.10494660587794,3.02748337876476));
#64076=CARTESIAN_POINT('Ctrl Pts',(6.1615044775537,-1.12474143331095,3.02018532102644));
#64077=CARTESIAN_POINT('Ctrl Pts',(6.16489885401067,-1.17722620165466,3.00024737443334));
#64078=CARTESIAN_POINT('Ctrl Pts',(6.16698978400142,-1.20978485802285,2.987267421338));
#64079=CARTESIAN_POINT('Ctrl Pts',(6.1765516726158,-1.35930219680581,2.92481464276314));
#64080=CARTESIAN_POINT('Ctrl Pts',(6.18374221081456,-1.47349319523562,2.86898354333662));
#64081=CARTESIAN_POINT('Ctrl Pts',(6.19770433795226,-1.69022356439396,2.74665471137447));
#64082=CARTESIAN_POINT('Ctrl Pts',(6.20447050041648,-1.79286398885752,2.68078467120398));
#64083=CARTESIAN_POINT('Ctrl Pts',(6.22174523216218,-2.041157682195,2.50078948819136));
#64084=CARTESIAN_POINT('Ctrl Pts',(6.23236606783285,-2.18115881205774,2.37966482749067));
#64085=CARTESIAN_POINT('Ctrl Pts',(6.24460345092098,-2.32247442787637,2.23440150736585));
#64086=CARTESIAN_POINT('Ctrl Pts',(6.2456881639417,-2.33484097019767,2.22147590313542));
#64087=CARTESIAN_POINT('Ctrl Pts',(6.24733502941737,-2.35337233938425,2.20178109697871));
#64088=CARTESIAN_POINT('Ctrl Pts',(6.24789373916421,-2.35961711808893,2.19508733769179));
#64089=CARTESIAN_POINT('Ctrl Pts',(6.24886725733398,-2.37042469176068,2.18340332139101));
#64090=CARTESIAN_POINT('Ctrl Pts',(6.2492815076807,-2.37500048041929,2.17842511922576));
#64091=CARTESIAN_POINT('Ctrl Pts',(6.25014703678115,-2.38451285786626,2.16801058960294));
#64092=CARTESIAN_POINT('Ctrl Pts',(6.25059843290165,-2.38944659574495,2.16257172149734));
#64093=CARTESIAN_POINT('Ctrl Pts',(6.25166792727152,-2.4010715459777,2.14966822706807));
#64094=CARTESIAN_POINT('Ctrl Pts',(6.25228670214189,-2.40774657355811,2.14218918147963));
#64095=CARTESIAN_POINT('Ctrl Pts',(6.25359196767678,-2.42171984071978,2.12638499487344));
#64096=CARTESIAN_POINT('Ctrl Pts',(6.25427877361462,-2.42901028008742,2.11805315978178));
#64097=CARTESIAN_POINT('Ctrl Pts',(6.25955085600118,-2.48449703295501,2.05397720278075));
#64098=CARTESIAN_POINT('Ctrl Pts',(6.26421311525487,-2.53080813159671,1.99663632618325));
#64099=CARTESIAN_POINT('Ctrl Pts',(6.27570067550211,-2.63823803695987,1.85387171413791));
#64100=CARTESIAN_POINT('Ctrl Pts',(6.28259802645541,-2.69722277558864,1.76695388816216));
#64101=CARTESIAN_POINT('Ctrl Pts',(6.29553432983563,-2.79819382187388,1.60129800499984));
#64102=CARTESIAN_POINT('Ctrl Pts',(6.30153843165868,-2.84135898120196,1.52339161236876));
#64103=CARTESIAN_POINT('Ctrl Pts',(6.31623877924124,-2.93870800537018,1.32912240599941));
#64104=CARTESIAN_POINT('Ctrl Pts',(6.32494511627583,-2.9892778123745,1.21111162310591));
#64105=CARTESIAN_POINT('Ctrl Pts',(6.33971242560796,-3.06446338854289,1.00200092214054));
#64106=CARTESIAN_POINT('Ctrl Pts',(6.34584922200872,-3.09236978229926,0.912246987247727));
#64107=CARTESIAN_POINT('Ctrl Pts',(6.35249324569459,-3.11920321585724,0.810442538773199));
#64108=CARTESIAN_POINT('Ctrl Pts',(6.35320484388622,-3.12203188112718,0.79947654918524));
#64109=CARTESIAN_POINT('Ctrl Pts',(6.35424075017343,-3.12608409086974,0.78341767112212));
#64110=CARTESIAN_POINT('Ctrl Pts',(6.35456761827228,-3.12735308021812,0.778336497403659));
#64111=CARTESIAN_POINT('Ctrl Pts',(6.35514590202078,-3.12958111450049,0.769321780665932));
#64112=CARTESIAN_POINT('Ctrl Pts',(6.35539760459214,-3.13054513902967,0.765389500619389));
#64113=CARTESIAN_POINT('Ctrl Pts',(6.35592772856685,-3.13256341375496,0.757089301730397));
#64114=CARTESIAN_POINT('Ctrl Pts',(6.35620604917879,-3.13361593727993,0.752721004226726));
#64115=CARTESIAN_POINT('Ctrl Pts',(6.35677270642933,-3.13574426683613,0.743805946100877));
#64116=CARTESIAN_POINT('Ctrl Pts',(6.35706099989135,-3.13681932845788,0.739259016657208));
#64117=CARTESIAN_POINT('Ctrl Pts',(6.35777869344282,-3.13947613799955,0.727912002815692));
#64118=CARTESIAN_POINT('Ctrl Pts',(6.35820740949357,-3.14104569359581,0.721109047052204));
#64119=CARTESIAN_POINT('Ctrl Pts',(6.35940976951335,-3.14539775027651,0.701962015149182));
#64120=CARTESIAN_POINT('Ctrl Pts',(6.36018067173886,-3.14812971049966,0.689606420923647));
#64121=CARTESIAN_POINT('Ctrl Pts',(6.37468856005444,-3.19841392860664,0.455662524500434));
#64122=CARTESIAN_POINT('Ctrl Pts',(6.38723176905914,-3.22253967884565,0.229656840923317));
#64123=CARTESIAN_POINT('Ctrl Pts',(6.39990164604897,-3.2227486308868,0.0029706257346402));
#64124=CARTESIAN_POINT('Ctrl Pts',(6.39990166558323,-3.22274863120894,0.00297027623255133));
#64125=CARTESIAN_POINT('Ctrl Pts',(6.41277784774664,-3.222960960657,-0.227407097632205));
#64126=CARTESIAN_POINT('Ctrl Pts',(6.42573644257657,-3.1984720160562,-0.457120151576906));
#64127=CARTESIAN_POINT('Ctrl Pts',(6.44079109024918,-3.14530149897629,-0.702587204161363));
#64128=CARTESIAN_POINT('Ctrl Pts',(6.44204399814821,-3.14070098266663,-0.722874543574654));
#64129=CARTESIAN_POINT('Ctrl Pts',(6.44401815107632,-3.13318070024313,-0.754609697770681));
#64130=CARTESIAN_POINT('Ctrl Pts',(6.44473515966878,-3.13039379046217,-0.766088641883618));
#64131=CARTESIAN_POINT('Ctrl Pts',(6.44594696810494,-3.12559072010532,-0.78540801266658));
#64132=CARTESIAN_POINT('Ctrl Pts',(6.44644068997747,-3.12360799595938,-0.793256693429814));
#64133=CARTESIAN_POINT('Ctrl Pts',(6.44741776269864,-3.11963342914898,-0.808744179914984));
#64134=CARTESIAN_POINT('Ctrl Pts',(6.44790106332227,-3.11764304864468,-0.816383304761118));
#64135=CARTESIAN_POINT('Ctrl Pts',(6.4488300379962,-3.11377066222345,-0.831024910474995));
#64136=CARTESIAN_POINT('Ctrl Pts',(6.44927556687871,-3.11189304939165,-0.838028511765836));
#64137=CARTESIAN_POINT('Ctrl Pts',(6.45029364337235,-3.10755607600124,-0.853990099987739));
#64138=CARTESIAN_POINT('Ctrl Pts',(6.45086668019823,-3.10508159562469,-0.862943878816772));
#64139=CARTESIAN_POINT('Ctrl Pts',(6.45266129072657,-3.09722842281783,-0.890889028782707));
#64140=CARTESIAN_POINT('Ctrl Pts',(6.45388727979266,-3.09171402376146,-0.909841487326335));
#64141=CARTESIAN_POINT('Ctrl Pts',(6.46958377096014,-3.01922682830068,-1.15070216269025));
#64142=CARTESIAN_POINT('Ctrl Pts',(6.48486602613934,-2.9286907098309,-1.36476249732738));
#64143=CARTESIAN_POINT('Ctrl Pts',(6.50745821405934,-2.76585436836356,-1.65734875183981));
#64144=CARTESIAN_POINT('Ctrl Pts',(6.51446175078708,-2.71140048421781,-1.74501077904379));
#64145=CARTESIAN_POINT('Ctrl Pts',(6.53088022225938,-2.57307049723676,-1.94554895291717));
#64146=CARTESIAN_POINT('Ctrl Pts',(6.54023563212587,-2.4858180065267,-2.05586252342072));
#64147=CARTESIAN_POINT('Ctrl Pts',(6.55021057344749,-2.38047906322105,-2.1724902683892));
#64148=CARTESIAN_POINT('Ctrl Pts',(6.55126054899762,-2.36922814285503,-2.18475457927284));
#64149=CARTESIAN_POINT('Ctrl Pts',(6.55260237375811,-2.35463233100135,-2.20041970523343));
#64150=CARTESIAN_POINT('Ctrl Pts',(6.55290059229195,-2.35137446021599,-2.20390073322507));
#64151=CARTESIAN_POINT('Ctrl Pts',(6.55348289142529,-2.34498552285598,-2.21069700638276));
#64152=CARTESIAN_POINT('Ctrl Pts',(6.55376702130051,-2.3418551224516,-2.21401285960518));
#64153=CARTESIAN_POINT('Ctrl Pts',(6.5543014601919,-2.33594227210772,-2.22024943105404));
#64154=CARTESIAN_POINT('Ctrl Pts',(6.55455188114838,-2.33316140900805,-2.22317153508758));
#64155=CARTESIAN_POINT('Ctrl Pts',(6.55512453924631,-2.32677870521814,-2.22985325225507));
#64156=CARTESIAN_POINT('Ctrl Pts',(6.55544648999754,-2.32317324227626,-2.23360935638398));
#64157=CARTESIAN_POINT('Ctrl Pts',(6.55643861215128,-2.31201049711778,-2.24518222797489));
#64158=CARTESIAN_POINT('Ctrl Pts',(6.55710644347141,-2.30442265263173,-2.25296960066857));
#64159=CARTESIAN_POINT('Ctrl Pts',(6.56257968698295,-2.24164300533202,-2.31675109437592));
#64160=CARTESIAN_POINT('Ctrl Pts',(6.56723584154511,-2.18445337731023,-2.37075193363298));
#64161=CARTESIAN_POINT('Ctrl Pts',(6.57400062266901,-2.09683274350277,-2.44762092280927));
#64162=CARTESIAN_POINT('Ctrl Pts',(6.57617951410607,-2.0678849459238,-2.47212616005106));
#64163=CARTESIAN_POINT('Ctrl Pts',(6.5822332578483,-1.98568409489452,-2.53925739233174));
#64164=CARTESIAN_POINT('Ctrl Pts',(6.58607189690449,-1.93149978239982,-2.58071280100383));
#64165=CARTESIAN_POINT('Ctrl Pts',(6.59751860008124,-1.76540025308559,-2.69962863215977));
#64166=CARTESIAN_POINT('Ctrl Pts',(6.60507068768653,-1.64985595492655,-2.7717516927804));
#64167=CARTESIAN_POINT('Ctrl Pts',(6.61910560286572,-1.4317232796006,-2.88942570756378));
#64168=CARTESIAN_POINT('Ctrl Pts',(6.62552776846441,-1.33065798105164,-2.93733868755377));
#64169=CARTESIAN_POINT('Ctrl Pts',(6.63444981263702,-1.19080439043145,-2.99493931834794));
#64170=CARTESIAN_POINT('Ctrl Pts',(6.63679906609222,-1.15402284443624,-3.00930352296862));
#64171=CARTESIAN_POINT('Ctrl Pts',(6.64082664512479,-1.0911223610592,-3.032545122067));
#64172=CARTESIAN_POINT('Ctrl Pts',(6.64249344409555,-1.0651359638427,-3.04176975303239));
#64173=CARTESIAN_POINT('Ctrl Pts',(6.64467473172646,-1.03120393356188,-3.05332678392861));
#64174=CARTESIAN_POINT('Ctrl Pts',(6.64517913145368,-1.0233626877562,-3.05596381021701));
#64175=CARTESIAN_POINT('Ctrl Pts',(6.64617434143269,-1.00790225700872,-3.06109700681205));
#64176=CARTESIAN_POINT('Ctrl Pts',(6.64666508757715,-1.00028373542448,-3.06359499470874));
#64177=CARTESIAN_POINT('Ctrl Pts',(6.6475995516659,-0.985787041364879,-3.06828838281788));
#64178=CARTESIAN_POINT('Ctrl Pts',(6.64804308920575,-0.978910648088813,
-3.07048915203513));
#64179=CARTESIAN_POINT('Ctrl Pts',(6.64905388346546,-0.963250121997491,
-3.07544330251065));
#64180=CARTESIAN_POINT('Ctrl Pts',(6.64962161328873,-0.954461500116476,
-3.07818218214338));
#64181=CARTESIAN_POINT('Ctrl Pts',(6.65109382911773,-0.931691119135956,
-3.08517143375974));
#64182=CARTESIAN_POINT('Ctrl Pts',(6.65200018867653,-0.917692086100695,
-3.08936439109155));
#64183=CARTESIAN_POINT('Ctrl Pts',(6.65765262601639,-0.830515814075435,
-3.11483041108697));
#64184=CARTESIAN_POINT('Ctrl Pts',(6.66247979776866,-0.756637045949777,
-3.13359598546297));
#64185=CARTESIAN_POINT('Ctrl Pts',(6.6699678015346,-0.642994869656276,-3.15820861050688));
#64186=CARTESIAN_POINT('Ctrl Pts',(6.67257014033762,-0.603668809639296,
-3.16596079991464));
#64187=CARTESIAN_POINT('Ctrl Pts',(6.67815697430394,-0.519580394928984,
-3.18091315895159));
#64188=CARTESIAN_POINT('Ctrl Pts',(6.68114627075611,-0.474790189092412,
-3.18790625992317));
#64189=CARTESIAN_POINT('Ctrl Pts',(6.69658279853086,-0.244368222847626,
-3.21891837639952));
#64190=CARTESIAN_POINT('Ctrl Pts',(6.709352441565,-0.0570513147570352,-3.22767549083771));
#64191=CARTESIAN_POINT('Ctrl Pts',(6.73052173880749,0.257276037426847,-3.21499066527969));
#64192=CARTESIAN_POINT('Ctrl Pts',(6.73898942867085,0.384200416649385,-3.20230435455845));
#64193=CARTESIAN_POINT('Ctrl Pts',(6.7483637614936,0.529546698612316,-3.17900733851338));
#64194=CARTESIAN_POINT('Ctrl Pts',(6.74961240372288,0.549012715273,-3.17570345728896));
#64195=CARTESIAN_POINT('Ctrl Pts',(6.75127395353869,0.575076612694543,-3.17103292406748));
#64196=CARTESIAN_POINT('Ctrl Pts',(6.75169541057584,0.581701854110343,-3.16982426497883));
#64197=CARTESIAN_POINT('Ctrl Pts',(6.75239442313732,0.592714540929362,-3.16777950352941));
#64198=CARTESIAN_POINT('Ctrl Pts',(6.75267263317171,0.597104085607614,-3.16695503939359));
#64199=CARTESIAN_POINT('Ctrl Pts',(6.7532025038105,0.605476903571851,-3.1653643921128));
#64200=CARTESIAN_POINT('Ctrl Pts',(6.75345424941978,0.609460396678054,-3.16459982314387));
#64201=CARTESIAN_POINT('Ctrl Pts',(6.75403328048411,0.618635133722468,-3.16282091035401));
#64202=CARTESIAN_POINT('Ctrl Pts',(6.75436026180352,0.623825327791362,-3.16180130637613));
#64203=CARTESIAN_POINT('Ctrl Pts',(6.75523444516756,0.637725041050718,-3.15903517541197));
#64204=CARTESIAN_POINT('Ctrl Pts',(6.75578034124197,0.646429964006964,-3.15726539483563));
#64205=CARTESIAN_POINT('Ctrl Pts',(6.7596832781468,0.708835525872825,-3.14430892907404));
#64206=CARTESIAN_POINT('Ctrl Pts',(6.76296783799149,0.762253851803676,-3.13178804442739));
#64207=CARTESIAN_POINT('Ctrl Pts',(6.76682137170641,0.825565353494423,-3.11523214759048));
#64208=CARTESIAN_POINT('Ctrl Pts',(6.76744231779076,0.835787461827807,-3.11250523048514));
#64209=CARTESIAN_POINT('Ctrl Pts',(6.77440546891616,0.950613957072339,-3.08126688312451));
#64210=CARTESIAN_POINT('Ctrl Pts',(6.7805479430104,1.05373662377573,-3.04754243911072));
#64211=CARTESIAN_POINT('Ctrl Pts',(6.80253774613786,1.41936937893766,-2.90718374429777));
#64212=CARTESIAN_POINT('Ctrl Pts',(6.81809505291899,1.66920859283577,-2.77129153495518));
#64213=CARTESIAN_POINT('Ctrl Pts',(6.83740520208559,1.93109223551615,-2.58043983867366));
#64214=CARTESIAN_POINT('Ctrl Pts',(6.83986259152405,1.96365072711764,-2.55575088271706));
#64215=CARTESIAN_POINT('Ctrl Pts',(6.84310109955373,2.00551186272474,-2.52273560546881));
#64216=CARTESIAN_POINT('Ctrl Pts',(6.84386008801061,2.01524882828709,-2.51496419853156));
#64217=CARTESIAN_POINT('Ctrl Pts',(6.8451043559084,2.0310896923243,-2.50216999932124));
#64218=CARTESIAN_POINT('Ctrl Pts',(6.84558827852859,2.03722066388927,-2.497180812162));
#64219=CARTESIAN_POINT('Ctrl Pts',(6.84651768419625,2.04893802932612,-2.48757372691249));
#64220=CARTESIAN_POINT('Ctrl Pts',(6.84696301905348,2.05452732774937,-2.48295943442657));
#64221=CARTESIAN_POINT('Ctrl Pts',(6.84797959230421,2.06722843763702,-2.47240167684161));
#64222=CARTESIAN_POINT('Ctrl Pts',(6.84855131484562,2.07433024656088,-2.46644632829341));
#64223=CARTESIAN_POINT('Ctrl Pts',(6.85033775734316,2.09639162670946,-2.44778368606331));
#64224=CARTESIAN_POINT('Ctrl Pts',(6.85155683524338,2.11126064583525,-2.43497048938502));
#64225=CARTESIAN_POINT('Ctrl Pts',(6.86310869874889,2.25039316012435,-2.31284226104784));
#64226=CARTESIAN_POINT('Ctrl Pts',(6.87383972080921,2.36615976996346,-2.19426099354943));
#64227=CARTESIAN_POINT('Ctrl Pts',(6.89345434934639,2.55517831926851,-1.96821614723181));
#64228=CARTESIAN_POINT('Ctrl Pts',(6.90220502793478,2.63202073044741,-1.86420894114727));
#64229=CARTESIAN_POINT('Ctrl Pts',(6.9190178968012,2.76738879535141,-1.65586855642765));
#64230=CARTESIAN_POINT('Ctrl Pts',(6.92706745972506,2.8267704290833,-1.55232520473732));
#64231=CARTESIAN_POINT('Ctrl Pts',(6.93808400264493,2.90188431920851,-1.40267769396412));
#64232=CARTESIAN_POINT('Ctrl Pts',(6.94121813379093,2.92252412319212,-1.35915068414243));
#64233=CARTESIAN_POINT('Ctrl Pts',(6.94606776273347,2.95341931601618,-1.29003496762093));
#64234=CARTESIAN_POINT('Ctrl Pts',(6.94781571105146,2.96433487376341,-1.2647508653687));
#64235=CARTESIAN_POINT('Ctrl Pts',(6.95001384645631,2.97779726074388,-1.23243531524486));
#64236=CARTESIAN_POINT('Ctrl Pts',(6.95048137584784,2.98064516138895,-1.22553162214712));
#64237=CARTESIAN_POINT('Ctrl Pts',(6.95122746015266,2.98516546230746,-1.2144648416895));
#64238=CARTESIAN_POINT('Ctrl Pts',(6.95150693305045,2.98685319056344,-1.21030810443518));
#64239=CARTESIAN_POINT('Ctrl Pts',(6.95203772450084,2.99004822486201,-1.20239160960812));
#64240=CARTESIAN_POINT('Ctrl Pts',(6.95228913390641,2.99155710433421,-1.19863257986645));
#64241=CARTESIAN_POINT('Ctrl Pts',(6.95286543614774,2.99500556283479,-1.18999445706198));
#64242=CARTESIAN_POINT('Ctrl Pts',(6.95319003432388,2.99694030640924,-1.18511346713992));
#64243=CARTESIAN_POINT('Ctrl Pts',(6.95405371182265,3.00206761242918,-1.17208539756747));
#64244=CARTESIAN_POINT('Ctrl Pts',(6.95459153401772,3.00523896416154,-1.16392993827157));
#64245=CARTESIAN_POINT('Ctrl Pts',(6.95832550725685,3.02710271983819,-1.10701991064165));
#64246=CARTESIAN_POINT('Ctrl Pts',(6.96145605413339,3.04464228220179,-1.05782705047883));
#64247=CARTESIAN_POINT('Ctrl Pts',(6.98349153082733,3.16150106403291,-0.703043295171254));
#64248=CARTESIAN_POINT('Ctrl Pts',(7.00059796009312,3.21582939435065,-0.384516819152284));
#64249=CARTESIAN_POINT('Ctrl Pts',(7.02354659429729,3.22364935835346,0.0142683079844779));
#64250=CARTESIAN_POINT('Ctrl Pts',(7.02806554300593,3.22237493104741,0.0917457403873097));
#64251=CARTESIAN_POINT('Ctrl Pts',(7.03542064431528,3.2158795514194,0.215367132216485));
#64252=CARTESIAN_POINT('Ctrl Pts',(7.03820221362001,3.21245105132584,0.26157637574521));
#64253=CARTESIAN_POINT('Ctrl Pts',(7.0418089856256,3.20677944532132,0.320708738415351));
#64254=CARTESIAN_POINT('Ctrl Pts',(7.0426052767562,3.20545197263471,0.333715671020363));
#64255=CARTESIAN_POINT('Ctrl Pts',(7.04389192683434,3.20318632791259,0.354652893595549));
#64256=CARTESIAN_POINT('Ctrl Pts',(7.04438071788972,3.20229775473078,0.362588491946789));
#64257=CARTESIAN_POINT('Ctrl Pts',(7.04531367500036,3.20054880436754,0.377699806791281));
#64258=CARTESIAN_POINT('Ctrl Pts',(7.04575766971974,3.19969376322551,0.384876101374628));
#64259=CARTESIAN_POINT('Ctrl Pts',(7.04677260050641,3.19768752625469,0.40124541578703));
#64260=CARTESIAN_POINT('Ctrl Pts',(7.04734402415462,3.19652081597348,0.410436437748819));
#64261=CARTESIAN_POINT('Ctrl Pts',(7.04883204598333,3.19338640414859,0.434304171531368));
#64262=CARTESIAN_POINT('Ctrl Pts',(7.04975058505057,3.19135716647256,0.448972453306252));
#64263=CARTESIAN_POINT('Ctrl Pts',(7.05561540897138,3.17780321955445,0.54220840077987));
#64264=CARTESIAN_POINT('Ctrl Pts',(7.0606499344613,3.16347993881912,0.620335502024622));
#64265=CARTESIAN_POINT('Ctrl Pts',(7.06609761137538,3.14518907872737,0.702800789693252));
#64266=CARTESIAN_POINT('Ctrl Pts',(7.06642507918124,3.14407904229985,0.707750143954934));
#64267=CARTESIAN_POINT('Ctrl Pts',(7.06706438648791,3.14189139619561,0.71739755364541));
#64268=CARTESIAN_POINT('Ctrl Pts',(7.0673761926074,3.14081492151291,0.722095855055939));
#64269=CARTESIAN_POINT('Ctrl Pts',(7.07163012442392,3.12599925968216,0.786099264453137));
#64270=CARTESIAN_POINT('Ctrl Pts',(7.07561923715654,3.11059363260896,0.845002949504906));
#64271=CARTESIAN_POINT('Ctrl Pts',(7.09556025874728,3.02611840228877,1.13426272846525));
#64272=CARTESIAN_POINT('Ctrl Pts',(7.11209313398907,2.93309142370641,1.35679951334675));
#64273=CARTESIAN_POINT('Ctrl Pts',(7.1326162753722,2.78313897319671,1.62630727125358));
#64274=CARTESIAN_POINT('Ctrl Pts',(7.13708637175668,2.74821706590087,1.68464895624599));
#64275=CARTESIAN_POINT('Ctrl Pts',(7.14372720747798,2.69249894086202,1.77138350379706));
#64276=CARTESIAN_POINT('Ctrl Pts',(7.14596405582013,2.67304181216371,1.80061039075857));
#64277=CARTESIAN_POINT('Ctrl Pts',(7.14867973121104,2.64851213245526,1.83618262873122));
#64278=CARTESIAN_POINT('Ctrl Pts',(7.14918714612422,2.64388905966814,1.8428330920991));
#64279=CARTESIAN_POINT('Ctrl Pts',(7.14998176575461,2.63658571321376,1.85325517568702));
#64280=CARTESIAN_POINT('Ctrl Pts',(7.1502701053596,2.63392234437909,1.85703851703648));
#64281=CARTESIAN_POINT('Ctrl Pts',(7.15080812635734,2.62892769936669,1.86410109753713));
#64282=CARTESIAN_POINT('Ctrl Pts',(7.15105793821985,2.62659845506331,1.86738167133472));
#64283=CARTESIAN_POINT('Ctrl Pts',(7.15162357823566,2.62130146123447,1.87481258901128));
#64284=CARTESIAN_POINT('Ctrl Pts',(7.15193914589485,2.61833000322528,1.87896024163595));
#64285=CARTESIAN_POINT('Ctrl Pts',(7.15287192304153,2.60949892455134,1.89122530430338));
#64286=CARTESIAN_POINT('Ctrl Pts',(7.15348722432998,2.60361124981536,1.89932257789342));
#64287=CARTESIAN_POINT('Ctrl Pts',(7.15778551053343,2.56205281956822,1.95592118110281));
#64288=CARTESIAN_POINT('Ctrl Pts',(7.16138142958591,2.52506416323742,2.00344562829945));
#64289=CARTESIAN_POINT('Ctrl Pts',(7.18336192184959,2.28679808374598,2.29248830535901));
#64290=CARTESIAN_POINT('Ctrl Pts',(7.20013846113611,2.05240281582212,2.50452306939585));
#64291=CARTESIAN_POINT('Ctrl Pts',(7.21827755053244,1.79046916109811,2.67961529540315));
#64292=CARTESIAN_POINT('Ctrl Pts',(7.21831331056787,1.78995273479898,2.67996028989249));
#64293=CARTESIAN_POINT('Ctrl Pts',(7.21834907457188,1.78943621037019,2.68030513403157));
#64294=CARTESIAN_POINT('Origin',(-1.72497344927317,0.,0.));
#64295=CARTESIAN_POINT('',(8.71691228903198,1.78943621037803,2.68030513402633));
#64296=CARTESIAN_POINT('',(8.46829646867762,1.78943615355263,2.68030517196433));
#64297=CARTESIAN_POINT('',(-1.72497344927317,1.78943621037804,2.68030513402633));
#64298=CARTESIAN_POINT('',(7.8965734492731,-3.22274887139593,-0.00269711257784768));
#64299=CARTESIAN_POINT('Ctrl Pts',(7.8965734492731,-3.22274887139593,-0.00269711257784768));
#64300=CARTESIAN_POINT('Ctrl Pts',(7.90619705313966,-3.2226187285209,-0.158203340630839));
#64301=CARTESIAN_POINT('Ctrl Pts',(7.91582065700621,-3.21123025196946,-0.313254007322803));
#64302=CARTESIAN_POINT('Ctrl Pts',(7.92544426087277,-3.18879700715618,-0.466573905883924));
#64303=CARTESIAN_POINT('Ctrl Pts',(7.9272223412999,-3.18465218635178,-0.494901662772128));
#64304=CARTESIAN_POINT('Ctrl Pts',(7.92900042172702,-3.18013043580562,-0.523170431299474));
#64305=CARTESIAN_POINT('Ctrl Pts',(7.93077850215415,-3.17523324768117,-0.551372274711115));
#64306=CARTESIAN_POINT('Ctrl Pts',(7.93695075024691,-3.15823364541348,-0.649269294190383));
#64307=CARTESIAN_POINT('Ctrl Pts',(7.94312299833967,-3.13667242061309,-0.74655170305749));
#64308=CARTESIAN_POINT('Ctrl Pts',(7.94929524643243,-3.11060617359134,-0.842761410670567));
#64309=CARTESIAN_POINT('Ctrl Pts',(7.95545913508506,-3.08457522962746,-0.93884081579429));
#64310=CARTESIAN_POINT('Ctrl Pts',(7.96162302373769,-3.05405150327207,-1.03384999174038));
#64311=CARTESIAN_POINT('Ctrl Pts',(7.96778691239031,-3.01914293225304,-1.12733913137375));
#64312=CARTESIAN_POINT('Ctrl Pts',(7.97394427404886,-2.98427132621656,-1.22072927456257));
#64313=CARTESIAN_POINT('Ctrl Pts',(7.9801016357074,-2.94502425764515,-1.31260217674605));
#64314=CARTESIAN_POINT('Ctrl Pts',(7.98625899736594,-2.90155972324655,-1.40252227609168));
#64315=CARTESIAN_POINT('Ctrl Pts',(7.99241186151225,-2.85812693658118,-1.49237669523702));
#64316=CARTESIAN_POINT('Ctrl Pts',(7.99856472565856,-2.81048299723078,-1.58028075753251));
#64317=CARTESIAN_POINT('Ctrl Pts',(8.00471758980487,-2.75883400138122,-1.66581887230362));
#64318=CARTESIAN_POINT('Ctrl Pts',(8.0108681229414,-2.70720457273012,-1.75132458099905));
#64319=CARTESIAN_POINT('Ctrl Pts',(8.01701865607794,-2.65157332675075,-1.83446575175514));
#64320=CARTESIAN_POINT('Ctrl Pts',(8.02316918921448,-2.59219185890672,-1.91485219511004));
#64321=CARTESIAN_POINT('Ctrl Pts',(8.02931903742969,-2.5328170037633,-1.99522968665721));
#64322=CARTESIAN_POINT('Ctrl Pts',(8.03546888564489,-2.46969301514349,-2.07285271131146));
#64323=CARTESIAN_POINT('Ctrl Pts',(8.0416187338601,-2.4031136986529,-2.14736166349471));
#64324=CARTESIAN_POINT('Ctrl Pts',(8.04776954223923,-2.33652398726221,-2.22188224861678));
#64325=CARTESIAN_POINT('Ctrl Pts',(8.05392035061836,-2.26647816592401,-2.29328747162887));
#64326=CARTESIAN_POINT('Ctrl Pts',(8.06007115899749,-2.19330835886251,-2.36125305832388));
#64327=CARTESIAN_POINT('Ctrl Pts',(8.06622854536368,-2.12006030029093,-2.42929133087122));
#64328=CARTESIAN_POINT('Ctrl Pts',(8.07238593172987,-2.04368190334552,-2.49388232527394));
#64329=CARTESIAN_POINT('Ctrl Pts',(8.07854331809606,-1.96453989401621,-2.55474080237483));
#64330=CARTESIAN_POINT('Ctrl Pts',(8.08470414083302,-1.88535371638699,-2.61563324393393));
#64331=CARTESIAN_POINT('Ctrl Pts',(8.09086496356998,-1.8034012111174,-2.67278877128187));
#64332=CARTESIAN_POINT('Ctrl Pts',(8.09702578630694,-1.71907798398794,-2.72596559909841));
#64333=CARTESIAN_POINT('Ctrl Pts',(8.10319690922362,-1.63461377822112,-2.77923133239189));
#64334=CARTESIAN_POINT('Ctrl Pts',(8.10936803214031,-1.54777131145734,-2.8285048646833));
#64335=CARTESIAN_POINT('Ctrl Pts',(8.115539155057,-1.45897078394203,-2.87359040472082));
#64336=CARTESIAN_POINT('Ctrl Pts',(8.1202346770026,-1.39140369261068,-2.90789536761548));
#64337=CARTESIAN_POINT('Ctrl Pts',(8.12493019894819,-1.32270349535213,-2.93977665558864));
#64338=CARTESIAN_POINT('Ctrl Pts',(8.12962572089379,-1.25306185638666,-2.96916714695701));
#64339=CARTESIAN_POINT('Ctrl Pts',(8.13579796898656,-1.16151815192487,-3.00780085081264));
#64340=CARTESIAN_POINT('Ctrl Pts',(8.14197021707933,-1.06802494737793,-3.04226495087972));
#64341=CARTESIAN_POINT('Ctrl Pts',(8.14814246517209,-0.972998197045154,
-3.07235936554416));
#64342=CARTESIAN_POINT('Ctrl Pts',(8.15430635382472,-0.87810014705278,-3.10241302156539));
#64343=CARTESIAN_POINT('Ctrl Pts',(8.16047024247735,-0.781673089943199,
-3.12810862511497));
#64344=CARTESIAN_POINT('Ctrl Pts',(8.16663413112998,-0.68415377052273,-3.14929375904814));
#64345=CARTESIAN_POINT('Ctrl Pts',(8.17279149278853,-0.586737715138465,
-3.17045645986292));
#64346=CARTESIAN_POINT('Ctrl Pts',(8.17894885444708,-0.488232119018895,
-3.18711809484292));
#64347=CARTESIAN_POINT('Ctrl Pts',(8.18510621610563,-0.38908881109783,-3.19917605948445));
#64348=CARTESIAN_POINT('Ctrl Pts',(8.19125908025193,-0.290017920271235,
-3.21122521664536));
#64349=CARTESIAN_POINT('Ctrl Pts',(8.19741194439824,-0.190310673636845,
-3.21867733671003));
#64350=CARTESIAN_POINT('Ctrl Pts',(8.20356480854455,-0.0904281080926534,
-3.22148107549413));
#64351=CARTESIAN_POINT('Ctrl Pts',(8.20971534168108,0.00941661698724765,
-3.22428375208307));
#64352=CARTESIAN_POINT('Ctrl Pts',(8.21586587481762,0.109436095279572,-3.22244153438794));
#64353=CARTESIAN_POINT('Ctrl Pts',(8.22201640795416,0.209166055687512,-3.21595508731825));
#64354=CARTESIAN_POINT('Ctrl Pts',(8.22816625616937,0.30888491020014,-3.20946936257715));
#64355=CARTESIAN_POINT('Ctrl Pts',(8.23431610438458,0.408313877467575,-3.19834046488288));
#64356=CARTESIAN_POINT('Ctrl Pts',(8.24046595259978,0.506991590372671,-3.18262110371175));
#64357=CARTESIAN_POINT('Ctrl Pts',(8.24661676097892,0.605684709638605,-3.16689928830711));
#64358=CARTESIAN_POINT('Ctrl Pts',(8.25276756935806,0.703625912563291,-3.14658565421469));
#64359=CARTESIAN_POINT('Ctrl Pts',(8.2589183777372,0.800362833824376,-3.12178424890841));
#64360=CARTESIAN_POINT('Ctrl Pts',(8.26507576410339,0.897203210464985,-3.09695631971894));
#64361=CARTESIAN_POINT('Ctrl Pts',(8.27123315046958,0.992836312011732,-3.06763114339496));
#64362=CARTESIAN_POINT('Ctrl Pts',(8.27739053683577,1.08682390024517,-3.03396298137533));
#64363=CARTESIAN_POINT('Ctrl Pts',(8.28355135957273,1.1808639419356,-3.00027602951843));
#64364=CARTESIAN_POINT('Ctrl Pts',(8.28971218230969,1.27325623976038,-2.96224143041404));
#64365=CARTESIAN_POINT('Ctrl Pts',(8.29587300504664,1.36358349365661,-2.92006123537285));
#64366=CARTESIAN_POINT('Ctrl Pts',(8.30204412796333,1.45406176422536,-2.87781051994688));
#64367=CARTESIAN_POINT('Ctrl Pts',(8.30821525088002,1.5424677097967,-2.83140056621136));
#64368=CARTESIAN_POINT('Ctrl Pts',(8.31438637379671,1.62840942244908,-2.78107898402384));
#64369=CARTESIAN_POINT('Ctrl Pts',(8.31908189574229,1.69380128115092,-2.74278998918649));
#64370=CARTESIAN_POINT('Ctrl Pts',(8.32377741768787,1.75776700488079,-2.702237309696));
#64371=CARTESIAN_POINT('Ctrl Pts',(8.32847293963344,1.82014649547395,-2.65954588182153));
#64372=CARTESIAN_POINT('Ctrl Pts',(8.33464518772621,1.90214412988047,-2.60342814084842));
#64373=CARTESIAN_POINT('Ctrl Pts',(8.34081743581898,1.98168837106901,-2.54341591556368));
#64374=CARTESIAN_POINT('Ctrl Pts',(8.34698968391174,2.05838599785357,-2.47975092425436));
#64375=CARTESIAN_POINT('Ctrl Pts',(8.35315357256437,2.13497974851229,-2.41617215820293));
#64376=CARTESIAN_POINT('Ctrl Pts',(8.359317461217,2.20873421638767,-2.34895073414032));
#64377=CARTESIAN_POINT('Ctrl Pts',(8.36548134986963,2.27928503443018,-2.27837163218001));
#64378=CARTESIAN_POINT('Ctrl Pts',(8.37163871152817,2.34976114561178,-2.2078672670307));
#64379=CARTESIAN_POINT('Ctrl Pts',(8.37779607318672,2.41704004592167,-2.13401259811834));
#64380=CARTESIAN_POINT('Ctrl Pts',(8.38395343484526,2.48079111500584,-2.05713222866399));
#64381=CARTESIAN_POINT('Ctrl Pts',(8.39010629899157,2.54449561849438,-1.98030801482001));
#64382=CARTESIAN_POINT('Ctrl Pts',(8.39625916313787,2.60467713750001,-1.90046282777002));
#64383=CARTESIAN_POINT('Ctrl Pts',(8.40241202728418,2.66104319346577,-1.81795673353617));
#64384=CARTESIAN_POINT('Ctrl Pts',(8.40856256042071,2.71738789517699,-1.7354818966984));
#64385=CARTESIAN_POINT('Ctrl Pts',(8.41471309355725,2.76991976126253,-1.65034851400117));
#64386=CARTESIAN_POINT('Ctrl Pts',(8.42086362669379,2.81838831491438,-1.56294749395304));
#64387=CARTESIAN_POINT('Ctrl Pts',(8.427013474909,2.86685147112417,-1.47555620685351));
#64388=CARTESIAN_POINT('Ctrl Pts',(8.43316332312421,2.91125200385418,-1.38589816433056));
#64389=CARTESIAN_POINT('Ctrl Pts',(8.43931317133941,2.9513847868615,-1.29438997306936));
#64390=CARTESIAN_POINT('Ctrl Pts',(8.44546397971855,2.99152383572274,-1.20286749481093));
#64391=CARTESIAN_POINT('Ctrl Pts',(8.45161478809768,3.02739363690701,-1.1094946919004));
#64392=CARTESIAN_POINT('Ctrl Pts',(8.45776559647682,3.05883711751518,-1.01470835761388));
#64393=CARTESIAN_POINT('Ctrl Pts',(8.46392298284301,3.09031422537939,-0.91982065400463));
#64394=CARTESIAN_POINT('Ctrl Pts',(8.4700803692092,3.11735542286021,-0.82351681339229));
#64395=CARTESIAN_POINT('Ctrl Pts',(8.47623775557539,3.13985351616262,-0.72624889641308));
#64396=CARTESIAN_POINT('Ctrl Pts',(8.48239857831235,3.16236416540771,-0.628926695260844));
#64397=CARTESIAN_POINT('Ctrl Pts',(8.4885594010493,3.18032658305296,-0.530639773553441));
#64398=CARTESIAN_POINT('Ctrl Pts',(8.49472022378626,3.19368509804519,-0.431848419036193));
#64399=CARTESIAN_POINT('Ctrl Pts',(8.50089134670295,3.20706594692224,-0.332891896853729));
#64400=CARTESIAN_POINT('Ctrl Pts',(8.50706246961964,3.21582748011222,-0.233429690190807));
#64401=CARTESIAN_POINT('Ctrl Pts',(8.51323359253633,3.21996608060853,-0.133925360669872));
#64402=CARTESIAN_POINT('Ctrl Pts',(8.51792911448191,3.22311508439872,-0.0582138946606126));
#64403=CARTESIAN_POINT('Ctrl Pts',(8.52262463642749,3.22358873069806,0.0175218913677458));
#64404=CARTESIAN_POINT('Ctrl Pts',(8.52732015837307,3.22140555029293,0.0930797670919089));
#64405=CARTESIAN_POINT('Ctrl Pts',(8.53349260195626,3.21853567596613,0.192403490967159));
#64406=CARTESIAN_POINT('Ctrl Pts',(8.53966504553945,3.21106286005284,0.291769188819021));
#64407=CARTESIAN_POINT('Ctrl Pts',(8.54583748912264,3.19897781935079,0.390715336020603));
#64408=CARTESIAN_POINT('Ctrl Pts',(8.55200152301338,3.18690924400386,0.489526673295419));
#64409=CARTESIAN_POINT('Ctrl Pts',(8.55816555690411,3.17024098656387,0.587919168678262));
#64410=CARTESIAN_POINT('Ctrl Pts',(8.56432959079485,3.14901576313197,0.68543218924002));
#64411=CARTESIAN_POINT('Ctrl Pts',(8.5706872032214,3.12712397171115,0.786007559567762));
#64412=CARTESIAN_POINT('Ctrl Pts',(8.57704481564794,3.10038424253534,0.885646832468236));
#64413=CARTESIAN_POINT('Ctrl Pts',(8.58340242807449,3.06890128795359,0.983850825733655));
#64414=CARTESIAN_POINT('Ctrl Pts',(8.5895550653343,3.03843337226252,1.07888863355971));
#64415=CARTESIAN_POINT('Ctrl Pts',(8.5957077025941,3.00352353248956,1.17258184148595));
#64416=CARTESIAN_POINT('Ctrl Pts',(8.60186033985391,2.96431812219575,1.26449026604472));
#64417=CARTESIAN_POINT('Ctrl Pts',(8.60801062858697,2.92512767702192,1.35636360818526));
#64418=CARTESIAN_POINT('Ctrl Pts',(8.61416091732003,2.88164509029373,1.44645312187698));
#64419=CARTESIAN_POINT('Ctrl Pts',(8.62031120605309,2.83406528913763,1.53433747898083));
#64420=CARTESIAN_POINT('Ctrl Pts',(8.62646079228314,2.78649092267814,1.62221179769012));
#64421=CARTESIAN_POINT('Ctrl Pts',(8.63261037851319,2.73482047968976,1.70788107903586));
#64422=CARTESIAN_POINT('Ctrl Pts',(8.63875996474324,2.67929491867307,1.79094843624061));
#64423=CARTESIAN_POINT('Ctrl Pts',(8.64491049345735,2.62376084782272,1.87402852432784));
#64424=CARTESIAN_POINT('Ctrl Pts',(8.65106102217145,2.56437072741458,1.95450553560679));
#64425=CARTESIAN_POINT('Ctrl Pts',(8.65721155088556,2.50140834880026,2.03201226252509));
#64426=CARTESIAN_POINT('Ctrl Pts',(8.66336781025768,2.4383873059839,2.10959120511231));
#64427=CARTESIAN_POINT('Ctrl Pts',(8.66952406962979,2.37178763653722,2.18419400263338));
#64428=CARTESIAN_POINT('Ctrl Pts',(8.6756803290019,2.30193266163687,2.25548743818036));
#64429=CARTESIAN_POINT('Ctrl Pts',(8.6818400435129,2.23203848133186,2.32682088645363));
#64430=CARTESIAN_POINT('Ctrl Pts',(8.6879997580239,2.15888567516763,2.39484097870944));
#64431=CARTESIAN_POINT('Ctrl Pts',(8.69415947253489,2.08283216097789,2.45925349480207));
#64432=CARTESIAN_POINT('Ctrl Pts',(8.70032745329708,2.00667658402995,2.52375245159536));
#64433=CARTESIAN_POINT('Ctrl Pts',(8.70649543405928,1.92761287423558,2.58463390673216));
#64434=CARTESIAN_POINT('Ctrl Pts',(8.71266341482147,1.84602926593963,2.64164598532703));
#64435=CARTESIAN_POINT('Ctrl Pts',(8.71407970622497,1.82729604228813,2.65473709567949));
#64436=CARTESIAN_POINT('Ctrl Pts',(8.71549599762847,1.80843006291833,2.66762438097374));
#64437=CARTESIAN_POINT('Ctrl Pts',(8.71691228903198,1.78943621037803,2.68030513402633));
#64438=CARTESIAN_POINT('Ctrl Pts',(7.46680874532643,1.78773599488645,2.67780888195817));
#64439=CARTESIAN_POINT('Ctrl Pts',(7.48890051844257,1.49107844583294,2.87932143490233));
#64440=CARTESIAN_POINT('Ctrl Pts',(7.57727469780527,0.178346421750044,3.49141846844679));
#64441=CARTESIAN_POINT('Ctrl Pts',(7.72052921189373,-2.37587491464765,2.8569912360958));
#64442=CARTESIAN_POINT('Ctrl Pts',(7.84169195286606,-3.21676692519514,0.884675566243836));
#64443=CARTESIAN_POINT('Ctrl Pts',(7.89657228759183,-3.22473260027238,-0.00267998977119858));
#64444=CARTESIAN_POINT('Ctrl Pts',(7.21834907457188,1.78943621037019,2.68030513403157));
#64445=CARTESIAN_POINT('Ctrl Pts',(7.22270752708506,1.72648891861646,2.72233026086458));
#64446=CARTESIAN_POINT('Ctrl Pts',(7.22712570793226,1.66208432132251,2.76212247942874));
#64447=CARTESIAN_POINT('Ctrl Pts',(7.23434679459875,1.55653469802985,2.8223070531524));
#64448=CARTESIAN_POINT('Ctrl Pts',(7.23709827465172,1.51624967549766,2.84415259211747));
#64449=CARTESIAN_POINT('Ctrl Pts',(7.2406712221416,1.46393554127367,2.87109385277185));
#64450=CARTESIAN_POINT('Ctrl Pts',(7.24146444832933,1.45232109917454,2.87698637423482));
#64451=CARTESIAN_POINT('Ctrl Pts',(7.242747333946,1.43353858973617,2.88637285487775));
#64452=CARTESIAN_POINT('Ctrl Pts',(7.24323544218663,1.42639263486401,2.88991093202463));
#64453=CARTESIAN_POINT('Ctrl Pts',(7.24416788331957,1.41274275071359,2.89660624724723));
#64454=CARTESIAN_POINT('Ctrl Pts',(7.24461204807172,1.4062411754839,2.89976819527053));
#64455=CARTESIAN_POINT('Ctrl Pts',(7.24562847364143,1.39136450800361,2.90694145125416));
#64456=CARTESIAN_POINT('Ctrl Pts',(7.24620122725826,1.38298263633295,2.91093847751239));
#64457=CARTESIAN_POINT('Ctrl Pts',(7.24796238515516,1.35721364019772,2.9230904042695));
#64458=CARTESIAN_POINT('Ctrl Pts',(7.24915490299827,1.339771044767,2.9311260461726));
#64459=CARTESIAN_POINT('Ctrl Pts',(7.26636363369988,1.08818779358593,3.04431331168145));
#64460=CARTESIAN_POINT('Ctrl Pts',(7.28339245695585,0.842425806593474,3.12125955627945));
#64461=CARTESIAN_POINT('Ctrl Pts',(7.31480604515554,0.385788925354882,3.20632482919754));
#64462=CARTESIAN_POINT('Ctrl Pts',(7.32897325131086,0.178154020570992,3.22453532280229));
#64463=CARTESIAN_POINT('Ctrl Pts',(7.34396457217594,-0.0560925156146685,
3.22236907424466));
#64464=CARTESIAN_POINT('Ctrl Pts',(7.34563235886566,-0.082380248798944,
3.22180421839427));
#64465=CARTESIAN_POINT('Ctrl Pts',(7.3477443166181,-0.116002420128938,3.22066995927508));
#64466=CARTESIAN_POINT('Ctrl Pts',(7.34820424156187,-0.123344945932712,
3.22039711446887));
#64467=CARTESIAN_POINT('Ctrl Pts',(7.34894106001226,-0.1351422229402,3.21991832624934));
#64468=CARTESIAN_POINT('Ctrl Pts',(7.34921883227003,-0.139597538732707,
3.219728245659));
#64469=CARTESIAN_POINT('Ctrl Pts',(7.34974839061793,-0.148106734812386,
3.21934751580332));
#64470=CARTESIAN_POINT('Ctrl Pts',(7.35000026191529,-0.152160637404317,
3.21915845726415));
#64471=CARTESIAN_POINT('Ctrl Pts',(7.35058027282254,-0.161511244223582,
3.21870467816941));
#64472=CARTESIAN_POINT('Ctrl Pts',(7.35090810714367,-0.166807692851852,
3.21843453900193));
#64473=CARTESIAN_POINT('Ctrl Pts',(7.35178606111625,-0.181021241547621,
3.21767441271638));
#64474=CARTESIAN_POINT('Ctrl Pts',(7.35233485704669,-0.18993708945039,3.21716042848042));
#64475=CARTESIAN_POINT('Ctrl Pts',(7.35629992751171,-0.254569196113896,
3.21316487132701));
#64476=CARTESIAN_POINT('Ctrl Pts',(7.35964110389463,-0.310192698922484,
3.20827295343363));
#64477=CARTESIAN_POINT('Ctrl Pts',(7.36388001593474,-0.381759299429711,
3.20009996864341));
#64478=CARTESIAN_POINT('Ctrl Pts',(7.36482855264889,-0.397839923285166,
3.19814061361746));
#64479=CARTESIAN_POINT('Ctrl Pts',(7.36758259199126,-0.444693921748337,
3.19207279257889));
#64480=CARTESIAN_POINT('Ctrl Pts',(7.36937665827904,-0.475424082876621,
3.1876407323286));
#64481=CARTESIAN_POINT('Ctrl Pts',(7.37940064766516,-0.647903425998109,
3.1602150804739));
#64482=CARTESIAN_POINT('Ctrl Pts',(7.38737871077107,-0.788061880049574,
3.1282104714415));
#64483=CARTESIAN_POINT('Ctrl Pts',(7.4087114387015,-1.15352247208885,3.01862732089911));
#64484=CARTESIAN_POINT('Ctrl Pts',(7.4221429349017,-1.3731169717395,2.92527821812058));
#64485=CARTESIAN_POINT('Ctrl Pts',(7.43772508804782,-1.59807114336533,2.79869542911663));
#64486=CARTESIAN_POINT('Ctrl Pts',(7.43895311889632,-1.61562169637333,2.78860072249558));
#64487=CARTESIAN_POINT('Ctrl Pts',(7.44076542579327,-1.64125529643807,2.7735336011334));
#64488=CARTESIAN_POINT('Ctrl Pts',(7.44134503125993,-1.64941358763059,2.76868965371863));
#64489=CARTESIAN_POINT('Ctrl Pts',(7.44237026776526,-1.66377365981172,2.76007743226706));
#64490=CARTESIAN_POINT('Ctrl Pts',(7.44281535011461,-1.66998435330849,2.75632408862421));
#64491=CARTESIAN_POINT('Ctrl Pts',(7.44368572440453,-1.68208365884651,2.74895614152154));
#64492=CARTESIAN_POINT('Ctrl Pts',(7.44411094202572,-1.68797343135774,2.74534351169583));
#64493=CARTESIAN_POINT('Ctrl Pts',(7.44513599471266,-1.70212015086395,2.73660355571567));
#64494=CARTESIAN_POINT('Ctrl Pts',(7.44573650945716,-1.71036557188482,2.73145778593083));
#64495=CARTESIAN_POINT('Ctrl Pts',(7.44794320959085,-1.74050901352501,2.71245598106358));
#64496=CARTESIAN_POINT('Ctrl Pts',(7.4495577912694,-1.76226250376938,2.69837356196476));
#64497=CARTESIAN_POINT('Ctrl Pts',(7.45182879486827,-1.79243385255415,2.6783212730013));
#64498=CARTESIAN_POINT('Ctrl Pts',(7.45247694652471,-1.80099685848298,2.67257072290762));
#64499=CARTESIAN_POINT('Ctrl Pts',(7.46932952229248,-2.02239549025275,2.52234159511696));
#64500=CARTESIAN_POINT('Ctrl Pts',(7.48654117351857,-2.21715924931966,2.35296506792326));
#64501=CARTESIAN_POINT('Ctrl Pts',(7.51666749577766,-2.51578605915985,2.02293344967028));
#64502=CARTESIAN_POINT('Ctrl Pts',(7.5294015190845,-2.6294647486432,1.87279693867572));
#64503=CARTESIAN_POINT('Ctrl Pts',(7.54301924288254,-2.74272515668253,1.69239558152509));
#64504=CARTESIAN_POINT('Ctrl Pts',(7.54460594958143,-2.75578740826049,1.67104157396195));
#64505=CARTESIAN_POINT('Ctrl Pts',(7.54663030078882,-2.77229541433005,1.64333436165265));
#64506=CARTESIAN_POINT('Ctrl Pts',(7.54708216675351,-2.77597001345854,1.63711947495283));
#64507=CARTESIAN_POINT('Ctrl Pts',(7.54780916399143,-2.78186596359057,1.62707066686433));
#64508=CARTESIAN_POINT('Ctrl Pts',(7.54808513316946,-2.78410032191038,1.62324446478614));
#64509=CARTESIAN_POINT('Ctrl Pts',(7.54861345297472,-2.78837075005443,1.61589686187077));
#64510=CARTESIAN_POINT('Ctrl Pts',(7.54886588036278,-2.79040803900595,1.61237622283212));
#64511=CARTESIAN_POINT('Ctrl Pts',(7.54945013220286,-2.79511609391671,1.60420458435597));
#64512=CARTESIAN_POINT('Ctrl Pts',(7.54978163678369,-2.79778193752195,1.59955073630183));
#64513=CARTESIAN_POINT('Ctrl Pts',(7.55085275697486,-2.80637705568191,1.58445873837941));
#64514=CARTESIAN_POINT('Ctrl Pts',(7.55158941752886,-2.81225971487244,1.57399395772257));
#64515=CARTESIAN_POINT('Ctrl Pts',(7.56110271878308,-2.88782989607416,1.43778442494053));
#64516=CARTESIAN_POINT('Ctrl Pts',(7.56937603927794,-2.94909592709333,1.30752823497906));
#64517=CARTESIAN_POINT('Ctrl Pts',(7.57974609714761,-3.01594038878124,1.13657448266298));
#64518=CARTESIAN_POINT('Ctrl Pts',(7.58197942455634,-3.02973129467388,1.09928447119959));
#64519=CARTESIAN_POINT('Ctrl Pts',(7.59357586053911,-3.09791659065456,0.903874532714543));
#64520=CARTESIAN_POINT('Ctrl Pts',(7.60283908487744,-3.14063237330092,0.741958632983487));
#64521=CARTESIAN_POINT('Ctrl Pts',(7.61754121784672,-3.18671880527437,0.488918089834536));
#64522=CARTESIAN_POINT('Ctrl Pts',(7.62276108635313,-3.19912812791481,0.399743609464253));
#64523=CARTESIAN_POINT('Ctrl Pts',(7.63115261927296,-3.21275994624103,0.258763558664508));
#64524=CARTESIAN_POINT('Ctrl Pts',(7.63424774807744,-3.21649401203621,0.207245902521712));
#64525=CARTESIAN_POINT('Ctrl Pts',(7.63820568676686,-3.2196440883069,0.142104749163024));
#64526=CARTESIAN_POINT('Ctrl Pts',(7.63903211384361,-3.22021405487645,0.128542783039022));
#64527=CARTESIAN_POINT('Ctrl Pts',(7.64035578381674,-3.22098717899455,0.106886428842214));
#64528=CARTESIAN_POINT('Ctrl Pts',(7.64085129074333,-3.22124554242144,0.0987940760160971));
#64529=CARTESIAN_POINT('Ctrl Pts',(7.64178959254758,-3.22167619797546,0.0834982463755718));
#64530=CARTESIAN_POINT('Ctrl Pts',(7.64223218538996,-3.22185483152836,0.0762949864943477));
#64531=CARTESIAN_POINT('Ctrl Pts',(7.6432337200344,-3.22220378767923,0.0600217215070409));
#64532=CARTESIAN_POINT('Ctrl Pts',(7.64379310228614,-3.2223599733766,0.0509515031461113));
#64533=CARTESIAN_POINT('Ctrl Pts',(7.64522977226866,-3.22266209169762,0.0277053106459614));
#64534=CARTESIAN_POINT('Ctrl Pts',(7.64610878618116,-3.22275278284227,0.0135289262543614));
#64535=CARTESIAN_POINT('Ctrl Pts',(7.65220990883545,-3.22273308219942,-0.0845383608562378));
#64536=CARTESIAN_POINT('Ctrl Pts',(7.6575312104897,-3.2194406456586,-0.168389637158447));
#64537=CARTESIAN_POINT('Ctrl Pts',(7.67504296064636,-3.19823618548505,-0.438724581475063));
#64538=CARTESIAN_POINT('Ctrl Pts',(7.68760645982744,-3.16734462500883,-0.623783053174723));
#64539=CARTESIAN_POINT('Ctrl Pts',(7.71400303989104,-3.06988932484729,-1.00152525256368));
#64540=CARTESIAN_POINT('Ctrl Pts',(7.72779509991838,-3.00077010396966,-1.19275638655029));
#64541=CARTESIAN_POINT('Ctrl Pts',(7.74218279297676,-2.90450098161446,-1.39660270344779));
#64542=CARTESIAN_POINT('Ctrl Pts',(7.74360945166138,-2.8946671433494,-1.4168723514056));
#64543=CARTESIAN_POINT('Ctrl Pts',(7.74547683978982,-2.88140089693966,-1.44350219663691));
#64544=CARTESIAN_POINT('Ctrl Pts',(7.74592884596621,-2.87815879463476,-1.44995574961309));
#64545=CARTESIAN_POINT('Ctrl Pts',(7.74662845224725,-2.87309205126529,-1.45995737752749));
#64546=CARTESIAN_POINT('Ctrl Pts',(7.7468769871049,-2.87128249500649,-1.46351300422069));
#64547=CARTESIAN_POINT('Ctrl Pts',(7.74735068042781,-2.86781513221406,-1.47029489790246));
#64548=CARTESIAN_POINT('Ctrl Pts',(7.74757590620517,-2.86615849890056,-1.47352169265097));
#64549=CARTESIAN_POINT('Ctrl Pts',(7.74810904511639,-2.86221805367737,-1.48116511485671));
#64550=CARTESIAN_POINT('Ctrl Pts',(7.74841665244911,-2.85992946946638,-1.4855792522561));
#64551=CARTESIAN_POINT('Ctrl Pts',(7.74932304378566,-2.85314181685436,-1.49859721131012));
#64552=CARTESIAN_POINT('Ctrl Pts',(7.74992003611143,-2.84861402411091,-1.50718611197421));
#64553=CARTESIAN_POINT('Ctrl Pts',(7.75467735501518,-2.81208203248767,-1.57573198345415));
#64554=CARTESIAN_POINT('Ctrl Pts',(7.75872544100792,-2.77822464329277,-1.63468835572986));
#64555=CARTESIAN_POINT('Ctrl Pts',(7.76911074259544,-2.68489030338494,-1.78592413821137));
#64556=CARTESIAN_POINT('Ctrl Pts',(7.77532039022041,-2.62251862462263,-1.8763156318332));
#64557=CARTESIAN_POINT('Ctrl Pts',(7.79778594579357,-2.37860363324139,-2.19381416530985));
#64558=CARTESIAN_POINT('Ctrl Pts',(7.81376844982143,-2.17122107756117,-2.39924142148023));
#64559=CARTESIAN_POINT('Ctrl Pts',(7.83221571778979,-1.92521365419544,-2.58456438404546));
#64560=CARTESIAN_POINT('Ctrl Pts',(7.83326266245454,-1.91122343905189,-2.59492690026823));
#64561=CARTESIAN_POINT('Ctrl Pts',(7.83539163323463,-1.88272327787785,-2.61568138959773));
#64562=CARTESIAN_POINT('Ctrl Pts',(7.83647384194945,-1.86820961477891,-2.62606719038239));
#64563=CARTESIAN_POINT('Ctrl Pts',(7.83811753888044,-1.84613069399354,-2.64159092821861));
#64564=CARTESIAN_POINT('Ctrl Pts',(7.83867560323731,-1.83862844166152,-2.64681820723603));
#64565=CARTESIAN_POINT('Ctrl Pts',(7.83964831225718,-1.82554208631229,-2.65585378699152));
#64566=CARTESIAN_POINT('Ctrl Pts',(7.84006240116454,-1.81996803353047,-2.65967659737022));
#64567=CARTESIAN_POINT('Ctrl Pts',(7.84092790106714,-1.8083113601468,-2.6676172029867));
#64568=CARTESIAN_POINT('Ctrl Pts',(7.84137943041316,-1.80222661083344,-2.67173179018521));
#64569=CARTESIAN_POINT('Ctrl Pts',(7.84244979749895,-1.78779463378079,-2.68141914698121));
#64570=CARTESIAN_POINT('Ctrl Pts',(7.84306931489334,-1.77943537162435,-2.68697377153767));
#64571=CARTESIAN_POINT('Ctrl Pts',(7.84512867852354,-1.75162881239101,-2.70526421333121));
#64572=CARTESIAN_POINT('Ctrl Pts',(7.84657492258486,-1.73207001980036,-2.71782842747284));
#64573=CARTESIAN_POINT('Ctrl Pts',(7.86125885491315,-1.53321556647318,-2.84255057561658));
#64574=CARTESIAN_POINT('Ctrl Pts',(7.87515985370853,-1.34346252634109,-2.93699193180482));
#64575=CARTESIAN_POINT('Ctrl Pts',(7.89891384783124,-1.01367689469022,-3.06244653104838));
#64576=CARTESIAN_POINT('Ctrl Pts',(7.90854442742319,-0.878324532900173,
-3.10397574460313));
#64577=CARTESIAN_POINT('Ctrl Pts',(7.92257474510199,-0.674750275792142,
-3.15204998618005));
#64578=CARTESIAN_POINT('Ctrl Pts',(7.92708076162079,-0.608339768478786,
-3.1655379889609));
#64579=CARTESIAN_POINT('Ctrl Pts',(7.93538218785758,-0.483244892185699,
-3.18686212858442));
#64580=CARTESIAN_POINT('Ctrl Pts',(7.93919359632799,-0.424672437409031,
-3.19519486756528));
#64581=CARTESIAN_POINT('Ctrl Pts',(7.94354923417066,-0.355997838730246,
-3.20304268251034));
#64582=CARTESIAN_POINT('Ctrl Pts',(7.94417484120883,-0.346090755795727,
-3.20412828739532));
#64583=CARTESIAN_POINT('Ctrl Pts',(7.9451162831124,-0.331113954737074,-3.20569915069122));
#64584=CARTESIAN_POINT('Ctrl Pts',(7.94543398734691,-0.326047972262028,
-3.2062183669239));
#64585=CARTESIAN_POINT('Ctrl Pts',(7.94600142585887,-0.316978200581188,
-3.20712621573901));
#64586=CARTESIAN_POINT('Ctrl Pts',(7.9462514124226,-0.312974910094125,-3.20751936074983));
#64587=CARTESIAN_POINT('Ctrl Pts',(7.94678842735814,-0.304358736245893,
-3.20834923143567));
#64588=CARTESIAN_POINT('Ctrl Pts',(7.94707531537645,-0.299745661070816,
-3.20878350321358));
#64589=CARTESIAN_POINT('Ctrl Pts',(7.94786402773044,-0.287036210177492,
-3.20995231532249));
#64590=CARTESIAN_POINT('Ctrl Pts',(7.94836469671031,-0.278937898661748,
-3.21066617770283));
#64591=CARTESIAN_POINT('Ctrl Pts',(7.95104403753049,-0.23544231261744,-3.21433448249454));
#64592=CARTESIAN_POINT('Ctrl Pts',(7.95319279001972,-0.199999078006694,
-3.21673434779658));
#64593=CARTESIAN_POINT('Ctrl Pts',(7.95944714467249,-0.0954702002396502,
-3.22207752418574));
#64594=CARTESIAN_POINT('Ctrl Pts',(7.9634786461395,-0.0263181613410355,
-3.2233843685004));
#64595=CARTESIAN_POINT('Ctrl Pts',(7.98087270299436,0.276513093002135,-3.21935971904321));
#64596=CARTESIAN_POINT('Ctrl Pts',(7.99360517135268,0.509175480666166,-3.19084444158489));
#64597=CARTESIAN_POINT('Ctrl Pts',(8.01544678785245,0.883335987896204,-3.10298522450987));
#64598=CARTESIAN_POINT('Ctrl Pts',(8.02419495284562,1.02734211337299,-3.05832618779181));
#64599=CARTESIAN_POINT('Ctrl Pts',(8.03446039186819,1.18573573371273,-2.99675212621991));
#64600=CARTESIAN_POINT('Ctrl Pts',(8.03563542747638,1.20372028013837,-2.98957354785839));
#64601=CARTESIAN_POINT('Ctrl Pts',(8.03738396599581,1.23026085342746,-2.97870149737942));
#64602=CARTESIAN_POINT('Ctrl Pts',(8.03795326127324,1.23886753363927,-2.97513220028749));
#64603=CARTESIAN_POINT('Ctrl Pts',(8.03896679114146,1.25412832149066,-2.96872565954965));
#64604=CARTESIAN_POINT('Ctrl Pts',(8.03941051899496,1.26078860947899,-2.96590322992612));
#64605=CARTESIAN_POINT('Ctrl Pts',(8.04034399781915,1.2747556767722,-2.95992885904588));
#64606=CARTESIAN_POINT('Ctrl Pts',(8.04083390651544,1.28206038835007,-2.95677223419126));
#64607=CARTESIAN_POINT('Ctrl Pts',(8.04212356929794,1.30122228321234,-2.9484073414143));
#64608=CARTESIAN_POINT('Ctrl Pts',(8.04292484281843,1.31305980335427,-2.94315463850966));
#64609=CARTESIAN_POINT('Ctrl Pts',(8.04652762976241,1.36597813536117,-2.91929020866937));
#64610=CARTESIAN_POINT('Ctrl Pts',(8.04935623574506,1.40669555042735,-2.89988946068429));
#64611=CARTESIAN_POINT('Ctrl Pts',(8.0569463639148,1.51371440293524,-2.84611356417834));
#64612=CARTESIAN_POINT('Ctrl Pts',(8.06175707318743,1.57924780534192,-2.81027910631698));
#64613=CARTESIAN_POINT('Ctrl Pts',(8.0865696889267,1.90583122703549,-2.61666731688652));
#64614=CARTESIAN_POINT('Ctrl Pts',(8.10772226585456,2.14473463461321,-2.42470856356327));
#64615=CARTESIAN_POINT('Ctrl Pts',(8.12866537074368,2.3621339315205,-2.19239962717325));
#64616=CARTESIAN_POINT('Ctrl Pts',(8.12953423746365,2.37112050556997,-2.18267734518999));
#64617=CARTESIAN_POINT('Ctrl Pts',(8.13425672408314,2.41979877218243,-2.12935847504616));
#64618=CARTESIAN_POINT('Ctrl Pts',(8.1380556964434,2.45835130896937,-2.0847310411057));
#64619=CARTESIAN_POINT('Ctrl Pts',(8.14239880609919,2.50195997198617,-2.03135742642959));
#64620=CARTESIAN_POINT('Ctrl Pts',(8.1430238032365,2.5082239172878,-2.0236179190327));
#64621=CARTESIAN_POINT('Ctrl Pts',(8.14396450901897,2.51763606645736,-2.01187775760692));
#64622=CARTESIAN_POINT('Ctrl Pts',(8.14428208274589,2.52081075441575,-2.00789855718698));
#64623=CARTESIAN_POINT('Ctrl Pts',(8.14484937945983,2.52647713959923,-2.00076160623584));
#64624=CARTESIAN_POINT('Ctrl Pts',(8.14509935420658,2.52897235580575,-1.99760670956104));
#64625=CARTESIAN_POINT('Ctrl Pts',(8.1456364456459,2.53433006029252,-1.99080641701001));
#64626=CARTESIAN_POINT('Ctrl Pts',(8.14592342159382,2.53719058263645,-1.98715952870808));
#64627=CARTESIAN_POINT('Ctrl Pts',(8.14671262186991,2.54505077302131,-1.97709390806203));
#64628=CARTESIAN_POINT('Ctrl Pts',(8.14721368847115,2.55003405928935,-1.97066234002228));
#64629=CARTESIAN_POINT('Ctrl Pts',(8.14989890865197,2.57669663283906,-1.93598039497329));
#64630=CARTESIAN_POINT('Ctrl Pts',(8.15205298719722,2.59793193104523,-1.90738972379317));
#64631=CARTESIAN_POINT('Ctrl Pts',(8.15832749232466,2.65913933760219,-1.82206241155872));
#64632=CARTESIAN_POINT('Ctrl Pts',(8.16237324929399,2.69775958907222,-1.76437749985757));
#64633=CARTESIAN_POINT('Ctrl Pts',(8.17973042986077,2.85771841028123,-1.50790778402274));
#64634=CARTESIAN_POINT('Ctrl Pts',(8.19241897208323,2.95917509220752,-1.29754939409999));
#64635=CARTESIAN_POINT('Ctrl Pts',(8.21423633109631,3.08762041836164,-0.935705033314829));
#64636=CARTESIAN_POINT('Ctrl Pts',(8.22301093996192,3.12808059903206,-0.789966183615571));
#64637=CARTESIAN_POINT('Ctrl Pts',(8.23330566319194,3.16202789838621,-0.622954609428063));
#64638=CARTESIAN_POINT('Ctrl Pts',(8.23448122518939,3.16571547391526,-0.603935748589158));
#64639=CARTESIAN_POINT('Ctrl Pts',(8.2362303982389,3.17092259661065,-0.575720675520048));
#64640=CARTESIAN_POINT('Ctrl Pts',(8.23679979717346,3.1725741302277,-0.566549022814592));
#64641=CARTESIAN_POINT('Ctrl Pts',(8.23781344390923,3.17543693747565,-0.550245534027593));
#64642=CARTESIAN_POINT('Ctrl Pts',(8.23825718455265,3.17666402775737,-0.543116511440173));
#64643=CARTESIAN_POINT('Ctrl Pts',(8.23919062140869,3.17919040083367,-0.52813754582156));
#64644=CARTESIAN_POINT('Ctrl Pts',(8.23968047509605,3.18048463359583,-0.5202868110051));
#64645=CARTESIAN_POINT('Ctrl Pts',(8.24096983736731,3.18380834860684,-0.499649455315324));
#64646=CARTESIAN_POINT('Ctrl Pts',(8.24177086409802,3.18578986035285,-0.486855354974451));
#64647=CARTESIAN_POINT('Ctrl Pts',(8.24537098411578,3.19432249874531,-0.429478595514511));
#64648=CARTESIAN_POINT('Ctrl Pts',(8.24819712074888,3.20001496834759,-0.384775207446276));
#64649=CARTESIAN_POINT('Ctrl Pts',(8.25577909867849,3.21263625367078,-0.265798766116731));
#64650=CARTESIAN_POINT('Ctrl Pts',(8.26058399714788,3.21792663024815,-0.191383023850869));
#64651=CARTESIAN_POINT('Ctrl Pts',(8.28535563960879,3.23167087840233,0.187420129541721));
#64652=CARTESIAN_POINT('Ctrl Pts',(8.30646911244158,3.19953801753341,0.491667855125711));
#64653=CARTESIAN_POINT('Ctrl Pts',(8.32732401693764,3.12220475326432,0.798816005853322));
#64654=CARTESIAN_POINT('Ctrl Pts',(8.32813348089154,3.11912625778183,0.810753309034786));
#64655=CARTESIAN_POINT('Ctrl Pts',(8.33289547681894,3.1005567195806,0.881087829253506));
#64656=CARTESIAN_POINT('Ctrl Pts',(8.33679078898704,3.08349328818076,0.939062303224461));
#64657=CARTESIAN_POINT('Ctrl Pts',(8.34123026524498,3.06170987306873,1.00605697594325));
#64658=CARTESIAN_POINT('Ctrl Pts',(8.34185935373205,3.05856669159628,1.01557263896808));
#64659=CARTESIAN_POINT('Ctrl Pts',(8.34280499636105,3.05375558950356,1.02991281945204));
#64660=CARTESIAN_POINT('Ctrl Pts',(8.34312344443103,3.05212054441772,1.03474818158688));
#64661=CARTESIAN_POINT('Ctrl Pts',(8.34369169241847,3.04917610173499,1.04338815988678));
#64662=CARTESIAN_POINT('Ctrl Pts',(8.34394174762198,3.0478710653295,1.04719421375755));
#64663=CARTESIAN_POINT('Ctrl Pts',(8.34447833247837,3.04505048285536,1.05537032025078));
#64664=CARTESIAN_POINT('Ctrl Pts',(8.34476472399109,3.04353266147634,1.05973954119427));
#64665=CARTESIAN_POINT('Ctrl Pts',(8.34555068255149,3.03933329498006,1.0717444556795));
#64666=CARTESIAN_POINT('Ctrl Pts',(8.34604910758547,3.03663236414828,1.07937340368117));
#64667=CARTESIAN_POINT('Ctrl Pts',(8.34869554778818,3.02209135181638,1.11995880689307));
#64668=CARTESIAN_POINT('Ctrl Pts',(8.35081450688765,3.00974289594773,1.15273232184558));
#64669=CARTESIAN_POINT('Ctrl Pts',(8.35695661735589,2.97195371437118,1.24827691267065));
#64670=CARTESIAN_POINT('Ctrl Pts',(8.36090879376775,2.94506465179451,1.31045776817446));
#64671=CARTESIAN_POINT('Ctrl Pts',(8.38223417320864,2.78716028414156,1.64615047639399));
#64672=CARTESIAN_POINT('Ctrl Pts',(8.39853242484469,2.62000650643114,1.90096299897209));
#64673=CARTESIAN_POINT('Ctrl Pts',(8.42125583970566,2.36211550142134,2.19411153584632));
#64674=CARTESIAN_POINT('Ctrl Pts',(8.42641767180924,2.30191591544548,2.25718766143644));
#64675=CARTESIAN_POINT('Ctrl Pts',(8.43261442510955,2.22827466976914,2.32833458440022));
#64676=CARTESIAN_POINT('Ctrl Pts',(8.43354026665903,2.21723662900804,2.3388483617885));
#64677=CARTESIAN_POINT('Ctrl Pts',(8.43503615047883,2.19934816541908,2.35564675256177));
#64678=CARTESIAN_POINT('Ctrl Pts',(8.43560406137452,2.19254432902844,2.36198080813105));
#64679=CARTESIAN_POINT('Ctrl Pts',(8.43661726402921,2.18038409009594,2.3732036094462));
#64680=CARTESIAN_POINT('Ctrl Pts',(8.43706205882664,2.17503839012877,2.37810389855715));
#64681=CARTESIAN_POINT('Ctrl Pts',(8.43799246817082,2.163841352113,2.38829864855058));
#64682=CARTESIAN_POINT('Ctrl Pts',(8.43847822120258,2.1579870229891,2.39358973899537));
#64683=CARTESIAN_POINT('Ctrl Pts',(8.43974516870894,2.14269600578364,2.40730792717624));
#64684=CARTESIAN_POINT('Ctrl Pts',(8.44052778648832,2.13322909022716,2.4157009895102));
#64685=CARTESIAN_POINT('Ctrl Pts',(8.4438838856222,2.09254386136987,2.45134554373438));
#64686=CARTESIAN_POINT('Ctrl Pts',(8.44647997823743,2.06085206379877,2.47804828428357));
#64687=CARTESIAN_POINT('Ctrl Pts',(8.45333417366201,1.97665070641126,2.54626176672654));
#64688=CARTESIAN_POINT('Ctrl Pts',(8.457630814468,1.92334955940649,2.58675905927182));
#64689=CARTESIAN_POINT('Ctrl Pts',(8.4640766961298,1.84263371133385,2.64421111819046));
#64690=CARTESIAN_POINT('Ctrl Pts',(8.46618101539425,1.81616623104617,2.66245952977608));
#64691=CARTESIAN_POINT('Ctrl Pts',(8.46829646867762,1.78943615355263,2.68030517196433));
#64692=CARTESIAN_POINT('Origin',(-1.72497344927317,0.,0.));
#64693=CARTESIAN_POINT('',(9.96714565479784,1.78929966408855,2.68008864808371));
#64694=CARTESIAN_POINT('',(9.72309722109888,1.78943620850078,2.68030513527963));
#64695=CARTESIAN_POINT('',(-1.72497344927317,1.78943621037804,2.68030513402633));
#64696=CARTESIAN_POINT('',(9.1465734492731,-3.22274934639606,0.00205251157118864));
#64697=CARTESIAN_POINT('Ctrl Pts',(9.14657521538943,-3.22641437747227,0.00202632845199172));
#64698=CARTESIAN_POINT('Ctrl Pts',(9.20528648803684,-3.21937259504748,-0.945983535466743));
#64699=CARTESIAN_POINT('Ctrl Pts',(9.33028016693079,-2.27611929708021,-2.97641430368825));
#64700=CARTESIAN_POINT('Ctrl Pts',(9.52155625207129,1.17754617868619,-3.6251807319632));
#64701=CARTESIAN_POINT('Ctrl Pts',(9.72040347081094,3.6862456230291,-0.969609998419201));
#64702=CARTESIAN_POINT('Ctrl Pts',(9.8689332717198,3.03086015932743,1.67926548359054));
#64703=CARTESIAN_POINT('Ctrl Pts',(9.9511806663821,2.00582045219481,2.53867724580072));
#64704=CARTESIAN_POINT('Ctrl Pts',(9.96714565479787,1.78929966408823,2.68008864808392));
#64705=CARTESIAN_POINT('Ctrl Pts',(8.71691228903198,1.78943621037803,2.68030513402633));
#64706=CARTESIAN_POINT('Ctrl Pts',(8.71999731839222,1.74806295018164,2.70792691820193));
#64707=CARTESIAN_POINT('Ctrl Pts',(8.72308234775247,1.70608288115806,2.73456856151953));
#64708=CARTESIAN_POINT('Ctrl Pts',(8.72616737711272,1.66354743586698,2.76020424808028));
#64709=CARTESIAN_POINT('Ctrl Pts',(8.73233962520549,1.57844635888673,2.81149381424136));
#64710=CARTESIAN_POINT('Ctrl Pts',(8.73851187329825,1.490821275427,2.85893428471293));
#64711=CARTESIAN_POINT('Ctrl Pts',(8.74468412139102,1.40105536769202,2.90226832308134));
#64712=CARTESIAN_POINT('Ctrl Pts',(8.75084801004365,1.31141103522761,2.94554367160221));
#64713=CARTESIAN_POINT('Ctrl Pts',(8.75701189869628,1.21963202918873,2.98472345510216));
#64714=CARTESIAN_POINT('Ctrl Pts',(8.76317578734891,1.12612890497739,3.01959455090819));
#64715=CARTESIAN_POINT('Ctrl Pts',(8.76933314900746,1.03272479201893,3.05442872141451));
#64716=CARTESIAN_POINT('Ctrl Pts',(8.77549051066601,0.937600595267945,3.08496312397248));
#64717=CARTESIAN_POINT('Ctrl Pts',(8.78164787232456,0.841188901471771,3.11103178938125));
#64718=CARTESIAN_POINT('Ctrl Pts',(8.78780073647087,0.744847629521407,3.13708141349468));
#64719=CARTESIAN_POINT('Ctrl Pts',(8.79395360061718,0.647221148303937,3.1586716726401));
#64720=CARTESIAN_POINT('Ctrl Pts',(8.80010646476349,0.548758466147658,3.17568602168591));
#64721=CARTESIAN_POINT('Ctrl Pts',(8.80625699790003,0.450333086533505,3.19269392485336));
#64722=CARTESIAN_POINT('Ctrl Pts',(8.81240753103656,0.351072563005815,3.2051292886564));
#64723=CARTESIAN_POINT('Ctrl Pts',(8.8185580641731,0.251436519468654,3.21292658477866));
#64724=CARTESIAN_POINT('Ctrl Pts',(8.82470791238831,0.151811571368268,3.22072301259662));
#64725=CARTESIAN_POINT('Ctrl Pts',(8.83085776060352,0.0518116194499468,
3.22388236570905));
#64726=CARTESIAN_POINT('Ctrl Pts',(8.83700760881872,-0.0480991672336635,
3.22239104278352));
#64727=CARTESIAN_POINT('Ctrl Pts',(8.84315841719786,-0.148025552795578,
3.22089948702061));
#64728=CARTESIAN_POINT('Ctrl Pts',(8.849309225577,-0.247862311103922,3.21475581947906));
#64729=CARTESIAN_POINT('Ctrl Pts',(8.85546003395614,-0.347146864219039,
3.20399853576166));
#64730=CARTESIAN_POINT('Ctrl Pts',(8.86161742032233,-0.446537597280619,
3.19322974765841));
#64731=CARTESIAN_POINT('Ctrl Pts',(8.86777480668852,-0.545374513179239,
3.17783753750097));
#64732=CARTESIAN_POINT('Ctrl Pts',(8.87393219305471,-0.643201858289325,
3.15791211593882));
#64733=CARTESIAN_POINT('Ctrl Pts',(8.88009301579167,-0.741083799783258,
3.13797557421427));
#64734=CARTESIAN_POINT('Ctrl Pts',(8.88625383852863,-0.837954627269075,
3.11350088915814));
#64735=CARTESIAN_POINT('Ctrl Pts',(8.89241466126559,-0.933372498500471,
3.08462855811571));
#64736=CARTESIAN_POINT('Ctrl Pts',(8.89858578418228,-1.028949897325,3.05570795589074));
#64737=CARTESIAN_POINT('Ctrl Pts',(8.90475690709897,-1.12306907804891,3.02237516665914));
#64738=CARTESIAN_POINT('Ctrl Pts',(8.91092803001566,-1.21530683639517,2.98481940088696));
#64739=CARTESIAN_POINT('Ctrl Pts',(8.91562355196123,-1.28548926905317,2.9562437389294));
#64740=CARTESIAN_POINT('Ctrl Pts',(8.92031907390679,-1.35458284365331,2.92522420355102));
#64741=CARTESIAN_POINT('Ctrl Pts',(8.92501459585236,-1.42241128634469,2.89186163136815));
#64742=CARTESIAN_POINT('Ctrl Pts',(8.93118684394513,-1.51157155029196,2.84800664039748));
#64743=CARTESIAN_POINT('Ctrl Pts',(8.93735909203789,-1.59885867678112,2.79994718722595));
#64744=CARTESIAN_POINT('Ctrl Pts',(8.94353134013065,-1.68384900158579,2.74786646370572));
#64745=CARTESIAN_POINT('Ctrl Pts',(8.94969522878329,-1.76872421897398,2.69585627618527));
#64746=CARTESIAN_POINT('Ctrl Pts',(8.95585911743592,-1.85130845041722,2.63983586828306));
#64747=CARTESIAN_POINT('Ctrl Pts',(8.96202300608855,-1.93120042371355,2.58003536525153));
#64748=CARTESIAN_POINT('Ctrl Pts',(8.96818036774709,-2.0110077987201,2.52029818548109));
#64749=CARTESIAN_POINT('Ctrl Pts',(8.97433772940562,-2.08812823751872,2.45678912733547));
#64750=CARTESIAN_POINT('Ctrl Pts',(8.98049509106415,-2.16218822125454,2.38978234539637));
#64751=CARTESIAN_POINT('Ctrl Pts',(8.98664795521046,-2.23619410947009,2.32282450711817));
#64752=CARTESIAN_POINT('Ctrl Pts',(8.99280081935677,-2.3071436659334,2.2523743150494));
#64753=CARTESIAN_POINT('Ctrl Pts',(8.99895368350307,-2.3746960684403,2.17874646185236));
#64754=CARTESIAN_POINT('Ctrl Pts',(9.00510421663961,-2.44222287875038,2.10514650253386));
#64755=CARTESIAN_POINT('Ctrl Pts',(9.01125474977615,-2.50635479905214,2.02837159385722));
#64756=CARTESIAN_POINT('Ctrl Pts',(9.01740528291268,-2.56678818299062,1.94877294371605));
#64757=CARTESIAN_POINT('Ctrl Pts',(9.02355513112789,-2.62721483708751,1.86918315765416));
#64758=CARTESIAN_POINT('Ctrl Pts',(9.0297049793431,-2.68394351101071,1.78677060126456));
#64759=CARTESIAN_POINT('Ctrl Pts',(9.0358548275583,-2.73671178223863,1.70191838331227));
#64760=CARTESIAN_POINT('Ctrl Pts',(9.04200563593743,-2.78948829207482,1.61705291754709));
#64761=CARTESIAN_POINT('Ctrl Pts',(9.04815644431656,-2.83830294163955,1.52974740255392));
#64762=CARTESIAN_POINT('Ctrl Pts',(9.05430725269569,-2.88293799314867,1.44041177798571));
#64763=CARTESIAN_POINT('Ctrl Pts',(9.06046463906188,-2.92762077965016,1.35098061336065));
#64764=CARTESIAN_POINT('Ctrl Pts',(9.06662202542807,-2.96811484769521,1.25951539302503));
#64765=CARTESIAN_POINT('Ctrl Pts',(9.07277941179426,-3.00424965263439,1.16644827881316));
#64766=CARTESIAN_POINT('Ctrl Pts',(9.07894023453122,-3.04040462401761,1.07332922485084));
#64767=CARTESIAN_POINT('Ctrl Pts',(9.08510105726818,-3.07219534907949,0.978606908438986));
#64768=CARTESIAN_POINT('Ctrl Pts',(9.09126188000514,-3.09950110681261,0.882728979567017));
#64769=CARTESIAN_POINT('Ctrl Pts',(9.09743300292183,-3.12685251659971,0.786690753939032));
#64770=CARTESIAN_POINT('Ctrl Pts',(9.10360412583852,-3.149703881888,0.689493479684278));
#64771=CARTESIAN_POINT('Ctrl Pts',(9.10977524875521,-3.16798553732232,0.591595468049439));
#64772=CARTESIAN_POINT('Ctrl Pts',(9.11447077070081,-3.18189579570684,0.517106227068816));
#64773=CARTESIAN_POINT('Ctrl Pts',(9.11916629264641,-3.19316148928379,0.442211515810729));
#64774=CARTESIAN_POINT('Ctrl Pts',(9.12386181459201,-3.2017721296376,0.367114140800825));
#64775=CARTESIAN_POINT('Ctrl Pts',(9.13143235948571,-3.21565498230386,0.246035365001745));
#64776=CARTESIAN_POINT('Ctrl Pts',(9.1390029043794,-3.22267158184634,0.124154455016588));
#64777=CARTESIAN_POINT('Ctrl Pts',(9.1465734492731,-3.22274934639606,0.00205251157118864));
#64778=CARTESIAN_POINT('',(8.90087508401166,-3.22274906885896,-0.00275535252744801));
#64779=CARTESIAN_POINT('Ctrl Pts',(8.46829646867762,1.78943615355263,2.68030517196433));
#64780=CARTESIAN_POINT('Ctrl Pts',(8.47579862762055,1.6946416754658,2.74359224390675));
#64781=CARTESIAN_POINT('Ctrl Pts',(8.48344479637332,1.59654484078101,2.80181370844835));
#64782=CARTESIAN_POINT('Ctrl Pts',(8.50195209470057,1.35386705840831,2.92894985201071));
#64783=CARTESIAN_POINT('Ctrl Pts',(8.51284534894163,1.20684476031786,2.9925294065602));
#64784=CARTESIAN_POINT('Ctrl Pts',(8.52879445311386,0.978937359159517,3.07154700259383));
#64785=CARTESIAN_POINT('Ctrl Pts',(8.53407697800821,0.901182328413188,3.09525318779629));
#64786=CARTESIAN_POINT('Ctrl Pts',(8.53989482736868,0.81200845620102,3.11879463803361));
#64787=CARTESIAN_POINT('Ctrl Pts',(8.54058342794267,0.801395218346658,3.12153863332567));
#64788=CARTESIAN_POINT('Ctrl Pts',(8.54159216788618,0.785757875946686,3.12549657372907));
#64789=CARTESIAN_POINT('Ctrl Pts',(8.54191468279844,0.780744659996072,3.1267526363276));
#64790=CARTESIAN_POINT('Ctrl Pts',(8.54248803414816,0.77180764340262,3.12896897425712));
#64791=CARTESIAN_POINT('Ctrl Pts',(8.54273914039506,0.767885040845833,3.12993393620606));
#64792=CARTESIAN_POINT('Ctrl Pts',(8.54327103542302,0.759557911930897,3.13196581692718));
#64793=CARTESIAN_POINT('Ctrl Pts',(8.54355171220243,0.755152960527299,3.13303081803977));
#64794=CARTESIAN_POINT('Ctrl Pts',(8.54429658617214,0.743434690794448,3.13583783726263));
#64795=CARTESIAN_POINT('Ctrl Pts',(8.54475985009215,0.736117444730943,3.13756357566068));
#64796=CARTESIAN_POINT('Ctrl Pts',(8.54694896760837,0.701405947062481,3.14562200541563));
#64797=CARTESIAN_POINT('Ctrl Pts',(8.54865638451767,0.673934621407378,3.1516218611702));
#64798=CARTESIAN_POINT('Ctrl Pts',(8.56494784998084,0.408430681921393,3.20597856931094));
#64799=CARTESIAN_POINT('Ctrl Pts',(8.57826032314767,0.165693583213242,3.22764541142062));
#64800=CARTESIAN_POINT('Ctrl Pts',(8.59708224166964,-0.170220816540769,
3.21959625910126));
#64801=CARTESIAN_POINT('Ctrl Pts',(8.60232269816301,-0.26309707283633,3.21334000292403));
#64802=CARTESIAN_POINT('Ctrl Pts',(8.61026033107898,-0.40083817832454,3.19804953755053));
#64803=CARTESIAN_POINT('Ctrl Pts',(8.61288901739599,-0.445994088857983,
3.19206533874573));
#64804=CARTESIAN_POINT('Ctrl Pts',(8.61601869660511,-0.499077665618734,
3.18388217956807));
#64805=CARTESIAN_POINT('Ctrl Pts',(8.61649533017392,-0.507143748292799,
3.18260733782146));
#64806=CARTESIAN_POINT('Ctrl Pts',(8.62148221528932,-0.591340166951187,
3.16897191262809));
#64807=CARTESIAN_POINT('Ctrl Pts',(8.62606392763189,-0.667003094716916,
3.1539136949829));
#64808=CARTESIAN_POINT('Ctrl Pts',(8.63162150771758,-0.756324351548435,
3.13277931512577));
#64809=CARTESIAN_POINT('Ctrl Pts',(8.63251280455146,-0.770576451799622,
3.12930418510241));
#64810=CARTESIAN_POINT('Ctrl Pts',(8.63396956607379,-0.793749191193171,
3.12348600795123));
#64811=CARTESIAN_POINT('Ctrl Pts',(8.63453312964858,-0.80268447730299,3.12120173130421));
#64812=CARTESIAN_POINT('Ctrl Pts',(8.63554022614174,-0.818599010302545,
3.11706037483392));
#64813=CARTESIAN_POINT('Ctrl Pts',(8.63598327553756,-0.825582078876997,
3.11521812233369));
#64814=CARTESIAN_POINT('Ctrl Pts',(8.63691921490108,-0.840295115951148,
3.11128362743157));
#64815=CARTESIAN_POINT('Ctrl Pts',(8.63741227681921,-0.848023586332021,
3.10918601685229));
#64816=CARTESIAN_POINT('Ctrl Pts',(8.6387191632251,-0.868448260122921,3.10356066806939));
#64817=CARTESIAN_POINT('Ctrl Pts',(8.63953458164963,-0.881130683297891,
3.09998385666104));
#64818=CARTESIAN_POINT('Ctrl Pts',(8.6432371330804,-0.938436432090628,3.083441901165));
#64819=CARTESIAN_POINT('Ctrl Pts',(8.64615308705334,-0.982796233532079,
3.06959086756475));
#64820=CARTESIAN_POINT('Ctrl Pts',(8.65405420063484,-1.10087972481441,3.0298981494575));
#64821=CARTESIAN_POINT('Ctrl Pts',(8.65909400260583,-1.17398544258651,3.00232834996836));
#64822=CARTESIAN_POINT('Ctrl Pts',(8.67890603670013,-1.45302467700679,2.88534616579206));
#64823=CARTESIAN_POINT('Ctrl Pts',(8.69421953878989,-1.65038777242848,2.77717544333505));
#64824=CARTESIAN_POINT('Ctrl Pts',(8.71905093925936,-1.95344401973431,2.56728895159755));
#64825=CARTESIAN_POINT('Ctrl Pts',(8.72864030112209,-2.06637437228752,2.47730167892635));
#64826=CARTESIAN_POINT('Ctrl Pts',(8.73850911137816,-2.18177419710493,2.37194499658698));
#64827=CARTESIAN_POINT('Ctrl Pts',(8.73926395522007,-2.19059586220245,2.36380022277344));
#64828=CARTESIAN_POINT('Ctrl Pts',(8.74035070909394,-2.20329235956693,2.3519458132815));
#64829=CARTESIAN_POINT('Ctrl Pts',(8.740685543336,-2.20720364321955,2.34827562451455));
#64830=CARTESIAN_POINT('Ctrl Pts',(8.7412729844112,-2.21406503361762,2.3418048883254));
#64831=CARTESIAN_POINT('Ctrl Pts',(8.74152590947406,-2.2170190241985,2.33900849830813));
#64832=CARTESIAN_POINT('Ctrl Pts',(8.7420534112226,-2.22317957448665,2.33315446823612));
#64833=CARTESIAN_POINT('Ctrl Pts',(8.7423279060333,-2.22638511886519,2.33009581264913));
#64834=CARTESIAN_POINT('Ctrl Pts',(8.74288523333201,-2.23289285678557,2.32386059118233));
#64835=CARTESIAN_POINT('Ctrl Pts',(8.74316802979512,-2.23619460511071,2.32068357296242));
#64836=CARTESIAN_POINT('Ctrl Pts',(8.74434994580997,-2.2499916264596,2.30735097648105));
#64837=CARTESIAN_POINT('Ctrl Pts',(8.74524416969898,-2.26042478779632,2.29713095953601));
#64838=CARTESIAN_POINT('Ctrl Pts',(8.75306418934751,-2.35156838881662,2.20662711441993));
#64839=CARTESIAN_POINT('Ctrl Pts',(8.75968384018178,-2.42805126080892,2.12218052517605));
#64840=CARTESIAN_POINT('Ctrl Pts',(8.77127008488088,-2.55638544950768,1.96443853329002));
#64841=CARTESIAN_POINT('Ctrl Pts',(8.7762819666804,-2.60994561832455,1.89269918634697));
#64842=CARTESIAN_POINT('Ctrl Pts',(8.79552434089202,-2.80420308197538,1.60855222531929));
#64843=CARTESIAN_POINT('Ctrl Pts',(8.80970634072327,-2.9225020827472,1.38201240868437));
#64844=CARTESIAN_POINT('Ctrl Pts',(8.82535694447938,-3.0153657940286,1.13742471245656));
#64845=CARTESIAN_POINT('Ctrl Pts',(8.82577329668741,-3.01781125126521,1.13092046533894));
#64846=CARTESIAN_POINT('Ctrl Pts',(8.82789580542811,-3.03015040431871,1.09777668066512));
#64847=CARTESIAN_POINT('Ctrl Pts',(8.82961252472462,-3.03971223508363,1.07101566859724));
#64848=CARTESIAN_POINT('Ctrl Pts',(8.83202358737759,-3.0525543651526,1.03351600618123));
#64849=CARTESIAN_POINT('Ctrl Pts',(8.83270798571006,-3.05613452465505,1.02288085789969));
#64850=CARTESIAN_POINT('Ctrl Pts',(8.83381136565364,-3.06180148247826,1.0057513474394));
#64851=CARTESIAN_POINT('Ctrl Pts',(8.83422918569213,-3.06392335451921,0.999268616279226));
#64852=CARTESIAN_POINT('Ctrl Pts',(8.83509570522546,-3.06827409109658,0.985832129140286));
#64853=CARTESIAN_POINT('Ctrl Pts',(8.83554450149965,-3.07049993268714,0.978877442231301));
#64854=CARTESIAN_POINT('Ctrl Pts',(8.8365964407798,-3.07565265923587,0.962587140210561));
#64855=CARTESIAN_POINT('Ctrl Pts',(8.83720019957919,-3.0785606948493,0.953245680561477));
#64856=CARTESIAN_POINT('Ctrl Pts',(8.83915575477198,-3.08782017987653,0.923017176599575));
#64857=CARTESIAN_POINT('Ctrl Pts',(8.84051309451524,-3.09400183495431,0.902079142337461));
#64858=CARTESIAN_POINT('Ctrl Pts',(8.84369819396764,-3.10793531702774,0.853055940438917));
#64859=CARTESIAN_POINT('Ctrl Pts',(8.84553126408412,-3.11551986500512,0.824925604795923));
#64860=CARTESIAN_POINT('Ctrl Pts',(8.86445762735885,-3.18938949060584,0.535387322419601));
#64861=CARTESIAN_POINT('Ctrl Pts',(8.88264150706362,-3.22297908382601,0.266799226859869));
#64862=CARTESIAN_POINT('Ctrl Pts',(8.90087535058479,-3.22274882416508,-0.00275296978013415));
#64863=CARTESIAN_POINT('Ctrl Pts',(8.90087550980276,-3.22274882215359,-0.00275532351062157));
#64864=CARTESIAN_POINT('Ctrl Pts',(8.91224051534764,-3.2226051804775,-0.170765011173096));
#64865=CARTESIAN_POINT('Ctrl Pts',(8.92354587169548,-3.20932355738335,-0.33853059364086));
#64866=CARTESIAN_POINT('Ctrl Pts',(8.93521580475408,-3.18065427738746,-0.519406634633492));
#64867=CARTESIAN_POINT('Ctrl Pts',(8.93617153842345,-3.17818944722932,-0.534281519399871));
#64868=CARTESIAN_POINT('Ctrl Pts',(8.93757479794722,-3.17439548953985,-0.556221631992641));
#64869=CARTESIAN_POINT('Ctrl Pts',(8.93802655248072,-3.1731470110333,-0.563300343135838));
#64870=CARTESIAN_POINT('Ctrl Pts',(8.93877518056322,-3.17103276706671,-0.575057728145776));
#64871=CARTESIAN_POINT('Ctrl Pts',(8.93907278167319,-3.17018031222907,-0.579738724902492));
#64872=CARTESIAN_POINT('Ctrl Pts',(8.9396540323799,-3.16849180496538,-0.588895556064934));
#64873=CARTESIAN_POINT('Ctrl Pts',(8.93993773047647,-3.16765662785408,-0.59337153850793));
#64874=CARTESIAN_POINT('Ctrl Pts',(8.9404718161381,-3.1660634018941,-0.601810917507669));
#64875=CARTESIAN_POINT('Ctrl Pts',(8.94072231371672,-3.16530740419647,-0.605774613508901));
#64876=CARTESIAN_POINT('Ctrl Pts',(8.94129575706035,-3.16355672083868,-0.614860686567186));
#64877=CARTESIAN_POINT('Ctrl Pts',(8.94161841357336,-3.16255703966688,-0.619982065558459));
#64878=CARTESIAN_POINT('Ctrl Pts',(8.94261486241257,-3.1594245648203,-0.635825040282631));
#64879=CARTESIAN_POINT('Ctrl Pts',(8.94328628502152,-3.15724962777492,-0.646538365906115));
#64880=CARTESIAN_POINT('Ctrl Pts',(8.94886844489445,-3.13863364347941,-0.735902605545982));
#64881=CARTESIAN_POINT('Ctrl Pts',(8.95362323213689,-3.11930940579938,-0.813931849445874));
#64882=CARTESIAN_POINT('Ctrl Pts',(8.963502097128,-3.07219572738373,-0.977667298684386));
#64883=CARTESIAN_POINT('Ctrl Pts',(8.96859789207978,-3.04369043916722,-1.06309461745316));
#64884=CARTESIAN_POINT('Ctrl Pts',(8.97718317709771,-2.98927715702551,-1.20593853762057));
#64885=CARTESIAN_POINT('Ctrl Pts',(8.9806909060247,-2.9651971265437,-1.26399043265779));
#64886=CARTESIAN_POINT('Ctrl Pts',(8.98737364882772,-2.91616952070017,-1.37305975243089));
#64887=CARTESIAN_POINT('Ctrl Pts',(8.99054673292551,-2.89154103096361,-1.42419384395159));
#64888=CARTESIAN_POINT('Ctrl Pts',(9.00276854552756,-2.7920892662199,-1.61745085841725));
#64889=CARTESIAN_POINT('Ctrl Pts',(9.01193861273916,-2.70804015747543,-1.75454256784271));
#64890=CARTESIAN_POINT('Ctrl Pts',(9.02413588741151,-2.58808546656617,-1.92091501708622));
#64891=CARTESIAN_POINT('Ctrl Pts',(9.02681088604528,-2.56129498884497,-1.95649394798408));
#64892=CARTESIAN_POINT('Ctrl Pts',(9.03030404766566,-2.52574517798408,-2.0017237039221));
#64893=CARTESIAN_POINT('Ctrl Pts',(9.03109567469073,-2.51765185174411,-2.01189354505197));
#64894=CARTESIAN_POINT('Ctrl Pts',(9.03237659625531,-2.50449804783152,-2.02821857301368));
#64895=CARTESIAN_POINT('Ctrl Pts',(9.03286434829349,-2.49947581793827,-2.03440450384066));
#64896=CARTESIAN_POINT('Ctrl Pts',(9.03379652246052,-2.48985215096608,-2.04616864358906));
#64897=CARTESIAN_POINT('Ctrl Pts',(9.03424077812246,-2.48525477296027,-2.05175012216357));
#64898=CARTESIAN_POINT('Ctrl Pts',(9.03525799416341,-2.47470345625165,-2.06447252541605));
#64899=CARTESIAN_POINT('Ctrl Pts',(9.03583145009875,-2.46873734307671,-2.07160322759412));
#64900=CARTESIAN_POINT('Ctrl Pts',(9.03759687789056,-2.45031637426936,-2.09342739292402));
#64901=CARTESIAN_POINT('Ctrl Pts',(9.03879299236848,-2.43776075092453,-2.10803488556374));
#64902=CARTESIAN_POINT('Ctrl Pts',(9.05586602196239,-2.25750943097432,-2.31397933176139));
#64903=CARTESIAN_POINT('Ctrl Pts',(9.07273631454037,-2.06789827110646,-2.48487293425201));
#64904=CARTESIAN_POINT('Ctrl Pts',(9.10065334617837,-1.73076510456206,-2.72317873296563));
#64905=CARTESIAN_POINT('Ctrl Pts',(9.11143511507569,-1.59472751437499,-2.80501315475837));
#64906=CARTESIAN_POINT('Ctrl Pts',(9.12512728749325,-1.40913016953806,-2.89877718813971));
#64907=CARTESIAN_POINT('Ctrl Pts',(9.12834357305445,-1.36453698370567,-2.92003362905785));
#64908=CARTESIAN_POINT('Ctrl Pts',(9.13329989218605,-1.29397457197227,-2.95169922486625));
#64909=CARTESIAN_POINT('Ctrl Pts',(9.13507425458027,-1.26832997059556,-2.96280909260864));
#64910=CARTESIAN_POINT('Ctrl Pts',(9.13729991857155,-1.2356292731601,-2.97647341814763));
#64911=CARTESIAN_POINT('Ctrl Pts',(9.1377690926105,-1.22870532632373,-2.97933833818105));
#64912=CARTESIAN_POINT('Ctrl Pts',(9.13851934174205,-1.21758306089822,-2.98389502807778));
#64913=CARTESIAN_POINT('Ctrl Pts',(9.13880133447235,-1.2133911120123,-2.98560212665149));
#64914=CARTESIAN_POINT('Ctrl Pts',(9.13933405370763,-1.20544995654027,-2.98881653717928));
#64915=CARTESIAN_POINT('Ctrl Pts',(9.13958488256228,-1.20170155650504,-2.9903256110171));
#64916=CARTESIAN_POINT('Ctrl Pts',(9.1401561478938,-1.19314340157343,-2.99375236053776));
#64917=CARTESIAN_POINT('Ctrl Pts',(9.14047630733692,-1.18833186480008,-2.99566549416561));
#64918=CARTESIAN_POINT('Ctrl Pts',(9.14147525414747,-1.17327239592296,-3.00161135545591));
#64919=CARTESIAN_POINT('Ctrl Pts',(9.14215161585377,-1.16300825742728,-3.00560320827811));
#64920=CARTESIAN_POINT('Ctrl Pts',(9.14788766440358,-1.07540582415381,-3.03915694671186));
#64921=CARTESIAN_POINT('Ctrl Pts',(9.15278168804475,-0.996967814978466,
-3.06578382271361));
#64922=CARTESIAN_POINT('Ctrl Pts',(9.16686966593601,-0.763743074814681,
-3.13505485880144));
#64923=CARTESIAN_POINT('Ctrl Pts',(9.17577891644022,-0.606693655685152,
-3.1691958176426));
#64924=CARTESIAN_POINT('Ctrl Pts',(9.19793182318241,-0.214292285908086,
-3.22424712106936));
#64925=CARTESIAN_POINT('Ctrl Pts',(9.21122842923173,0.0220131353451677,
-3.23128224789386));
#64926=CARTESIAN_POINT('Ctrl Pts',(9.22680682806551,0.279721004876056,-3.21066896726612));
#64927=CARTESIAN_POINT('Ctrl Pts',(9.22819023182167,0.302464112998689,-3.20860631379817));
#64928=CARTESIAN_POINT('Ctrl Pts',(9.23018820073404,0.335096371752607,-3.20529675243454));
#64929=CARTESIAN_POINT('Ctrl Pts',(9.23079660292102,0.345004999948714,-3.20424537075899));
#64930=CARTESIAN_POINT('Ctrl Pts',(9.23185525135656,0.36219660348664,-3.20234054269281));
#64931=CARTESIAN_POINT('Ctrl Pts',(9.23230482977598,0.369481875210079,-3.20150815607772));
#64932=CARTESIAN_POINT('Ctrl Pts',(9.23317135436664,0.383493411875749,-3.19985878991128));
#64933=CARTESIAN_POINT('Ctrl Pts',(9.23358818332162,0.390220072232276,-3.19904544613428));
#64934=CARTESIAN_POINT('Ctrl Pts',(9.23468224203442,0.40784024945324,-3.19685852813553));
#64935=CARTESIAN_POINT('Ctrl Pts',(9.23536055872445,0.418729329706685,-3.1954504943188));
#64936=CARTESIAN_POINT('Ctrl Pts',(9.23771202446459,0.456353415744524,-3.19038982312557));
#64937=CARTESIAN_POINT('Ctrl Pts',(9.23939400886271,0.483049024088982,-3.18645715999095));
#64938=CARTESIAN_POINT('Ctrl Pts',(9.24164246422415,0.51844063841155,-3.18078848381864));
#64939=CARTESIAN_POINT('Ctrl Pts',(9.24219944087821,0.527183924948733,-3.17935106289005));
#64940=CARTESIAN_POINT('Ctrl Pts',(9.25891251672479,0.788826771570012,-3.13522729858176));
#64941=CARTESIAN_POINT('Ctrl Pts',(9.27606973854272,1.03568860024296,-3.06254739481556));
#64942=CARTESIAN_POINT('Ctrl Pts',(9.30618997581978,1.44460000158168,-2.88700974242692));
#64943=CARTESIAN_POINT('Ctrl Pts',(9.31897241823912,1.61107388810878,-2.79752558416033));
#64944=CARTESIAN_POINT('Ctrl Pts',(9.33263140044182,1.78966634581512,-2.68026798232784));
#64945=CARTESIAN_POINT('Ctrl Pts',(9.33421565278191,1.81039709216274,-2.66630916186032));
#64946=CARTESIAN_POINT('Ctrl Pts',(9.33623615299508,1.83688604780093,-2.64802171331546));
#64947=CARTESIAN_POINT('Ctrl Pts',(9.3366865740106,1.84279434496339,-2.64391345382737));
#64948=CARTESIAN_POINT('Ctrl Pts',(9.33741388889364,1.85234085162141,-2.63722786456178));
#64949=CARTESIAN_POINT('Ctrl Pts',(9.33769160498529,1.8559875196805,-2.63466274266243));
#64950=CARTESIAN_POINT('Ctrl Pts',(9.33822112365766,1.86294361389825,-2.6297481107604));
#64951=CARTESIAN_POINT('Ctrl Pts',(9.33847301118517,1.86625391508573,-2.62739992372382));
#64952=CARTESIAN_POINT('Ctrl Pts',(9.33905314923752,1.87388097487463,-2.62196792475276));
#64953=CARTESIAN_POINT('Ctrl Pts',(9.33938109403584,1.87819458808512,-2.61887968350456));
#64954=CARTESIAN_POINT('Ctrl Pts',(9.34025953676007,1.8897541368965,-2.61056061576621));
#64955=CARTESIAN_POINT('Ctrl Pts',(9.34080870865557,1.89698603654271,-2.60531023259536));
#64956=CARTESIAN_POINT('Ctrl Pts',(9.34478188790707,1.94933636742768,-2.56697017301981));
#64957=CARTESIAN_POINT('Ctrl Pts',(9.34813045205917,1.99361129656449,-2.53273824835489));
#64958=CARTESIAN_POINT('Ctrl Pts',(9.37013789024603,2.28343370469918,-2.29634496191581));
#64959=CARTESIAN_POINT('Ctrl Pts',(9.38708912513479,2.49879953537757,-2.05993196855712));
#64960=CARTESIAN_POINT('Ctrl Pts',(9.40982523295586,2.71892855776573,-1.7318957997226));
#64961=CARTESIAN_POINT('Ctrl Pts',(9.41431388588081,2.75949098806638,-1.66650645985457));
#64962=CARTESIAN_POINT('Ctrl Pts',(9.42162387105256,2.8205549434693,-1.5597154418363));
#64963=CARTESIAN_POINT('Ctrl Pts',(9.42439147636278,2.84257451167856,-1.51921435807367));
#64964=CARTESIAN_POINT('Ctrl Pts',(9.42798255387318,2.8697034942563,-1.46665938338225));
#64965=CARTESIAN_POINT('Ctrl Pts',(9.42877742659947,2.87561935197151,-1.45502619445156));
#64966=CARTESIAN_POINT('Ctrl Pts',(9.43006233452078,2.88503827499106,-1.4362226131326));
#64967=CARTESIAN_POINT('Ctrl Pts',(9.4305508095628,2.88858569315519,-1.42907450264978));
#64968=CARTESIAN_POINT('Ctrl Pts',(9.43148352719014,2.89529570289232,-1.4154266506862));
#64969=CARTESIAN_POINT('Ctrl Pts',(9.43192759991667,2.89846305138215,-1.40892929172338));
#64970=CARTESIAN_POINT('Ctrl Pts',(9.4329432191861,2.9056444767612,-1.39407092941752));
#64971=CARTESIAN_POINT('Ctrl Pts',(9.43351525571424,2.90964435925304,-1.38570317217162));
#64972=CARTESIAN_POINT('Ctrl Pts',(9.4350059047907,2.91995040821661,-1.36390154049367));
#64973=CARTESIAN_POINT('Ctrl Pts',(9.43592646952617,2.9261999471462,-1.35044128197498));
#64974=CARTESIAN_POINT('Ctrl Pts',(9.44182600409199,2.96551508401014,-1.26420995249721));
#64975=CARTESIAN_POINT('Ctrl Pts',(9.44689440918493,2.99595413964917,-1.19027874119255));
#64976=CARTESIAN_POINT('Ctrl Pts',(9.45232646143493,3.02509565988156,-1.11127503054821));
#64977=CARTESIAN_POINT('Ctrl Pts',(9.45260328141914,3.02657139333901,-1.10724954084855));
#64978=CARTESIAN_POINT('Ctrl Pts',(9.45320921850452,3.02978126913138,-1.09843931317509));
#64979=CARTESIAN_POINT('Ctrl Pts',(9.45353843293577,3.03151211723777,-1.09365339395287));
#64980=CARTESIAN_POINT('Ctrl Pts',(9.45780945528202,3.05379719549257,-1.03157416258614));
#64981=CARTESIAN_POINT('Ctrl Pts',(9.46179819635579,3.07273457301046,-0.973716650350957));
#64982=CARTESIAN_POINT('Ctrl Pts',(9.47139175739874,3.11391114044204,-0.83471511462636));
#64983=CARTESIAN_POINT('Ctrl Pts',(9.47702893715218,3.13463338340288,-0.753169448658125));
#64984=CARTESIAN_POINT('Ctrl Pts',(9.49348833839362,3.18543560395888,-0.514485094867738));
#64985=CARTESIAN_POINT('Ctrl Pts',(9.50439107007879,3.20703993925166,-0.355797007696331));
#64986=CARTESIAN_POINT('Ctrl Pts',(9.519356838288,3.22074719636618,-0.131014046475662));
#64987=CARTESIAN_POINT('Ctrl Pts',(9.52364321072553,3.22274014830239,-0.0657591063378676));
#64988=CARTESIAN_POINT('Ctrl Pts',(9.5300427223429,3.22275509668956,0.0336522451780141));
#64989=CARTESIAN_POINT('Ctrl Pts',(9.53221674279805,3.2222178393868,0.067788702774648));
#64990=CARTESIAN_POINT('Ctrl Pts',(9.53486660012739,3.22088440998653,0.109934569285275));
#64991=CARTESIAN_POINT('Ctrl Pts',(9.53536943133128,3.22060060609335,0.117956480589242));
#64992=CARTESIAN_POINT('Ctrl Pts',(9.53615848086697,3.22010659777117,0.13058453245184));
#64993=CARTESIAN_POINT('Ctrl Pts',(9.53644580820198,3.21991647691811,0.1351913585726));
#64994=CARTESIAN_POINT('Ctrl Pts',(9.53698294629936,3.21954184550008,0.143819584395547));
#64995=CARTESIAN_POINT('Ctrl Pts',(9.53723288311561,3.2193596888457,0.147841001910388));
#64996=CARTESIAN_POINT('Ctrl Pts',(9.5378001113901,3.21892844877052,0.156982418848073));
#64997=CARTESIAN_POINT('Ctrl Pts',(9.53811713643678,3.21867468516704,0.162102159335523));
#64998=CARTESIAN_POINT('Ctrl Pts',(9.5390793551515,3.21786567718921,0.177672652391502));
#64999=CARTESIAN_POINT('Ctrl Pts',(9.53972240837416,3.21727173462848,0.18812145135249));
#65000=CARTESIAN_POINT('Ctrl Pts',(9.5445067231819,3.2124541016798,0.266163126042912));
#65001=CARTESIAN_POINT('Ctrl Pts',(9.54853756729726,3.20615125333803,0.333616286835064));
#65002=CARTESIAN_POINT('Ctrl Pts',(9.57048108520218,3.15942202685472,0.706414661652402));
#65003=CARTESIAN_POINT('Ctrl Pts',(9.58695246412331,3.07751141456086,1.00495322649634));
#65004=CARTESIAN_POINT('Ctrl Pts',(9.60903085842283,2.92441801111841,1.35630144035339));
#65005=CARTESIAN_POINT('Ctrl Pts',(9.61342288661609,2.89197162552098,1.42417457591874));
#65006=CARTESIAN_POINT('Ctrl Pts',(9.62058879222815,2.83620861836092,1.53104338944347));
#65007=CARTESIAN_POINT('Ctrl Pts',(9.62331162368465,2.81438970362274,1.57079071505846));
#65008=CARTESIAN_POINT('Ctrl Pts',(9.62685234361941,2.785258219264,1.62130273620062));
#65009=CARTESIAN_POINT('Ctrl Pts',(9.62764262153349,2.77870831173117,1.63250299264775));
#65010=CARTESIAN_POINT('Ctrl Pts',(9.62892188620645,2.76802973272116,1.65051276000309));
#65011=CARTESIAN_POINT('Ctrl Pts',(9.62940933777753,2.76394309995595,1.65734713037626));
#65012=CARTESIAN_POINT('Ctrl Pts',(9.63034128794528,2.75609656990768,1.6703597117097));
#65013=CARTESIAN_POINT('Ctrl Pts',(9.63078562148982,2.75234111774853,1.6765405570258));
#65014=CARTESIAN_POINT('Ctrl Pts',(9.6318035101147,2.74370540923748,1.69064626996315));
#65015=CARTESIAN_POINT('Ctrl Pts',(9.63237756309586,2.73881158192146,1.69856271554553));
#65016=CARTESIAN_POINT('Ctrl Pts',(9.63414662535567,2.72365846178123,1.72283924120721));
#65017=CARTESIAN_POINT('Ctrl Pts',(9.63534580207198,2.71328650530564,1.73912816705631));
#65018=CARTESIAN_POINT('Ctrl Pts',(9.64576089042307,2.6223540992812,1.87914190738608));
#65019=CARTESIAN_POINT('Ctrl Pts',(9.65529088838688,2.5335377332488,1.99727085087541));
#65020=CARTESIAN_POINT('Ctrl Pts',(9.68080555917827,2.28138840766265,2.28864545183788));
#65021=CARTESIAN_POINT('Ctrl Pts',(9.69714489084295,2.10643103788596,2.45062561851598));
#65022=CARTESIAN_POINT('Ctrl Pts',(9.71637844323449,1.8740305301894,2.62235688793788));
#65023=CARTESIAN_POINT('Ctrl Pts',(9.71976084273286,1.83207611166568,2.65183770981903));
#65024=CARTESIAN_POINT('Ctrl Pts',(9.72309722109888,1.78943620850078,2.68030513527963));
#65025=CARTESIAN_POINT('Origin',(-1.72497344927317,0.,0.));
#65026=CARTESIAN_POINT('',(11.2169460942912,1.78943621037803,2.68030513402634));
#65027=CARTESIAN_POINT('',(10.9707498958509,1.78943619500353,2.68030514429072));
#65028=CARTESIAN_POINT('',(-1.72497344927317,1.78943621037804,2.68030513402633));
#65029=CARTESIAN_POINT('',(10.3965734181394,-3.22264900191168,0.00167813006824187));
#65030=CARTESIAN_POINT('Ctrl Pts',(10.3965734492731,-3.22274956332349,0.00167767645253299));
#65031=CARTESIAN_POINT('Ctrl Pts',(10.4028071609904,-3.22280237398476,-0.0997694978905451));
#65032=CARTESIAN_POINT('Ctrl Pts',(10.4090408727076,-3.21806073881439,-0.201213091985544));
#65033=CARTESIAN_POINT('Ctrl Pts',(10.4152745844248,-3.2085521348123,-0.302176704415585));
#65034=CARTESIAN_POINT('Ctrl Pts',(10.4215102145758,-3.19904060452368,-0.40317138854223));
#65035=CARTESIAN_POINT('Ctrl Pts',(10.4277458447268,-3.18475922563231,-0.503685381087188));
#65036=CARTESIAN_POINT('Ctrl Pts',(10.4339814748778,-3.16578725712547,-0.603248377637264));
#65037=CARTESIAN_POINT('Ctrl Pts',(10.440220511964,-3.14680492298318,-0.702865772007254));
#65038=CARTESIAN_POINT('Ctrl Pts',(10.4464595490503,-3.12312697832341,-0.801530726483487));
#65039=CARTESIAN_POINT('Ctrl Pts',(10.4526985861366,-3.09488341232439,-0.898784861142722));
#65040=CARTESIAN_POINT('Ctrl Pts',(10.4589468229978,-3.06659819976241,-0.996182401929993));
#65041=CARTESIAN_POINT('Ctrl Pts',(10.4651950598589,-3.03373404194455,-1.09216456804687));
#65042=CARTESIAN_POINT('Ctrl Pts',(10.4714432967201,-2.9964703228284,-1.18628966399809));
#65043=CARTESIAN_POINT('Ctrl Pts',(10.4776968263823,-2.9591750380959,-1.28049449210534));
#65044=CARTESIAN_POINT('Ctrl Pts',(10.4839503560444,-2.91747294016046,-1.3728387366443));
#65045=CARTESIAN_POINT('Ctrl Pts',(10.4902038857066,-2.87159005554164,-1.46290400075138));
#65046=CARTESIAN_POINT('Ctrl Pts',(10.4964685379496,-2.82562556323518,-1.55312945570087));
#65047=CARTESIAN_POINT('Ctrl Pts',(10.5027331901926,-2.77546564344743,-1.64106747487174));
#65048=CARTESIAN_POINT('Ctrl Pts',(10.5089978424356,-2.72138049366528,-1.72632724916168));
#65049=CARTESIAN_POINT('Ctrl Pts',(10.5112626768803,-2.70182730772331,-1.75715087129783));
#65050=CARTESIAN_POINT('Ctrl Pts',(10.5135275113249,-2.68176147800805,-1.78762475090533));
#65051=CARTESIAN_POINT('Ctrl Pts',(10.5157923457695,-2.66119704885975,-1.81773150647729));
#65052=CARTESIAN_POINT('Ctrl Pts',(10.5219645938623,-2.60515376547963,-1.89978004874445));
#65053=CARTESIAN_POINT('Ctrl Pts',(10.5281368419551,-2.54521377229132,-1.97937873407576));
#65054=CARTESIAN_POINT('Ctrl Pts',(10.5343090900478,-2.48161843053037,-2.05613412202414));
#65055=CARTESIAN_POINT('Ctrl Pts',(10.5404729787005,-2.41810921969672,-2.13278555561742));
#65056=CARTESIAN_POINT('Ctrl Pts',(10.5466368673531,-2.35095477495504,-2.20660101426971));
#65057=CARTESIAN_POINT('Ctrl Pts',(10.5528007560057,-2.28043974554222,-2.27721587238701));
#65058=CARTESIAN_POINT('Ctrl Pts',(10.5589581176643,-2.20999938509354,-2.34775595583071));
#65059=CARTESIAN_POINT('Ctrl Pts',(10.5651154793228,-2.1362058199504,-2.41510187100397));
#65060=CARTESIAN_POINT('Ctrl Pts',(10.5712728409814,-2.05938335307498,-2.47892270302598));
#65061=CARTESIAN_POINT('Ctrl Pts',(10.5774257051277,-1.98261699951621,-2.54269691849556));
#65062=CARTESIAN_POINT('Ctrl Pts',(10.583578569274,-1.90282647595889,-2.6029508932634));
#65063=CARTESIAN_POINT('Ctrl Pts',(10.5897314334203,-1.8203715827754,-2.65939182203822));
#65064=CARTESIAN_POINT('Ctrl Pts',(10.5958819665568,-1.73794792759052,-2.71581136819297));
#65065=CARTESIAN_POINT('Ctrl Pts',(10.6020324996934,-1.65286226648796,-2.76842049362427));
#65066=CARTESIAN_POINT('Ctrl Pts',(10.6081830328299,-1.5655052804415,-2.81696836677478));
#65067=CARTESIAN_POINT('Ctrl Pts',(10.6143328810451,-1.47815802244004,-2.86551083365024));
#65068=CARTESIAN_POINT('Ctrl Pts',(10.6204827292603,-1.3885403220472,-2.90999273639795));
#65069=CARTESIAN_POINT('Ctrl Pts',(10.6266325774755,-1.29706859957037,-2.95020857067912));
#65070=CARTESIAN_POINT('Ctrl Pts',(10.6327833858547,-1.20558259579014,-2.99043068378084));
#65071=CARTESIAN_POINT('Ctrl Pts',(10.6389341942338,-1.11224239265235,-3.02638523062204));
#65072=CARTESIAN_POINT('Ctrl Pts',(10.6450850026129,-1.01748464066806,-3.05791474186325));
#65073=CARTESIAN_POINT('Ctrl Pts',(10.6512423889791,-0.922625549928435,
-3.08947797236604));
#65074=CARTESIAN_POINT('Ctrl Pts',(10.6573997753453,-0.826346296011019,
-3.11660657983079));
#65075=CARTESIAN_POINT('Ctrl Pts',(10.6635571617115,-0.729098842059141,
-3.13919296014247));
#65076=CARTESIAN_POINT('Ctrl Pts',(10.6697179844484,-0.631797115354364,
-3.16179194566886));
#65077=CARTESIAN_POINT('Ctrl Pts',(10.6758788071854,-0.533526539772602,
-3.1798435772076));
#65078=CARTESIAN_POINT('Ctrl Pts',(10.6820396299224,-0.434747352333379,
-3.19329176589599));
#65079=CARTESIAN_POINT('Ctrl Pts',(10.6882107528391,-0.335803017570888,
-3.20676243839319));
#65080=CARTESIAN_POINT('Ctrl Pts',(10.6943818757557,-0.23634880528944,-3.21561425614854));
#65081=CARTESIAN_POINT('Ctrl Pts',(10.7005529986724,-0.136848273637104,
-3.21984318135256));
#65082=CARTESIAN_POINT('Ctrl Pts',(10.705248520618,-0.0611396973734168,
-3.22306091196168));
#65083=CARTESIAN_POINT('Ctrl Pts',(10.7099440425636,0.0145956274916145,
-3.22360330825906));
#65084=CARTESIAN_POINT('Ctrl Pts',(10.7146395645092,0.0901554538964496,
-3.22148871744613));
#65085=CARTESIAN_POINT('Ctrl Pts',(10.7208118126019,0.18947859620559,-3.21870909480496));
#65086=CARTESIAN_POINT('Ctrl Pts',(10.7269840606947,0.288847887914431,-3.21132686240753));
#65087=CARTESIAN_POINT('Ctrl Pts',(10.7331563087875,0.3878018569203,-3.19933231819847));
#65088=CARTESIAN_POINT('Ctrl Pts',(10.7393201974401,0.486621806721703,-3.18735401890903));
#65089=CARTESIAN_POINT('Ctrl Pts',(10.7454840860928,0.585027124420842,-3.17077587567332));
#65090=CARTESIAN_POINT('Ctrl Pts',(10.7516479747454,0.682557170960763,-3.14964018117468));
#65091=CARTESIAN_POINT('Ctrl Pts',(10.7578053364039,0.779983942105353,-3.1285268674426));
#65092=CARTESIAN_POINT('Ctrl Pts',(10.7639626980625,0.876536862540032,-3.10286568854105));
#65093=CARTESIAN_POINT('Ctrl Pts',(10.770120059721,0.971762209784996,-3.07275052194834));
#65094=CARTESIAN_POINT('Ctrl Pts',(10.7762729238673,1.06691800172549,-3.04265735233062));
#65095=CARTESIAN_POINT('Ctrl Pts',(10.7824257880136,1.16074773549109,-3.00811679376037));
#65096=CARTESIAN_POINT('Ctrl Pts',(10.78857865216,1.25281055291525,-2.96927319069906));
#65097=CARTESIAN_POINT('Ctrl Pts',(10.7947291852965,1.3448384923831,-2.93044430351902));
#65098=CARTESIAN_POINT('Ctrl Pts',(10.800879718433,1.43510044582828,-2.88731577973072));
#65099=CARTESIAN_POINT('Ctrl Pts',(10.8070302515696,1.52317416630603,-2.84008063646051));
#65100=CARTESIAN_POINT('Ctrl Pts',(10.8131800997848,1.61123807892349,-2.79285075328018));
#65101=CARTESIAN_POINT('Ctrl Pts',(10.819329948,1.69711386024882,-2.74151536512039));
#65102=CARTESIAN_POINT('Ctrl Pts',(10.8254797962152,1.7804034754763,-2.68631365015553));
#65103=CARTESIAN_POINT('Ctrl Pts',(10.8316306045943,1.86370609455052,-2.63110331665354));
#65104=CARTESIAN_POINT('Ctrl Pts',(10.8377814129734,1.94442138342291,-2.57202569734984));
#65105=CARTESIAN_POINT('Ctrl Pts',(10.8439322213526,2.02218077607909,-2.50936296126251));
#65106=CARTESIAN_POINT('Ctrl Pts',(10.8500896077188,2.10002332858144,-2.44663321046075));
#65107=CARTESIAN_POINT('Ctrl Pts',(10.8562469940849,2.17490333342493,-2.38031095965062));
#65108=CARTESIAN_POINT('Ctrl Pts',(10.8624043804511,2.24648589196946,-2.31071822161037));
#65109=CARTESIAN_POINT('Ctrl Pts',(10.8685652031881,2.3181083999661,-2.24108664461532));
#65110=CARTESIAN_POINT('Ctrl Pts',(10.874726025925,2.38642949976062,-2.16818126244611));
#65111=CARTESIAN_POINT('Ctrl Pts',(10.880886848662,2.45115315403284,-2.09235890276379));
#65112=CARTESIAN_POINT('Ctrl Pts',(10.8870579715787,2.51598501873414,-2.01640977690659));
#65113=CARTESIAN_POINT('Ctrl Pts',(10.8932290944954,2.57720715764875,-1.93753427548303));
#65114=CARTESIAN_POINT('Ctrl Pts',(10.8994002174121,2.63456552349819,-1.85612016445453));
#65115=CARTESIAN_POINT('Ctrl Pts',(10.9040957393577,2.67820870955119,-1.79417329511235));
#65116=CARTESIAN_POINT('Ctrl Pts',(10.9087912613032,2.71961584377549,-1.73075734395263));
#65117=CARTESIAN_POINT('Ctrl Pts',(10.9134867832488,2.75869300294346,-1.66605236352607));
#65118=CARTESIAN_POINT('Ctrl Pts',(10.9196590313416,2.81005979963616,-1.58099788041255));
#65119=CARTESIAN_POINT('Ctrl Pts',(10.9258312794343,2.85757979342656,-1.49341589779036));
#65120=CARTESIAN_POINT('Ctrl Pts',(10.9320035275271,2.90099530016819,-1.40368936410521));
#65121=CARTESIAN_POINT('Ctrl Pts',(10.9381674161797,2.94435200672493,-1.31408435236384));
#65122=CARTESIAN_POINT('Ctrl Pts',(10.9443313048324,2.98361508772724,-1.2223409501225));
#65123=CARTESIAN_POINT('Ctrl Pts',(10.950495193485,3.01857104790268,-1.12886951914901));
#65124=CARTESIAN_POINT('Ctrl Pts',(10.9566525551436,3.05348999291475,-1.03549706586832));
#65125=CARTESIAN_POINT('Ctrl Pts',(10.9628099168021,3.08411073317958,-0.940400626330777));
#65126=CARTESIAN_POINT('Ctrl Pts',(10.9689672784607,3.1102669068782,-0.844012636444691));
#65127=CARTESIAN_POINT('Ctrl Pts',(10.975120142607,3.13640397536295,-0.747695051090338));
#65128=CARTESIAN_POINT('Ctrl Pts',(10.9812730067533,3.15808284738326,-0.650088208949003));
#65129=CARTESIAN_POINT('Ctrl Pts',(10.9874258708996,3.17518657026213,-0.551641012368562));
#65130=CARTESIAN_POINT('Ctrl Pts',(10.9935764040361,3.19228381340342,-0.453231112463453));
#65131=CARTESIAN_POINT('Ctrl Pts',(10.9997269371727,3.20480927717755,-0.353981918203898));
#65132=CARTESIAN_POINT('Ctrl Pts',(11.0058774703092,3.21269701606526,-0.254352993820366));
#65133=CARTESIAN_POINT('Ctrl Pts',(11.0120273185245,3.22058387657698,-0.154735164080839));
#65134=CARTESIAN_POINT('Ctrl Pts',(11.0181771667397,3.22383400470857,-0.0547381213100465));
#65135=CARTESIAN_POINT('Ctrl Pts',(11.0243270149549,3.22243337777737,0.0451739779774047));
#65136=CARTESIAN_POINT('Ctrl Pts',(11.030477823334,3.221032532169,0.145101676347971));
#65137=CARTESIAN_POINT('Ctrl Pts',(11.0366286317132,3.21497949533838,0.244943970519831));
#65138=CARTESIAN_POINT('Ctrl Pts',(11.0427794400923,3.20431234296101,0.344238247799028));
#65139=CARTESIAN_POINT('Ctrl Pts',(11.0489368264585,3.19363378258881,0.443638715424195));
#65140=CARTESIAN_POINT('Ctrl Pts',(11.0550942128247,3.17833129933227,0.542489563089042));
#65141=CARTESIAN_POINT('Ctrl Pts',(11.0612515991909,3.15849469008713,0.640334955465823));
#65142=CARTESIAN_POINT('Ctrl Pts',(11.0674124219278,3.1386470102448,0.738234954298347));
#65143=CARTESIAN_POINT('Ctrl Pts',(11.0735732446648,3.11426027108816,0.83512795910089));
#65144=CARTESIAN_POINT('Ctrl Pts',(11.0797340674017,3.08547456881628,0.930572000270806));
#65145=CARTESIAN_POINT('Ctrl Pts',(11.0859051903184,3.05664074019508,1.02617561278701));
#65146=CARTESIAN_POINT('Ctrl Pts',(11.0920763132351,3.02339340266776,1.12032501302636));
#65147=CARTESIAN_POINT('Ctrl Pts',(11.0982474361518,2.98592138245298,1.21259682512783));
#65148=CARTESIAN_POINT('Ctrl Pts',(11.1029429580973,2.95740944132999,1.2828051688165));
#65149=CARTESIAN_POINT('Ctrl Pts',(11.1076384800429,2.92645263936735,1.35192687335538));
#65150=CARTESIAN_POINT('Ctrl Pts',(11.1123340019885,2.89315165312483,1.41978557343038));
#65151=CARTESIAN_POINT('Ctrl Pts',(11.1185060393616,2.8493791111084,1.50898256533272));
#65152=CARTESIAN_POINT('Ctrl Pts',(11.1246780767348,2.80140069572558,1.59631036494504));
#65153=CARTESIAN_POINT('Ctrl Pts',(11.1308501141079,2.74939919461041,1.68134518501575));
#65154=CARTESIAN_POINT('Ctrl Pts',(11.1370141305733,2.69746527235467,1.76626949758132));
#65155=CARTESIAN_POINT('Ctrl Pts',(11.1431781470386,2.64151887807904,1.8489063846602));
#65156=CARTESIAN_POINT('Ctrl Pts',(11.1493421635039,2.58178978586484,1.9288543397841));
#65157=CARTESIAN_POINT('Ctrl Pts',(11.1554989370549,2.52213087722364,2.00870835353142));
#65158=CARTESIAN_POINT('Ctrl Pts',(11.1616557106059,2.45869837090181,2.08587937444902));
#65159=CARTESIAN_POINT('Ctrl Pts',(11.1678124841569,2.39176600122626,2.1599937402405));
#65160=CARTESIAN_POINT('Ctrl Pts',(11.1739650205478,2.32487969515251,2.23405709970052));
#65161=CARTESIAN_POINT('Ctrl Pts',(11.1801175569387,2.25449860285767,2.30506766354026));
#65162=CARTESIAN_POINT('Ctrl Pts',(11.1862700933296,2.180937051948,2.37268437385598));
#65163=CARTESIAN_POINT('Ctrl Pts',(11.1924205778935,2.1074000332913,2.44027853448071));
#65164=CARTESIAN_POINT('Ctrl Pts',(11.1985710624573,2.03068498090266,2.50448079474425));
#65165=CARTESIAN_POINT('Ctrl Pts',(11.2047215470212,1.95114281282732,2.56498719030959));
#65166=CARTESIAN_POINT('Ctrl Pts',(11.2087963961112,1.8984441469199,2.60507418318789));
#65167=CARTESIAN_POINT('Ctrl Pts',(11.2128712452012,1.84450530305379,2.64353968249036));
#65168=CARTESIAN_POINT('Ctrl Pts',(11.2169460942912,1.78943621037803,2.68030513402633));
#65169=CARTESIAN_POINT('Ctrl Pts',(9.96714565479787,1.78929966408823,2.68008864808392));
#65170=CARTESIAN_POINT('Ctrl Pts',(10.0174630726286,1.1068834492758,3.12577995893357));
#65171=CARTESIAN_POINT('Ctrl Pts',(10.134062896706,-0.878469227045605,3.57370670682763));
#65172=CARTESIAN_POINT('Ctrl Pts',(10.2772050334654,-2.93845908265942,1.93904361562529));
#65173=CARTESIAN_POINT('Ctrl Pts',(10.370029752394,-3.22029997028472,0.433048261942794));
#65174=CARTESIAN_POINT('Ctrl Pts',(10.3965720650762,-3.21827862215745,0.00169784412032958));
#65175=CARTESIAN_POINT('Ctrl Pts',(9.72309722109888,1.78943620850078,2.68030513527963));
#65176=CARTESIAN_POINT('Ctrl Pts',(9.7242170283104,1.7751247408481,2.68985981548279));
#65177=CARTESIAN_POINT('Ctrl Pts',(9.72533164044246,1.76073605209593,2.69930033597531));
#65178=CARTESIAN_POINT('Ctrl Pts',(9.72871374303097,1.71661506552156,2.7277454696974));
#65179=CARTESIAN_POINT('Ctrl Pts',(9.73096215783177,1.68664511362727,2.74637782173567));
#65180=CARTESIAN_POINT('Ctrl Pts',(9.73368993023612,1.64941476940892,2.76868457807351));
#65181=CARTESIAN_POINT('Ctrl Pts',(9.73419817379337,1.64243999751583,2.77282784037055));
#65182=CARTESIAN_POINT('Ctrl Pts',(9.73499380012874,1.6314603398369,2.77929418300549));
#65183=CARTESIAN_POINT('Ctrl Pts',(9.73528232250075,1.6274660254918,2.78163501068398));
#65184=CARTESIAN_POINT('Ctrl Pts',(9.73582050426074,1.61999135292766,2.78599385566529));
#65185=CARTESIAN_POINT('Ctrl Pts',(9.73607029491332,1.61651229760799,2.78801394173177));
#65186=CARTESIAN_POINT('Ctrl Pts',(9.73663565439229,1.60861597043393,2.7925791324879));
#65187=CARTESIAN_POINT('Ctrl Pts',(9.73695096377379,1.60419644835263,2.79512026708795));
#65188=CARTESIAN_POINT('Ctrl Pts',(9.73788227665554,1.59109718297368,2.80261077389247));
#65189=CARTESIAN_POINT('Ctrl Pts',(9.73849638086095,1.58240033436922,2.80753033528512));
#65190=CARTESIAN_POINT('Ctrl Pts',(9.74276796523527,1.52150554517015,2.84160394762827));
#65191=CARTESIAN_POINT('Ctrl Pts',(9.74633960102522,1.46852418426929,2.86934311564922));
#65192=CARTESIAN_POINT('Ctrl Pts',(9.75058938439789,1.40346964295228,2.90112900219003));
#65193=CARTESIAN_POINT('Ctrl Pts',(9.75132662156438,1.39210894695473,2.90659753211927));
#65194=CARTESIAN_POINT('Ctrl Pts',(9.76981632473928,1.10539376941059,3.04254272970068));
#65195=CARTESIAN_POINT('Ctrl Pts',(9.78613082430114,0.812935778881522,3.13338987824595));
#65196=CARTESIAN_POINT('Ctrl Pts',(9.80799496037242,0.438341017266595,3.19367310124625));
#65197=CARTESIAN_POINT('Ctrl Pts',(9.81235558095486,0.364250191463403,3.202969146157));
#65198=CARTESIAN_POINT('Ctrl Pts',(9.81947459180323,0.2449983516337,3.21374028439948));
#65199=CARTESIAN_POINT('Ctrl Pts',(9.82218279112177,0.20001127873527,3.21685342973216));
#65200=CARTESIAN_POINT('Ctrl Pts',(9.82570704234468,0.14204055902889,3.21964434965233));
#65201=CARTESIAN_POINT('Ctrl Pts',(9.82649580296943,0.129102300021097,3.22018910114445));
#65202=CARTESIAN_POINT('Ctrl Pts',(9.82777320426698,0.108209008553722,3.22094267155724));
#65203=CARTESIAN_POINT('Ctrl Pts',(9.82826031796067,0.100255784043493,3.22120003398721));
#65204=CARTESIAN_POINT('Ctrl Pts',(9.82919201756163,0.0850709966132224,
3.22163511507204));
#65205=CARTESIAN_POINT('Ctrl Pts',(9.82963644001139,0.077839619679537,3.22181794665359));
#65206=CARTESIAN_POINT('Ctrl Pts',(9.83065509138243,0.0612921126182172,
3.22218057562408));
#65207=CARTESIAN_POINT('Ctrl Pts',(9.83122982086193,0.0519757279983785,
3.2223443183149));
#65208=CARTESIAN_POINT('Ctrl Pts',(9.83300300638038,0.0232943657432221,
3.22272400054317));
#65209=CARTESIAN_POINT('Ctrl Pts',(9.8342056581021,0.00392832252921362,
3.22280578891355));
#65210=CARTESIAN_POINT('Ctrl Pts',(9.84481509158386,-0.16612887688819,3.22199120692338));
#65211=CARTESIAN_POINT('Ctrl Pts',(9.85454958421465,-0.316562037210817,
3.21070131167907));
#65212=CARTESIAN_POINT('Ctrl Pts',(9.87998875949124,-0.696358851500265,
3.15524482243257));
#65213=CARTESIAN_POINT('Ctrl Pts',(9.89600695041051,-0.922722733447225,
3.09662011878858));
#65214=CARTESIAN_POINT('Ctrl Pts',(9.91615920122354,-1.2057548975785,2.98949836462194));
#65215=CARTESIAN_POINT('Ctrl Pts',(9.92073187157282,-1.26993080403929,2.96280651262359));
#65216=CARTESIAN_POINT('Ctrl Pts',(9.92750682114723,-1.36564500857909,2.91931524183972));
#65217=CARTESIAN_POINT('Ctrl Pts',(9.92977820623368,-1.39784724941572,2.90403359031089));
#65218=CARTESIAN_POINT('Ctrl Pts',(9.93252998454896,-1.43708442503564,2.88460953153163));
#65219=CARTESIAN_POINT('Ctrl Pts',(9.93303986006551,-1.44436432053156,2.88097127841597));
#65220=CARTESIAN_POINT('Ctrl Pts',(9.93383746880248,-1.45576893942671,2.87521752985387));
#65221=CARTESIAN_POINT('Ctrl Pts',(9.93412635090912,-1.45990295175398,2.87312067638743));
#65222=CARTESIAN_POINT('Ctrl Pts',(9.93466485027207,-1.4676157879915,2.86918762727532));
#65223=CARTESIAN_POINT('Ctrl Pts',(9.93491460035531,-1.47119566029323,2.86735367038217));
#65224=CARTESIAN_POINT('Ctrl Pts',(9.93547941308754,-1.4792976736869,2.86318386769925));
#65225=CARTESIAN_POINT('Ctrl Pts',(9.93579421834005,-1.48381770832149,2.86084401478782));
#65226=CARTESIAN_POINT('Ctrl Pts',(9.93672267622904,-1.49716055424297,2.8538967931669));
#65227=CARTESIAN_POINT('Ctrl Pts',(9.93733444687229,-1.5059676840556,2.84925919703602));
#65228=CARTESIAN_POINT('Ctrl Pts',(9.94154927397929,-1.56673762903177,2.81689890129026));
#65229=CARTESIAN_POINT('Ctrl Pts',(9.94506906754459,-1.61795726223066,2.7877951050235));
#65230=CARTESIAN_POINT('Ctrl Pts',(9.9601105285728,-1.83708548414832,2.65520770474694));
#65231=CARTESIAN_POINT('Ctrl Pts',(9.97100128985003,-1.99610579756827,2.53783131175034));
#65232=CARTESIAN_POINT('Ctrl Pts',(9.99470044078522,-2.3123985528551,2.25613407300244));
#65233=CARTESIAN_POINT('Ctrl Pts',(10.0075163036593,-2.46504196299989,2.08827099512459));
#65234=CARTESIAN_POINT('Ctrl Pts',(10.0224614780322,-2.61158264873225,1.88844326831934));
#65235=CARTESIAN_POINT('Ctrl Pts',(10.0237676669307,-2.62415093308953,1.87093927063035));
#65236=CARTESIAN_POINT('Ctrl Pts',(10.0256736052011,-2.64213905263031,1.84534915377964));
#65237=CARTESIAN_POINT('Ctrl Pts',(10.026267958528,-2.64769945929229,1.8373621969502));
#65238=CARTESIAN_POINT('Ctrl Pts',(10.0273101924407,-2.657363804548,1.82334537947321));
#65239=CARTESIAN_POINT('Ctrl Pts',(10.0277574637398,-2.66148362753223,1.81732651484466));
#65240=CARTESIAN_POINT('Ctrl Pts',(10.0286254025381,-2.66942463159479,1.80564016909386));
#65241=CARTESIAN_POINT('Ctrl Pts',(10.0290459729667,-2.67324828726924,1.7999744102273));
#65242=CARTESIAN_POINT('Ctrl Pts',(10.0301633898312,-2.68334292216137,1.78491342092498));
#65243=CARTESIAN_POINT('Ctrl Pts',(10.0308614140203,-2.68958253735429,1.77549737472506));
#65244=CARTESIAN_POINT('Ctrl Pts',(10.0333497530227,-2.71158951157577,1.74190498787643));
#65245=CARTESIAN_POINT('Ctrl Pts',(10.035150325361,-2.72708106450095,1.71755042030322));
#65246=CARTESIAN_POINT('Ctrl Pts',(10.0373655062192,-2.74560927301591,1.68753913862809));
#65247=CARTESIAN_POINT('Ctrl Pts',(10.0377685601623,-2.74895924693956,1.68207659819142));
#65248=CARTESIAN_POINT('Ctrl Pts',(10.0540903884395,-2.88375849933772,1.46079179042319));
#65249=CARTESIAN_POINT('Ctrl Pts',(10.0709790884471,-2.98935975393753,1.23030711642551));
#65250=CARTESIAN_POINT('Ctrl Pts',(10.1019689068757,-3.13000161150293,0.79457011166922));
#65251=CARTESIAN_POINT('Ctrl Pts',(10.1158968899463,-3.17425201923646,0.593628257732955));
#65252=CARTESIAN_POINT('Ctrl Pts',(10.1298458127443,-3.20088609811125,0.375056110129359));
#65253=CARTESIAN_POINT('Ctrl Pts',(10.1307831431634,-3.20258342439748,0.360275351213151));
#65254=CARTESIAN_POINT('Ctrl Pts',(10.1320853574264,-3.20481250574597,0.339601762408255));
#65255=CARTESIAN_POINT('Ctrl Pts',(10.1324549312643,-3.20543045259679,0.333718697269679));
#65256=CARTESIAN_POINT('Ctrl Pts',(10.1330821623206,-3.20645425034305,0.323706528123644));
#65257=CARTESIAN_POINT('Ctrl Pts',(10.1333402819942,-3.20686833023153,0.319578298871961));
#65258=CARTESIAN_POINT('Ctrl Pts',(10.1338317752187,-3.20764298779661,0.311702104883322));
#65259=CARTESIAN_POINT('Ctrl Pts',(10.1340652291919,-3.20800496984906,0.307954303625351));
#65260=CARTESIAN_POINT('Ctrl Pts',(10.1346144597447,-3.20884245598749,0.299121609191988));
#65261=CARTESIAN_POINT('Ctrl Pts',(10.134929925151,-3.20931244464507,0.294036184726138));
#65262=CARTESIAN_POINT('Ctrl Pts',(10.1358613281048,-3.21066724024816,0.278986562221429));
#65263=CARTESIAN_POINT('Ctrl Pts',(10.1364753760229,-3.21151775507444,0.269019226943299));
#65264=CARTESIAN_POINT('Ctrl Pts',(10.1423322201904,-3.21921784167636,0.1735343665046));
#65265=CARTESIAN_POINT('Ctrl Pts',(10.1473964818277,-3.22269714196437,0.0877708669080378));
#65266=CARTESIAN_POINT('Ctrl Pts',(10.1614615971817,-3.22284531126189,-0.155513546596334));
#65267=CARTESIAN_POINT('Ctrl Pts',(10.1702053842559,-3.21139874199951,-0.312795122825867));
#65268=CARTESIAN_POINT('Ctrl Pts',(10.182884821753,-3.17842100158645,-0.537177319232002));
#65269=CARTESIAN_POINT('Ctrl Pts',(10.1867660237474,-3.16613619377615,-0.605393121046213));
#65270=CARTESIAN_POINT('Ctrl Pts',(10.2003368748682,-3.11597686409796,-0.84023413326679));
#65271=CARTESIAN_POINT('Ctrl Pts',(10.2101985353254,-3.06706809071662,-1.00418451432855));
#65272=CARTESIAN_POINT('Ctrl Pts',(10.2217039401308,-2.99828820939168,-1.18185183055689));
#65273=CARTESIAN_POINT('Ctrl Pts',(10.2228995794535,-2.99100524156142,-1.20016396972577));
#65274=CARTESIAN_POINT('Ctrl Pts',(10.2246667940159,-2.98004514245773,-1.22700232058778));
#65275=CARTESIAN_POINT('Ctrl Pts',(10.2252339572216,-2.97649829017663,-1.23558151149479));
#65276=CARTESIAN_POINT('Ctrl Pts',(10.2262463041613,-2.97011554517664,-1.2508332321287));
#65277=CARTESIAN_POINT('Ctrl Pts',(10.2266909939114,-2.96729409999333,-1.25751176896197));
#65278=CARTESIAN_POINT('Ctrl Pts',(10.227621671401,-2.96135238791694,-1.27144483211296));
#65279=CARTESIAN_POINT('Ctrl Pts',(10.2281077993873,-2.95822794719211,-1.2786975159146));
#65280=CARTESIAN_POINT('Ctrl Pts',(10.2293767979458,-2.95001784100771,-1.29756427620765));
#65281=CARTESIAN_POINT('Ctrl Pts',(10.2301611004046,-2.94489027682285,-1.30915986924683));
#65282=CARTESIAN_POINT('Ctrl Pts',(10.2335850374336,-2.92227564295642,-1.3594959542296));
#65283=CARTESIAN_POINT('Ctrl Pts',(10.2362485701396,-2.90409220539152,-1.3979171530288));
#65284=CARTESIAN_POINT('Ctrl Pts',(10.2432997457529,-2.85444537153338,-1.49766798205524));
#65285=CARTESIAN_POINT('Ctrl Pts',(10.2477284009941,-2.82176639780071,-1.55836485655799));
#65286=CARTESIAN_POINT('Ctrl Pts',(10.2648409901199,-2.68987320655635,-1.78556926750999));
#65287=CARTESIAN_POINT('Ctrl Pts',(10.2779381718605,-2.57766739839873,-1.94403971976498));
#65288=CARTESIAN_POINT('Ctrl Pts',(10.303865643101,-2.32903098828973,-2.23552968987077));
#65289=CARTESIAN_POINT('Ctrl Pts',(10.3166378124708,-2.19366101476323,-2.36851166465479));
#65290=CARTESIAN_POINT('Ctrl Pts',(10.3293401042552,-2.0382951890375,-2.49631902173543));
#65291=CARTESIAN_POINT('Ctrl Pts',(10.3300795223942,-2.02916974372735,-2.50374241828974));
#65292=CARTESIAN_POINT('Ctrl Pts',(10.3311481740507,-2.01585921023581,-2.51444974075624));
#65293=CARTESIAN_POINT('Ctrl Pts',(10.3314801992703,-2.01170644514313,-2.51777342781664));
#65294=CARTESIAN_POINT('Ctrl Pts',(10.3320643936386,-2.00436886839051,-2.52361635176553));
#65295=CARTESIAN_POINT('Ctrl Pts',(10.3323168699729,-2.00118750110262,-2.52613986897755));
#65296=CARTESIAN_POINT('Ctrl Pts',(10.3328452126039,-1.99450843883459,-2.53141728427047));
#65297=CARTESIAN_POINT('Ctrl Pts',(10.3331209905702,-1.99100981332341,-2.53416994369122));
#65298=CARTESIAN_POINT('Ctrl Pts',(10.3338484512345,-1.98174864253183,-2.5414254587406));
#65299=CARTESIAN_POINT('Ctrl Pts',(10.3342992594775,-1.97597641376645,-2.54591599610226));
#65300=CARTESIAN_POINT('Ctrl Pts',(10.3363433829882,-1.94965550341923,-2.5662490542001));
#65301=CARTESIAN_POINT('Ctrl Pts',(10.3379210977266,-1.92893054594401,-2.58186324951926));
#65302=CARTESIAN_POINT('Ctrl Pts',(10.3516667065893,-1.74501523835665,-2.71697425225623));
#65303=CARTESIAN_POINT('Ctrl Pts',(10.3629371012686,-1.57107655501851,-2.82112898772703));
#65304=CARTESIAN_POINT('Ctrl Pts',(10.3877311799588,-1.1706688430331,-3.01229440063833));
#65305=CARTESIAN_POINT('Ctrl Pts',(10.4012327373334,-0.941875378491943,
-3.09147790260617));
#65306=CARTESIAN_POINT('Ctrl Pts',(10.4161281187374,-0.698899990141334,
-3.14606348481142));
#65307=CARTESIAN_POINT('Ctrl Pts',(10.4165886969103,-0.691394335867417,
-3.1477214802931));
#65308=CARTESIAN_POINT('Ctrl Pts',(10.4187360982335,-0.656435764466007,
-3.15531274465253));
#65309=CARTESIAN_POINT('Ctrl Pts',(10.4204330798588,-0.628912608161079,
-3.16091367875017));
#65310=CARTESIAN_POINT('Ctrl Pts',(10.422820768766,-0.590350840207027,-3.16823738374792));
#65311=CARTESIAN_POINT('Ctrl Pts',(10.4235017853887,-0.579370628540423,
-3.17026369631467));
#65312=CARTESIAN_POINT('Ctrl Pts',(10.4246011302531,-0.561676403519434,
-3.17343403335881));
#65313=CARTESIAN_POINT('Ctrl Pts',(10.4250183130926,-0.554968841715986,
-3.17461391825002));
#65314=CARTESIAN_POINT('Ctrl Pts',(10.4258846115094,-0.541055336556297,
-3.17701591187964));
#65315=CARTESIAN_POINT('Ctrl Pts',(10.4263338273917,-0.533848881150081,
-3.17823478557589));
#65316=CARTESIAN_POINT('Ctrl Pts',(10.4273886769716,-0.516946642286728,
-3.18103446045096));
#65317=CARTESIAN_POINT('Ctrl Pts',(10.4279949365267,-0.507247693449419,
-3.18259545710934));
#65318=CARTESIAN_POINT('Ctrl Pts',(10.4299667277611,-0.475754086150861,
-3.18751657392744));
#65319=CARTESIAN_POINT('Ctrl Pts',(10.4313379322094,-0.453932408916524,
-3.19069728879393));
#65320=CARTESIAN_POINT('Ctrl Pts',(10.4345604543195,-0.402842076917451,
-3.19760947292065));
#65321=CARTESIAN_POINT('Ctrl Pts',(10.4364172527804,-0.373551789251474,
-3.20116338975306));
#65322=CARTESIAN_POINT('Ctrl Pts',(10.4429590063349,-0.270892359774016,
-3.2121913901471));
#65323=CARTESIAN_POINT('Ctrl Pts',(10.4477080674907,-0.197323449741024,
-3.21754848855274));
#65324=CARTESIAN_POINT('Ctrl Pts',(10.4720769771105,0.175468752340868,-3.23186110226117));
#65325=CARTESIAN_POINT('Ctrl Pts',(10.4928047832428,0.474662806166883,-3.20161979873633));
#65326=CARTESIAN_POINT('Ctrl Pts',(10.5177168547732,0.841170418536165,-3.11201549386957));
#65327=CARTESIAN_POINT('Ctrl Pts',(10.5227843773255,0.916288802256226,-3.09073214964787));
#65328=CARTESIAN_POINT('Ctrl Pts',(10.5283920864336,1.00089395866206,-3.06340441741788));
#65329=CARTESIAN_POINT('Ctrl Pts',(10.5290737534882,1.01120444271738,-3.06001649082249));
#65330=CARTESIAN_POINT('Ctrl Pts',(10.5300777557858,1.02643207013185,-3.0549274679298));
#65331=CARTESIAN_POINT('Ctrl Pts',(10.5304023975709,1.03136239318668,-3.0532664875073));
#65332=CARTESIAN_POINT('Ctrl Pts',(10.5309774650425,1.04010791172096,-3.05029660243918));
#65333=CARTESIAN_POINT('Ctrl Pts',(10.5312281709373,1.04392468599982,-3.04899246989969));
#65334=CARTESIAN_POINT('Ctrl Pts',(10.5317615417091,1.05205360617127,-3.04619789041504));
#65335=CARTESIAN_POINT('Ctrl Pts',(10.5320440858951,1.05636502373971,-3.04470545620776));
#65336=CARTESIAN_POINT('Ctrl Pts',(10.5328087734813,1.06804731944303,-3.04063372799684));
#65337=CARTESIAN_POINT('Ctrl Pts',(10.5332898756308,1.0754120738229,-3.03803677049178));
#65338=CARTESIAN_POINT('Ctrl Pts',(10.5356972953418,1.11233460981676,-3.02486606916646));
#65339=CARTESIAN_POINT('Ctrl Pts',(10.5376004270362,1.1417474393168,-3.01388718749809));
#65340=CARTESIAN_POINT('Ctrl Pts',(10.5429528616661,1.22492045291542,-2.98144890046001));
#65341=CARTESIAN_POINT('Ctrl Pts',(10.5463511199705,1.27827149882508,-2.95896780277302));
#65342=CARTESIAN_POINT('Ctrl Pts',(10.5586066870712,1.47113673242454,-2.87150728269124));
#65343=CARTESIAN_POINT('Ctrl Pts',(10.5671623297528,1.60655966041255,-2.79799384641693));
#65344=CARTESIAN_POINT('Ctrl Pts',(10.589531218879,1.94372765879357,-2.58238432939216));
#65345=CARTESIAN_POINT('Ctrl Pts',(10.6034021450438,2.13530823631491,-2.42635973749053));
#65346=CARTESIAN_POINT('Ctrl Pts',(10.6194523721098,2.3208319350965,-2.23612063388472));
#65347=CARTESIAN_POINT('Ctrl Pts',(10.6206333251522,2.33429365170153,-2.22206423898009));
#65348=CARTESIAN_POINT('Ctrl Pts',(10.622388995463,2.35402353745781,-2.20108562353435));
#65349=CARTESIAN_POINT('Ctrl Pts',(10.6229594545618,2.36039043564438,-2.19425653137055));
#65350=CARTESIAN_POINT('Ctrl Pts',(10.6239742975914,2.37163895355098,-2.18208583659073));
#65351=CARTESIAN_POINT('Ctrl Pts',(10.624418170063,2.3765324474879,-2.17675525701232));
#65352=CARTESIAN_POINT('Ctrl Pts',(10.625351182649,2.38676293509036,-2.16553536602062));
#65353=CARTESIAN_POINT('Ctrl Pts',(10.6258404776851,2.39209617223901,-2.15964270905134));
#65354=CARTESIAN_POINT('Ctrl Pts',(10.627126787901,2.40603281485262,-2.14412924859541));
#65355=CARTESIAN_POINT('Ctrl Pts',(10.627925308176,2.41460025327575,-2.13447645803894));
#65356=CARTESIAN_POINT('Ctrl Pts',(10.6314984553164,2.45255988323372,-2.09118696136463));
#65357=CARTESIAN_POINT('Ctrl Pts',(10.6342996304876,2.48130766314658,-2.05699412870558));
#65358=CARTESIAN_POINT('Ctrl Pts',(10.6417993727623,2.55558353607874,-1.96482643519855));
#65359=CARTESIAN_POINT('Ctrl Pts',(10.6465456971064,2.59984705735918,-1.90587093827602));
#65360=CARTESIAN_POINT('Ctrl Pts',(10.6708943001748,2.8133044833873,-1.60027408578584));
#65361=CARTESIAN_POINT('Ctrl Pts',(10.6916025761996,2.94957062066833,-1.33249807195055));
#65362=CARTESIAN_POINT('Ctrl Pts',(10.7165210401835,3.07249120300411,-0.975732475722724));
#65363=CARTESIAN_POINT('Ctrl Pts',(10.7216090816676,3.09530589282189,-0.900744022280118));
#65364=CARTESIAN_POINT('Ctrl Pts',(10.7272368731575,3.11814697053601,-0.814490663607777));
#65365=CARTESIAN_POINT('Ctrl Pts',(10.7279192110614,3.12087476727411,-0.803975289369373));
#65366=CARTESIAN_POINT('Ctrl Pts',(10.7289240095848,3.1248307704871,-0.788401741682506));
#65367=CARTESIAN_POINT('Ctrl Pts',(10.7292487819674,3.12609994296325,-0.783354197017556));
#65368=CARTESIAN_POINT('Ctrl Pts',(10.7298239946462,3.12833102816343,-0.774389314858562));
#65369=CARTESIAN_POINT('Ctrl Pts',(10.7300747156756,3.12929781782347,-0.770473231703493));
#65370=CARTESIAN_POINT('Ctrl Pts',(10.730608025257,3.13134216978543,-0.76212504368436));
#65371=CARTESIAN_POINT('Ctrl Pts',(10.7308904934686,3.13241767255121,-0.757692478378062));
#65372=CARTESIAN_POINT('Ctrl Pts',(10.7316547620564,3.13530769291171,-0.745670254177494));
#65373=CARTESIAN_POINT('Ctrl Pts',(10.7321355231264,3.13710407497373,-0.738076204030587));
#65374=CARTESIAN_POINT('Ctrl Pts',(10.7345384862177,3.14597300160057,-0.699966193493866));
#65375=CARTESIAN_POINT('Ctrl Pts',(10.7364376051507,3.15262823995214,-0.669353532881595));
#65376=CARTESIAN_POINT('Ctrl Pts',(10.7417757375914,3.17027144166617,-0.58208786926934));
#65377=CARTESIAN_POINT('Ctrl Pts',(10.745164034441,3.18018611901837,-0.525227916032883));
#65378=CARTESIAN_POINT('Ctrl Pts',(10.7573768535991,3.21083602520803,-0.316462106376153));
#65379=CARTESIAN_POINT('Ctrl Pts',(10.7659014796836,3.22225482488633,-0.163389725945583));
#65380=CARTESIAN_POINT('Ctrl Pts',(10.7882859263881,3.22350722279396,0.237111557682078));
#65381=CARTESIAN_POINT('Ctrl Pts',(10.8022022832353,3.19584058820361,0.483529069628185));
#65382=CARTESIAN_POINT('Ctrl Pts',(10.8183046115567,3.13592297253823,0.743291725833529));
#65383=CARTESIAN_POINT('Ctrl Pts',(10.8194842042186,3.13138236488608,0.762194160719128));
#65384=CARTESIAN_POINT('Ctrl Pts',(10.8212382352313,3.12440935112047,0.790108132561338));
#65385=CARTESIAN_POINT('Ctrl Pts',(10.821808427056,3.12210830819242,0.799152278065535));
#65386=CARTESIAN_POINT('Ctrl Pts',(10.8228229683182,3.11795353117459,0.815190587172139));
#65387=CARTESIAN_POINT('Ctrl Pts',(10.8232668073812,3.11611545678689,0.822188770657707));
#65388=CARTESIAN_POINT('Ctrl Pts',(10.8241999260801,3.11220838095086,0.836863046753264));
#65389=CARTESIAN_POINT('Ctrl Pts',(10.8246893612792,3.1101345142624,0.844537782971282));
#65390=CARTESIAN_POINT('Ctrl Pts',(10.8259764372727,3.10461669839605,0.864661527429642));
#65391=CARTESIAN_POINT('Ctrl Pts',(10.8267755864329,3.10112629315396,0.877097547071779));
#65392=CARTESIAN_POINT('Ctrl Pts',(10.8303554819545,3.08520505807529,0.932540301366794));
#65393=CARTESIAN_POINT('Ctrl Pts',(10.8331629000169,3.07195417578322,0.975304506446505));
#65394=CARTESIAN_POINT('Ctrl Pts',(10.8406831837549,3.03447088267411,1.08791959432837));
#65395=CARTESIAN_POINT('Ctrl Pts',(10.845444129525,3.00871946608693,1.1572330658912));
#65396=CARTESIAN_POINT('Ctrl Pts',(10.8699004850444,2.86634931776009,1.50347268331905));
#65397=CARTESIAN_POINT('Ctrl Pts',(10.890712285405,2.71381761622682,1.7639560446698));
#65398=CARTESIAN_POINT('Ctrl Pts',(10.9155966251401,2.4798461379286,2.05970069838304));
#65399=CARTESIAN_POINT('Ctrl Pts',(10.9205758654179,2.4301064643684,2.11815688440933));
#65400=CARTESIAN_POINT('Ctrl Pts',(10.9260970994815,2.37103048902065,2.1827617290786));
#65401=CARTESIAN_POINT('Ctrl Pts',(10.9267758536748,2.36369773219541,2.19070020414672));
#65402=CARTESIAN_POINT('Ctrl Pts',(10.9277763978277,2.35278196808258,2.20239904329441));
#65403=CARTESIAN_POINT('Ctrl Pts',(10.9281004717222,2.34922967206045,2.20618777171223));
#65404=CARTESIAN_POINT('Ctrl Pts',(10.9286749084147,2.34290301571094,2.21290290836365));
#65405=CARTESIAN_POINT('Ctrl Pts',(10.9289255491392,2.34013231224789,2.21583270684163));
#65406=CARTESIAN_POINT('Ctrl Pts',(10.9294591889812,2.33421127349482,2.22207024151147));
#65407=CARTESIAN_POINT('Ctrl Pts',(10.9297420658761,2.33105941349185,2.22537647127609));
#65408=CARTESIAN_POINT('Ctrl Pts',(10.9305085887633,2.32248325499181,2.23433445513798));
#65409=CARTESIAN_POINT('Ctrl Pts',(10.9309911849699,2.3170453190932,2.23997319613711));
#65410=CARTESIAN_POINT('Ctrl Pts',(10.9334182343379,2.28950636297631,2.26832148214583));
#65411=CARTESIAN_POINT('Ctrl Pts',(10.9353390460352,2.26709089235329,2.29072495001229));
#65412=CARTESIAN_POINT('Ctrl Pts',(10.9407546571137,2.20225113750743,2.35364576343924));
#65413=CARTESIAN_POINT('Ctrl Pts',(10.9441969491787,2.15904451397014,2.39334203342413));
#65414=CARTESIAN_POINT('Ctrl Pts',(10.9554913726172,2.01169529692556,2.5214798547272));
#65415=CARTESIAN_POINT('Ctrl Pts',(10.9631176861465,1.90302858750051,2.60446813034321));
#65416=CARTESIAN_POINT('Ctrl Pts',(10.9707498958509,1.78943619500353,2.68030514429072));
#65417=CARTESIAN_POINT('Origin',(-1.72497344927317,0.,0.));
#65418=CARTESIAN_POINT('',(12.4667878339183,1.79025515774613,2.68151164616949));
#65419=CARTESIAN_POINT('',(12.2173276938518,1.7894362103767,2.68030513402722));
#65420=CARTESIAN_POINT('',(-1.72497344927317,1.78943621037804,2.68030513402633));
#65421=CARTESIAN_POINT('',(11.6465734492731,-3.22274887732977,-0.00269001295207406));
#65422=CARTESIAN_POINT('Ctrl Pts',(11.6465747305505,-3.22026798849898,-0.00270873231344248));
#65423=CARTESIAN_POINT('Ctrl Pts',(11.6673417064361,-3.2229090083008,-0.339678147765568));
#65424=CARTESIAN_POINT('Ctrl Pts',(11.7543910885683,-3.01891887064386,-1.7490389311053));
#65425=CARTESIAN_POINT('Ctrl Pts',(11.907722876947,-0.972955838686834,-3.68536392752478));
#65426=CARTESIAN_POINT('Ctrl Pts',(12.1065700956867,2.57407380339523,-2.81117313536718));
#65427=CARTESIAN_POINT('Ctrl Pts',(12.2929250813438,3.68232104515272,0.428156541268224));
#65428=CARTESIAN_POINT('Ctrl Pts',(12.4129976607543,2.50903651599755,2.1911214231777));
#65429=CARTESIAN_POINT('Ctrl Pts',(12.4667878339183,1.79025515774624,2.68151164616941));
#65430=CARTESIAN_POINT('Ctrl Pts',(11.2169460942912,1.78943621037803,2.68030513402633));
#65431=CARTESIAN_POINT('Ctrl Pts',(11.2230963946181,1.70631866388706,2.7357964083296));
#65432=CARTESIAN_POINT('Ctrl Pts',(11.2292466949449,1.62062521831425,2.78741264291572));
#65433=CARTESIAN_POINT('Ctrl Pts',(11.2353969952718,1.53275713616186,2.83492030294414));
#65434=CARTESIAN_POINT('Ctrl Pts',(11.2417123473931,1.44253099279797,2.88370289657322));
#65435=CARTESIAN_POINT('Ctrl Pts',(11.2480276995145,1.35001224982185,2.92815301162533));
#65436=CARTESIAN_POINT('Ctrl Pts',(11.2543430516358,1.255660393657,2.96806915995924));
#65437=CARTESIAN_POINT('Ctrl Pts',(11.2605026451217,1.16363558372603,3.00700083669474));
#65438=CARTESIAN_POINT('Ctrl Pts',(11.2666622386076,1.06986747153118,3.04161951169496));
#65439=CARTESIAN_POINT('Ctrl Pts',(11.2728218320935,0.974799396232359,3.07178835527532));
#65440=CARTESIAN_POINT('Ctrl Pts',(11.2792150635326,0.876125318268297,3.10310152548705));
#65441=CARTESIAN_POINT('Ctrl Pts',(11.2856082949717,0.776051206474808,3.12962045609803));
#65442=CARTESIAN_POINT('Ctrl Pts',(11.2920015264108,0.675084567951585,3.15125028974431));
#65443=CARTESIAN_POINT('Ctrl Pts',(11.2983947578499,0.574117929428362,3.1728801233906));
#65444=CARTESIAN_POINT('Ctrl Pts',(11.304787989289,0.472259284429195,3.18962084680127));
#65445=CARTESIAN_POINT('Ctrl Pts',(11.3111812207281,0.370020441882947,3.20143755758077));
#65446=CARTESIAN_POINT('Ctrl Pts',(11.3173534688209,0.271315505744682,3.21284582134635));
#65447=CARTESIAN_POINT('Ctrl Pts',(11.3235257169136,0.171908744046664,3.21970506464383));
#65448=CARTESIAN_POINT('Ctrl Pts',(11.3296979650064,0.0722555323739138,
3.22193989710258));
#65449=CARTESIAN_POINT('Ctrl Pts',(11.335861853659,-0.0272627130683952,
3.22417170279573));
#65450=CARTESIAN_POINT('Ctrl Pts',(11.3420257423116,-0.127026314615012,
3.22179153662295));
#65451=CARTESIAN_POINT('Ctrl Pts',(11.3481896309643,-0.226573308854009,
3.21477559064625));
#65452=CARTESIAN_POINT('Ctrl Pts',(11.3543469926228,-0.32601489193455,3.20776707391438));
#65453=CARTESIAN_POINT('Ctrl Pts',(11.3605043542813,-0.425239892800191,
3.19613256703912));
#65454=CARTESIAN_POINT('Ctrl Pts',(11.3666617159398,-0.523785840049014,
3.17990030602598));
#65455=CARTESIAN_POINT('Ctrl Pts',(11.3728145800861,-0.622259806532849,
3.16367990151835));
#65456=CARTESIAN_POINT('Ctrl Pts',(11.3789674442324,-0.720055278225169,
3.14286849019346));
#65457=CARTESIAN_POINT('Ctrl Pts',(11.3851203083787,-0.816715322076124,
3.11754609351427));
#65458=CARTESIAN_POINT('Ctrl Pts',(11.3912708415153,-0.913338746313807,
3.09223329021345));
#65459=CARTESIAN_POINT('Ctrl Pts',(11.3974213746518,-1.00882717769941,3.06241300725973));
#65460=CARTESIAN_POINT('Ctrl Pts',(11.4035719077884,-1.10273516554363,3.02821609486071));
#65461=CARTESIAN_POINT('Ctrl Pts',(11.4097217560036,-1.19663269582537,2.99402299061855));
#65462=CARTESIAN_POINT('Ctrl Pts',(11.4158716042188,-1.28894972431919,2.95545437454502));
#65463=CARTESIAN_POINT('Ctrl Pts',(11.422021452434,-1.37925818446261,2.91269023809483));
#65464=CARTESIAN_POINT('Ctrl Pts',(11.4281722608131,-1.46958074429175,2.86991942496248));
#65465=CARTESIAN_POINT('Ctrl Pts',(11.4343230691923,-1.55789372027088,2.8229519762973));
#65466=CARTESIAN_POINT('Ctrl Pts',(11.4404738775714,-1.64379208487014,2.77201463636437));
#65467=CARTESIAN_POINT('Ctrl Pts',(11.4466312639376,-1.72978231354553,2.72102282145167));
#65468=CARTESIAN_POINT('Ctrl Pts',(11.4527886503038,-1.81335239988673,2.66605285922856));
#65469=CARTESIAN_POINT('Ctrl Pts',(11.45894603667,-1.89412495974367,2.60737573038027));
#65470=CARTESIAN_POINT('Ctrl Pts',(11.465106859407,-1.97494259789311,2.54866585446068));
#65471=CARTESIAN_POINT('Ctrl Pts',(11.4712676821439,-2.05295926112704,2.48624496305228));
#65472=CARTESIAN_POINT('Ctrl Pts',(11.4774285048809,-2.127831066487,2.42042403619548));
#65473=CARTESIAN_POINT('Ctrl Pts',(11.4835996277976,-2.20282804880539,2.35449306439738));
#65474=CARTESIAN_POINT('Ctrl Pts',(11.4897707507142,-2.27466935819926,2.28515100441456));
#65475=CARTESIAN_POINT('Ctrl Pts',(11.4959418736309,-2.34304826231248,2.21274544468506));
#65476=CARTESIAN_POINT('Ctrl Pts',(11.5006373955765,-2.39507682327521,2.1576530572407));
#65477=CARTESIAN_POINT('Ctrl Pts',(11.5053329175221,-2.44510160318005,2.10078782162479));
#65478=CARTESIAN_POINT('Ctrl Pts',(11.5100284394677,-2.49300396984336,2.04231456167879));
#65479=CARTESIAN_POINT('Ctrl Pts',(11.5161753576691,-2.55571306436904,1.96576708729302));
#65480=CARTESIAN_POINT('Ctrl Pts',(11.5223222758705,-2.61501043062012,1.8861856458203));
#65481=CARTESIAN_POINT('Ctrl Pts',(11.5284691940719,-2.67058657367766,1.80390823352869));
#65482=CARTESIAN_POINT('Ctrl Pts',(11.5346081463955,-2.72609069482889,1.72173744569416));
#65483=CARTESIAN_POINT('Ctrl Pts',(11.5407470987191,-2.77788292895277,1.6368779856665));
#65484=CARTESIAN_POINT('Ctrl Pts',(11.5468860510426,-2.82569326207592,1.54970163294705));
#65485=CARTESIAN_POINT('Ctrl Pts',(11.5530187220747,-2.87345467632444,1.46261447787151));
#65486=CARTESIAN_POINT('Ctrl Pts',(11.5591513931068,-2.91724207532969,1.37321552164076));
#65487=CARTESIAN_POINT('Ctrl Pts',(11.5652840641389,-2.95682870747237,1.28190544002561));
#65488=CARTESIAN_POINT('Ctrl Pts',(11.5714121324141,-2.99638562863891,1.19066388941475));
#65489=CARTESIAN_POINT('Ctrl Pts',(11.5775402006893,-3.03174787601952,1.09751446474921));
#65490=CARTESIAN_POINT('Ctrl Pts',(11.5836682689645,-3.06273511933149,1.00288142435361));
#65491=CARTESIAN_POINT('Ctrl Pts',(11.5897941624647,-3.09371136565719,0.908281968044084));
#65492=CARTESIAN_POINT('Ctrl Pts',(11.5959200559648,-3.12031555343767,0.812200356622423));
#65493=CARTESIAN_POINT('Ctrl Pts',(11.602045949465,-3.14241621670073,0.715078935164695));
#65494=CARTESIAN_POINT('Ctrl Pts',(11.6081705753739,-3.16451230681726,0.61797761041113));
#65495=CARTESIAN_POINT('Ctrl Pts',(11.6142952012828,-3.18210663260681,0.519837331328192));
#65496=CARTESIAN_POINT('Ctrl Pts',(11.6204198271917,-3.19511844360702,0.421112447954533));
#65497=CARTESIAN_POINT('Ctrl Pts',(11.6265465006768,-3.20813460469738,0.322354559018285));
#65498=CARTESIAN_POINT('Ctrl Pts',(11.6326731741619,-3.21656513731015,0.223012110210783));
#65499=CARTESIAN_POINT('Ctrl Pts',(11.638799847647,-3.2203810356016,0.123545732575258));
#65500=CARTESIAN_POINT('Ctrl Pts',(11.641391048189,-3.22199492244333,0.081477662150113));
#65501=CARTESIAN_POINT('Ctrl Pts',(11.6439822487311,-3.22278399919107,0.0393874569608355));
#65502=CARTESIAN_POINT('Ctrl Pts',(11.6465734492731,-3.22274887732977,-0.00269001295207406));
#65503=CARTESIAN_POINT('',(11.3976152427918,-3.22274951656853,0.0017652074350194));
#65504=CARTESIAN_POINT('Ctrl Pts',(10.9707498958509,1.78943619500353,2.68030514429072));
#65505=CARTESIAN_POINT('Ctrl Pts',(10.9718368339688,1.77325897948024,2.6911054425528));
#65506=CARTESIAN_POINT('Ctrl Pts',(10.9729237869157,1.75698185694029,2.70176070299239));
#65507=CARTESIAN_POINT('Ctrl Pts',(10.9875885956393,1.53619922227114,2.84344859257259));
#65508=CARTESIAN_POINT('Ctrl Pts',(11.0012823145276,1.31765202879979,2.95108085726157));
#65509=CARTESIAN_POINT('Ctrl Pts',(11.0171292205013,1.07071394942961,3.03974852536468));
#65510=CARTESIAN_POINT('Ctrl Pts',(11.0183149464139,1.05226214588065,3.04618512393336));
#65511=CARTESIAN_POINT('Ctrl Pts',(11.0200702493911,1.0249902733019,3.05542110014015));
#65512=CARTESIAN_POINT('Ctrl Pts',(11.0206355003337,1.01621462759011,3.05835102422926));
#65513=CARTESIAN_POINT('Ctrl Pts',(11.0216456627691,1.00054408801691,3.06350805268522));
#65514=CARTESIAN_POINT('Ctrl Pts',(11.022090087887,0.993654043688113,3.06574977795534));
#65515=CARTESIAN_POINT('Ctrl Pts',(11.0230044453405,0.979487662776576,3.07030613838045));
#65516=CARTESIAN_POINT('Ctrl Pts',(11.0234744596856,0.972210547718029,3.07261818555624));
#65517=CARTESIAN_POINT('Ctrl Pts',(11.0246938897476,0.953343721318345,3.07853872057092));
#65518=CARTESIAN_POINT('Ctrl Pts',(11.0254446014442,0.941741796796257,3.08210760466307));
#65519=CARTESIAN_POINT('Ctrl Pts',(11.0270846667164,0.916425070743717,3.08973902594954));
#65520=CARTESIAN_POINT('Ctrl Pts',(11.0279748425143,0.902702878308592,3.09377595530366));
#65521=CARTESIAN_POINT('Ctrl Pts',(11.0305656686192,0.862822576045433,3.10522042298376));
#65522=CARTESIAN_POINT('Ctrl Pts',(11.0322740408339,0.836597534483415,3.11238833782364));
#65523=CARTESIAN_POINT('Ctrl Pts',(11.0518854871312,0.536413459545543,3.19036762710496));
#65524=CARTESIAN_POINT('Ctrl Pts',(11.0710092006518,0.254411689949558,3.22511944150195));
#65525=CARTESIAN_POINT('Ctrl Pts',(11.0975325258762,-0.137952484776181,
3.22165853962935));
#65526=CARTESIAN_POINT('Ctrl Pts',(11.1048982611787,-0.247365993983254,
3.21510927837613));
#65527=CARTESIAN_POINT('Ctrl Pts',(11.1124168568245,-0.361312424122708,
3.20243609595026));
#65528=CARTESIAN_POINT('Ctrl Pts',(11.1127511832243,-0.36638413259871,3.2018598164832));
#65529=CARTESIAN_POINT('Ctrl Pts',(11.1169490120882,-0.430129084324271,
3.19446327175443));
#65530=CARTESIAN_POINT('Ctrl Pts',(11.1207552645447,-0.488610045497838,
3.18604267260742));
#65531=CARTESIAN_POINT('Ctrl Pts',(11.1251057086072,-0.556648412653623,
3.17432817338858));
#65532=CARTESIAN_POINT('Ctrl Pts',(11.1257310630043,-0.566458405833313,
3.17259226631824));
#65533=CARTESIAN_POINT('Ctrl Pts',(11.1266721999898,-0.581269898261237,
3.16990043887911));
#65534=CARTESIAN_POINT('Ctrl Pts',(11.1269898501709,-0.58627733014959,3.16897812867731));
#65535=CARTESIAN_POINT('Ctrl Pts',(11.127557229945,-0.595236781301901,3.16730593989917));
#65536=CARTESIAN_POINT('Ctrl Pts',(11.1278072116061,-0.599189586693744,
3.16656052879805));
#65537=CARTESIAN_POINT('Ctrl Pts',(11.1283442581897,-0.60769320316757,3.16494044296602));
#65538=CARTESIAN_POINT('Ctrl Pts',(11.1286311825967,-0.612243509586681,
3.16406335624155));
#65539=CARTESIAN_POINT('Ctrl Pts',(11.1294200968633,-0.624773891949282,
3.16162004048108));
#65540=CARTESIAN_POINT('Ctrl Pts',(11.1299209303861,-0.632750023117147,
3.16003340299419));
#65541=CARTESIAN_POINT('Ctrl Pts',(11.1326027023724,-0.675567655438603,
3.15134736687674));
#65542=CARTESIAN_POINT('Ctrl Pts',(11.1347536571604,-0.710297485816712,
3.14370157835538));
#65543=CARTESIAN_POINT('Ctrl Pts',(11.1410163408013,-0.812267226869926,
3.11947666494039));
#65544=CARTESIAN_POINT('Ctrl Pts',(11.145053734089,-0.879110470177674,3.10130275835436));
#65545=CARTESIAN_POINT('Ctrl Pts',(11.1577397054458,-1.09029099463534,3.03650754478775));
#65546=CARTESIAN_POINT('Ctrl Pts',(11.1661509258008,-1.23194855734697,2.98184841461059));
#65547=CARTESIAN_POINT('Ctrl Pts',(11.1876080596871,-1.57918355028459,2.81887988327354));
#65548=CARTESIAN_POINT('Ctrl Pts',(11.2007322267722,-1.77784822848497,2.69798787723824));
#65549=CARTESIAN_POINT('Ctrl Pts',(11.2158089183299,-1.97592310769465,2.54600900866633));
#65550=CARTESIAN_POINT('Ctrl Pts',(11.2168876356507,-1.98994601667987,2.53506387115332));
#65551=CARTESIAN_POINT('Ctrl Pts',(11.2185269142277,-2.01102696603919,2.51832711156122));
#65552=CARTESIAN_POINT('Ctrl Pts',(11.2190840778183,-2.01815234209973,2.51262054842001));
#65553=CARTESIAN_POINT('Ctrl Pts',(11.2200556580019,-2.03050804388148,2.50263866345888));
#65554=CARTESIAN_POINT('Ctrl Pts',(11.2204695220742,-2.03574937626996,2.4983770075835));
#65555=CARTESIAN_POINT('Ctrl Pts',(11.2213041390252,-2.0462751502121,2.48976353007093));
#65556=CARTESIAN_POINT('Ctrl Pts',(11.2217249077217,-2.05155920084512,2.48541128796058));
#65557=CARTESIAN_POINT('Ctrl Pts',(11.2227338125685,-2.06417510733382,2.47495247128393));
#65558=CARTESIAN_POINT('Ctrl Pts',(11.2233225910699,-2.07149375642266,2.46883013243413));
#65559=CARTESIAN_POINT('Ctrl Pts',(11.225191312501,-2.09458314865225,2.44933999474911));
#65560=CARTESIAN_POINT('Ctrl Pts',(11.2264761514391,-2.11025225930368,2.43585310445739));
#65561=CARTESIAN_POINT('Ctrl Pts',(11.2294840622157,-2.14645148418414,2.404083873935));
#65562=CARTESIAN_POINT('Ctrl Pts',(11.2312118246945,-2.16687934674344,2.38568796537753));
#65563=CARTESIAN_POINT('Ctrl Pts',(11.237176870011,-2.23614780132993,2.32168596204598));
#65564=CARTESIAN_POINT('Ctrl Pts',(11.2414664326412,-2.28380137768591,2.2748259112261));
#65565=CARTESIAN_POINT('Ctrl Pts',(11.2552982617909,-2.43068994919603,2.1211131561897));
#65566=CARTESIAN_POINT('Ctrl Pts',(11.2650488663257,-2.52413955721057,2.00900135770178));
#65567=CARTESIAN_POINT('Ctrl Pts',(11.2838536365566,-2.68748177603925,1.7835764632471));
#65568=CARTESIAN_POINT('Ctrl Pts',(11.2928713978114,-2.75859073274239,1.67149084831187));
#65569=CARTESIAN_POINT('Ctrl Pts',(11.3035754993457,-2.83595355167587,1.53109484604014));
#65570=CARTESIAN_POINT('Ctrl Pts',(11.3054163610485,-2.84900159904479,1.50667645141132));
#65571=CARTESIAN_POINT('Ctrl Pts',(11.3126311950841,-2.89917968335977,1.40978889754674));
#65572=CARTESIAN_POINT('Ctrl Pts',(11.3179253588035,-2.93387582409759,1.33608486955994));
#65573=CARTESIAN_POINT('Ctrl Pts',(11.3237545640332,-2.97003741146751,1.25104581404986));
#65574=CARTESIAN_POINT('Ctrl Pts',(11.3244435323143,-2.97427788081487,1.24093067906316));
#65575=CARTESIAN_POINT('Ctrl Pts',(11.3254527073168,-2.98044087341587,1.22601651032825));
#65576=CARTESIAN_POINT('Ctrl Pts',(11.3257752924799,-2.98240356605414,1.22123431560168));
#65577=CARTESIAN_POINT('Ctrl Pts',(11.3263487229751,-2.98587955837324,1.21270653676102));
#65578=CARTESIAN_POINT('Ctrl Pts',(11.3265998383929,-2.98739732881588,1.20896281245088));
#65579=CARTESIAN_POINT('Ctrl Pts',(11.3271317027224,-2.9906026122995,1.20101378401744));
#65580=CARTESIAN_POINT('Ctrl Pts',(11.3274123398188,-2.99228829153394,1.19680778533733));
#65581=CARTESIAN_POINT('Ctrl Pts',(11.3281665194033,-2.99680308307457,1.1854736007213));
#65582=CARTESIAN_POINT('Ctrl Pts',(11.3286390689375,-2.99961565315903,1.1783387937617));
#65583=CARTESIAN_POINT('Ctrl Pts',(11.3309374204723,-3.01321363547832,1.14347981896391));
#65584=CARTESIAN_POINT('Ctrl Pts',(11.3327424821882,-3.02364071801884,1.11561618237339));
#65585=CARTESIAN_POINT('Ctrl Pts',(11.3377492264172,-3.05178482937016,1.03711361747349));
#65586=CARTESIAN_POINT('Ctrl Pts',(11.3409074667142,-3.06862616184151,0.986169078056509));
#65587=CARTESIAN_POINT('Ctrl Pts',(11.3623755437678,-3.17588836406284,0.632287999099733));
#65588=CARTESIAN_POINT('Ctrl Pts',(11.3792697007114,-3.2225763519801,0.317912807196488));
#65589=CARTESIAN_POINT('Ctrl Pts',(11.3976152427918,-3.22274951656853,0.0017652074350194));
#65590=CARTESIAN_POINT('Ctrl Pts',(11.3976154732117,-3.22274951874103,0.00176123662453421));
#65591=CARTESIAN_POINT('Ctrl Pts',(11.4030792833307,-3.22280097590727,-0.0923962181032172));
#65592=CARTESIAN_POINT('Ctrl Pts',(11.4086442726123,-3.21872604207397,-0.186504860719464));
#65593=CARTESIAN_POINT('Ctrl Pts',(11.4150735136718,-3.20948468991639,-0.292356193350574));
#65594=CARTESIAN_POINT('Ctrl Pts',(11.4158081189327,-3.20836384239092,-0.304410195696163));
#65595=CARTESIAN_POINT('Ctrl Pts',(11.4170449194469,-3.20636824705999,-0.324634789139963));
#65596=CARTESIAN_POINT('Ctrl Pts',(11.4175459637667,-3.20553011141684,-0.332808931539696));
#65597=CARTESIAN_POINT('Ctrl Pts',(11.4184631617949,-3.2039417628058,-0.347736852810806));
#65598=CARTESIAN_POINT('Ctrl Pts',(11.41887900224,-3.20320143059321,-0.354491653189587));
#65599=CARTESIAN_POINT('Ctrl Pts',(11.4196944510381,-3.20171021030252,-0.367711368535341));
#65600=CARTESIAN_POINT('Ctrl Pts',(11.420094001709,-3.2009610903856,-0.374176453233502));
#65601=CARTESIAN_POINT('Ctrl Pts',(11.4210105781851,-3.19920042452651,-0.388979105426583));
#65602=CARTESIAN_POINT('Ctrl Pts',(11.4215280130225,-3.19817586278079,-0.397315050482128));
#65603=CARTESIAN_POINT('Ctrl Pts',(11.4229443857749,-3.19528796698414,-0.420076095344427));
#65604=CARTESIAN_POINT('Ctrl Pts',(11.4238453764884,-3.1933595606329,-0.4344926042981));
#65605=CARTESIAN_POINT('Ctrl Pts',(11.4282934748942,-3.18339222412179,-0.505353428532012));
#65606=CARTESIAN_POINT('Ctrl Pts',(11.431884648095,-3.17395443872685,-0.561587652131957));
#65607=CARTESIAN_POINT('Ctrl Pts',(11.436089493383,-3.16132581214271,-0.626271369944102));
#65608=CARTESIAN_POINT('Ctrl Pts',(11.4366582334135,-3.15958483873269,-0.634996349361112));
#65609=CARTESIAN_POINT('Ctrl Pts',(11.440006725582,-3.14914215379932,-0.686224060302044));
#65610=CARTESIAN_POINT('Ctrl Pts',(11.442810917839,-3.13961935580033,-0.728553217834638));
#65611=CARTESIAN_POINT('Ctrl Pts',(11.455929507767,-3.09148973603396,-0.923978321230943));
#65612=CARTESIAN_POINT('Ctrl Pts',(11.4665281641835,-3.04252339067055,-1.07428438254756));
#65613=CARTESIAN_POINT('Ctrl Pts',(11.4910622932218,-2.90517930777043,-1.40996812232759));
#65614=CARTESIAN_POINT('Ctrl Pts',(11.5050073547806,-2.80970595055505,-1.59174251365625));
#65615=CARTESIAN_POINT('Ctrl Pts',(11.5197868151541,-2.68333164367721,-1.78508551439961));
#65616=CARTESIAN_POINT('Ctrl Pts',(11.521442551638,-2.66878384496777,-1.80676282240783));
#65617=CARTESIAN_POINT('Ctrl Pts',(11.5235415179782,-2.6498160353469,-1.83429720984378));
#65618=CARTESIAN_POINT('Ctrl Pts',(11.5240002692345,-2.64563773796944,-1.84031851513517));
#65619=CARTESIAN_POINT('Ctrl Pts',(11.5247356574136,-2.63888650232743,-1.84997714550969));
#65620=CARTESIAN_POINT('Ctrl Pts',(11.525013167092,-2.63632652874139,-1.8536234368134));
#65621=CARTESIAN_POINT('Ctrl Pts',(11.5255425405405,-2.63141944797384,-1.86058209483606));
#65622=CARTESIAN_POINT('Ctrl Pts',(11.525794488299,-2.62907365017095,-1.86389532563395));
#65623=CARTESIAN_POINT('Ctrl Pts',(11.526375096267,-2.62364404829406,-1.87153351160692));
#65624=CARTESIAN_POINT('Ctrl Pts',(11.5267034491326,-2.62055578809358,-1.87585530882985));
#65625=CARTESIAN_POINT('Ctrl Pts',(11.5277542090972,-2.61061700614116,-1.88969147247413));
#65626=CARTESIAN_POINT('Ctrl Pts',(11.5284738159496,-2.60372515030398,-1.89917623337547));
#65627=CARTESIAN_POINT('Ctrl Pts',(11.5409088711975,-2.4831811780661,-2.06318259227469));
#65628=CARTESIAN_POINT('Ctrl Pts',(11.551723860799,-2.3559893126563,-2.20731713202712));
#65629=CARTESIAN_POINT('Ctrl Pts',(11.5716761621756,-2.09726358159207,-2.4524849316899));
#65630=CARTESIAN_POINT('Ctrl Pts',(11.5808062213939,-1.96932393292658,-2.55635631036144));
#65631=CARTESIAN_POINT('Ctrl Pts',(11.5951825475722,-1.76287525931155,-2.69923579317916));
#65632=CARTESIAN_POINT('Ctrl Pts',(11.6002083844087,-1.68978363771895,-2.74558419614712));
#65633=CARTESIAN_POINT('Ctrl Pts',(11.6072971642213,-1.58631966490739,-2.80549455872093));
#65634=CARTESIAN_POINT('Ctrl Pts',(11.60927117705,-1.55746718152246,-2.82161401652705));
#65635=CARTESIAN_POINT('Ctrl Pts',(11.6122528586553,-1.51386493772445,-2.84510141472059));
#65636=CARTESIAN_POINT('Ctrl Pts',(11.613248771968,-1.49929769998549,-2.85280484805979));
#65637=CARTESIAN_POINT('Ctrl Pts',(11.61507719748,-1.47255171575014,-2.86668719804918));
#65638=CARTESIAN_POINT('Ctrl Pts',(11.6159084616364,-1.46039148888122,-2.87290110119645));
#65639=CARTESIAN_POINT('Ctrl Pts',(11.6172348221687,-1.44098995887658,-2.88266031635028));
#65640=CARTESIAN_POINT('Ctrl Pts',(11.61772814228,-1.43377412030901,-2.88625610975673));
#65641=CARTESIAN_POINT('Ctrl Pts',(11.6182245488201,-1.42651366986361,-2.8898401882122));
#65642=CARTESIAN_POINT('Ctrl Pts',(11.6182266852154,-1.42648242291999,-2.88985561245097));
#65643=CARTESIAN_POINT('Ctrl Pts',(11.6182309903186,-1.42641945644778,-2.88988669293767));
#65644=CARTESIAN_POINT('Ctrl Pts',(11.6182331590115,-1.42638773713914,-2.88990234905786));
#65645=CARTESIAN_POINT('Ctrl Pts',(11.6182375292541,-1.42632381797779,-2.889933897178));
#65646=CARTESIAN_POINT('Ctrl Pts',(11.6182397307896,-1.42629161833368,-2.88994978905521));
#65647=CARTESIAN_POINT('Ctrl Pts',(11.6182441672579,-1.42622673059869,-2.88998181253002));
#65648=CARTESIAN_POINT('Ctrl Pts',(11.6182464021847,-1.42619404259534,-2.889997944064));
#65649=CARTESIAN_POINT('Ctrl Pts',(11.6182509060011,-1.42612816987234,-2.89003045087171));
#65650=CARTESIAN_POINT('Ctrl Pts',(11.6182531748815,-1.42609498528727,-2.89004682605797));
#65651=CARTESIAN_POINT('Ctrl Pts',(11.6182577471864,-1.4260281108968,-2.890079824303));
#65652=CARTESIAN_POINT('Ctrl Pts',(11.6182600505973,-1.42599442129138,-2.89009644724134));
#65653=CARTESIAN_POINT('Ctrl Pts',(11.618264692537,-1.42592652847227,-2.89012994506363));
#65654=CARTESIAN_POINT('Ctrl Pts',(11.6182670310597,-1.42589232534842,-2.89014681988077));
#65655=CARTESIAN_POINT('Ctrl Pts',(11.6182717438154,-1.42582339682499,-2.89018082566915));
#65656=CARTESIAN_POINT('Ctrl Pts',(11.6182741180425,-1.42578867151328,-2.89019795657384));
#65657=CARTESIAN_POINT('Ctrl Pts',(11.618278902819,-1.42571868966853,-2.89023247888041));
#65658=CARTESIAN_POINT('Ctrl Pts',(11.6182813133581,-1.42568343328511,-2.89024987018454));
#65659=CARTESIAN_POINT('Ctrl Pts',(11.6182861713715,-1.42561238033184,-2.89028491764006));
#65660=CARTESIAN_POINT('Ctrl Pts',(11.6182886188383,-1.42557658387282,-2.89030257371206));
#65661=CARTESIAN_POINT('Ctrl Pts',(11.6182935513334,-1.42550444161099,-2.89033815514544));
#65662=CARTESIAN_POINT('Ctrl Pts',(11.6182960363549,-1.42546809590557,-2.89035608043327));
#65663=CARTESIAN_POINT('Ctrl Pts',(11.6183010445995,-1.42539484579282,-2.89039220483662));
#65664=CARTESIAN_POINT('Ctrl Pts',(11.6183035678154,-1.42535794148883,-2.89041040387482));
#65665=CARTESIAN_POINT('Ctrl Pts',(11.6183086530986,-1.4252835646723,-2.89044708038748));
#65666=CARTESIAN_POINT('Ctrl Pts',(11.61831121516,-1.42524609224698,-2.89046555779173));
#65667=CARTESIAN_POINT('Ctrl Pts',(11.6183163787931,-1.42517056955159,-2.89050279570591));
#65668=CARTESIAN_POINT('Ctrl Pts',(11.6183189803616,-1.42513251932988,-2.8905215561639));
#65669=CARTESIAN_POINT('Ctrl Pts',(11.6183242236813,-1.42505583120969,-2.8905593649484));
#65670=CARTESIAN_POINT('Ctrl Pts',(11.6183268654291,-1.42501719336021,-2.89057841322173));
#65671=CARTESIAN_POINT('Ctrl Pts',(11.6183321898058,-1.42493931977284,-2.89061680258362));
#65672=CARTESIAN_POINT('Ctrl Pts',(11.6183348724246,-1.42490008418203,-2.8906361435697));
#65673=CARTESIAN_POINT('Ctrl Pts',(11.6183402792324,-1.42482100503457,-2.89067512323426));
#65674=CARTESIAN_POINT('Ctrl Pts',(11.6183430034191,-1.42478116151051,-2.89069476186572));
#65675=CARTESIAN_POINT('Ctrl Pts',(11.6183484940705,-1.42470085614672,-2.89073434182901));
#65676=CARTESIAN_POINT('Ctrl Pts',(11.6183512605342,-1.42466039432034,-2.89075428312228));
#65677=CARTESIAN_POINT('Ctrl Pts',(11.6183568364996,-1.42457884123547,-2.89079447379136));
#65678=CARTESIAN_POINT('Ctrl Pts',(11.6183596459939,-1.42453775008669,-2.89081472308002));
#65679=CARTESIAN_POINT('Ctrl Pts',(11.6183652768917,-1.42445539364287,-2.89085530529253));
#65680=CARTESIAN_POINT('Ctrl Pts',(11.6183680983677,-1.42441412728829,-2.89087563872917));
#65681=CARTESIAN_POINT('Ctrl Pts',(11.6183739319694,-1.42432880620964,-2.89091767726326));
#65682=CARTESIAN_POINT('Ctrl Pts',(11.6183769440835,-1.4242847516575,-2.89093938212267));
#65683=CARTESIAN_POINT('Ctrl Pts',(11.6183831719932,-1.4241936635957,-2.89098425693097));
#65684=CARTESIAN_POINT('Ctrl Pts',(11.618386387773,-1.42414663031743,-2.89100742659102));
#65685=CARTESIAN_POINT('Ctrl Pts',(11.6183930369296,-1.42404938128599,-2.89105533072135));
#65686=CARTESIAN_POINT('Ctrl Pts',(11.6183964702986,-1.42399916564901,-2.89108006493495));
#65687=CARTESIAN_POINT('Ctrl Pts',(11.618403569509,-1.42389533434632,-2.89113120471877));
#65688=CARTESIAN_POINT('Ctrl Pts',(11.6184072353477,-1.42384171872246,-2.8911576100409));
#65689=CARTESIAN_POINT('Ctrl Pts',(11.6188556032743,-1.41728400732104,-2.89438701066855));
#65690=CARTESIAN_POINT('Ctrl Pts',(11.619301071121,-1.41076916561674,-2.89756802938455));
#65691=CARTESIAN_POINT('Ctrl Pts',(11.6203186765309,-1.39588840160288,-2.90477181616293));
#65692=CARTESIAN_POINT('Ctrl Pts',(11.6208913017214,-1.38751574950751,-2.90878046192627));
#65693=CARTESIAN_POINT('Ctrl Pts',(11.6226833516792,-1.36131748750213,-2.92118477677408));
#65694=CARTESIAN_POINT('Ctrl Pts',(11.6239071737684,-1.34343238389581,-2.92945305542688));
#65695=CARTESIAN_POINT('Ctrl Pts',(11.6356827956183,-1.17142594406243,-3.00706513261379));
#65696=CARTESIAN_POINT('Ctrl Pts',(11.646650579351,-1.01217578535702,-3.064337342645));
#65697=CARTESIAN_POINT('Ctrl Pts',(11.6701116120815,-0.672518935328235,
-3.15711548937967));
#65698=CARTESIAN_POINT('Ctrl Pts',(11.6826159514843,-0.492056530533508,
-3.190224904393));
#65699=CARTESIAN_POINT('Ctrl Pts',(11.7034103860448,-0.183907028303194,
-3.21998227296595));
#65700=CARTESIAN_POINT('Ctrl Pts',(11.7117821620842,-0.0574185693492307,
-3.22471988302917));
#65701=CARTESIAN_POINT('Ctrl Pts',(11.7207068582696,0.0834890059778667,
-3.22170082170197));
#65702=CARTESIAN_POINT('Ctrl Pts',(11.7216175048805,0.0979418457486973,
-3.22129384130052));
#65703=CARTESIAN_POINT('Ctrl Pts',(11.7228890511351,0.118235853103794,-3.2205856672979));
#65704=CARTESIAN_POINT('Ctrl Pts',(11.7232543552747,0.124079422455464,-3.22036582635705));
#65705=CARTESIAN_POINT('Ctrl Pts',(11.7238764975805,0.134054811634172,-3.21996334986497));
#65706=CARTESIAN_POINT('Ctrl Pts',(11.7241337805494,0.138186921520019,-3.21978866424567));
#65707=CARTESIAN_POINT('Ctrl Pts',(11.7246252767023,0.14609398827626,-3.21943914207546));
#65708=CARTESIAN_POINT('Ctrl Pts',(11.7248595646832,0.149868975183894,-3.21926562022571));
#65709=CARTESIAN_POINT('Ctrl Pts',(11.7254129406066,0.158798792764812,-3.21883940912449));
#65710=CARTESIAN_POINT('Ctrl Pts',(11.7257317057489,0.163953358006502,-3.21858097545954));
#65711=CARTESIAN_POINT('Ctrl Pts',(11.7266793887766,0.179308656952439,-3.2177741254784));
#65712=CARTESIAN_POINT('Ctrl Pts',(11.7273063229699,0.189507544197452,-3.2171895832011));
#65713=CARTESIAN_POINT('Ctrl Pts',(11.7337090286984,0.294059267496227,-3.2106983683862));
#65714=CARTESIAN_POINT('Ctrl Pts',(11.7392677841558,0.38812170402163,-3.20069057901056));
#65715=CARTESIAN_POINT('Ctrl Pts',(11.7611131741272,0.763381562901674,-3.14397374492723));
#65716=CARTESIAN_POINT('Ctrl Pts',(11.7764741001173,1.03825792402893,-3.06420658437873));
#65717=CARTESIAN_POINT('Ctrl Pts',(11.7970687682451,1.36478608382635,-2.92038216434556));
#65718=CARTESIAN_POINT('Ctrl Pts',(11.8012685460282,1.42950656879135,-2.88925300980226));
#65719=CARTESIAN_POINT('Ctrl Pts',(11.8072622704578,1.51878196931448,-2.84257924121321));
#65720=CARTESIAN_POINT('Ctrl Pts',(11.8089957409726,1.54425101628792,-2.82882380698595));
#65721=CARTESIAN_POINT('Ctrl Pts',(11.8116437641757,1.58260276374439,-2.807438345634));
#65722=CARTESIAN_POINT('Ctrl Pts',(11.8125494998335,1.59562369186246,-2.80005831987655));
#65723=CARTESIAN_POINT('Ctrl Pts',(11.8142257945611,1.61954036245628,-2.78628178738399));
#65724=CARTESIAN_POINT('Ctrl Pts',(11.8149954072263,1.6304508486999,-2.77991136678741));
#65725=CARTESIAN_POINT('Ctrl Pts',(11.8162454066413,1.64805683454,-2.76949227278751));
#65726=CARTESIAN_POINT('Ctrl Pts',(11.8167243538346,1.65477561402784,-2.7654830399795));
#65727=CARTESIAN_POINT('Ctrl Pts',(11.8176474422113,1.66767245046208,-2.75772340780324));
#65728=CARTESIAN_POINT('Ctrl Pts',(11.8180914493801,1.67385262838838,-2.75397661084079));
#65729=CARTESIAN_POINT('Ctrl Pts',(11.8191064903596,1.68792779920184,-2.74537851181137));
#65730=CARTESIAN_POINT('Ctrl Pts',(11.8196780121361,1.69581454967065,-2.74051390047317));
#65731=CARTESIAN_POINT('Ctrl Pts',(11.8214316948556,1.71989659673098,-2.72551613957464));
#65732=CARTESIAN_POINT('Ctrl Pts',(11.8226179187405,1.73602263766676,-2.71527308142578));
#65733=CARTESIAN_POINT('Ctrl Pts',(11.8400198874576,1.97018231416575,-2.56359913336304));
#65734=CARTESIAN_POINT('Ctrl Pts',(11.8572762406115,2.17037034543168,-2.39647568615865));
#65735=CARTESIAN_POINT('Ctrl Pts',(11.8887207414989,2.48874109729795,-2.05775185658825));
#65736=CARTESIAN_POINT('Ctrl Pts',(11.9026829934451,2.61462272152304,-1.89524083545589));
#65737=CARTESIAN_POINT('Ctrl Pts',(11.9174788617099,2.7381668774314,-1.69977701998558));
#65738=CARTESIAN_POINT('Ctrl Pts',(11.9191355373413,2.75185340937114,-1.67752874304802));
#65739=CARTESIAN_POINT('Ctrl Pts',(11.9212355165374,2.7690331145288,-1.64882591778891));
#65740=CARTESIAN_POINT('Ctrl Pts',(11.9216943595615,2.77277635363194,-1.64252323933809));
#65741=CARTESIAN_POINT('Ctrl Pts',(11.9224298595712,2.77876017988937,-1.63236922190783));
#65742=CARTESIAN_POINT('Ctrl Pts',(11.9227073897806,2.78101431474668,-1.62852595795106));
#65743=CARTESIAN_POINT('Ctrl Pts',(11.9232367776326,2.78530699158226,-1.6211721082669));
#65744=CARTESIAN_POINT('Ctrl Pts',(11.9234887193588,2.78734686483042,-1.61766235576016));
#65745=CARTESIAN_POINT('Ctrl Pts',(11.9240692803987,2.79204022854193,-1.60955184208211));
#65746=CARTESIAN_POINT('Ctrl Pts',(11.92439759253,2.79468899824165,-1.60494834004477));
#65747=CARTESIAN_POINT('Ctrl Pts',(11.9252776609965,2.80177433085987,-1.59256346597219));
#65748=CARTESIAN_POINT('Ctrl Pts',(11.9258280836053,2.80618989201173,-1.58477004281781));
#65749=CARTESIAN_POINT('Ctrl Pts',(11.9298283319623,2.83815844446283,-1.52779329544939));
#65750=CARTESIAN_POINT('Ctrl Pts',(11.9332015567738,2.86445112991647,-1.47790945149096));
#65751=CARTESIAN_POINT('Ctrl Pts',(11.9552060438616,3.03012217461485,-1.1425389407093));
#65752=CARTESIAN_POINT('Ctrl Pts',(11.9721397753154,3.12794966611081,-0.838460047124573));
#65753=CARTESIAN_POINT('Ctrl Pts',(11.9948518934996,3.1922289418811,-0.449110757560269));
#65754=CARTESIAN_POINT('Ctrl Pts',(11.9993370828402,3.20203165270326,-0.372851335452781));
#65755=CARTESIAN_POINT('Ctrl Pts',(12.0066419083099,3.21333437417297,-0.250443915989653));
#65756=CARTESIAN_POINT('Ctrl Pts',(12.0094079149258,3.21658594061573,-0.204485975277617));
#65757=CARTESIAN_POINT('Ctrl Pts',(12.012997195294,3.21949282842075,-0.145443284963265));
#65758=CARTESIAN_POINT('Ctrl Pts',(12.0137919051916,3.22005530523614,-0.13240711756587));
#65759=CARTESIAN_POINT('Ctrl Pts',(12.0150766131214,3.220834143467,-0.111394135025089));
#65760=CARTESIAN_POINT('Ctrl Pts',(12.0155650518879,3.22110007561357,-0.103419215386652));
#65761=CARTESIAN_POINT('Ctrl Pts',(12.0164977420998,3.22155045962202,-0.088218188554183));
#65762=CARTESIAN_POINT('Ctrl Pts',(12.0169418238561,3.22174022264801,-0.0809922780188563));
#65763=CARTESIAN_POINT('Ctrl Pts',(12.0179575225214,3.22211798695037,-0.0644924862200333));
#65764=CARTESIAN_POINT('Ctrl Pts',(12.0185296296927,3.22229026230542,-0.0552183409577267));
#65765=CARTESIAN_POINT('Ctrl Pts',(12.0202868625372,3.22269552504108,-0.0267937921074276));
#65766=CARTESIAN_POINT('Ctrl Pts',(12.0214760751535,3.2227978412322,-0.00764221514064361));
#65767=CARTESIAN_POINT('Ctrl Pts',(12.0387792645531,3.22180722401552,0.269753237045434));
#65768=CARTESIAN_POINT('Ctrl Pts',(12.0559195218478,3.18984880331787,0.526895148246636));
#65769=CARTESIAN_POINT('Ctrl Pts',(12.0873486623927,3.07775653403808,0.97784951508932));
#65770=CARTESIAN_POINT('Ctrl Pts',(12.1014157192694,3.00877757872783,1.17305043184118));
#65771=CARTESIAN_POINT('Ctrl Pts',(12.116311573329,2.91052126951814,1.38407743461582));
#65772=CARTESIAN_POINT('Ctrl Pts',(12.1179739504862,2.89916920904953,1.4077011073894));
#65773=CARTESIAN_POINT('Ctrl Pts',(12.1200800774014,2.88427056839706,1.43776031173633));
#65774=CARTESIAN_POINT('Ctrl Pts',(12.120539476472,2.88098884599977,1.44432499717204));
#65775=CARTESIAN_POINT('Ctrl Pts',(12.1212756540901,2.87567794129688,1.45485869054886));
#65776=CARTESIAN_POINT('Ctrl Pts',(12.1215533087006,2.87366292372441,1.45883475175053));
#65777=CARTESIAN_POINT('Ctrl Pts',(12.1220827840209,2.86979732086402,1.46642332707834));
#65778=CARTESIAN_POINT('Ctrl Pts',(12.1223346893922,2.86794816573895,1.47003651513041));
#65779=CARTESIAN_POINT('Ctrl Pts',(12.1229149669742,2.86366544997617,1.47836596215495));
#65780=CARTESIAN_POINT('Ctrl Pts',(12.123243032978,2.8612270468626,1.4830797398334));
#65781=CARTESIAN_POINT('Ctrl Pts',(12.124291951952,2.85337630155461,1.49816491150735));
#65782=CARTESIAN_POINT('Ctrl Pts',(12.1250100184607,2.84791905122703,1.50851301213808));
#65783=CARTESIAN_POINT('Ctrl Pts',(12.1375151949251,2.7514553837827,1.68903921497881));
#65784=CARTESIAN_POINT('Ctrl Pts',(12.148390680195,2.64538503910836,1.85076253007993));
#65785=CARTESIAN_POINT('Ctrl Pts',(12.1683845093426,2.42347221361037,2.13069321539516));
#65786=CARTESIAN_POINT('Ctrl Pts',(12.177495362016,2.31180279152574,2.25136323263004));
#65787=CARTESIAN_POINT('Ctrl Pts',(12.1918248093078,2.12835995277317,2.42148731095344));
#65788=CARTESIAN_POINT('Ctrl Pts',(12.1968227738933,2.06297622413764,2.47742694812193));
#65789=CARTESIAN_POINT('Ctrl Pts',(12.2048876579758,1.95617728974188,2.56163767281453));
#65790=CARTESIAN_POINT('Ctrl Pts',(12.2078854404039,1.91620444743983,2.59167460435374));
#65791=CARTESIAN_POINT('Ctrl Pts',(12.2117345993995,1.86463379678907,2.62858109694496));
#65792=CARTESIAN_POINT('Ctrl Pts',(12.2125520079288,1.8536683092901,2.63632539151649));
#65793=CARTESIAN_POINT('Ctrl Pts',(12.2138645988867,1.83603968070425,2.64861112072296));
#65794=CARTESIAN_POINT('Ctrl Pts',(12.2143580963784,1.82940724634574,2.6531965066852));
#65795=CARTESIAN_POINT('Ctrl Pts',(12.2152947508577,1.81681075893974,2.66183550015097));
#65796=CARTESIAN_POINT('Ctrl Pts',(12.2157377148675,1.81085016323904,2.66589408053177));
#65797=CARTESIAN_POINT('Ctrl Pts',(12.2165629633247,1.79973938080712,2.67340497611388));
#65798=CARTESIAN_POINT('Ctrl Pts',(12.2169450469949,1.79459275143243,2.67686250312364));
#65799=CARTESIAN_POINT('Ctrl Pts',(12.2173276938518,1.78943621037674,2.68030513402719));
#65800=CARTESIAN_POINT('Origin',(-1.72497344927317,0.,0.));
#65801=CARTESIAN_POINT('',(13.7170510877849,1.78943621037804,2.68030513402632));
#65802=CARTESIAN_POINT('',(13.4707798281485,1.78943605929599,2.68030523489233));
#65803=CARTESIAN_POINT('',(-1.72497344927317,1.78943621037804,2.68030513402633));
#65804=CARTESIAN_POINT('',(12.8965733803554,-3.22322736952655,-0.000539841530475302));
#65805=CARTESIAN_POINT('Ctrl Pts',(12.8965734492731,-3.22274995461277,-0.000540872794637355));
#65806=CARTESIAN_POINT('Ctrl Pts',(12.8983686230638,-3.22274510388462,-0.0294435724144985));
#65807=CARTESIAN_POINT('Ctrl Pts',(12.9001637968545,-3.22235144858765,-0.0583426038275036));
#65808=CARTESIAN_POINT('Ctrl Pts',(12.9019589706452,-3.22156922997986,-0.087231066409683));
#65809=CARTESIAN_POINT('Ctrl Pts',(12.908131218738,-3.21887977042166,-0.186556691036267));
#65810=CARTESIAN_POINT('Ctrl Pts',(12.9143034668308,-3.21158774489631,-0.285932643125343));
#65811=CARTESIAN_POINT('Ctrl Pts',(12.9204757149235,-3.19968303244483,-0.384897459571556));
#65812=CARTESIAN_POINT('Ctrl Pts',(12.9266396035761,-3.18779444324854,-0.483728242121913));
#65813=CARTESIAN_POINT('Ctrl Pts',(12.9328034922288,-3.17130563561325,-0.582148568311957));
#65814=CARTESIAN_POINT('Ctrl Pts',(12.9389673808814,-3.15025848405349,-0.679697760882756));
#65815=CARTESIAN_POINT('Ctrl Pts',(12.94512474254,-3.12923361950138,-0.777143657784523));
#65816=CARTESIAN_POINT('Ctrl Pts',(12.9512821041985,-3.10366009840369,-0.87371983272308));
#65817=CARTESIAN_POINT('Ctrl Pts',(12.9574394658571,-3.07363138632727,-0.968972478187012));
#65818=CARTESIAN_POINT('Ctrl Pts',(12.9635923300034,-3.04362460807703,-1.064155548407));
#65819=CARTESIAN_POINT('Ctrl Pts',(12.9697451941497,-3.00916923895926,-1.15801659817647));
#65820=CARTESIAN_POINT('Ctrl Pts',(12.975898058296,-2.97040922318094,-1.25011463847986));
#65821=CARTESIAN_POINT('Ctrl Pts',(12.9820485914325,-2.93166389161689,-1.34217778748273));
#65822=CARTESIAN_POINT('Ctrl Pts',(12.9881991245691,-2.88861732211819,-1.43247885424437));
#65823=CARTESIAN_POINT('Ctrl Pts',(12.9943496577056,-2.84146214843125,-1.52059541678004));
#65824=CARTESIAN_POINT('Ctrl Pts',(13.0004995059208,-2.79431222592883,-1.6087021666845));
#65825=CARTESIAN_POINT('Ctrl Pts',(13.006649354136,-2.74305481383244,-1.69462451302655));
#65826=CARTESIAN_POINT('Ctrl Pts',(13.0127992023512,-2.68792872889643,-1.77796420404721));
#65827=CARTESIAN_POINT('Ctrl Pts',(13.0189500107304,-2.63279403723115,-1.86131690673301));
#65828=CARTESIAN_POINT('Ctrl Pts',(13.0251008191095,-2.57378971267325,-1.94208579086444));
#65829=CARTESIAN_POINT('Ctrl Pts',(13.0312516274886,-2.51119758955371,-2.01990203443623));
#65830=CARTESIAN_POINT('Ctrl Pts',(13.0374090138548,-2.44853852723692,-2.09780149865334));
#65831=CARTESIAN_POINT('Ctrl Pts',(13.043566400221,-2.38228427709887,-2.17274167757312));
#65832=CARTESIAN_POINT('Ctrl Pts',(13.0497237865872,-2.31275654777633,-2.24438738038194));
#65833=CARTESIAN_POINT('Ctrl Pts',(13.0558846093242,-2.24319001577965,-2.31607306788301));
#65834=CARTESIAN_POINT('Ctrl Pts',(13.0620454320611,-2.17034668305933,-2.38446032038353));
#65835=CARTESIAN_POINT('Ctrl Pts',(13.0682062547981,-2.09458310839748,-2.44925277677008));
#65836=CARTESIAN_POINT('Ctrl Pts',(13.0743773777148,-2.01869286584251,-2.51415355861484));
#65837=CARTESIAN_POINT('Ctrl Pts',(13.0805485006314,-1.93987297214905,-2.57544727261753));
#65838=CARTESIAN_POINT('Ctrl Pts',(13.0867196235481,-1.85851096250388,-2.63287951960452));
#65839=CARTESIAN_POINT('Ctrl Pts',(13.0914151454937,-1.79660373638251,-2.67657892079172));
#65840=CARTESIAN_POINT('Ctrl Pts',(13.0961106674393,-1.73322539924232,-2.71804360465058));
#65841=CARTESIAN_POINT('Ctrl Pts',(13.1008061893849,-1.66855591829974,-2.75717948454701));
#65842=CARTESIAN_POINT('Ctrl Pts',(13.1069784374777,-1.58354809914073,-2.80862346944334));
#65843=CARTESIAN_POINT('Ctrl Pts',(13.1131506855704,-1.49600928952659,-2.8562229473945));
#65844=CARTESIAN_POINT('Ctrl Pts',(13.1193229336632,-1.40632220382896,-2.89971988673349));
#65845=CARTESIAN_POINT('Ctrl Pts',(13.1254868223158,-1.3167565866485,-2.94315791559855));
#65846=CARTESIAN_POINT('Ctrl Pts',(13.1316507109685,-1.22504886380467,-2.98250426174899));
#65847=CARTESIAN_POINT('Ctrl Pts',(13.1378145996211,-1.13160920309297,-3.01754505748883));
#65848=CARTESIAN_POINT('Ctrl Pts',(13.1439719612796,-1.03826848643223,-3.05254874823223));
#65849=CARTESIAN_POINT('Ctrl Pts',(13.1501293229382,-0.943199882470942,
-3.08325580097137));
#65850=CARTESIAN_POINT('Ctrl Pts',(13.1562866845967,-0.846835675922031,
-3.10949946140624));
#65851=CARTESIAN_POINT('Ctrl Pts',(13.162439548743,-0.750541856532804,-3.13572395272444));
#65852=CARTESIAN_POINT('Ctrl Pts',(13.1685924128893,-0.652954733899122,
-3.1574914197555));
#65853=CARTESIAN_POINT('Ctrl Pts',(13.1747452770356,-0.554523104018507,
-3.17468450237337));
#65854=CARTESIAN_POINT('Ctrl Pts',(13.1808958101722,-0.456128764915871,
-3.19187107139976));
#65855=CARTESIAN_POINT('Ctrl Pts',(13.1870463433087,-0.356890981709488,
-3.20448662482355));
#65856=CARTESIAN_POINT('Ctrl Pts',(13.1931968764452,-0.257269258577538,
-3.21246479997695));
#65857=CARTESIAN_POINT('Ctrl Pts',(13.1993467246604,-0.157658629287641,
-3.22044208668342));
#65858=CARTESIAN_POINT('Ctrl Pts',(13.2054965728757,-0.057664578065635,
-3.22378298715598));
#65859=CARTESIAN_POINT('Ctrl Pts',(13.2116464210909,0.0422487514944001,
-3.22247305737335));
#65860=CARTESIAN_POINT('Ctrl Pts',(13.21779722947,0.142177680329623,-3.22116292307392));
#65861=CARTESIAN_POINT('Ctrl Pts',(13.2239480378491,0.242025428091404,-3.2152005219422));
#65862=CARTESIAN_POINT('Ctrl Pts',(13.2300988462283,0.341329347712653,-3.20462350969502));
#65863=CARTESIAN_POINT('Ctrl Pts',(13.2362562325944,0.440739467992037,-3.19403518585344));
#65864=CARTESIAN_POINT('Ctrl Pts',(13.2424136189606,0.539604165966645,-3.17882244210764));
#65865=CARTESIAN_POINT('Ctrl Pts',(13.2485710053268,0.637467524982191,-3.1590746615256));
#65866=CARTESIAN_POINT('Ctrl Pts',(13.2547318280638,0.735385500480527,-3.13931585992069));
#65867=CARTESIAN_POINT('Ctrl Pts',(13.2608926508007,0.832300602756806,-3.11501708675905));
#65868=CARTESIAN_POINT('Ctrl Pts',(13.2670534735377,0.92777073521625,-3.08631803697809));
#65869=CARTESIAN_POINT('Ctrl Pts',(13.2732245964544,1.02340048264355,-3.05757100572073));
#65870=CARTESIAN_POINT('Ctrl Pts',(13.2793957193711,1.11758002481608,-3.02440914729465));
#65871=CARTESIAN_POINT('Ctrl Pts',(13.2855668422878,1.20988581463768,-2.98702090351549));
#65872=CARTESIAN_POINT('Ctrl Pts',(13.2902623642334,1.28012001150308,-2.95857270672186));
#65873=CARTESIAN_POINT('Ctrl Pts',(13.2949578861789,1.3492697890222,-2.92767866368436));
#65874=CARTESIAN_POINT('Ctrl Pts',(13.2996534081245,1.41715869056307,-2.89443929082328));
#65875=CARTESIAN_POINT('Ctrl Pts',(13.3058256562173,1.50639842746816,-2.8507462449544));
#65876=CARTESIAN_POINT('Ctrl Pts',(13.31199790431,1.59377266331493,-2.80284534308314));
#65877=CARTESIAN_POINT('Ctrl Pts',(13.3181701524028,1.67885740198553,-2.75091900758608));
#65878=CARTESIAN_POINT('Ctrl Pts',(13.3243340410554,1.76382690536929,-2.69906299899206));
#65879=CARTESIAN_POINT('Ctrl Pts',(13.3304979297081,1.84651270724534,-2.64319261727962));
#65880=CARTESIAN_POINT('Ctrl Pts',(13.3366618183607,1.92651311827456,-2.58353725880159));
#65881=CARTESIAN_POINT('Ctrl Pts',(13.3428191800192,2.00642881618858,-2.5239450698897));
#65882=CARTESIAN_POINT('Ctrl Pts',(13.3489765416778,2.0836644302682,-2.46057613061492));
#65883=CARTESIAN_POINT('Ctrl Pts',(13.3551339033363,2.15784594453925,-2.39370391697376));
#65884=CARTESIAN_POINT('Ctrl Pts',(13.3612867674826,2.23197327452057,-2.32688054870107));
#65885=CARTESIAN_POINT('Ctrl Pts',(13.3674396316289,2.30305061824771,-2.25655928354203));
#65886=CARTESIAN_POINT('Ctrl Pts',(13.3735924957753,2.37073658274529,-2.18305419486856));
#65887=CARTESIAN_POINT('Ctrl Pts',(13.3797430289118,2.43839690444613,-2.10957695356436));
#65888=CARTESIAN_POINT('Ctrl Pts',(13.3858935620483,2.5026681059385,-2.03291860462162));
#65889=CARTESIAN_POINT('Ctrl Pts',(13.3920440951849,2.56324590374062,-1.95342980407716));
#65890=CARTESIAN_POINT('Ctrl Pts',(13.3981939434001,2.62381695561926,-1.87394985537916));
#65891=CARTESIAN_POINT('Ctrl Pts',(13.4043437916153,2.68069515823319,-1.79164042722443));
#65892=CARTESIAN_POINT('Ctrl Pts',(13.4104936398305,2.73361739394918,-1.70688415131153));
#65893=CARTESIAN_POINT('Ctrl Pts',(13.4166444482096,2.78654789231168,-1.62211464256488));
#65894=CARTESIAN_POINT('Ctrl Pts',(13.4227952565888,2.83552096690627,-1.53489789574915));
#65895=CARTESIAN_POINT('Ctrl Pts',(13.4289460649679,2.88031813605132,-1.44564345453291));
#65896=CARTESIAN_POINT('Ctrl Pts',(13.4351034513341,2.92516321356555,-1.35629356008153));
#65897=CARTESIAN_POINT('Ctrl Pts',(13.4412608377003,2.96582327240875,-1.2649020085423));
#65898=CARTESIAN_POINT('Ctrl Pts',(13.4474182240665,3.00212698361132,-1.17190065140899));
#65899=CARTESIAN_POINT('Ctrl Pts',(13.4535790468034,3.03845095552267,-1.07884739122357));
#65900=CARTESIAN_POINT('Ctrl Pts',(13.4597398695404,3.0704135990708,-0.984182947825881));
#65901=CARTESIAN_POINT('Ctrl Pts',(13.4659006922773,3.0978933807268,-0.888354751295375));
#65902=CARTESIAN_POINT('Ctrl Pts',(13.472071815194,3.12541910538458,-0.792366341155497));
#65903=CARTESIAN_POINT('Ctrl Pts',(13.4782429381107,3.14844689724348,-0.695210714348815));
#65904=CARTESIAN_POINT('Ctrl Pts',(13.4844140610274,3.16690625898691,-0.59734605488738));
#65905=CARTESIAN_POINT('Ctrl Pts',(13.489109582973,3.18095173164045,-0.522882191113662));
#65906=CARTESIAN_POINT('Ctrl Pts',(13.4938051049186,3.1923533799869,-0.448008056453126));
#65907=CARTESIAN_POINT('Ctrl Pts',(13.4985006268642,3.20110034742735,-0.372926438055179));
#65908=CARTESIAN_POINT('Ctrl Pts',(13.504672874957,3.21259820724514,-0.27423189859225));
#65909=CARTESIAN_POINT('Ctrl Pts',(13.5108451230497,3.21954768556084,-0.17483140442333));
#65910=CARTESIAN_POINT('Ctrl Pts',(13.5170173711425,3.22187297866149,-0.0751802625091805));
#65911=CARTESIAN_POINT('Ctrl Pts',(13.5231812597951,3.22419512248036,0.0243359159779369));
#65912=CARTESIAN_POINT('Ctrl Pts',(13.5293451484477,3.22190551905884,0.124101637048659));
#65913=CARTESIAN_POINT('Ctrl Pts',(13.5355090371004,3.21497994111518,0.223654959093386));
#65914=CARTESIAN_POINT('Ctrl Pts',(13.5416663987589,3.20806169672486,0.323102863279242));
#65915=CARTESIAN_POINT('Ctrl Pts',(13.5478237604175,3.19651726749164,0.422338384645109));
#65916=CARTESIAN_POINT('Ctrl Pts',(13.553981122076,3.18037446959469,0.520899026347988));
#65917=CARTESIAN_POINT('Ctrl Pts',(13.5601339862223,3.16424346285687,0.619387676552421));
#65918=CARTESIAN_POINT('Ctrl Pts',(13.5662868503686,3.14352083528047,0.717201999793968));
#65919=CARTESIAN_POINT('Ctrl Pts',(13.5724397145149,3.11828619350824,0.813884990570474));
#65920=CARTESIAN_POINT('Ctrl Pts',(13.5785902476515,3.09306111186852,0.910531353040098));
#65921=CARTESIAN_POINT('Ctrl Pts',(13.584740780788,3.06332752212783,1.00604681485144));
#65922=CARTESIAN_POINT('Ctrl Pts',(13.5908913139245,3.0292158700759,1.09998580671767));
#65923=CARTESIAN_POINT('Ctrl Pts',(13.5970411621397,2.99510801668623,1.19391433756891));
#65924=CARTESIAN_POINT('Ctrl Pts',(13.603191010355,2.95662321854592,1.28626633921399));
#65925=CARTESIAN_POINT('Ctrl Pts',(13.6093408585702,2.91394107845225,1.37661358187711));
#65926=CARTESIAN_POINT('Ctrl Pts',(13.6154916669493,2.87125227447843,1.46697493028086));
#65927=CARTESIAN_POINT('Ctrl Pts',(13.6216424753284,2.8243650124737,1.55533050521576));
#65928=CARTESIAN_POINT('Ctrl Pts',(13.6277932837076,2.77350566894046,1.64127507348863));
#65929=CARTESIAN_POINT('Ctrl Pts',(13.6339506700738,2.72259193384072,1.72731155525029));
#65930=CARTESIAN_POINT('Ctrl Pts',(13.6401080564399,2.66769785615239,1.81093150689242));
#65931=CARTESIAN_POINT('Ctrl Pts',(13.6462654428061,2.60909407387347,1.891757298434));
#65932=CARTESIAN_POINT('Ctrl Pts',(13.6524262655431,2.55045758545717,1.97262819797613));
#65933=CARTESIAN_POINT('Ctrl Pts',(13.6585870882801,2.48810754045786,2.05070149248175));
#65934=CARTESIAN_POINT('Ctrl Pts',(13.664747911017,2.42235460662338,2.12563301683769));
#65935=CARTESIAN_POINT('Ctrl Pts',(13.6709190339337,2.35649174152399,2.20068981799534));
#65936=CARTESIAN_POINT('Ctrl Pts',(13.6770901568504,2.28721492504014,2.2725940439905));
#65937=CARTESIAN_POINT('Ctrl Pts',(13.6832612797671,2.2148714670262,2.34103864706528));
#65938=CARTESIAN_POINT('Ctrl Pts',(13.6879568017126,2.15982633191722,2.39311719745757));
#65939=CARTESIAN_POINT('Ctrl Pts',(13.6926523236582,2.10300653040755,2.44319357694469));
#65940=CARTESIAN_POINT('Ctrl Pts',(13.6973478456038,2.04457677858076,2.49114900377081));
#65941=CARTESIAN_POINT('Ctrl Pts',(13.7035210191478,1.96775954668602,2.55419570562972));
#65942=CARTESIAN_POINT('Ctrl Pts',(13.7096941926918,1.88788818637792,2.61379695146731));
#65943=CARTESIAN_POINT('Ctrl Pts',(13.7158673662358,1.8053048747192,2.6696426487107));
#65944=CARTESIAN_POINT('Ctrl Pts',(13.7162619400855,1.80002635549901,2.67321216633289));
#65945=CARTESIAN_POINT('Ctrl Pts',(13.7166565139352,1.79473676925109,2.67676635336204));
#65946=CARTESIAN_POINT('Ctrl Pts',(13.7170510877849,1.78943621037804,2.68030513402632));
#65947=CARTESIAN_POINT('Ctrl Pts',(12.4667878339183,1.79025515774624,2.68151164616941));
#65948=CARTESIAN_POINT('Ctrl Pts',(12.4792800670008,1.62332533145098,2.79539990134072));
#65949=CARTESIAN_POINT('Ctrl Pts',(12.5580547063299,0.504984143122603,3.41174297579092));
#65950=CARTESIAN_POINT('Ctrl Pts',(12.7013163267104,-2.11419727950624,3.1526668518075));
#65951=CARTESIAN_POINT('Ctrl Pts',(12.8320857140083,-3.22555599009752,1.03940890035993));
#65952=CARTESIAN_POINT('Ctrl Pts',(12.8965726950595,-3.22797463642135,-0.000529586957199449));
#65953=CARTESIAN_POINT('Ctrl Pts',(12.2173276938518,1.78943621037674,2.68030513402719));
#65954=CARTESIAN_POINT('Ctrl Pts',(12.2175082861032,1.78700255296618,2.68192990228168));
#65955=CARTESIAN_POINT('Ctrl Pts',(12.2176890037932,1.78456668780849,2.68355135254919));
#65956=CARTESIAN_POINT('Ctrl Pts',(12.21875701983,1.77016807067626,2.69310761627513));
#65957=CARTESIAN_POINT('Ctrl Pts',(12.2196472004852,1.75815477405948,2.70096564417186));
#65958=CARTESIAN_POINT('Ctrl Pts',(12.2250259925943,1.68549892884792,2.74780050765236));
#65959=CARTESIAN_POINT('Ctrl Pts',(12.2295869497539,1.62361922962322,2.78481121793989));
#65960=CARTESIAN_POINT('Ctrl Pts',(12.2548611819108,1.27957128225792,2.97522258044692));
#65961=CARTESIAN_POINT('Ctrl Pts',(12.2770413484719,0.976938385617913,3.08784228310247));
#65962=CARTESIAN_POINT('Ctrl Pts',(12.3028501154113,0.597203166083887,3.16764182028854));
#65963=CARTESIAN_POINT('Ctrl Pts',(12.3072540220057,0.531218693434361,3.1793732465229));
#65964=CARTESIAN_POINT('Ctrl Pts',(12.313808082369,0.430516074478871,3.19405411924663));
#65965=CARTESIAN_POINT('Ctrl Pts',(12.3160224408997,0.396039253244913,3.19851199073312));
#65966=CARTESIAN_POINT('Ctrl Pts',(12.3187145772716,0.353472729569948,3.20331699578125));
#65967=CARTESIAN_POINT('Ctrl Pts',(12.319220367574,0.345446573956067,3.20419247453594));
#65968=CARTESIAN_POINT('Ctrl Pts',(12.3200130132617,0.33282143975266,3.20552161215935));
#65969=CARTESIAN_POINT('Ctrl Pts',(12.3203009943319,0.328224698168925,3.20599554973681));
#65970=CARTESIAN_POINT('Ctrl Pts',(12.3208387011516,0.319623105208247,3.20686370570056));
#65971=CARTESIAN_POINT('Ctrl Pts',(12.3210885558094,0.315618578457668,3.20726030585165));
#65972=CARTESIAN_POINT('Ctrl Pts',(12.3216547516289,0.306526683270243,3.20814355543555));
#65973=CARTESIAN_POINT('Ctrl Pts',(12.3219708302213,0.301438906653007,3.20862560393892));
#65974=CARTESIAN_POINT('Ctrl Pts',(12.3229065071985,0.286342287769512,3.21001972959777));
#65975=CARTESIAN_POINT('Ctrl Pts',(12.3235241796891,0.276330188958877,3.21089710254032));
#65976=CARTESIAN_POINT('Ctrl Pts',(12.3278762048834,0.205474301993766,3.21677241839931));
#65977=CARTESIAN_POINT('Ctrl Pts',(12.3315210053964,0.144498824347654,3.22008784208063));
#65978=CARTESIAN_POINT('Ctrl Pts',(12.3352173604744,0.0814932148166845,
3.22172008329158));
#65979=CARTESIAN_POINT('Ctrl Pts',(12.3353327651569,0.079524905079508,3.22176926992739));
#65980=CARTESIAN_POINT('Ctrl Pts',(12.3419286388201,-0.033039973876497,
3.22447896583268));
#65981=CARTESIAN_POINT('Ctrl Pts',(12.348196521495,-0.143708579799369,3.22144495746909));
#65982=CARTESIAN_POINT('Ctrl Pts',(12.370286277878,-0.535933731974559,3.19043430586768));
#65983=CARTESIAN_POINT('Ctrl Pts',(12.3858229800298,-0.813666830578774,
3.13113870813219));
#65984=CARTESIAN_POINT('Ctrl Pts',(12.4051216551378,-1.11880799765079,3.0225940186862));
#65985=CARTESIAN_POINT('Ctrl Pts',(12.4075929575794,-1.15725310287701,3.00808426725228));
#65986=CARTESIAN_POINT('Ctrl Pts',(12.4108497053235,-1.20703952530353,2.98819845331322));
#65987=CARTESIAN_POINT('Ctrl Pts',(12.4116127630578,-1.21864273442523,2.98348525904341));
#65988=CARTESIAN_POINT('Ctrl Pts',(12.4128586131186,-1.23748534121262,2.97570317989714));
#65989=CARTESIAN_POINT('Ctrl Pts',(12.4133400148783,-1.24474157267366,2.97267519249744));
#65990=CARTESIAN_POINT('Ctrl Pts',(12.4142677089574,-1.25867706710805,2.96680001379763));
#65991=CARTESIAN_POINT('Ctrl Pts',(12.4147138654395,-1.26535793858731,2.96395674175801));
#65992=CARTESIAN_POINT('Ctrl Pts',(12.4157366975768,-1.28062542218801,2.95739811729555));
#65993=CARTESIAN_POINT('Ctrl Pts',(12.4163138784503,-1.28920554775183,2.95366791444566));
#65994=CARTESIAN_POINT('Ctrl Pts',(12.4178473921346,-1.31190791460179,2.94368031182628));
#65995=CARTESIAN_POINT('Ctrl Pts',(12.4188059224268,-1.32600148793925,2.93735871068346));
#65996=CARTESIAN_POINT('Ctrl Pts',(12.4254405491666,-1.42287926716492,2.89306536762836));
#65997=CARTESIAN_POINT('Ctrl Pts',(12.4312335199165,-1.50405952672247,2.85170385571505));
#65998=CARTESIAN_POINT('Ctrl Pts',(12.4397463988756,-1.61843272684388,2.78718735086989));
#65999=CARTESIAN_POINT('Ctrl Pts',(12.4423764169247,-1.65311718939539,2.76675643553268));
#66000=CARTESIAN_POINT('Ctrl Pts',(12.4454486558068,-1.6928984282206,2.74230815045632));
#66001=CARTESIAN_POINT('Ctrl Pts',(12.4458730682651,-1.69837787511089,2.73891797483863));
#66002=CARTESIAN_POINT('Ctrl Pts',(12.4464402168789,-1.70567876064533,2.73437052803579));
#66003=CARTESIAN_POINT('Ctrl Pts',(12.4465825549347,-1.70750927934305,2.73322781341703));
#66004=CARTESIAN_POINT('Ctrl Pts',(12.4630327794531,-1.91885819176681,2.6009965345449));
#66005=CARTESIAN_POINT('Ctrl Pts',(12.4800284580523,-2.11257915185544,2.44626063872923));
#66006=CARTESIAN_POINT('Ctrl Pts',(12.5011274510788,-2.33582100310214,2.22146702915632));
#66007=CARTESIAN_POINT('Ctrl Pts',(12.5057148641371,-2.38332093199774,2.17042811416539));
#66008=CARTESIAN_POINT('Ctrl Pts',(12.5125090539377,-2.4526026338903,2.09096473464335));
#66009=CARTESIAN_POINT('Ctrl Pts',(12.5147853718186,-2.47562613251794,2.06365421292259));
#66010=CARTESIAN_POINT('Ctrl Pts',(12.5175423022222,-2.50333678607804,2.02965238877069));
#66011=CARTESIAN_POINT('Ctrl Pts',(12.518052525847,-2.50845772518312,2.02331997670889));
#66012=CARTESIAN_POINT('Ctrl Pts',(12.5188505574029,-2.51645648056312,2.01335189216453));
#66013=CARTESIAN_POINT('Ctrl Pts',(12.5191395162065,-2.51935050474163,2.0097293586838));
#66014=CARTESIAN_POINT('Ctrl Pts',(12.5196780834841,-2.52474045729685,2.00295266139086));
#66015=CARTESIAN_POINT('Ctrl Pts',(12.5199278251179,-2.52723827219303,1.99980010408442));
#66016=CARTESIAN_POINT('Ctrl Pts',(12.5204925222027,-2.5328824512004,1.99264897517752));
#66017=CARTESIAN_POINT('Ctrl Pts',(12.5208072206912,-2.53602524359466,1.98864763459287));
#66018=CARTESIAN_POINT('Ctrl Pts',(12.5217350744747,-2.54528305293136,1.97680313899963));
#66019=CARTESIAN_POINT('Ctrl Pts',(12.5223463514273,-2.55137132380825,1.968939014804));
#66020=CARTESIAN_POINT('Ctrl Pts',(12.5265510556383,-2.59316490409663,1.91443553431141));
#66021=CARTESIAN_POINT('Ctrl Pts',(12.5300616715577,-2.62762833748178,1.86685242558578));
#66022=CARTESIAN_POINT('Ctrl Pts',(12.5343011110822,-2.66835372312316,1.80725937002168));
#66023=CARTESIAN_POINT('Ctrl Pts',(12.5350869306436,-2.67586391314629,1.79612091745949));
#66024=CARTESIAN_POINT('Ctrl Pts',(12.5536417794413,-2.85219836434135,1.53103629765233));
#66025=CARTESIAN_POINT('Ctrl Pts',(12.5699677570529,-2.98421278816317,1.25443891072778));
#66026=CARTESIAN_POINT('Ctrl Pts',(12.5918475413813,-3.09771585957471,0.892106056522236));
#66027=CARTESIAN_POINT('Ctrl Pts',(12.5962104392558,-3.11755823854856,0.820076958875613));
#66028=CARTESIAN_POINT('Ctrl Pts',(12.6033328513673,-3.14534151019582,0.703547590821815));
#66029=CARTESIAN_POINT('Ctrl Pts',(12.6060421129321,-3.15488053953082,0.659455003292693));
#66030=CARTESIAN_POINT('Ctrl Pts',(12.6095675599293,-3.16596294164801,0.602464902008854));
#66031=CARTESIAN_POINT('Ctrl Pts',(12.6103564309675,-3.16835852941827,0.589736828969605));
#66032=CARTESIAN_POINT('Ctrl Pts',(12.611633967861,-3.17210205589667,0.56916556154873));
#66033=CARTESIAN_POINT('Ctrl Pts',(12.6121211061404,-3.17349779534033,0.561331123891866));
#66034=CARTESIAN_POINT('Ctrl Pts',(12.6130528239263,-3.17610683168556,0.546365519946078));
#66035=CARTESIAN_POINT('Ctrl Pts',(12.6134972398592,-3.17732516559131,0.53923527184978));
#66036=CARTESIAN_POINT('Ctrl Pts',(12.6145158354977,-3.18005779573373,0.522911833884906));
#66037=CARTESIAN_POINT('Ctrl Pts',(12.6150905155675,-3.181556245963,0.513716089953671));
#66038=CARTESIAN_POINT('Ctrl Pts',(12.6168633997489,-3.18604588195182,0.485390659530308));
#66039=CARTESIAN_POINT('Ctrl Pts',(12.6180657974757,-3.18890452245745,0.466240683068948));
#66040=CARTESIAN_POINT('Ctrl Pts',(12.6286611072834,-3.21246413851608,0.298049476772166));
#66041=CARTESIAN_POINT('Ctrl Pts',(12.6383807299955,-3.22287293526502,0.147775904085055));
#66042=CARTESIAN_POINT('Ctrl Pts',(12.663765228805,-3.22255713465583,-0.235249454019123));
#66043=CARTESIAN_POINT('Ctrl Pts',(12.6797418286628,-3.19718744435591,-0.467115696392172));
#66044=CARTESIAN_POINT('Ctrl Pts',(12.6973545232474,-3.14022827584774,-0.725326481530957));
#66045=CARTESIAN_POINT('Ctrl Pts',(12.6994649411198,-3.13290593759274,-0.756328384760312));
#66046=CARTESIAN_POINT('Ctrl Pts',(12.7061664106279,-3.1080213560631,-0.855116119409178));
#66047=CARTESIAN_POINT('Ctrl Pts',(12.710698602809,-3.08870788244638,-0.922445470318466));
#66048=CARTESIAN_POINT('Ctrl Pts',(12.7157797890273,-3.06397403567384,-0.999145703616312));
#66049=CARTESIAN_POINT('Ctrl Pts',(12.7164427695479,-3.06068433859602,-1.00917808890834));
#66050=CARTESIAN_POINT('Ctrl Pts',(12.7174245619309,-3.05571844058919,-1.02407462561977));
#66051=CARTESIAN_POINT('Ctrl Pts',(12.7177455370936,-3.05407983901003,-1.02895109933651));
#66052=CARTESIAN_POINT('Ctrl Pts',(12.7183165509912,-3.05113763585001,-1.03763813964229));
#66053=CARTESIAN_POINT('Ctrl Pts',(12.7185668551912,-3.04983856513048,-1.04145019517142));
#66054=CARTESIAN_POINT('Ctrl Pts',(12.7191020520803,-3.04704081066854,-1.04960993148744));
#66055=CARTESIAN_POINT('Ctrl Pts',(12.7193868139527,-3.04553997141236,-1.05395682706434));
#66056=CARTESIAN_POINT('Ctrl Pts',(12.720163748881,-3.04141180678738,-1.06583082306111));
#66057=CARTESIAN_POINT('Ctrl Pts',(12.7206548231636,-3.03876582559905,-1.07335147188336));
#66058=CARTESIAN_POINT('Ctrl Pts',(12.7231967010293,-3.02488057960672,-1.11235448143615));
#66059=CARTESIAN_POINT('Ctrl Pts',(12.7252211031928,-3.01317939961965,-1.14367177412547));
#66060=CARTESIAN_POINT('Ctrl Pts',(12.7310122441603,-2.97790988991909,-1.23376650135124));
#66061=CARTESIAN_POINT('Ctrl Pts',(12.7347173096923,-2.9530929661366,-1.29204104550629));
#66062=CARTESIAN_POINT('Ctrl Pts',(12.759680734869,-2.77176770798535,-1.68525484019817));
#66063=CARTESIAN_POINT('Ctrl Pts',(12.7793114816512,-2.56036699912831,-1.99181835500209));
#66064=CARTESIAN_POINT('Ctrl Pts',(12.8019968630355,-2.29458726531418,-2.26298168424145));
#66065=CARTESIAN_POINT('Ctrl Pts',(12.8025934725884,-2.28758053693351,-2.27006433941809));
#66066=CARTESIAN_POINT('Ctrl Pts',(12.8048834608465,-2.26062389562583,-2.29706154748031));
#66067=CARTESIAN_POINT('Ctrl Pts',(12.8065865111038,-2.24044630668845,-2.31674608453141));
#66068=CARTESIAN_POINT('Ctrl Pts',(12.8089813892909,-2.21190711264614,-2.34386636671604));
#66069=CARTESIAN_POINT('Ctrl Pts',(12.8096634487079,-2.20376069033802,-2.3515274684278));
#66070=CARTESIAN_POINT('Ctrl Pts',(12.8107640375246,-2.19058671461077,-2.36378802700875));
#66071=CARTESIAN_POINT('Ctrl Pts',(12.8111814165442,-2.18558411136279,-2.36841425470458));
#66072=CARTESIAN_POINT('Ctrl Pts',(12.8120477811564,-2.17518667362029,-2.37796843676708));
#66073=CARTESIAN_POINT('Ctrl Pts',(12.812496865962,-2.16978968038776,-2.38289397431717));
#66074=CARTESIAN_POINT('Ctrl Pts',(12.813550810065,-2.15710660877617,-2.39439029879254));
#66075=CARTESIAN_POINT('Ctrl Pts',(12.8141562920881,-2.14980721212989,-2.4009462242707));
#66076=CARTESIAN_POINT('Ctrl Pts',(12.8161230258421,-2.1260559839001,-2.42208314961587));
#66077=CARTESIAN_POINT('Ctrl Pts',(12.8174899098611,-2.10948514511078,-2.43652892744612));
#66078=CARTESIAN_POINT('Ctrl Pts',(12.8207007622298,-2.07041864948751,-2.46988823534968));
#66079=CARTESIAN_POINT('Ctrl Pts',(12.8225501579173,-2.04780977320846,-2.48866557014003));
#66080=CARTESIAN_POINT('Ctrl Pts',(12.8290584038212,-1.96789026682442,-2.55321459396083));
#66081=CARTESIAN_POINT('Ctrl Pts',(12.8337806385978,-1.90928009563021,-2.59733421521482));
#66082=CARTESIAN_POINT('Ctrl Pts',(12.857947290195,-1.60620693452165,-2.80967259501224));
#66083=CARTESIAN_POINT('Ctrl Pts',(12.878480093807,-1.34089305313427,-2.94552639301652));
#66084=CARTESIAN_POINT('Ctrl Pts',(12.9034549364483,-0.984193596455357,
-3.0698627342375));
#66085=CARTESIAN_POINT('Ctrl Pts',(12.9087270931367,-0.906627829442088,
-3.09365847365901));
#66086=CARTESIAN_POINT('Ctrl Pts',(12.9145348243538,-0.817651136448685,
-3.1173200401385));
#66087=CARTESIAN_POINT('Ctrl Pts',(12.915223096416,-0.807047898911263,-3.12008193972554));
#66088=CARTESIAN_POINT('Ctrl Pts',(12.9162314476559,-0.791423744262382,
-3.1240666956274));
#66089=CARTESIAN_POINT('Ctrl Pts',(12.9165538997877,-0.78641377994868,-3.12533160309534));
#66090=CARTESIAN_POINT('Ctrl Pts',(12.9171271804215,-0.777481886066626,
-3.12756387562323));
#66091=CARTESIAN_POINT('Ctrl Pts',(12.9173782784857,-0.773561162090664,
-3.1285359209158));
#66092=CARTESIAN_POINT('Ctrl Pts',(12.917910201009,-0.765237290179472,-3.13058301199037));
#66093=CARTESIAN_POINT('Ctrl Pts',(12.9181909132995,-0.760833713043868,
-3.13165613804309));
#66094=CARTESIAN_POINT('Ctrl Pts',(12.9189455068588,-0.748967689231045,
-3.13452131303299));
#66095=CARTESIAN_POINT('Ctrl Pts',(12.9194183932892,-0.74150102369259,-3.13629601537658));
#66096=CARTESIAN_POINT('Ctrl Pts',(12.9217209379303,-0.705000426156909,
-3.14483396455468));
#66097=CARTESIAN_POINT('Ctrl Pts',(12.9235297645199,-0.675878811909328,
-3.15122107232191));
#66098=CARTESIAN_POINT('Ctrl Pts',(12.9285496328213,-0.59396137430529,-3.16799974301118));
#66099=CARTESIAN_POINT('Ctrl Pts',(12.9317169560221,-0.540985953826797,
-3.17747499758863));
#66100=CARTESIAN_POINT('Ctrl Pts',(12.9395397404302,-0.40777740105488,-3.19787243648056));
#66101=CARTESIAN_POINT('Ctrl Pts',(12.9441375043166,-0.327322177920481,
-3.2071064925347));
#66102=CARTESIAN_POINT('Ctrl Pts',(12.9596418103576,-0.0527331887067016,
-3.22817949065799));
#66103=CARTESIAN_POINT('Ctrl Pts',(12.970349173668,0.142078089434734,-3.22548241986068));
#66104=CARTESIAN_POINT('Ctrl Pts',(12.9841694255106,0.382449136231198,-3.20032538366344));
#66105=CARTESIAN_POINT('Ctrl Pts',(12.9868920797059,0.42932483451619,-3.19437471686906));
#66106=CARTESIAN_POINT('Ctrl Pts',(12.9947224233249,0.56240071229516,-3.17449925429227));
#66107=CARTESIAN_POINT('Ctrl Pts',(12.9998925138557,0.648183538491109,-3.15810007989066));
#66108=CARTESIAN_POINT('Ctrl Pts',(13.0060983581657,0.748041253378878,-3.13477023988422));
#66109=CARTESIAN_POINT('Ctrl Pts',(13.00702465875,0.762867884958379,-3.13119509952796));
#66110=CARTESIAN_POINT('Ctrl Pts',(13.0085211415974,0.786691751649836,-3.12527120513962));
#66111=CARTESIAN_POINT('Ctrl Pts',(13.0090891897106,0.795705289339191,-3.1229884898045));
#66112=CARTESIAN_POINT('Ctrl Pts',(13.0101025495026,0.811731236554076,-3.11885596920034));
#66113=CARTESIAN_POINT('Ctrl Pts',(13.0105473636733,0.818747546073128,-3.1170214326257));
#66114=CARTESIAN_POINT('Ctrl Pts',(13.0114777242701,0.833384155988676,-3.1131416066481));
#66115=CARTESIAN_POINT('Ctrl Pts',(13.0119634088592,0.841003249001174,-3.11109198640883));
#66116=CARTESIAN_POINT('Ctrl Pts',(13.0132299819313,0.860815188738119,-3.10568425884255));
#66117=CARTESIAN_POINT('Ctrl Pts',(13.0140122921546,0.8729958420741,-3.10228234646362));
#66118=CARTESIAN_POINT('Ctrl Pts',(13.0174158217113,0.925741765850736,-3.08721579221525));
#66119=CARTESIAN_POINT('Ctrl Pts',(13.02006058831,0.966094190786457,-3.07482697174894));
#66120=CARTESIAN_POINT('Ctrl Pts',(13.0270512426366,1.07105559185683,-3.04033212687478));
#66121=CARTESIAN_POINT('Ctrl Pts',(13.0314372770037,1.1352229695049,-3.01695993157272));
#66122=CARTESIAN_POINT('Ctrl Pts',(13.0407209396395,1.26757227455672,-2.96393312033488));
#66123=CARTESIAN_POINT('Ctrl Pts',(13.0456268607271,1.33556806564255,-2.93392157159599));
#66124=CARTESIAN_POINT('Ctrl Pts',(13.0674644228375,1.63035628042295,-2.79143775745219));
#66125=CARTESIAN_POINT('Ctrl Pts',(13.0849315394035,1.84446838418932,-2.65482919779079));
#66126=CARTESIAN_POINT('Ctrl Pts',(13.105376225506,2.08635025638369,-2.45698717147311));
#66127=CARTESIAN_POINT('Ctrl Pts',(13.1092029600397,2.13126816163645,-2.41812746900493));
#66128=CARTESIAN_POINT('Ctrl Pts',(13.113574032838,2.18245247804216,-2.37131151562391));
#66129=CARTESIAN_POINT('Ctrl Pts',(13.1142003890212,2.18978398008975,-2.36454292618618));
#66130=CARTESIAN_POINT('Ctrl Pts',(13.11514273502,2.2008115153091,-2.35426680640552));
#66131=CARTESIAN_POINT('Ctrl Pts',(13.115460599477,2.20453077802059,-2.35078445870171));
#66132=CARTESIAN_POINT('Ctrl Pts',(13.1160282121656,2.2111717768091,-2.34453686653071));
#66133=CARTESIAN_POINT('Ctrl Pts',(13.1162782133297,2.21409659722264,-2.34177496866304));
#66134=CARTESIAN_POINT('Ctrl Pts',(13.1168151347719,2.22037786377466,-2.33582130244095));
#66135=CARTESIAN_POINT('Ctrl Pts',(13.1171019151755,2.2237325905681,-2.33262778453086));
#66136=CARTESIAN_POINT('Ctrl Pts',(13.117890030471,2.23295080522356,-2.32381458479684));
#66137=CARTESIAN_POINT('Ctrl Pts',(13.1183902129057,2.23880000208949,-2.31817990610197));
#66138=CARTESIAN_POINT('Ctrl Pts',(13.1210623798833,2.27003735635501,-2.28785967402665));
#66139=CARTESIAN_POINT('Ctrl Pts',(13.1232046344547,2.2950398326074,-2.2627779165049));
#66140=CARTESIAN_POINT('Ctrl Pts',(13.1294344400404,2.36740885795147,-2.18774555316099));
#66141=CARTESIAN_POINT('Ctrl Pts',(13.1334485802628,2.41359657849865,-2.13668157410871));
#66142=CARTESIAN_POINT('Ctrl Pts',(13.150940014997,2.61051507064295,-1.90443200673598));
#66143=CARTESIAN_POINT('Ctrl Pts',(13.1637732408591,2.74274496155342,-1.70851163527425));
#66144=CARTESIAN_POINT('Ctrl Pts',(13.1856518047563,2.92184448168582,-1.36791255785595));
#66145=CARTESIAN_POINT('Ctrl Pts',(13.1943186110963,2.98200085172074,-1.23126852975339));
#66146=CARTESIAN_POINT('Ctrl Pts',(13.2044940247293,3.039023449488,-1.07276650536422));
#66147=CARTESIAN_POINT('Ctrl Pts',(13.2056674540597,3.04540554640454,-1.05451246283088));
#66148=CARTESIAN_POINT('Ctrl Pts',(13.2074140561683,3.05461701655015,-1.02738462255336));
#66149=CARTESIAN_POINT('Ctrl Pts',(13.2079830349804,3.05757290118923,-1.01855399046954));
#66150=CARTESIAN_POINT('Ctrl Pts',(13.2089962081628,3.06275659790965,-1.00284191214116));
#66151=CARTESIAN_POINT('Ctrl Pts',(13.2094398970793,3.06499960333466,-0.995965515964025));
#66152=CARTESIAN_POINT('Ctrl Pts',(13.2103735045716,3.06966249328517,-0.981505530450563));
#66153=CARTESIAN_POINT('Ctrl Pts',(13.2108635816401,3.0720774640332,-0.973920418796821));
#66154=CARTESIAN_POINT('Ctrl Pts',(13.2121541642164,3.07835110344488,-0.953960208133823));
#66155=CARTESIAN_POINT('Ctrl Pts',(13.2129561931015,3.08216322391658,-0.941570734479675));
#66156=CARTESIAN_POINT('Ctrl Pts',(13.2165671553425,3.09893769248793,-0.885859758819815));
#66157=CARTESIAN_POINT('Ctrl Pts',(13.2194033324161,3.11106161616452,-0.842293071962168));
#66158=CARTESIAN_POINT('Ctrl Pts',(13.2270184662554,3.14083241944924,-0.725882574918161));
#66159=CARTESIAN_POINT('Ctrl Pts',(13.2318470099064,3.15686092078427,-0.652657248439238));
#66160=CARTESIAN_POINT('Ctrl Pts',(13.2567846833419,3.22539771378096,-0.277347066708537));
#66161=CARTESIAN_POINT('Ctrl Pts',(13.2780565231288,3.23714975393023,0.0305091848345442));
#66162=CARTESIAN_POINT('Ctrl Pts',(13.3027840689352,3.19802319714815,0.404466412541073));
#66163=CARTESIAN_POINT('Ctrl Pts',(13.307280548735,3.18855910661355,0.473326460270088));
#66164=CARTESIAN_POINT('Ctrl Pts',(13.3123264121893,3.17510363626401,0.552218687450564));
#66165=CARTESIAN_POINT('Ctrl Pts',(13.3129880452872,3.17328121253321,0.562596599037311));
#66166=CARTESIAN_POINT('Ctrl Pts',(13.313968233868,3.17049404139079,0.578023803150978));
#66167=CARTESIAN_POINT('Ctrl Pts',(13.3142889424863,3.16956808015658,0.583079899869845));
#66168=CARTESIAN_POINT('Ctrl Pts',(13.3148596635336,3.16789513211846,0.592093075716802));
#66169=CARTESIAN_POINT('Ctrl Pts',(13.3151099403547,3.16715282382727,0.596050979003713));
#66170=CARTESIAN_POINT('Ctrl Pts',(13.3156452784644,3.16554640269932,0.604528500378822));
#66171=CARTESIAN_POINT('Ctrl Pts',(13.3159302081776,3.16468003136645,0.609047646012802));
#66172=CARTESIAN_POINT('Ctrl Pts',(13.3167080714707,3.16228378801627,0.621403704146416));
#66173=CARTESIAN_POINT('Ctrl Pts',(13.3171999018621,3.16073445224038,0.629236875177134));
#66174=CARTESIAN_POINT('Ctrl Pts',(13.3197523144135,3.1525163661566,0.669989772137144));
#66175=CARTESIAN_POINT('Ctrl Pts',(13.3217862338167,3.14536209054367,0.702810973070717));
#66176=CARTESIAN_POINT('Ctrl Pts',(13.3276123422465,3.1231445091183,0.797590725890267));
#66177=CARTESIAN_POINT('Ctrl Pts',(13.3313419632393,3.10675349864384,0.859224269780721));
#66178=CARTESIAN_POINT('Ctrl Pts',(13.3468383578079,3.02996967264681,1.11690247681396));
#66179=CARTESIAN_POINT('Ctrl Pts',(13.3580852468134,2.95276129958134,1.30743957168383));
#66180=CARTESIAN_POINT('Ctrl Pts',(13.3801102443004,2.77202014439468,1.65426857644279));
#66181=CARTESIAN_POINT('Ctrl Pts',(13.3907933963139,2.67197953989103,1.81141134429158));
#66182=CARTESIAN_POINT('Ctrl Pts',(13.4031008725692,2.54807952088654,1.97325332152803));
#66183=CARTESIAN_POINT('Ctrl Pts',(13.4041861748634,2.53708142364502,1.98737408293258));
#66184=CARTESIAN_POINT('Ctrl Pts',(13.405833785832,2.52027974522329,2.00857945289795));
#66185=CARTESIAN_POINT('Ctrl Pts',(13.4063926473557,2.51456253198622,2.01573229442725));
#66186=CARTESIAN_POINT('Ctrl Pts',(13.407366355856,2.50457036223762,2.0281248956465));
#66187=CARTESIAN_POINT('Ctrl Pts',(13.4077806442104,2.50030923373066,2.03337577106563));
#66188=CARTESIAN_POINT('Ctrl Pts',(13.4086461804021,2.49138682586354,2.04430016451609));
#66189=CARTESIAN_POINT('Ctrl Pts',(13.4090975453754,2.48672262437183,2.04997123558883));
#66190=CARTESIAN_POINT('Ctrl Pts',(13.4101668353825,2.47564670862519,2.06334470544812));
#66191=CARTESIAN_POINT('Ctrl Pts',(13.4107854363271,2.46921839445977,2.07103320018091));
#66192=CARTESIAN_POINT('Ctrl Pts',(13.4128386636382,2.44781439087196,2.0963918467958));
#66193=CARTESIAN_POINT('Ctrl Pts',(13.414279635533,2.43268433662111,2.11393021187192));
#66194=CARTESIAN_POINT('Ctrl Pts',(13.4275582750778,2.29229789045478,2.27315930625846));
#66195=CARTESIAN_POINT('Ctrl Pts',(13.4399191301818,2.15500790329576,2.40370579156247));
#66196=CARTESIAN_POINT('Ctrl Pts',(13.4586189051824,1.93676066724341,2.5774320677658));
#66197=CARTESIAN_POINT('Ctrl Pts',(13.4646996484832,1.8641442850022,2.63042823160763));
#66198=CARTESIAN_POINT('Ctrl Pts',(13.4707798281485,1.78943605929599,2.68030523489233));
#66199=CARTESIAN_POINT('Origin',(-1.72497344927317,0.,0.));
#66200=CARTESIAN_POINT('',(14.9670297268737,1.78943621037805,2.68030513402632));
#66201=CARTESIAN_POINT('',(14.7230445264018,1.78943621037785,2.68030513402645));
#66202=CARTESIAN_POINT('',(-1.72497344927317,1.78943621037804,2.68030513402633));
#66203=CARTESIAN_POINT('',(14.1465734492221,-3.22274864077389,0.00295988007753989));
#66204=CARTESIAN_POINT('Ctrl Pts',(14.1465734492731,-3.22274864077465,0.00295987925103317));
#66205=CARTESIAN_POINT('Ctrl Pts',(14.1527116181293,-3.2228400216292,-0.0965365865984671));
#66206=CARTESIAN_POINT('Ctrl Pts',(14.1588497869856,-3.21831936874255,-0.196145750536572));
#66207=CARTESIAN_POINT('Ctrl Pts',(14.1649879558418,-3.20918300970089,-0.29540137566902));
#66208=CARTESIAN_POINT('Ctrl Pts',(14.1710741749034,-3.20012397534469,-0.39381696047922));
#66209=CARTESIAN_POINT('Ctrl Pts',(14.177160393965,-3.18652710916992,-0.49188451750038));
#66210=CARTESIAN_POINT('Ctrl Pts',(14.1832466130266,-3.16844108362263,-0.589150797429849));
#66211=CARTESIAN_POINT('Ctrl Pts',(14.1893312277177,-3.15035982567973,-0.686391437279283));
#66212=CARTESIAN_POINT('Ctrl Pts',(14.1954158424088,-3.12779184018672,-0.782830782726507));
#66213=CARTESIAN_POINT('Ctrl Pts',(14.2015004571,-3.10083725806307,-0.878023838803871));
#66214=CARTESIAN_POINT('Ctrl Pts',(14.2075851795943,-3.07388219837611,-0.973218581448363));
#66215=CARTESIAN_POINT('Ctrl Pts',(14.2136699020886,-3.04254050992401,-1.06716656333512));
#66216=CARTESIAN_POINT('Ctrl Pts',(14.2197546245829,-3.00696242124333,-1.15943717368837));
#66217=CARTESIAN_POINT('Ctrl Pts',(14.2259325310195,-2.9708394750826,-1.25312085411097));
#66218=CARTESIAN_POINT('Ctrl Pts',(14.2321104374562,-2.93034944389814,-1.34507491116444));
#66219=CARTESIAN_POINT('Ctrl Pts',(14.2382883438928,-2.88569996812181,-1.43487046679544));
#66220=CARTESIAN_POINT('Ctrl Pts',(14.2443818447686,-2.84166051518834,-1.5234391918944));
#66221=CARTESIAN_POINT('Ctrl Pts',(14.2504753456443,-2.7935748445443,-1.60990766984916));
#66222=CARTESIAN_POINT('Ctrl Pts',(14.2565688465201,-2.74168740894939,-1.69389129347441));
#66223=CARTESIAN_POINT('Ctrl Pts',(14.2627889557372,-2.68872187682301,-1.77961989548011));
#66224=CARTESIAN_POINT('Ctrl Pts',(14.2690090649543,-2.63179511432025,-1.86275882929278));
#66225=CARTESIAN_POINT('Ctrl Pts',(14.2752291741714,-2.57121110622653,-1.94293360918929));
#66226=CARTESIAN_POINT('Ctrl Pts',(14.2814492833885,-2.51062709813282,-2.02310838908579));
#66227=CARTESIAN_POINT('Ctrl Pts',(14.2876693926056,-2.44638620976731,-2.10031868870361));
#66228=CARTESIAN_POINT('Ctrl Pts',(14.2938895018227,-2.37883175388096,-2.17423021992328));
#66229=CARTESIAN_POINT('Ctrl Pts',(14.3000617499155,-2.31179710112032,-2.24757303299623));
#66230=CARTESIAN_POINT('Ctrl Pts',(14.3062339980083,-2.24124938505372,-2.31794187018767));
#66231=CARTESIAN_POINT('Ctrl Pts',(14.312406246101,-2.16748294549879,-2.38498118304356));
#66232=CARTESIAN_POINT('Ctrl Pts',(14.3185701347537,-2.09381641218971,-2.45192970059862));
#66233=CARTESIAN_POINT('Ctrl Pts',(14.3247340234063,-2.01694013862246,-2.51555736712038));
#66234=CARTESIAN_POINT('Ctrl Pts',(14.3308979120589,-1.93718726555775,-2.57554325544358));
#66235=CARTESIAN_POINT('Ctrl Pts',(14.3370552737175,-1.8575188434882,-2.63546562419976));
#66236=CARTESIAN_POINT('Ctrl Pts',(14.343212635376,-1.77498022299545,-2.69175362180343));
#66237=CARTESIAN_POINT('Ctrl Pts',(14.3493699970346,-1.68993905853801,-2.74412527792149));
#66238=CARTESIAN_POINT('Ctrl Pts',(14.3555228611809,-1.60496001056795,-2.79645868029106));
#66239=CARTESIAN_POINT('Ctrl Pts',(14.3616757253272,-1.5174824216187,-2.84488120146152));
#66240=CARTESIAN_POINT('Ctrl Pts',(14.3678285894735,-1.42790372571685,-2.88915359795632));
#66241=CARTESIAN_POINT('Ctrl Pts',(14.37397912261,-1.33835896666301,-2.93340922187394));
#66242=CARTESIAN_POINT('Ctrl Pts',(14.3801296557466,-1.24671507129056,-2.97351765296854));
#66243=CARTESIAN_POINT('Ctrl Pts',(14.3862801888831,-1.15339413842594,-3.00928555041636));
#66244=CARTESIAN_POINT('Ctrl Pts',(14.3924300370983,-1.06008359774944,-3.04504946476299));
#66245=CARTESIAN_POINT('Ctrl Pts',(14.3985798853135,-0.965096796479779,
-3.07647365099464));
#66246=CARTESIAN_POINT('Ctrl Pts',(14.4047297335287,-0.868874936119754,
-3.10341326733693));
#66247=CARTESIAN_POINT('Ctrl Pts',(14.4108805419079,-0.772638052826602,
-3.13035708970947));
#66248=CARTESIAN_POINT('Ctrl Pts',(14.417031350287,-0.675166145768034,-3.15281483435817));
#66249=CARTESIAN_POINT('Ctrl Pts',(14.4231821586661,-0.576913683691185,
-3.17069206389865));
#66250=CARTESIAN_POINT('Ctrl Pts',(14.4293395450323,-0.478556145438334,
-3.18858841225689));
#66251=CARTESIAN_POINT('Ctrl Pts',(14.4354969313985,-0.379416813419197,
-3.20189438552719));
#66252=CARTESIAN_POINT('Ctrl Pts',(14.4416543177647,-0.279958297388894,
-3.21056707050688));
#66253=CARTESIAN_POINT('Ctrl Pts',(14.4478151405016,-0.180444274635945,
-3.2192445956183));
#66254=CARTESIAN_POINT('Ctrl Pts',(14.4539759632386,-0.0806111471565075,
-3.22328366531775));
#66255=CARTESIAN_POINT('Ctrl Pts',(14.4601367859755,0.0190775352223847,
-3.2226935333894));
#66256=CARTESIAN_POINT('Ctrl Pts',(14.4663079088922,0.118932885494522,-3.22210241482903));
#66257=CARTESIAN_POINT('Ctrl Pts',(14.4724790318089,0.218642874306915,-3.216866658042));
#66258=CARTESIAN_POINT('Ctrl Pts',(14.4786501547256,0.317747990616377,-3.20704751710343));
#66259=CARTESIAN_POINT('Ctrl Pts',(14.4833456766712,0.393155700823049,-3.19957626877693));
#66260=CARTESIAN_POINT('Ctrl Pts',(14.4880411986168,0.468213306109871,-3.18945255825233));
#66261=CARTESIAN_POINT('Ctrl Pts',(14.4927367205624,0.542723155715793,-3.17672301889068));
#66262=CARTESIAN_POINT('Ctrl Pts',(14.4989089686552,0.640666106989588,-3.15999008143301));
#66263=CARTESIAN_POINT('Ctrl Pts',(14.5050812167479,0.738006872541942,-3.13869386459617));
#66264=CARTESIAN_POINT('Ctrl Pts',(14.5112534648407,0.834287209290707,-3.11288972096891));
#66265=CARTESIAN_POINT('Ctrl Pts',(14.5174173534933,0.930437147892872,-3.08712052541742));
#66266=CARTESIAN_POINT('Ctrl Pts',(14.5235812421459,1.02552909642609,-3.05685564959215));
#66267=CARTESIAN_POINT('Ctrl Pts',(14.5297451307985,1.11911295547774,-3.02220180586636));
#66268=CARTESIAN_POINT('Ctrl Pts',(14.5359024924571,1.21259771778585,-2.98758465739014));
#66269=CARTESIAN_POINT('Ctrl Pts',(14.5420598541157,1.30457716035915,-2.94858793071974));
#66270=CARTESIAN_POINT('Ctrl Pts',(14.5482172157742,1.39461529270972,-2.90536843581673));
#66271=CARTESIAN_POINT('Ctrl Pts',(14.5543700799205,1.48458765864516,-2.86218050966321));
#66272=CARTESIAN_POINT('Ctrl Pts',(14.5605229440668,1.57262114314431,-2.81477613505698));
#66273=CARTESIAN_POINT('Ctrl Pts',(14.5666758082131,1.65829959581446,-2.76336027564659));
#66274=CARTESIAN_POINT('Ctrl Pts',(14.5728263413497,1.74394558924198,-2.71196389511103));
#66275=CARTESIAN_POINT('Ctrl Pts',(14.5789768744862,1.82723795159911,-2.6565592727689));
#66276=CARTESIAN_POINT('Ctrl Pts',(14.5851274076227,1.907785809704,-2.59739694055261));
#66277=CARTESIAN_POINT('Ctrl Pts',(14.5912772558379,1.98832469802615,-2.53824119663399));
#66278=CARTESIAN_POINT('Ctrl Pts',(14.5974271040532,2.06611933963936,-2.47532883193487));
#66279=CARTESIAN_POINT('Ctrl Pts',(14.6035769522684,2.14080933018176,-2.40895267166184));
#66280=CARTESIAN_POINT('Ctrl Pts',(14.6097277606475,2.21551098192824,-2.34256614820701));
#66281=CARTESIAN_POINT('Ctrl Pts',(14.6158785690267,2.28710669509953,-2.27271504359239));
#66282=CARTESIAN_POINT('Ctrl Pts',(14.6220293774058,2.35527129222109,-2.19973059771855));
#66283=CARTESIAN_POINT('Ctrl Pts',(14.628186763772,2.42350878802674,-2.12666809856943));
#66284=CARTESIAN_POINT('Ctrl Pts',(14.6343441501382,2.48830754328356,-2.05046588472324));
#66285=CARTESIAN_POINT('Ctrl Pts',(14.6405015365044,2.54938132119157,-1.9714899040217));
#66286=CARTESIAN_POINT('Ctrl Pts',(14.6466623592413,2.61048918371497,-1.89246984767889));
#66287=CARTESIAN_POINT('Ctrl Pts',(14.6528231819783,2.66786767939096,-1.81067329726025));
#66288=CARTESIAN_POINT('Ctrl Pts',(14.6589840047153,2.72127394644741,-1.72649519862829));
#66289=CARTESIAN_POINT('Ctrl Pts',(14.665155127632,2.77476950257646,-1.6421763639971));
#66290=CARTESIAN_POINT('Ctrl Pts',(14.6713262505487,2.82427934919663,-1.55546840527507));
#66291=CARTESIAN_POINT('Ctrl Pts',(14.6774973734654,2.86960655145587,-1.46679098795348));
#66292=CARTESIAN_POINT('Ctrl Pts',(14.6821928954109,2.90409539178722,-1.39931756946389));
#66293=CARTESIAN_POINT('Ctrl Pts',(14.6868884173565,2.93616365195819,-1.33070444888417));
#66294=CARTESIAN_POINT('Ctrl Pts',(14.691583939302,2.96574368857752,-1.2611431069322));
#66295=CARTESIAN_POINT('Ctrl Pts',(14.6977561873948,3.00462654904005,-1.16970495262861));
#66296=CARTESIAN_POINT('Ctrl Pts',(14.7039284354875,3.03934513022564,-1.0763059504372));
#66297=CARTESIAN_POINT('Ctrl Pts',(14.7101006835803,3.0696982184988,-0.981361508235005));
#66298=CARTESIAN_POINT('Ctrl Pts',(14.7162645722329,3.10001019779172,-0.886545654898761));
#66299=CARTESIAN_POINT('Ctrl Pts',(14.7224284608855,3.1259683047,-0.790188931883361));
#66300=CARTESIAN_POINT('Ctrl Pts',(14.7285923495381,3.14741893326219,-0.692727667299834));
#66301=CARTESIAN_POINT('Ctrl Pts',(14.7347497111967,3.16884684757155,-0.595369605277483));
#66302=CARTESIAN_POINT('Ctrl Pts',(14.7409070728552,3.18577667986992,-0.496909748861693));
#66303=CARTESIAN_POINT('Ctrl Pts',(14.7470644345138,3.19810459557383,-0.397799645889211));
#66304=CARTESIAN_POINT('Ctrl Pts',(14.7532172986601,3.21042350661716,-0.298761935757283));
#66305=CARTESIAN_POINT('Ctrl Pts',(14.7593701628064,3.21814713059089,-0.199075353121563));
#66306=CARTESIAN_POINT('Ctrl Pts',(14.7655230269527,3.22122286796484,-0.0992007933454522));
#66307=CARTESIAN_POINT('Ctrl Pts',(14.7716735600892,3.22429744009709,0.000635928999288105));
#66308=CARTESIAN_POINT('Ctrl Pts',(14.7778240932258,3.22272761107258,0.100660053293039));
#66309=CARTESIAN_POINT('Ctrl Pts',(14.7839746263623,3.21651278145447,0.200407308349853));
#66310=CARTESIAN_POINT('Ctrl Pts',(14.7901244745775,3.21029864391772,0.300143455585391));
#66311=CARTESIAN_POINT('Ctrl Pts',(14.7962743227927,3.19944056119897,0.399602361347613));
#66312=CARTESIAN_POINT('Ctrl Pts',(14.8024241710079,3.18398998614359,0.498322516687104));
#66313=CARTESIAN_POINT('Ctrl Pts',(14.8085749793871,3.16853699881972,0.597058085013978));
#66314=CARTESIAN_POINT('Ctrl Pts',(14.8147257877662,3.14849016215056,0.695054244632298));
#66315=CARTESIAN_POINT('Ctrl Pts',(14.8208765961454,3.12395229130314,0.791858348545924));
#66316=CARTESIAN_POINT('Ctrl Pts',(14.8270339825116,3.09938817840969,0.88876597968758));
#66317=CARTESIAN_POINT('Ctrl Pts',(14.8331913688777,3.07032354730051,0.984478587511042));
#66318=CARTESIAN_POINT('Ctrl Pts',(14.8393487552439,3.03691146539358,1.0785575153236));
#66319=CARTESIAN_POINT('Ctrl Pts',(14.8455095779809,3.00348073656488,1.17268894756889));
#66320=CARTESIAN_POINT('Ctrl Pts',(14.8516704007179,2.96569788932944,1.26518448195395));
#66321=CARTESIAN_POINT('Ctrl Pts',(14.8578312234548,2.92376383782047,1.35562626971939));
#66322=CARTESIAN_POINT('Ctrl Pts',(14.8640023463715,2.88175967745015,1.44621926564458));
#66323=CARTESIAN_POINT('Ctrl Pts',(14.8701734692882,2.83559065065569,1.53475127106041));
#66324=CARTESIAN_POINT('Ctrl Pts',(14.8763445922049,2.78550329909836,1.62082970518563));
#66325=CARTESIAN_POINT('Ctrl Pts',(14.8810401141505,2.74739252710284,1.68632559336259));
#66326=CARTESIAN_POINT('Ctrl Pts',(14.8857356360961,2.70701419507206,1.75040151652101));
#66327=CARTESIAN_POINT('Ctrl Pts',(14.8904311580417,2.66449280281853,1.81289703685241));
#66328=CARTESIAN_POINT('Ctrl Pts',(14.896814372111,2.60668812158707,1.89785506479306));
#66329=CARTESIAN_POINT('Ctrl Pts',(14.9031975861804,2.54471076740869,1.98020031839695));
#66330=CARTESIAN_POINT('Ctrl Pts',(14.9095808002497,2.4788277800295,2.05949760850894));
#66331=CARTESIAN_POINT('Ctrl Pts',(14.9157437809061,2.41521788501559,2.13605898648471));
#66332=CARTESIAN_POINT('Ctrl Pts',(14.9219067615624,2.34796770090169,2.20977885970649));
#66333=CARTESIAN_POINT('Ctrl Pts',(14.9280697422188,2.27736254300406,2.28029327285375));
#66334=CARTESIAN_POINT('Ctrl Pts',(14.93422696709,2.20682332529757,2.35074183055902));
#66335=CARTESIAN_POINT('Ctrl Pts',(14.9403841919612,2.1329356642205,2.41799057041968));
#66336=CARTESIAN_POINT('Ctrl Pts',(14.9465414168324,2.05602455353546,2.48170920894437));
#66337=CARTESIAN_POINT('Ctrl Pts',(14.9526938749316,1.97917298553922,2.54537851806749));
#66338=CARTESIAN_POINT('Ctrl Pts',(14.9588463330308,1.89930295711581,2.60552288544783));
#66339=CARTESIAN_POINT('Ctrl Pts',(14.9649987911301,1.81677481890174,2.66185026248746));
#66340=CARTESIAN_POINT('Ctrl Pts',(14.9656757697113,1.80769393106497,2.66804817999905));
#66341=CARTESIAN_POINT('Ctrl Pts',(14.9663527482925,1.79858089349769,2.67419992350421));
#66342=CARTESIAN_POINT('Ctrl Pts',(14.9670297268737,1.78943621037805,2.68030513402632));
#66343=CARTESIAN_POINT('Ctrl Pts',(13.7170510877849,1.78943621037804,2.68030513402632));
#66344=CARTESIAN_POINT('Ctrl Pts',(13.7232145029839,1.70663917467239,2.73558242761607));
#66345=CARTESIAN_POINT('Ctrl Pts',(13.729377918183,1.62116213230005,2.78709722951691));
#66346=CARTESIAN_POINT('Ctrl Pts',(13.735541333382,1.53338255777923,2.8345820669013));
#66347=CARTESIAN_POINT('Ctrl Pts',(13.7416983388329,1.44569427111637,2.88201752162333));
#66348=CARTESIAN_POINT('Ctrl Pts',(13.7478553442837,1.35570859301182,2.92543113856176));
#66349=CARTESIAN_POINT('Ctrl Pts',(13.7540123497345,1.26383127914569,2.96459913990964));
#66350=CARTESIAN_POINT('Ctrl Pts',(13.7601650149657,1.1720187317849,3.00373953080112));
#66351=CARTESIAN_POINT('Ctrl Pts',(13.7663176801968,1.07831759813188,3.03864008627275));
#66352=CARTESIAN_POINT('Ctrl Pts',(13.772470345428,0.983156677035549,3.06912373665521));
#66353=CARTESIAN_POINT('Ctrl Pts',(13.7786207852646,0.88803017526618,3.09959636122248));
#66354=CARTESIAN_POINT('Ctrl Pts',(13.7847712251012,0.79144534845544,3.1256551227528));
#66355=CARTESIAN_POINT('Ctrl Pts',(13.7909216649377,0.693848494545505,3.14717203678428));
#66356=CARTESIAN_POINT('Ctrl Pts',(13.7970715253643,0.596260834872262,3.16868692378731));
#66357=CARTESIAN_POINT('Ctrl Pts',(13.8032213857908,0.497661761876166,3.18566072054238));
#66358=CARTESIAN_POINT('Ctrl Pts',(13.8093712462173,0.39850918345149,3.19801625905886));
#66359=CARTESIAN_POINT('Ctrl Pts',(13.8155221722997,0.299339423737481,3.21037393855932));
#66360=CARTESIAN_POINT('Ctrl Pts',(13.8216730983822,0.199616399148244,3.21811171650219));
#66361=CARTESIAN_POINT('Ctrl Pts',(13.8278240244646,0.0998035720947606,
3.22120424833588));
#66362=CARTESIAN_POINT('Ctrl Pts',(13.8339815866838,-0.000116941437965382,
3.22430011665322));
#66363=CARTESIAN_POINT('Ctrl Pts',(13.840139148903,-0.100127015923435,3.22274071845078));
#66364=CARTESIAN_POINT('Ctrl Pts',(13.8462967111223,-0.199762881389789,
3.21655286816785));
#66365=CARTESIAN_POINT('Ctrl Pts',(13.852457804526,-0.299455885154504,3.21036146933107));
#66366=CARTESIAN_POINT('Ctrl Pts',(13.8586188979298,-0.398773820829627,
3.19953637987179));
#66367=CARTESIAN_POINT('Ctrl Pts',(13.8647799913335,-0.497259817801285,
3.18415612621307));
#66368=CARTESIAN_POINT('Ctrl Pts',(13.87095126572,-0.595908559299551,3.16875045724479));
#66369=CARTESIAN_POINT('Ctrl Pts',(13.8771225401064,-0.693722190827123,
3.1487746774174));
#66370=CARTESIAN_POINT('Ctrl Pts',(13.8832938144928,-0.790255683867928,
3.12435809673194));
#66371=CARTESIAN_POINT('Ctrl Pts',(13.8875942311097,-0.857524486316286,
3.10734354467486));
#66372=CARTESIAN_POINT('Ctrl Pts',(13.8918946477266,-0.92417195614628,3.08817363542435));
#66373=CARTESIAN_POINT('Ctrl Pts',(13.8961950643434,-0.990053149394673,
3.06690598549641));
#66374=CARTESIAN_POINT('Ctrl Pts',(13.9023673124362,-1.08461028318089,3.03638121931658));
#66375=CARTESIAN_POINT('Ctrl Pts',(13.908539560529,-1.17792084127548,3.00142562980689));
#66376=CARTESIAN_POINT('Ctrl Pts',(13.9147118086217,-1.26953915206813,2.96215933127611));
#66377=CARTESIAN_POINT('Ctrl Pts',(13.9208756972744,-1.36103337877134,2.92294621341257));
#66378=CARTESIAN_POINT('Ctrl Pts',(13.927039585927,-1.45083951786046,2.87943416029511));
#66379=CARTESIAN_POINT('Ctrl Pts',(13.9332034745796,-1.53852728006174,2.83179296047678));
#66380=CARTESIAN_POINT('Ctrl Pts',(13.9393608362382,-1.62612218894626,2.78420220832989));
#66381=CARTESIAN_POINT('Ctrl Pts',(13.9455181978967,-1.71160280099547,2.73249120842891));
#66382=CARTESIAN_POINT('Ctrl Pts',(13.9516755595552,-1.79455993366075,2.67687732386068));
#66383=CARTESIAN_POINT('Ctrl Pts',(13.9578284237016,-1.8774564720748,2.6213040612569));
#66384=CARTESIAN_POINT('Ctrl Pts',(13.9639812878479,-1.95783283603126,2.56183382296913));
#66385=CARTESIAN_POINT('Ctrl Pts',(13.9701341519942,-2.03530634521766,2.49872880553627));
#66386=CARTESIAN_POINT('Ctrl Pts',(13.9762846851307,-2.11275050360052,2.43564769541042));
#66387=CARTESIAN_POINT('Ctrl Pts',(13.9824352182672,-2.1872936559862,2.36893481632169));
#66388=CARTESIAN_POINT('Ctrl Pts',(13.9885857514038,-2.2585846373055,2.29889386415023));
#66389=CARTESIAN_POINT('Ctrl Pts',(13.994735599619,-2.32986767968476,2.22886071171598));
#66390=CARTESIAN_POINT('Ctrl Pts',(14.0008854478342,-2.39789896117152,2.15550052745351));
#66391=CARTESIAN_POINT('Ctrl Pts',(14.0070352960494,-2.4623635036378,2.07915452490972));
#66392=CARTESIAN_POINT('Ctrl Pts',(14.0131861044285,-2.52683811082871,2.00279660261188));
#66393=CARTESIAN_POINT('Ctrl Pts',(14.0193369128077,-2.58774459265207,1.92345226801713));
#66394=CARTESIAN_POINT('Ctrl Pts',(14.0254877211868,-2.64480831446049,1.84149573506448));
#66395=CARTESIAN_POINT('Ctrl Pts',(14.031645107553,-2.70193306311283,1.75945155363069));
#66396=CARTESIAN_POINT('Ctrl Pts',(14.0378024939192,-2.75520659652984,1.67478995244602));
#66397=CARTESIAN_POINT('Ctrl Pts',(14.0439598802854,-2.80439777096574,1.58791394751176));
#66398=CARTESIAN_POINT('Ctrl Pts',(14.0501207030223,-2.85361639846433,1.50098945801829));
#66399=CARTESIAN_POINT('Ctrl Pts',(14.0562815257593,-2.89874793352452,1.41184849117653));
#66400=CARTESIAN_POINT('Ctrl Pts',(14.0624423484963,-2.93960829835813,1.32091658128892));
#66401=CARTESIAN_POINT('Ctrl Pts',(14.068613471413,-2.98053697697379,1.22983264381422));
#66402=CARTESIAN_POINT('Ctrl Pts',(14.0747845943296,-3.01718006214866,1.13695218662884));
#66403=CARTESIAN_POINT('Ctrl Pts',(14.0809557172463,-3.04940245795269,1.04271866384566));
#66404=CARTESIAN_POINT('Ctrl Pts',(14.0856512391919,-3.07392003257883,0.971017681672536));
#66405=CARTESIAN_POINT('Ctrl Pts',(14.0903467611375,-3.09587927461857,0.898533715754632));
#66406=CARTESIAN_POINT('Ctrl Pts',(14.0950422830831,-3.11524052904747,0.825465934294087));
#66407=CARTESIAN_POINT('Ctrl Pts',(14.103012046215,-3.14810260775223,0.701447152662187));
#66408=CARTESIAN_POINT('Ctrl Pts',(14.1109818093469,-3.17357360472713,0.575393662707508));
#66409=CARTESIAN_POINT('Ctrl Pts',(14.1189515724789,-3.1914490294726,0.448074385318351));
#66410=CARTESIAN_POINT('Ctrl Pts',(14.1267580871456,-3.20895830335422,0.323363049506169));
#66411=CARTESIAN_POINT('Ctrl Pts',(14.1345646018123,-3.21918000356653,0.197437022552735));
#66412=CARTESIAN_POINT('Ctrl Pts',(14.142371116479,-3.22196690437122,0.0710410419164153));
#66413=CARTESIAN_POINT('Ctrl Pts',(14.14377189406,-3.22246697749405,0.0483609261964654));
#66414=CARTESIAN_POINT('Ctrl Pts',(14.1451726716411,-3.22272778695068,0.0256657426919609));
#66415=CARTESIAN_POINT('Ctrl Pts',(14.1465734492221,-3.22274864077389,0.00295988007751842));
#66416=CARTESIAN_POINT('',(13.9029341371857,-3.2227499320172,-0.000661954035870993));
#66417=CARTESIAN_POINT('Ctrl Pts',(13.4707798281485,1.78943605929599,2.68030523489233));
#66418=CARTESIAN_POINT('Ctrl Pts',(13.475472116723,1.73178109296317,2.71879707321372));
#66419=CARTESIAN_POINT('Ctrl Pts',(13.4801636509946,1.67288025823499,2.75543124047819));
#66420=CARTESIAN_POINT('Ctrl Pts',(13.493465968281,1.50136856300259,2.85457222591761));
#66421=CARTESIAN_POINT('Ctrl Pts',(13.5019812961287,1.38613982879161,2.91226967971131));
#66422=CARTESIAN_POINT('Ctrl Pts',(13.5107900562878,1.25789466570531,2.96714232882057));
#66423=CARTESIAN_POINT('Ctrl Pts',(13.5114645950295,1.24801312210909,2.97131214182194));
#66424=CARTESIAN_POINT('Ctrl Pts',(13.5124674222476,1.23322790220917,2.9774644371597));
#66425=CARTESIAN_POINT('Ctrl Pts',(13.5127979037898,1.22833998453966,2.97948425346831));
#66426=CARTESIAN_POINT('Ctrl Pts',(13.5133653525216,1.21992019566557,2.98293929071808));
#66427=CARTESIAN_POINT('Ctrl Pts',(13.5136026679237,1.21639072845848,2.98438028608694));
#66428=CARTESIAN_POINT('Ctrl Pts',(13.5140898232778,1.20912847488498,2.98733026366069));
#66429=CARTESIAN_POINT('Ctrl Pts',(13.5143396153137,1.2053954191628,2.98883851296559));
#66430=CARTESIAN_POINT('Ctrl Pts',(13.5149316619497,1.19652569748437,2.99240278539666));
#66431=CARTESIAN_POINT('Ctrl Pts',(13.515273539967,1.19138651387857,2.99445259612165));
#66432=CARTESIAN_POINT('Ctrl Pts',(13.515998713832,1.18044934496868,2.9987823729667));
#66433=CARTESIAN_POINT('Ctrl Pts',(13.5163817990303,1.17464996508667,3.00105878607369));
#66434=CARTESIAN_POINT('Ctrl Pts',(13.5174238949676,1.15881634818069,3.00722097907478));
#66435=CARTESIAN_POINT('Ctrl Pts',(13.518080993253,1.14876909012087,3.01107338514536));
#66436=CARTESIAN_POINT('Ctrl Pts',(13.5235938274091,1.06396343499389,3.04310403401477));
#66437=CARTESIAN_POINT('Ctrl Pts',(13.5283005706941,0.988193594633139,3.06854624511862));
#66438=CARTESIAN_POINT('Ctrl Pts',(13.5420905676021,0.759304431918389,3.13604347317865));
#66439=CARTESIAN_POINT('Ctrl Pts',(13.5508994701619,0.603940597876467,3.16963309849849));
#66440=CARTESIAN_POINT('Ctrl Pts',(13.5730984713102,0.21075901405121,3.22466578552728));
#66441=CARTESIAN_POINT('Ctrl Pts',(13.5865532958815,-0.0281045624538035,
3.23142020954005));
#66442=CARTESIAN_POINT('Ctrl Pts',(13.6021255296921,-0.285069768765774,
3.21017722171395));
#66443=CARTESIAN_POINT('Ctrl Pts',(13.6033160245126,-0.304609100386139,
3.20838212148868));
#66444=CARTESIAN_POINT('Ctrl Pts',(13.6050770586258,-0.33335060441998,3.20547669094511));
#66445=CARTESIAN_POINT('Ctrl Pts',(13.60564323057,-0.342566575631864,3.20450488844888));
#66446=CARTESIAN_POINT('Ctrl Pts',(13.6066544443938,-0.358982585442898,
3.20270223336299));
#66447=CARTESIAN_POINT('Ctrl Pts',(13.6070989962349,-0.36618428238834,3.20188681283525));
#66448=CARTESIAN_POINT('Ctrl Pts',(13.6080300358674,-0.381235016701606,
3.2001312341273));
#66449=CARTESIAN_POINT('Ctrl Pts',(13.6085166662575,-0.389083459426482,
3.19918647681224));
#66450=CARTESIAN_POINT('Ctrl Pts',(13.609788412441,-0.409546387809323,3.1966468349702));
#66451=CARTESIAN_POINT('Ctrl Pts',(13.6105749716476,-0.422154958041425,
3.19500616826451));
#66452=CARTESIAN_POINT('Ctrl Pts',(13.6140221714417,-0.477202963293567,
3.18751161019373));
#66453=CARTESIAN_POINT('Ctrl Pts',(13.6167071135228,-0.51953136647452,3.180886638509));
#66454=CARTESIAN_POINT('Ctrl Pts',(13.6238275203275,-0.6303054192645,3.16127899633989));
#66455=CARTESIAN_POINT('Ctrl Pts',(13.6283050005167,-0.698481106291388,
3.14691798264134));
#66456=CARTESIAN_POINT('Ctrl Pts',(13.6447324808073,-0.943339291470875,
3.08699063100358));
#66457=CARTESIAN_POINT('Ctrl Pts',(13.6570369473876,-1.11652416412197,3.0286565524379));
#66458=CARTESIAN_POINT('Ctrl Pts',(13.6755877892468,-1.36790432791554,2.91947908262879));
#66459=CARTESIAN_POINT('Ctrl Pts',(13.6817895632028,-1.45038972070421,2.87939072543201));
#66460=CARTESIAN_POINT('Ctrl Pts',(13.6951250068285,-1.62612411582044,2.78451258837201));
#66461=CARTESIAN_POINT('Ctrl Pts',(13.7022196045532,-1.71856270516239,2.72843133565982));
#66462=CARTESIAN_POINT('Ctrl Pts',(13.7097749313434,-1.81763559166391,2.66128791999342));
#66463=CARTESIAN_POINT('Ctrl Pts',(13.7105051270001,-1.82721776355131,2.65471802484882));
#66464=CARTESIAN_POINT('Ctrl Pts',(13.7115629374804,-1.84111281487212,2.64508018245146));
#66465=CARTESIAN_POINT('Ctrl Pts',(13.7118932661591,-1.84545386263266,2.64205329441554));
#66466=CARTESIAN_POINT('Ctrl Pts',(13.7124683645968,-1.85301537392027,2.63675314071104));
#66467=CARTESIAN_POINT('Ctrl Pts',(13.712713459211,-1.85623914591273,2.63448464313061));
#66468=CARTESIAN_POINT('Ctrl Pts',(13.7129589099059,-1.85946888746914,2.63220307331843));
#66469=CARTESIAN_POINT('Ctrl Pts',(13.7129596769703,-1.85947898083185,2.63219594302911));
#66470=CARTESIAN_POINT('Ctrl Pts',(13.7129612068001,-1.85949911101411,2.63218172221995));
#66471=CARTESIAN_POINT('Ctrl Pts',(13.7129619675692,-1.85950912156391,2.63217465026007));
#66472=CARTESIAN_POINT('Ctrl Pts',(13.7129634823091,-1.85952905323436,2.63216056934711));
#66473=CARTESIAN_POINT('Ctrl Pts',(13.7129642362126,-1.85953897346787,2.63215356102232));
#66474=CARTESIAN_POINT('Ctrl Pts',(13.7129657373464,-1.85955872615025,2.63213960622233));
#66475=CARTESIAN_POINT('Ctrl Pts',(13.7129664844812,-1.85956855734053,2.63213266063782));
#66476=CARTESIAN_POINT('Ctrl Pts',(13.7129679721254,-1.85958813256602,2.63211883087806));
#66477=CARTESIAN_POINT('Ctrl Pts',(13.7129687125591,-1.85959787560478,2.6321119474083));
#66478=CARTESIAN_POINT('Ctrl Pts',(13.7129701868977,-1.85961727579403,2.63209824098743));
#66479=CARTESIAN_POINT('Ctrl Pts',(13.7129709207116,-1.85962693174755,2.63209141888347));
#66480=CARTESIAN_POINT('Ctrl Pts',(13.7129723819031,-1.85964615898363,2.63207783433844));
#66481=CARTESIAN_POINT('Ctrl Pts',(13.7129731091826,-1.85965572897624,2.6320710728102));
#66482=CARTESIAN_POINT('Ctrl Pts',(13.7129745573532,-1.85967478492103,2.63205760897531));
#66483=CARTESIAN_POINT('Ctrl Pts',(13.7129752781642,-1.85968426981796,2.63205090741566));
#66484=CARTESIAN_POINT('Ctrl Pts',(13.712976713489,-1.85970315677204,2.63203756267377));
#66485=CARTESIAN_POINT('Ctrl Pts',(13.7129774279097,-1.85971255760438,2.63203092035831));
#66486=CARTESIAN_POINT('Ctrl Pts',(13.7129788505282,-1.8597312774026,2.6320176934211));
#66487=CARTESIAN_POINT('Ctrl Pts',(13.7129795586303,-1.85974059511145,2.63201110968891));
#66488=CARTESIAN_POINT('Ctrl Pts',(13.7129809687011,-1.85975914984145,2.63199799908929));
#66489=CARTESIAN_POINT('Ctrl Pts',(13.7129816705651,-1.85976838548415,2.6319914731972));
#66490=CARTESIAN_POINT('Ctrl Pts',(13.712983068205,-1.85978677667963,2.63197847785927));
#66491=CARTESIAN_POINT('Ctrl Pts',(13.7129837638899,-1.85979593103509,2.63197200926078));
#66492=CARTESIAN_POINT('Ctrl Pts',(13.7129851492796,-1.85981416107415,2.63195912751181));
#66493=CARTESIAN_POINT('Ctrl Pts',(13.7129858388699,-1.85982323525057,2.63195271542762));
#66494=CARTESIAN_POINT('Ctrl Pts',(13.7129872121093,-1.85984130544608,2.63193994634741));
#66495=CARTESIAN_POINT('Ctrl Pts',(13.7129878956613,-1.85985030018644,2.63193359025623));
#66496=CARTESIAN_POINT('Ctrl Pts',(13.7129892569308,-1.85986821291092,2.63192093217559));
#66497=CARTESIAN_POINT('Ctrl Pts',(13.7129899345292,-1.85987712932796,2.63191463129474));
#66498=CARTESIAN_POINT('Ctrl Pts',(13.7129912839212,-1.85989488579754,2.6319020833615));
#66499=CARTESIAN_POINT('Ctrl Pts',(13.7129919556219,-1.85990372462671,2.63189583717484));
#66500=CARTESIAN_POINT('Ctrl Pts',(13.7129932932905,-1.85992132686555,2.63188339796564));
#66501=CARTESIAN_POINT('Ctrl Pts',(13.7129939591565,-1.85993008893525,2.63187720589124));
#66502=CARTESIAN_POINT('Ctrl Pts',(13.7129952852474,-1.85994753886252,2.63186487405676));
#66503=CARTESIAN_POINT('Ctrl Pts',(13.7129959453508,-1.85995622512023,2.63185873542847));
#66504=CARTESIAN_POINT('Ctrl Pts',(13.7129972599885,-1.85997352437223,2.63184650981911));
#66505=CARTESIAN_POINT('Ctrl Pts',(13.7129979144007,-1.85998213575863,2.63184042397549));
#66506=CARTESIAN_POINT('Ctrl Pts',(13.7129992176853,-1.85999928565061,2.63182830366839));
#66507=CARTESIAN_POINT('Ctrl Pts',(13.7129998664553,-1.86000782280877,2.63182227015828));
#66508=CARTESIAN_POINT('Ctrl Pts',(13.7130011585583,-1.86002482559782,2.63181025356479));
#66509=CARTESIAN_POINT('Ctrl Pts',(13.7130018017641,-1.86003328955411,2.63180427166603));
#66510=CARTESIAN_POINT('Ctrl Pts',(13.7130030827644,-1.86005014627723,2.63179235805966));
#66511=CARTESIAN_POINT('Ctrl Pts',(13.7130037204523,-1.8600585376403,2.63178642734525));
#66512=CARTESIAN_POINT('Ctrl Pts',(13.7130049905155,-1.86007525047453,2.63177461519362));
#66513=CARTESIAN_POINT('Ctrl Pts',(13.7130056227575,-1.86008357019278,2.63176873499637));
#66514=CARTESIAN_POINT('Ctrl Pts',(13.7130068819857,-1.86010014048178,2.63175702335595));
#66515=CARTESIAN_POINT('Ctrl Pts',(13.713007508845,-1.86010838938452,2.63175119309275));
#66516=CARTESIAN_POINT('Ctrl Pts',(13.7130087573378,-1.86012481843846,2.63173958104355));
#66517=CARTESIAN_POINT('Ctrl Pts',(13.7130093788593,-1.86013299711738,2.63173380029919));
#66518=CARTESIAN_POINT('Ctrl Pts',(13.7130106167791,-1.86014928707204,2.63172228633755));
#66519=CARTESIAN_POINT('Ctrl Pts',(13.7130112330371,-1.8601573965026,2.63171655442548));
#66520=CARTESIAN_POINT('Ctrl Pts',(13.7130123086086,-1.86017155012259,2.63170655025804));
#66521=CARTESIAN_POINT('Ctrl Pts',(13.713012767825,-1.86017759302839,2.63170227893443));
#66522=CARTESIAN_POINT('Ctrl Pts',(13.713013677046,-1.86018955763162,2.63169382190114));
#66523=CARTESIAN_POINT('Ctrl Pts',(13.7130141332754,-1.86019556124156,2.63168957829215));
#66524=CARTESIAN_POINT('Ctrl Pts',(13.7130150448454,-1.86020755677272,2.63168109927472));
#66525=CARTESIAN_POINT('Ctrl Pts',(13.7130155001755,-1.86021354855704,2.63167686396316));
#66526=CARTESIAN_POINT('Ctrl Pts',(13.7130164099625,-1.86022552064425,2.6316684013944));
#66527=CARTESIAN_POINT('Ctrl Pts',(13.7130168643996,-1.86023150068554,2.63166417432223));
#66528=CARTESIAN_POINT('Ctrl Pts',(13.7130177724066,-1.86024344936588,2.63165572817666));
#66529=CARTESIAN_POINT('Ctrl Pts',(13.7130182259544,-1.8602494177128,2.63165150930987));
#66530=CARTESIAN_POINT('Ctrl Pts',(13.7130191321948,-1.86026134316285,2.63164307946337));
#66531=CARTESIAN_POINT('Ctrl Pts',(13.7130195848623,-1.86026729993606,2.631638868717));
#66532=CARTESIAN_POINT('Ctrl Pts',(13.7130204893233,-1.8602792019874,2.63163045528935));
#66533=CARTESIAN_POINT('Ctrl Pts',(13.7130209411047,-1.86028514710763,2.6316262527198));
#66534=CARTESIAN_POINT('Ctrl Pts',(13.7130218438284,-1.86029702631449,2.63161785531991));
#66535=CARTESIAN_POINT('Ctrl Pts',(13.7130222947422,-1.86030296002579,2.63161366075501));
#66536=CARTESIAN_POINT('Ctrl Pts',(13.7130231956894,-1.86031481587198,2.63160527974848));
#66537=CARTESIAN_POINT('Ctrl Pts',(13.7130236457219,-1.86032073799564,2.63160109331491));
#66538=CARTESIAN_POINT('Ctrl Pts',(13.7130245449389,-1.8603325710911,2.63159272827128));
#66539=CARTESIAN_POINT('Ctrl Pts',(13.7130249940981,-1.8603384817295,2.63158854989702));
#66540=CARTESIAN_POINT('Ctrl Pts',(13.7130258915968,-1.86035029223039,2.63158020070656));
#66541=CARTESIAN_POINT('Ctrl Pts',(13.7130263398986,-1.86035619159505,2.63157603024242));
#66542=CARTESIAN_POINT('Ctrl Pts',(13.7130272356506,-1.86036797912614,2.63156769717111));
#66543=CARTESIAN_POINT('Ctrl Pts',(13.7130276830874,-1.86037386711608,2.63156353468882));
#66544=CARTESIAN_POINT('Ctrl Pts',(13.7133048829,-1.86402164702195,2.62898473826822));
#66545=CARTESIAN_POINT('Ctrl Pts',(13.7135811096231,-1.8676582163532,2.62640252856947));
#66546=CARTESIAN_POINT('Ctrl Pts',(13.7141487305406,-1.87513398028595,2.62107085310928));
#66547=CARTESIAN_POINT('Ctrl Pts',(13.7144400617531,-1.87897251860471,2.61832048000925));
#66548=CARTESIAN_POINT('Ctrl Pts',(13.7151681126134,-1.88856873985323,2.61141266595074));
#66549=CARTESIAN_POINT('Ctrl Pts',(13.7156041177429,-1.89431878584141,2.60724458707641));
#66550=CARTESIAN_POINT('Ctrl Pts',(13.7168323983563,-1.91052450261047,2.59541551514139));
#66551=CARTESIAN_POINT('Ctrl Pts',(13.7176217835708,-1.92094793331699,2.58771030476677));
#66552=CARTESIAN_POINT('Ctrl Pts',(13.720216106041,-1.95521892891283,2.56205530311659));
#66553=CARTESIAN_POINT('Ctrl Pts',(13.722004327061,-1.97886434183239,2.54383656871033));
#66554=CARTESIAN_POINT('Ctrl Pts',(13.7296389589279,-2.07969913920053,2.46388662809098));
#66555=CARTESIAN_POINT('Ctrl Pts',(13.735309721038,-2.15428497136974,2.39894669424279));
#66556=CARTESIAN_POINT('Ctrl Pts',(13.7593860216655,-2.4620357535809,2.10504768684837));
#66557=CARTESIAN_POINT('Ctrl Pts',(13.7770964017509,-2.66259972762664,1.84483235428617));
#66558=CARTESIAN_POINT('Ctrl Pts',(13.7969862789744,-2.82320412401723,1.55424079467385));
#66559=CARTESIAN_POINT('Ctrl Pts',(13.7973059838386,-2.82577086204425,1.54956929771163));
#66560=CARTESIAN_POINT('Ctrl Pts',(13.7992709366899,-2.84145546747076,1.52085454470699));
#66561=CARTESIAN_POINT('Ctrl Pts',(13.8009262495942,-2.85427766985789,1.49665180732512));
#66562=CARTESIAN_POINT('Ctrl Pts',(13.8032646468596,-2.87183683464052,1.46246122029424));
#66563=CARTESIAN_POINT('Ctrl Pts',(13.8039385673435,-2.87683350937794,1.45260751072356));
#66564=CARTESIAN_POINT('Ctrl Pts',(13.8050294551156,-2.88481835889024,1.43665816459803));
#66565=CARTESIAN_POINT('Ctrl Pts',(13.8054453106767,-2.88783814294646,1.43057838118803));
#66566=CARTESIAN_POINT('Ctrl Pts',(13.8063112075927,-2.89407576595085,1.41791983480526));
#66567=CARTESIAN_POINT('Ctrl Pts',(13.8067613567944,-2.89729043131036,1.41133955950519));
#66568=CARTESIAN_POINT('Ctrl Pts',(13.8078225657722,-2.90480276983812,1.39582830716606));
#66569=CARTESIAN_POINT('Ctrl Pts',(13.8084342734203,-2.90908170977681,1.38688838666615));
#66570=CARTESIAN_POINT('Ctrl Pts',(13.8104417426095,-2.92295572100962,1.35755492591218));
#66571=CARTESIAN_POINT('Ctrl Pts',(13.811843466801,-2.93237794250448,1.33708080704151));
#66572=CARTESIAN_POINT('Ctrl Pts',(13.8151486393364,-2.953971720138,1.2888320867976));
#66573=CARTESIAN_POINT('Ctrl Pts',(13.8170579556481,-2.96596737648447,1.26098155892362));
#66574=CARTESIAN_POINT('Ctrl Pts',(13.823838915862,-3.00688527815918,1.1621663707528));
#66575=CARTESIAN_POINT('Ctrl Pts',(13.8287799402461,-3.03366598657939,1.09034806074541));
#66576=CARTESIAN_POINT('Ctrl Pts',(13.8564405433384,-3.16716600015925,0.689203114943928));
#66577=CARTESIAN_POINT('Ctrl Pts',(13.8806910018625,-3.22282100853309,0.345376931363903));
#66578=CARTESIAN_POINT('Ctrl Pts',(13.9029341371857,-3.2227499320172,-0.000661954035870993));
#66579=CARTESIAN_POINT('Ctrl Pts',(13.9029343323106,-3.22274993139226,-0.000664989615965877));
#66580=CARTESIAN_POINT('Ctrl Pts',(13.904215504374,-3.22274581871248,-0.0205963361621372));
#66581=CARTESIAN_POINT('Ctrl Pts',(13.9054885607806,-3.22255680548054,-0.0405278534713367));
#66582=CARTESIAN_POINT('Ctrl Pts',(13.9076135515616,-3.22192814459894,-0.074033680711978));
#66583=CARTESIAN_POINT('Ctrl Pts',(13.9084703521966,-3.22158759675995,-0.0876089400347084));
#66584=CARTESIAN_POINT('Ctrl Pts',(13.9096535050165,-3.22099568948733,-0.106452512377118));
#66585=CARTESIAN_POINT('Ctrl Pts',(13.9099837438076,-3.22081719442239,-0.11172273773818));
#66586=CARTESIAN_POINT('Ctrl Pts',(13.9105629791671,-3.2204807015838,-0.120985870745676));
#66587=CARTESIAN_POINT('Ctrl Pts',(13.9108122780473,-3.22032821198566,-0.124978949004372));
#66588=CARTESIAN_POINT('Ctrl Pts',(13.9113011899043,-3.22001406553136,-0.132822561126043));
#66589=CARTESIAN_POINT('Ctrl Pts',(13.9115408315839,-3.21985292762392,-0.136673113912842));
#66590=CARTESIAN_POINT('Ctrl Pts',(13.9120191671923,-3.21951694725458,-0.144371125512332));
#66591=CARTESIAN_POINT('Ctrl Pts',(13.9122578614134,-3.21934211555479,-0.148218551227557));
#66592=CARTESIAN_POINT('Ctrl Pts',(13.9129002099964,-3.21885227313186,-0.158588289752942));
#66593=CARTESIAN_POINT('Ctrl Pts',(13.9133031396712,-3.21852433359483,-0.165110016997159));
#66594=CARTESIAN_POINT('Ctrl Pts',(13.9147859447218,-3.21724111963642,-0.18917102367664));
#66595=CARTESIAN_POINT('Ctrl Pts',(13.9158590842077,-3.21616225834951,-0.206703793240447));
#66596=CARTESIAN_POINT('Ctrl Pts',(13.9185985462839,-3.21302142154262,-0.251736674087955));
#66597=CARTESIAN_POINT('Ctrl Pts',(13.9202542934914,-3.21074969519869,-0.279221259841623));
#66598=CARTESIAN_POINT('Ctrl Pts',(13.9374338652326,-3.18326959943628,-0.566691067286937));
#66599=CARTESIAN_POINT('Ctrl Pts',(13.9516129073683,-3.12689232925233,-0.822754421194623));
#66600=CARTESIAN_POINT('Ctrl Pts',(13.9714255379752,-3.01019132116688,-1.15457856374885));
#66601=CARTESIAN_POINT('Ctrl Pts',(13.9765692811185,-2.97659420506073,-1.23862381874234));
#66602=CARTESIAN_POINT('Ctrl Pts',(13.9875992713221,-2.89852797860838,-1.41231936371177));
#66603=CARTESIAN_POINT('Ctrl Pts',(13.9935011572372,-2.853331977305,-1.50153389217408));
#66604=CARTESIAN_POINT('Ctrl Pts',(14.0005497576198,-2.79594350547301,-1.60283782427328));
#66605=CARTESIAN_POINT('Ctrl Pts',(14.0015513664645,-2.78771037645488,-1.61711472012142));
#66606=CARTESIAN_POINT('Ctrl Pts',(14.0030896146388,-2.77494911995102,-1.63885666208952));
#66607=CARTESIAN_POINT('Ctrl Pts',(14.0036233991778,-2.77049947892214,-1.64636764184584));
#66608=CARTESIAN_POINT('Ctrl Pts',(14.0045982203501,-2.76233480772296,-1.66002274787548));
#66609=CARTESIAN_POINT('Ctrl Pts',(14.005038893793,-2.75862964764942,-1.66617273390393));
#66610=CARTESIAN_POINT('Ctrl Pts',(14.0059931505848,-2.75057571541557,-1.67944049332981));
#66611=CARTESIAN_POINT('Ctrl Pts',(14.0065069941959,-2.7462198076236,-1.68655385416343));
#66612=CARTESIAN_POINT('Ctrl Pts',(14.0079043020552,-2.73432343312714,-1.70581279722629));
#66613=CARTESIAN_POINT('Ctrl Pts',(14.0087897285464,-2.72672975359577,-1.71792513701592));
#66614=CARTESIAN_POINT('Ctrl Pts',(14.0130542472654,-2.68989430187898,-1.77582018755457));
#66615=CARTESIAN_POINT('Ctrl Pts',(14.0164731733668,-2.65958008668491,-1.82090688286336));
#66616=CARTESIAN_POINT('Ctrl Pts',(14.020649293548,-2.62164515003427,-1.87435863532592));
#66617=CARTESIAN_POINT('Ctrl Pts',(14.0213662998812,-2.61510022377665,-1.88347933387328));
#66618=CARTESIAN_POINT('Ctrl Pts',(14.0236300633617,-2.59433655904905,-1.91209772542658));
#66619=CARTESIAN_POINT('Ctrl Pts',(14.0251830186322,-2.57994664605889,-1.93146968611412));
#66620=CARTESIAN_POINT('Ctrl Pts',(14.030702084704,-2.52829218468731,-1.99940058543471));
#66621=CARTESIAN_POINT('Ctrl Pts',(14.0347087736727,-2.48986488953538,-2.04705549329416));
#66622=CARTESIAN_POINT('Ctrl Pts',(14.0549204115848,-2.29127835244114,-2.2794597095774));
#66623=CARTESIAN_POINT('Ctrl Pts',(14.0717370377799,-2.11183361977564,-2.44663774271791));
#66624=CARTESIAN_POINT('Ctrl Pts',(14.0924586966739,-1.86128058299915,-2.63177721136415));
#66625=CARTESIAN_POINT('Ctrl Pts',(14.0968678567232,-1.80609949481193,-2.66994803975714));
#66626=CARTESIAN_POINT('Ctrl Pts',(14.1026704461328,-1.7304386653517,-2.71886541668517));
#66627=CARTESIAN_POINT('Ctrl Pts',(14.1041419105404,-1.71097971748581,-2.73115279724182));
#66628=CARTESIAN_POINT('Ctrl Pts',(14.1062820343509,-1.6822509565403,-2.74886605000701));
#66629=CARTESIAN_POINT('Ctrl Pts',(14.1069601957909,-1.67308344247473,-2.75445541688525));
#66630=CARTESIAN_POINT('Ctrl Pts',(14.1080268012456,-1.65856059933289,-2.76321063206034));
#66631=CARTESIAN_POINT('Ctrl Pts',(14.108417116168,-1.65322383925897,-2.76640691106741));
#66632=CARTESIAN_POINT('Ctrl Pts',(14.1091520225251,-1.6431327096732,-2.77241103514451));
#66633=CARTESIAN_POINT('Ctrl Pts',(14.1094968206847,-1.63838032300039,-2.77522214744606));
#66634=CARTESIAN_POINT('Ctrl Pts',(14.1100915733927,-1.63015132766132,-2.78006122418263));
#66635=CARTESIAN_POINT('Ctrl Pts',(14.1103419002772,-1.62667811168026,-2.78209490904811));
#66636=CARTESIAN_POINT('Ctrl Pts',(14.1108285463644,-1.61990695112023,-2.78604263638415));
#66637=CARTESIAN_POINT('Ctrl Pts',(14.1110649094346,-1.61660942337796,-2.78795733013341));
#66638=CARTESIAN_POINT('Ctrl Pts',(14.1116283896445,-1.60872749470395,-2.79251524853918));
#66639=CARTESIAN_POINT('Ctrl Pts',(14.1119551553953,-1.60413994839402,-2.79515305349255));
#66640=CARTESIAN_POINT('Ctrl Pts',(14.1129427805934,-1.59022443850809,-2.80310882558141));
#66641=CARTESIAN_POINT('Ctrl Pts',(14.1136014155708,-1.58087626224603,-2.80839155102719));
#66642=CARTESIAN_POINT('Ctrl Pts',(14.1222084563203,-1.45784981981265,-2.87710578602502));
#66643=CARTESIAN_POINT('Ctrl Pts',(14.1297440702819,-1.34044074676066,-2.93364809932216));
#66644=CARTESIAN_POINT('Ctrl Pts',(14.1451446028459,-1.08917613345362,-3.0364066739481));
#66645=CARTESIAN_POINT('Ctrl Pts',(14.1529695774844,-0.955056731399472,
-3.08122360094422));
#66646=CARTESIAN_POINT('Ctrl Pts',(14.1725895787907,-0.616626357708059,
-3.17008206154289));
#66647=CARTESIAN_POINT('Ctrl Pts',(14.184478592267,-0.41018881889637,-3.20333818142817));
#66648=CARTESIAN_POINT('Ctrl Pts',(14.1983384781767,-0.180900128263713,
-3.21773829586386));
#66649=CARTESIAN_POINT('Ctrl Pts',(14.1996203355713,-0.159786380194437,
-3.21885583350487));
#66650=CARTESIAN_POINT('Ctrl Pts',(14.2014971775982,-0.129015546987957,
-3.22018102094396));
#66651=CARTESIAN_POINT('Ctrl Pts',(14.2020869975005,-0.119365813841638,
-3.2205531540873));
#66652=CARTESIAN_POINT('Ctrl Pts',(14.2031239783926,-0.102436861993183,
-3.22112981409548));
#66653=CARTESIAN_POINT('Ctrl Pts',(14.2035705488083,-0.0951583167500675,
-3.22135305164167));
#66654=CARTESIAN_POINT('Ctrl Pts',(14.2044391229376,-0.0810249372306493,
-3.22173858916093));
#66655=CARTESIAN_POINT('Ctrl Pts',(14.204861036382,-0.0741702134103058,
-3.22190368503225));
#66656=CARTESIAN_POINT('Ctrl Pts',(14.205986733496,-0.0559099602525115,
-3.22228517854179));
#66657=CARTESIAN_POINT('Ctrl Pts',(14.2066917276389,-0.0445037985140977,
-3.22246289382074));
#66658=CARTESIAN_POINT('Ctrl Pts',(14.2092307360877,-0.00353386313378993,
-3.22288366971615));
#66659=CARTESIAN_POINT('Ctrl Pts',(14.2110755657518,0.0260312731350481,
-3.22278046344612));
#66660=CARTESIAN_POINT('Ctrl Pts',(14.2342540185632,0.394860917139358,-3.21641748073574));
#66661=CARTESIAN_POINT('Ctrl Pts',(14.2574473391875,0.731025103735886,-3.15701530245414));
#66662=CARTESIAN_POINT('Ctrl Pts',(14.288153653159,1.1632912229544,-3.00779467591996));
#66663=CARTESIAN_POINT('Ctrl Pts',(14.2959779260124,1.27277573590477,-2.96312728248251));
#66664=CARTESIAN_POINT('Ctrl Pts',(14.3043358080653,1.39146986954189,-2.90690600898772));
#66665=CARTESIAN_POINT('Ctrl Pts',(14.3051698618159,1.40333541110378,-2.90119642222333));
#66666=CARTESIAN_POINT('Ctrl Pts',(14.3064523366813,1.42161797961378,-2.89226061366347));
#66667=CARTESIAN_POINT('Ctrl Pts',(14.3069036903497,1.42805961936003,-2.88908547176378));
#66668=CARTESIAN_POINT('Ctrl Pts',(14.3076517531045,1.43874892792106,-2.88377213003578));
#66669=CARTESIAN_POINT('Ctrl Pts',(14.3079491881449,1.44300253520505,-2.88164603302372));
#66670=CARTESIAN_POINT('Ctrl Pts',(14.3085256554515,1.45125363579077,-2.87749900273544));
#66671=CARTESIAN_POINT('Ctrl Pts',(14.3088047527989,1.45525164964701,-2.87547913623503));
#66672=CARTESIAN_POINT('Ctrl Pts',(14.3093268774783,1.46273731810461,-2.87167763481586));
#66673=CARTESIAN_POINT('Ctrl Pts',(14.3095700226823,1.46622589705797,-2.86989799802544));
#66674=CARTESIAN_POINT('Ctrl Pts',(14.3101299809209,1.47426592871497,-2.86577803153793));
#66675=CARTESIAN_POINT('Ctrl Pts',(14.3104465069657,1.47881504761461,-2.86343322087745));
#66676=CARTESIAN_POINT('Ctrl Pts',(14.3114057242902,1.49261334336807,-2.85627933560318));
#66677=CARTESIAN_POINT('Ctrl Pts',(14.3120462946643,1.50184490055567,-2.85143615349296));
#66678=CARTESIAN_POINT('Ctrl Pts',(14.3167679378365,1.56999953848465,-2.81525715370515));
#66679=CARTESIAN_POINT('Ctrl Pts',(14.3207418257078,1.6279648599433,-2.78214005176248));
#66680=CARTESIAN_POINT('Ctrl Pts',(14.3426896464391,1.94811558478924,-2.5857939849455));
#66681=CARTESIAN_POINT('Ctrl Pts',(14.3592009975871,2.18681205147607,-2.38733680873805));
#66682=CARTESIAN_POINT('Ctrl Pts',(14.3813340928892,2.4440914760308,-2.1019545067161));
#66683=CARTESIAN_POINT('Ctrl Pts',(14.3857341947261,2.49256676315334,-2.04423717344593));
#66684=CARTESIAN_POINT('Ctrl Pts',(14.3929121501563,2.56693565923299,-1.94910755786534));
#66685=CARTESIAN_POINT('Ctrl Pts',(14.3956387366972,2.59413871364243,-1.91275272082248));
#66686=CARTESIAN_POINT('Ctrl Pts',(14.3991836820937,2.62811964878319,-1.86528099464661));
#66687=CARTESIAN_POINT('Ctrl Pts',(14.3999743481373,2.63561163539639,-1.85467985834762));
#66688=CARTESIAN_POINT('Ctrl Pts',(14.4012540894808,2.64759648489574,-1.83750206752296));
#66689=CARTESIAN_POINT('Ctrl Pts',(14.4017416274903,2.65212942369649,-1.83095344374043));
#66690=CARTESIAN_POINT('Ctrl Pts',(14.4026736419855,2.66073201189848,-1.8184265244883));
#66691=CARTESIAN_POINT('Ctrl Pts',(14.4031179530116,2.66480590900591,-1.81245119384582));
#66692=CARTESIAN_POINT('Ctrl Pts',(14.4041356475997,2.67407497961227,-1.79875710834075));
#66693=CARTESIAN_POINT('Ctrl Pts',(14.4047095283861,2.67925689008154,-1.79102949317902));
#66694=CARTESIAN_POINT('Ctrl Pts',(14.4064775419898,2.6950828502744,-1.76720636981167));
#66695=CARTESIAN_POINT('Ctrl Pts',(14.4076758350766,2.70561571061902,-1.75103784188162));
#66696=CARTESIAN_POINT('Ctrl Pts',(14.4246654213182,2.85221418552439,-1.52152011888532));
#66697=CARTESIAN_POINT('Ctrl Pts',(14.4414383828598,2.96280666625669,-1.29300977619716));
#66698=CARTESIAN_POINT('Ctrl Pts',(14.4728185426104,3.11459202453157,-0.85441663366588));
#66699=CARTESIAN_POINT('Ctrl Pts',(14.4872192208717,3.16387849642374,-0.64853607561234));
#66700=CARTESIAN_POINT('Ctrl Pts',(14.5024328071761,3.19627895368416,-0.413061615847468));
#66701=CARTESIAN_POINT('Ctrl Pts',(14.5041130587061,3.19956581077213,-0.386778721202662));
#66702=CARTESIAN_POINT('Ctrl Pts',(14.5062384445783,3.20335232666292,-0.353136942635103));
#66703=CARTESIAN_POINT('Ctrl Pts',(14.5066995750162,3.20415116975536,-0.345813696777634));
#66704=CARTESIAN_POINT('Ctrl Pts',(14.5074378624624,3.20539372001431,-0.334048777774984));
#66705=CARTESIAN_POINT('Ctrl Pts',(14.5077159043965,3.20585331609835,-0.329608862866269));
#66706=CARTESIAN_POINT('Ctrl Pts',(14.5082456549275,3.20671303508197,-0.32113164383283));
#66707=CARTESIAN_POINT('Ctrl Pts',(14.5084974477463,3.2071147539433,-0.317094587182505));
#66708=CARTESIAN_POINT('Ctrl Pts',(14.5090768531731,3.20802317653495,-0.307787093319658));
#66709=CARTESIAN_POINT('Ctrl Pts',(14.5094041603489,3.20852451584369,-0.302516161849091));
#66710=CARTESIAN_POINT('Ctrl Pts',(14.5104221666001,3.21004674249933,-0.286082372272008));
#66711=CARTESIAN_POINT('Ctrl Pts',(14.5111103628342,3.21102239493499,-0.274915260769156));
#66712=CARTESIAN_POINT('Ctrl Pts',(14.5176069921243,3.21972106140518,-0.168980381820534));
#66713=CARTESIAN_POINT('Ctrl Pts',(14.5231963998168,3.22330565110424,-0.0739093700151808));
#66714=CARTESIAN_POINT('Ctrl Pts',(14.5367032274469,3.22176233073709,0.160802273314587));
#66715=CARTESIAN_POINT('Ctrl Pts',(14.5444750960817,3.21177292296152,0.300214516479386));
#66716=CARTESIAN_POINT('Ctrl Pts',(14.5658855549688,3.15964155633866,0.679749956806448));
#66717=CARTESIAN_POINT('Ctrl Pts',(14.5795790608378,3.09929183890609,0.916385890315111));
#66718=CARTESIAN_POINT('Ctrl Pts',(14.5956346641905,3.00469667411899,1.1655246046522));
#66719=CARTESIAN_POINT('Ctrl Pts',(14.5970319733792,2.99627713411096,1.1870016851379));
#66720=CARTESIAN_POINT('Ctrl Pts',(14.599046467676,2.98387640023237,1.21766140436178));
#66721=CARTESIAN_POINT('Ctrl Pts',(14.5996573463794,2.98008174235401,1.22691909793273));
#66722=CARTESIAN_POINT('Ctrl Pts',(14.6007189073718,2.97342870361746,1.24293731957862));
#66723=CARTESIAN_POINT('Ctrl Pts',(14.601168911418,2.97059020758859,1.24970606666598));
#66724=CARTESIAN_POINT('Ctrl Pts',(14.6020352653524,2.96509069730047,1.26269572731159));
#66725=CARTESIAN_POINT('Ctrl Pts',(14.6024514946043,2.96243316366149,1.26891807959101));
#66726=CARTESIAN_POINT('Ctrl Pts',(14.6034335400205,2.95612703373186,1.28355547136469));
#66727=CARTESIAN_POINT('Ctrl Pts',(14.6039999136637,2.95246208376798,1.29196336200113));
#66728=CARTESIAN_POINT('Ctrl Pts',(14.6056788153165,2.9415157719382,1.31678585310519));
#66729=CARTESIAN_POINT('Ctrl Pts',(14.6067948126359,2.93413314490471,1.3331551621737));
#66730=CARTESIAN_POINT('Ctrl Pts',(14.6206375805125,2.84126188978362,1.53456758078043));
#66731=CARTESIAN_POINT('Ctrl Pts',(14.6339823251602,2.73855735501287,1.71112318763954));
#66732=CARTESIAN_POINT('Ctrl Pts',(14.6595098741317,2.5172433211441,2.02006774846566));
#66733=CARTESIAN_POINT('Ctrl Pts',(14.6715528773686,2.4030128061943,2.15469642417142));
#66734=CARTESIAN_POINT('Ctrl Pts',(14.6880677156243,2.22777418122208,2.32986114775148));
#66735=CARTESIAN_POINT('Ctrl Pts',(14.6927781300022,2.1755284700299,2.37871984003691));
#66736=CARTESIAN_POINT('Ctrl Pts',(14.6997325016839,2.09433871536258,2.44973140536204));
#66737=CARTESIAN_POINT('Ctrl Pts',(14.7020496758095,2.06657617604555,2.47319667478674));
#66738=CARTESIAN_POINT('Ctrl Pts',(14.70484923715,2.0320784729426,2.5013679658587));
#66739=CARTESIAN_POINT('Ctrl Pts',(14.7053623126116,2.02571592961146,2.50652340838883));
#66740=CARTESIAN_POINT('Ctrl Pts',(14.7061638075118,2.01571245248916,2.5145660582924));
#66741=CARTESIAN_POINT('Ctrl Pts',(14.706453394149,2.0120848621521,2.51746969411458));
#66742=CARTESIAN_POINT('Ctrl Pts',(14.7069925199739,2.00530632102573,2.52287143746179));
#66743=CARTESIAN_POINT('Ctrl Pts',(14.7072421950402,2.00215700757154,2.52537146740743));
#66744=CARTESIAN_POINT('Ctrl Pts',(14.707805957418,1.99502314413299,2.53101283297701));
#66745=CARTESIAN_POINT('Ctrl Pts',(14.708119791282,1.99103586090291,2.53415064819724));
#66746=CARTESIAN_POINT('Ctrl Pts',(14.709042759419,1.97926286280839,2.54337053735513));
#66747=CARTESIAN_POINT('Ctrl Pts',(14.7096500447466,1.97145648566775,2.54942630829948));
#66748=CARTESIAN_POINT('Ctrl Pts',(14.7137736555209,1.91805009855655,2.59046414027467));
#66749=CARTESIAN_POINT('Ctrl Pts',(14.7172107414847,1.87154598619488,2.6242593674698));
#66750=CARTESIAN_POINT('Ctrl Pts',(14.7207375929196,1.82208491536441,2.65821941469869));
#66751=CARTESIAN_POINT('Ctrl Pts',(14.7208854110345,1.82000863697762,2.65964141509207));
#66752=CARTESIAN_POINT('Ctrl Pts',(14.7217058337026,1.80846691779303,2.66752625712666));
#66753=CARTESIAN_POINT('Ctrl Pts',(14.7223762419931,1.7989686232505,2.67394106579032));
#66754=CARTESIAN_POINT('Ctrl Pts',(14.7230445264018,1.78943621037797,2.68030513402637));
#66755=CARTESIAN_POINT('Origin',(-1.72497344927317,0.,0.));
#66756=CARTESIAN_POINT('',(16.2168686787502,1.78943621037802,2.68030513402634));
#66757=CARTESIAN_POINT('',(15.9683010644095,1.78943598014216,2.68030528773733));
#66758=CARTESIAN_POINT('',(-1.72497344927317,1.78943621037804,2.68030513402633));
#66759=CARTESIAN_POINT('',(15.3965734493107,-3.22274990038605,-0.000801287517437093));
#66760=CARTESIAN_POINT('Ctrl Pts',(15.3965734493107,-3.22274990038605,-0.000801287517414983));
#66761=CARTESIAN_POINT('Ctrl Pts',(15.403151483107,-3.22272326425235,-0.107930870065952));
#66762=CARTESIAN_POINT('Ctrl Pts',(15.4097295169033,-3.21735064918231,-0.214916416866613));
#66763=CARTESIAN_POINT('Ctrl Pts',(15.4163075506996,-3.2067002897671,-0.321233270549037));
#66764=CARTESIAN_POINT('Ctrl Pts',(15.4229099905891,-3.19601041494748,-0.427944585423264));
#66765=CARTESIAN_POINT('Ctrl Pts',(15.4295124304787,-3.18000365239334,-0.533981909528027));
#66766=CARTESIAN_POINT('Ctrl Pts',(15.4361148703683,-3.15879978879431,-0.638828190371247));
#66767=CARTESIAN_POINT('Ctrl Pts',(15.4427299993246,-3.13755517401168,-0.743875972701292));
#66768=CARTESIAN_POINT('Ctrl Pts',(15.449345128281,-3.11109360027254,-0.847727819155364));
#66769=CARTESIAN_POINT('Ctrl Pts',(15.4559602572373,-3.07958468072366,-0.949881969905816));
#66770=CARTESIAN_POINT('Ctrl Pts',(15.4625955718556,-3.04797961363123,-1.05234783780807));
#66771=CARTESIAN_POINT('Ctrl Pts',(15.4692308864739,-3.01129650796592,-1.15310533350681));
#66772=CARTESIAN_POINT('Ctrl Pts',(15.4758662010922,-2.96975371305879,-1.25167106153076));
#66773=CARTESIAN_POINT('Ctrl Pts',(15.4795684054817,-2.94657471906928,-1.30666626400921));
#66774=CARTESIAN_POINT('Ctrl Pts',(15.4832706098711,-2.92188366837227,-1.36097957634467));
#66775=CARTESIAN_POINT('Ctrl Pts',(15.4869728142606,-2.8957245434024,-1.41453063990744));
#66776=CARTESIAN_POINT('Ctrl Pts',(15.4931450623534,-2.85211252412471,-1.50381000300276));
#66777=CARTESIAN_POINT('Ctrl Pts',(15.4993173104461,-2.8042909571443,-1.59122768554707));
#66778=CARTESIAN_POINT('Ctrl Pts',(15.5054895585389,-2.75244187987435,-1.67635952600084));
#66779=CARTESIAN_POINT('Ctrl Pts',(15.5116534471915,-2.70066302487203,-1.76137606737506));
#66780=CARTESIAN_POINT('Ctrl Pts',(15.5178173358442,-2.64486772534409,-1.84411255228448));
#66781=CARTESIAN_POINT('Ctrl Pts',(15.5239812244968,-2.58528501290985,-1.9241670833178));
#66782=CARTESIAN_POINT('Ctrl Pts',(15.5301385861553,-2.52576539311624,-2.00413684392777));
#66783=CARTESIAN_POINT('Ctrl Pts',(15.5362959478139,-2.46246659163317,-2.08142995020427));
#66784=CARTESIAN_POINT('Ctrl Pts',(15.5424533094724,-2.39566174482634,-2.15567213807565));
#66785=CARTESIAN_POINT('Ctrl Pts',(15.5486061736187,-2.32890569418134,-2.22986009733957));
#66786=CARTESIAN_POINT('Ctrl Pts',(15.554759037765,-2.25864897942454,-2.30100124686958));
#66787=CARTESIAN_POINT('Ctrl Pts',(15.5609119019113,-2.18520536389433,-2.36875390872658));
#66788=CARTESIAN_POINT('Ctrl Pts',(15.5670624350479,-2.11178957244427,-2.43648090251863));
#66789=CARTESIAN_POINT('Ctrl Pts',(15.5732129681844,-2.03518959814623,-2.50082166519245));
#66790=CARTESIAN_POINT('Ctrl Pts',(15.5793635013209,-1.95575582067506,-2.56147159507882));
#66791=CARTESIAN_POINT('Ctrl Pts',(15.5855133495362,-1.87633088892305,-2.62211477100907));
#66792=CARTESIAN_POINT('Ctrl Pts',(15.5916631977514,-1.79407312664577,-2.67906766769473));
#66793=CARTESIAN_POINT('Ctrl Pts',(15.5978130459666,-1.70936492653555,-2.73206682027181));
#66794=CARTESIAN_POINT('Ctrl Pts',(15.6039638543457,-1.62464350109758,-2.78507424750427));
#66795=CARTESIAN_POINT('Ctrl Pts',(15.6101146627248,-1.53747124619339,-2.8341264741131));
#66796=CARTESIAN_POINT('Ctrl Pts',(15.616265471104,-1.44825750699312,-2.87900464673784));
#66797=CARTESIAN_POINT('Ctrl Pts',(15.6224228574701,-1.3589483580865,-2.92393081436099));
#66798=CARTESIAN_POINT('Ctrl Pts',(15.6285802438363,-1.26759375392542,-2.96467381837952));
#66799=CARTESIAN_POINT('Ctrl Pts',(15.6347376302025,-1.17462539029952,-3.00106193787528));
#66800=CARTESIAN_POINT('Ctrl Pts',(15.6408984529395,-1.08160514203481,-3.03747036518719));
#66801=CARTESIAN_POINT('Ctrl Pts',(15.6470592756764,-0.986969752166327,
-3.06951892850637));
#66802=CARTESIAN_POINT('Ctrl Pts',(15.6532200984134,-0.891166540265468,
-3.09708568819322));
#66803=CARTESIAN_POINT('Ctrl Pts',(15.6593912213301,-0.795203156526662,
-3.12469853629901));
#66804=CARTESIAN_POINT('Ctrl Pts',(15.6655623442468,-0.698068473542096,
-3.14781451301599));
#66805=CARTESIAN_POINT('Ctrl Pts',(15.6717334671635,-0.600220611140134,
-3.16636270513385));
#66806=CARTESIAN_POINT('Ctrl Pts',(15.676428989109,-0.525769528016257,-3.18047576758883));
#66807=CARTESIAN_POINT('Ctrl Pts',(15.6811245110546,-0.450905774207009,
-3.19194537925502));
#66808=CARTESIAN_POINT('Ctrl Pts',(15.6858200330002,-0.375832126923022,
-3.20076049945517));
#66809=CARTESIAN_POINT('Ctrl Pts',(15.691992281093,-0.277148065463111,-3.21234794585055));
#66810=CARTESIAN_POINT('Ctrl Pts',(15.6981645291858,-0.177753920732704,
-3.21938765345787));
#66811=CARTESIAN_POINT('Ctrl Pts',(15.7043367772785,-0.0781049306931113,
-3.22180340528429));
#66812=CARTESIAN_POINT('Ctrl Pts',(15.7105006659312,0.0214090988338605,
-3.22421588531533));
#66813=CARTESIAN_POINT('Ctrl Pts',(15.7166645545838,0.121176857218107,-3.2220168465318));
#66814=CARTESIAN_POINT('Ctrl Pts',(15.7228284432364,0.220736425033003,-3.21518164232811));
#66815=CARTESIAN_POINT('Ctrl Pts',(15.728985804895,0.320190568375327,-3.20835367598024));
#66816=CARTESIAN_POINT('Ctrl Pts',(15.7351431665535,0.419436528467584,-3.19689933390213));
#66817=CARTESIAN_POINT('Ctrl Pts',(15.7413005282121,0.518011783406816,-3.18084601242369));
#66818=CARTESIAN_POINT('Ctrl Pts',(15.7474533923584,0.616515036173647,-3.16480441674826));
#66819=CARTESIAN_POINT('Ctrl Pts',(15.7536062565047,0.7143481303619,-3.14417058999656));
#66820=CARTESIAN_POINT('Ctrl Pts',(15.759759120651,0.811053988393693,-3.11902372392559));
#66821=CARTESIAN_POINT('Ctrl Pts',(15.7659096537875,0.907723209455384,-3.09388638473334));
#66822=CARTESIAN_POINT('Ctrl Pts',(15.7720601869241,1.0032656229845,-3.0642395127072));
#66823=CARTESIAN_POINT('Ctrl Pts',(15.7782107200606,1.09723554146382,-3.03021314911156));
#66824=CARTESIAN_POINT('Ctrl Pts',(15.7843605682758,1.1911949954842,-2.99619057468048));
#66825=CARTESIAN_POINT('Ctrl Pts',(15.790510416491,1.28358189417931,-2.95778962618623));
#66826=CARTESIAN_POINT('Ctrl Pts',(15.7966602647062,1.37396784491287,-2.91518951762068));
#66827=CARTESIAN_POINT('Ctrl Pts',(15.8028110730854,1.46436790743041,-2.87258275798243));
#66828=CARTESIAN_POINT('Ctrl Pts',(15.8089618814645,1.55276600851309,-2.82577572127488));
#66829=CARTESIAN_POINT('Ctrl Pts',(15.8151126898436,1.63875670963832,-2.77499441605121));
#66830=CARTESIAN_POINT('Ctrl Pts',(15.8212700762098,1.72483937358922,-2.72415880271912));
#66831=CARTESIAN_POINT('Ctrl Pts',(15.827427462576,1.80850912162653,-2.66934065480024));
#66832=CARTESIAN_POINT('Ctrl Pts',(15.8335848489422,1.8893880782495,-2.61081026738227));
#66833=CARTESIAN_POINT('Ctrl Pts',(15.8397456716792,1.97031217254386,-2.55224721478779));
#66834=CARTESIAN_POINT('Ctrl Pts',(15.8459064944161,2.04844203398604,-2.48996806757623));
#66835=CARTESIAN_POINT('Ctrl Pts',(15.8520673171531,2.12343321559177,-2.42428318094681));
#66836=CARTESIAN_POINT('Ctrl Pts',(15.8582384400698,2.19854977373921,-2.3584884768195));
#66837=CARTESIAN_POINT('Ctrl Pts',(15.8644095629864,2.27051685708402,-2.28927696092124));
#66838=CARTESIAN_POINT('Ctrl Pts',(15.8705806859031,2.33902710271958,-2.21699566423646));
#66839=CARTESIAN_POINT('Ctrl Pts',(15.8752762078487,2.39115559962716,-2.16199782682172));
#66840=CARTESIAN_POINT('Ctrl Pts',(15.8799717297943,2.44128353743214,-2.10522350623952));
#66841=CARTESIAN_POINT('Ctrl Pts',(15.8846672517399,2.48929198490435,-2.04683731067981));
#66842=CARTESIAN_POINT('Ctrl Pts',(15.8908394998326,2.55239893058178,-1.97008884940888));
#66843=CARTESIAN_POINT('Ctrl Pts',(15.8970117479254,2.61206422714657,-1.8902840508331));
#66844=CARTESIAN_POINT('Ctrl Pts',(15.9031839960182,2.667977608358,-1.80776465387515));
#66845=CARTESIAN_POINT('Ctrl Pts',(15.9093478846708,2.72381526277492,-1.72535701781023));
#66846=CARTESIAN_POINT('Ctrl Pts',(15.9155117733234,2.77591086024843,-1.64024244732748));
#66847=CARTESIAN_POINT('Ctrl Pts',(15.9216756619761,2.82399390327054,-1.55279618649417));
#66848=CARTESIAN_POINT('Ctrl Pts',(15.9278330236346,2.8720260307497,-1.46544252324972));
#66849=CARTESIAN_POINT('Ctrl Pts',(15.9339903852932,2.91605384290952,-1.37576245688326));
#66850=CARTESIAN_POINT('Ctrl Pts',(15.9401477469517,2.95585029545812,-1.28415987841863));
#66851=CARTESIAN_POINT('Ctrl Pts',(15.946300611098,2.99561767954489,-1.19262420908497));
#66852=CARTESIAN_POINT('Ctrl Pts',(15.9524534752443,3.03115967630921,-1.09916921675777));
#66853=CARTESIAN_POINT('Ctrl Pts',(15.9586063393906,3.06229575603652,-1.00422221896386));
#66854=CARTESIAN_POINT('Ctrl Pts',(15.9647568725272,3.09342003987426,-0.90931119179668));
#66855=CARTESIAN_POINT('Ctrl Pts',(15.9709074056637,3.12014158812306,-0.812909694593116));
#66856=CARTESIAN_POINT('Ctrl Pts',(15.9770579388002,3.1423288048497,-0.715462958308727));
#66857=CARTESIAN_POINT('Ctrl Pts',(15.9832077870154,3.16451355081524,-0.61802707366056));
#66858=CARTESIAN_POINT('Ctrl Pts',(15.9893576352306,3.18216487272335,-0.519546604882973));
#66859=CARTESIAN_POINT('Ctrl Pts',(15.9955074834458,3.19520189069667,-0.42047882252074));
#66860=CARTESIAN_POINT('Ctrl Pts',(16.001658291825,3.20824094411444,-0.321395572896909));
#66861=CARTESIAN_POINT('Ctrl Pts',(16.0078091002041,3.21666420597336,-0.221725258258982));
#66862=CARTESIAN_POINT('Ctrl Pts',(16.0139599085833,3.2204425719225,-0.121931142245125));
#66863=CARTESIAN_POINT('Ctrl Pts',(16.0201172949494,3.22422497864819,-0.0220303013322788));
#66864=CARTESIAN_POINT('Ctrl Pts',(16.0262746813156,3.22335255343781,0.0779941704340612));
#66865=CARTESIAN_POINT('Ctrl Pts',(16.0324320676818,3.21784834977617,0.177678249492705));
#66866=CARTESIAN_POINT('Ctrl Pts',(16.0385928904188,3.21234107427797,0.277417961158298));
#66867=CARTESIAN_POINT('Ctrl Pts',(16.0447537131557,3.2021969165482,0.376816469649774));
#66868=CARTESIAN_POINT('Ctrl Pts',(16.0509145358927,3.18749070413578,0.475416210859515));
#66869=CARTESIAN_POINT('Ctrl Pts',(16.0570856588094,3.17275990464505,0.574180799379308));
#66870=CARTESIAN_POINT('Ctrl Pts',(16.0632567817261,3.15345189936077,0.67214352673028));
#66871=CARTESIAN_POINT('Ctrl Pts',(16.0694279046428,3.12969241956978,0.768858193288883));
#66872=CARTESIAN_POINT('Ctrl Pts',(16.0741234265884,3.11161416051055,0.842447043392282));
#66873=CARTESIAN_POINT('Ctrl Pts',(16.0788189485339,3.09095978518413,0.915313567983737));
#66874=CARTESIAN_POINT('Ctrl Pts',(16.0835144704795,3.06780345613332,0.987268715718499));
#66875=CARTESIAN_POINT('Ctrl Pts',(16.089685502756,3.03737053395065,1.08183488839853));
#66876=CARTESIAN_POINT('Ctrl Pts',(16.0958565350325,3.00250740618948,1.17515899787367));
#66877=CARTESIAN_POINT('Ctrl Pts',(16.1020275673089,2.96333370680217,1.26679552597493));
#66878=CARTESIAN_POINT('Ctrl Pts',(16.1081908020022,2.92420950645555,1.35831626413793));
#66879=CARTESIAN_POINT('Ctrl Pts',(16.1143540366956,2.8807857250492,1.4481532619653));
#66880=CARTESIAN_POINT('Ctrl Pts',(16.1205172713889,2.83323169421114,1.53587620901473));
#66881=CARTESIAN_POINT('Ctrl Pts',(16.1266743676933,2.78572502570034,1.62351178675282));
#66882=CARTESIAN_POINT('Ctrl Pts',(16.1328314639976,2.73409648872252,1.70903711853518));
#66883=CARTESIAN_POINT('Ctrl Pts',(16.138988560302,2.67856303153204,1.7920428701931));
#66884=CARTESIAN_POINT('Ctrl Pts',(16.145141171698,2.62307002562788,1.87498815939114));
#66885=CARTESIAN_POINT('Ctrl Pts',(16.151293783094,2.56367799531519,1.95541715741891));
#66886=CARTESIAN_POINT('Ctrl Pts',(16.15744639449,2.50064874131153,2.03294698284954));
#66887=CARTESIAN_POINT('Ctrl Pts',(16.1635967978572,2.43764210703775,2.11044898463326));
#66888=CARTESIAN_POINT('Ctrl Pts',(16.1697472012245,2.37100111535886,2.18505354373481));
#66889=CARTESIAN_POINT('Ctrl Pts',(16.1758976045917,2.30102910816362,2.25640922837231));
#66890=CARTESIAN_POINT('Ctrl Pts',(16.182046812984,2.23107069597825,2.32775104916232));
#66891=CARTESIAN_POINT('Ctrl Pts',(16.1881960213763,2.15778286269837,2.39584494405235));
#66892=CARTESIAN_POINT('Ctrl Pts',(16.1943452297685,2.08150641312365,2.46037570598986));
#66893=CARTESIAN_POINT('Ctrl Pts',(16.200496116594,2.00520914380899,2.5249240816691));
#66894=CARTESIAN_POINT('Ctrl Pts',(16.2066470034194,1.9259219639394,2.58590710539825));
#66895=CARTESIAN_POINT('Ctrl Pts',(16.2127978902448,1.84401883694316,2.64304977090837));
#66896=CARTESIAN_POINT('Ctrl Pts',(16.2141548197466,1.82595042299473,2.65565585046137));
#66897=CARTESIAN_POINT('Ctrl Pts',(16.2155117492484,1.80775481277862,2.66807519421725));
#66898=CARTESIAN_POINT('Ctrl Pts',(16.2168686787502,1.78943621037802,2.68030513402634));
#66899=CARTESIAN_POINT('Ctrl Pts',(14.9670297268737,1.78943621037805,2.68030513402632));
#66900=CARTESIAN_POINT('Ctrl Pts',(14.9731800598208,1.70635700013351,2.73577081412889));
#66901=CARTESIAN_POINT('Ctrl Pts',(14.9793303927678,1.62066352453859,2.7873922156097));
#66902=CARTESIAN_POINT('Ctrl Pts',(14.9854807257148,1.53275005607261,2.83492413092651));
#66903=CARTESIAN_POINT('Ctrl Pts',(14.9916306108541,1.44484298861588,2.88245258542855));
#66904=CARTESIAN_POINT('Ctrl Pts',(14.9977804959933,1.35471663189435,2.92589193935345));
#66905=CARTESIAN_POINT('Ctrl Pts',(15.0039303811325,1.26279030761724,2.9650426980885));
#66906=CARTESIAN_POINT('Ctrl Pts',(15.0100814635135,1.17084608739051,3.00420107857948));
#66907=CARTESIAN_POINT('Ctrl Pts',(15.0162325458945,1.07710160317344,3.03906903518434));
#66908=CARTESIAN_POINT('Ctrl Pts',(15.0223836282755,0.981995675153088,3.0694954074702));
#66909=CARTESIAN_POINT('Ctrl Pts',(15.0285414183548,0.886786034999967,3.09995495943294));
#66910=CARTESIAN_POINT('Ctrl Pts',(15.034699208434,0.790212401369721,3.12596312440363));
#66911=CARTESIAN_POINT('Ctrl Pts',(15.0408569985133,0.692728123241261,3.14741883291224));
#66912=CARTESIAN_POINT('Ctrl Pts',(15.0470184380535,0.595186070318326,3.16888725730871));
#66913=CARTESIAN_POINT('Ctrl Pts',(15.0531798775936,0.496732726148102,3.18579777944097));
#66914=CARTESIAN_POINT('Ctrl Pts',(15.0593413171338,0.397828923788017,3.19810095367511));
#66915=CARTESIAN_POINT('Ctrl Pts',(15.0655127909436,0.298764050719617,3.21042416435822));
#66916=CARTESIAN_POINT('Ctrl Pts',(15.0716842647535,0.199247687356821,3.21812501017596));
#66917=CARTESIAN_POINT('Ctrl Pts',(15.0778557385634,0.0997430830037804,
3.22120612191969));
#66918=CARTESIAN_POINT('Ctrl Pts',(15.081663284636,0.0383528256379945,3.22310704142136));
#66919=CARTESIAN_POINT('Ctrl Pts',(15.0854708307087,-0.0230329793170104,
3.22325054454222));
#66920=CARTESIAN_POINT('Ctrl Pts',(15.0892783767813,-0.0843066070415162,
3.22164708782777));
#66921=CARTESIAN_POINT('Ctrl Pts',(15.0954506248741,-0.183634632138016,
3.21904779356874));
#66922=CARTESIAN_POINT('Ctrl Pts',(15.1016228729669,-0.283017162718341,
3.21184598092432));
#66923=CARTESIAN_POINT('Ctrl Pts',(15.1077951210596,-0.381992745054684,
3.20003111004027));
#66924=CARTESIAN_POINT('Ctrl Pts',(15.1139590097123,-0.480834278914442,
3.18823224073365));
#66925=CARTESIAN_POINT('Ctrl Pts',(15.120122898365,-0.579269532494049,3.17183278228601));
#66926=CARTESIAN_POINT('Ctrl Pts',(15.1262867870176,-0.67683779071223,3.15087419100855));
#66927=CARTESIAN_POINT('Ctrl Pts',(15.1324441486762,-0.774302733072408,
3.12993779296156));
#66928=CARTESIAN_POINT('Ctrl Pts',(15.1386015103347,-0.870902082932757,
3.10445195074111));
#66929=CARTESIAN_POINT('Ctrl Pts',(15.1447588719933,-0.966181948124195,
3.0745097179256));
#66930=CARTESIAN_POINT('Ctrl Pts',(15.1509117361396,-1.0613922181895,3.04458935576939));
#66931=CARTESIAN_POINT('Ctrl Pts',(15.1570646002859,-1.15528450661803,3.01021920449644));
#66932=CARTESIAN_POINT('Ctrl Pts',(15.1632174644322,-1.24741769390861,2.97154280794064));
#66933=CARTESIAN_POINT('Ctrl Pts',(15.1693679975688,-1.33951597658323,2.93288106392001));
#66934=CARTESIAN_POINT('Ctrl Pts',(15.1755185307053,-1.42985608225006,2.88991648418273));
#66935=CARTESIAN_POINT('Ctrl Pts',(15.1816690638418,-1.51801541423247,2.8428413189365));
#66936=CARTESIAN_POINT('Ctrl Pts',(15.1878189120571,-1.60616492882119,2.79577139596491));
#66937=CARTESIAN_POINT('Ctrl Pts',(15.1939687602723,-1.69213376937722,2.74459200216956));
#66938=CARTESIAN_POINT('Ctrl Pts',(15.2001186084875,-1.77552346751651,2.6895415926879));
#66939=CARTESIAN_POINT('Ctrl Pts',(15.2062694168666,-1.85892618512797,2.63448258829235));
#66940=CARTESIAN_POINT('Ctrl Pts',(15.2124202252458,-1.93974859796171,2.57555160710201));
#66941=CARTESIAN_POINT('Ctrl Pts',(15.2185710336249,-2.01762162832546,2.51303014852853));
#66942=CARTESIAN_POINT('Ctrl Pts',(15.2247284199911,-2.09557794006541,2.45044182632989));
#66943=CARTESIAN_POINT('Ctrl Pts',(15.2308858063573,-2.17057823130809,2.38425563145967));
#66944=CARTESIAN_POINT('Ctrl Pts',(15.2370431927234,-2.2422870193426,2.31479296814806));
#66945=CARTESIAN_POINT('Ctrl Pts',(15.2432040154604,-2.31403582727659,2.24529153847488));
#66946=CARTESIAN_POINT('Ctrl Pts',(15.2493648381974,-2.3824891761296,2.17251031522878));
#66947=CARTESIAN_POINT('Ctrl Pts',(15.2555256609343,-2.44735038123923,2.09680558801912));
#66948=CARTESIAN_POINT('Ctrl Pts',(15.261696783851,-2.51232002674694,2.02097429130244));
#66949=CARTESIAN_POINT('Ctrl Pts',(15.2678679067677,-2.57368526532954,1.94221007028928));
#66950=CARTESIAN_POINT('Ctrl Pts',(15.2740390296844,-2.63119134612786,1.86090022907244));
#66951=CARTESIAN_POINT('Ctrl Pts',(15.2787345516299,-2.6749469264387,1.7990326971865));
#66952=CARTESIAN_POINT('Ctrl Pts',(15.2834300735755,-2.71646912576312,1.73569202629276));
#66953=CARTESIAN_POINT('Ctrl Pts',(15.288125595521,-2.75566369413806,1.67105809812507));
#66954=CARTESIAN_POINT('Ctrl Pts',(15.2944981381896,-2.80885672831925,1.58333995520794));
#66955=CARTESIAN_POINT('Ctrl Pts',(15.3008706808582,-2.85793822589388,1.492946968511));
#66956=CARTESIAN_POINT('Ctrl Pts',(15.3072432235268,-2.90263902050083,1.40028721309809));
#66957=CARTESIAN_POINT('Ctrl Pts',(15.3136052317173,-2.94726592002897,1.30778063393155));
#66958=CARTESIAN_POINT('Ctrl Pts',(15.3199672399077,-2.98752635647166,1.21301509644927));
#66959=CARTESIAN_POINT('Ctrl Pts',(15.3263292480982,-3.02319551557037,1.1164257418813));
#66960=CARTESIAN_POINT('Ctrl Pts',(15.3326790949963,-3.05879649131245,1.02002102262786));
#66961=CARTESIAN_POINT('Ctrl Pts',(15.3390289418944,-3.08982353762513,0.921799800806557));
#66962=CARTESIAN_POINT('Ctrl Pts',(15.3453787887925,-3.11609915948835,0.822218700064662));
#66963=CARTESIAN_POINT('Ctrl Pts',(15.3517214721691,-3.14234513875027,0.722749940826297));
#66964=CARTESIAN_POINT('Ctrl Pts',(15.3580641555458,-3.16385025754267,0.621924735618091));
#66965=CARTESIAN_POINT('Ctrl Pts',(15.3644068389225,-3.18048614095612,0.52021675260036));
#66966=CARTESIAN_POINT('Ctrl Pts',(15.370741969782,-3.19710221527828,0.418629877832159));
#66967=CARTESIAN_POINT('Ctrl Pts',(15.3770771006416,-3.20886053925029,0.316162708355363));
#66968=CARTESIAN_POINT('Ctrl Pts',(15.3834122315011,-3.21568353572234,0.213300165457598));
#66969=CARTESIAN_POINT('Ctrl Pts',(15.3877993040918,-3.22040845482382,0.142067944284031));
#66970=CARTESIAN_POINT('Ctrl Pts',(15.3921863766824,-3.22276766474656,0.0706463933296931));
#66971=CARTESIAN_POINT('Ctrl Pts',(15.3965734492731,-3.22274990038621,-0.000801286904994983));
#66972=CARTESIAN_POINT('Ctrl Pts',(14.7230445264018,1.78943621037797,2.68030513402637));
#66973=CARTESIAN_POINT('Ctrl Pts',(14.7231109020367,1.78848942791742,2.68093722878183));
#66974=CARTESIAN_POINT('Ctrl Pts',(14.7231772567185,1.78754230888135,2.68156882298579));
#66975=CARTESIAN_POINT('Ctrl Pts',(14.740998021613,1.53300616988584,2.8511135885443));
#66976=CARTESIAN_POINT('Ctrl Pts',(14.7573121250989,1.25673265540303,2.9832222007102));
#66977=CARTESIAN_POINT('Ctrl Pts',(14.7791757212824,0.894772783146178,3.09694562165537));
#66978=CARTESIAN_POINT('Ctrl Pts',(14.7835362633534,0.822801268485764,3.1168393313995));
#66979=CARTESIAN_POINT('Ctrl Pts',(14.7906551569377,0.706355328689767,3.14471189485576));
#66980=CARTESIAN_POINT('Ctrl Pts',(14.7933633196308,0.66228946747602,3.15428646533951));
#66981=CARTESIAN_POINT('Ctrl Pts',(14.7968875296238,0.605329505237608,3.16541647293248));
#66982=CARTESIAN_POINT('Ctrl Pts',(14.7976762864409,0.592605465375178,3.16782322924968));
#66983=CARTESIAN_POINT('Ctrl Pts',(14.7989536830623,0.572039874526359,3.17158497674564));
#66984=CARTESIAN_POINT('Ctrl Pts',(14.7994407959081,0.564207120008644,3.17298774134116));
#66985=CARTESIAN_POINT('Ctrl Pts',(14.8003724948821,0.549244199334205,3.17561028759485));
#66986=CARTESIAN_POINT('Ctrl Pts',(14.8008169175567,0.542114955278675,3.17683510165145));
#66987=CARTESIAN_POINT('Ctrl Pts',(14.8018355708504,0.525793088696647,3.17958267912424));
#66988=CARTESIAN_POINT('Ctrl Pts',(14.8024103020343,0.516597896706989,3.18108959253035));
#66989=CARTESIAN_POINT('Ctrl Pts',(14.8041834979483,0.488271595204182,3.18560566704075));
#66990=CARTESIAN_POINT('Ctrl Pts',(14.8053861584324,0.469120065326275,3.18848223368005));
#66991=CARTESIAN_POINT('Ctrl Pts',(14.8159960790056,0.300718782544522,3.21222612231473));
#66992=CARTESIAN_POINT('Ctrl Pts',(14.8257310844947,0.150223831730027,3.22277047595897));
#66993=CARTESIAN_POINT('Ctrl Pts',(14.8512025107649,-0.234086092629859,
3.22271816971552));
#66994=CARTESIAN_POINT('Ctrl Pts',(14.867254889849,-0.467015383726354,3.19727902450478));
#66995=CARTESIAN_POINT('Ctrl Pts',(14.8874126177165,-0.762645635207184,
3.13197524460535));
#66996=CARTESIAN_POINT('Ctrl Pts',(14.8919617223615,-0.829661344020823,
3.11489336394149));
#66997=CARTESIAN_POINT('Ctrl Pts',(14.8987058986138,-0.930197392890896,
3.08579194146998));
#66998=CARTESIAN_POINT('Ctrl Pts',(14.9009693826722,-0.964151033816046,
3.07535235914933));
#66999=CARTESIAN_POINT('Ctrl Pts',(14.9037129064292,-1.00565666227512,3.06183577739324));
#67000=CARTESIAN_POINT('Ctrl Pts',(14.9042222226442,-1.01337707916199,3.05928922282954));
#67001=CARTESIAN_POINT('Ctrl Pts',(14.9050191520123,-1.02548255968639,3.05524541578073));
#67002=CARTESIAN_POINT('Ctrl Pts',(14.9053079108635,-1.02987410570936,3.05376789522469));
#67003=CARTESIAN_POINT('Ctrl Pts',(14.9058463012314,-1.03807228041073,3.05098995151447));
#67004=CARTESIAN_POINT('Ctrl Pts',(14.9060960650402,-1.04187962023797,3.04969188620403));
#67005=CARTESIAN_POINT('Ctrl Pts',(14.9066610642988,-1.05050158088802,3.04673430492583));
#67006=CARTESIAN_POINT('Ctrl Pts',(14.9069760416528,-1.05531469179807,3.04507050794947));
#67007=CARTESIAN_POINT('Ctrl Pts',(14.9079054737319,-1.06953562417976,3.04011684648877));
#67008=CARTESIAN_POINT('Ctrl Pts',(14.9085180405688,-1.07893225633188,3.0367947056147));
#67009=CARTESIAN_POINT('Ctrl Pts',(14.9127492429446,-1.14398953195297,3.01345388902557));
#67010=CARTESIAN_POINT('Ctrl Pts',(14.9162838824298,-1.19910931367296,2.99194824296677));
#67011=CARTESIAN_POINT('Ctrl Pts',(14.9207680918513,-1.26946239458452,2.96224220838299));
#67012=CARTESIAN_POINT('Ctrl Pts',(14.9217732865504,-1.28526140170285,2.95542159792267));
#67013=CARTESIAN_POINT('Ctrl Pts',(14.9309017188953,-1.42889426110301,2.8920440450787));
#67014=CARTESIAN_POINT('Ctrl Pts',(14.9387201600622,-1.55298555893522,2.82734838787098));
#67015=CARTESIAN_POINT('Ctrl Pts',(14.9554249674204,-1.80847568802037,2.67223525482221));
#67016=CARTESIAN_POINT('Ctrl Pts',(14.9642923982549,-1.93815656787172,2.57972304022086));
#67017=CARTESIAN_POINT('Ctrl Pts',(14.9778115373712,-2.11864765716188,2.42964490453971));
#67018=CARTESIAN_POINT('Ctrl Pts',(14.9822289224596,-2.17509998416226,2.37923960578189));
#67019=CARTESIAN_POINT('Ctrl Pts',(14.989432666156,-2.26260332415189,2.29539048986673));
#67020=CARTESIAN_POINT('Ctrl Pts',(14.9921672826353,-2.29481018978089,2.26319181233338));
#67021=CARTESIAN_POINT('Ctrl Pts',(14.9957212625431,-2.33531615542333,2.22094234234419));
#67022=CARTESIAN_POINT('Ctrl Pts',(14.9965127568558,-2.34425253016377,2.2115077437988));
#67023=CARTESIAN_POINT('Ctrl Pts',(14.9977935154294,-2.35857548584112,2.19620188536729));
#67024=CARTESIAN_POINT('Ctrl Pts',(14.998281237909,-2.36399784137874,2.19036418155847));
#67025=CARTESIAN_POINT('Ctrl Pts',(14.9992133899913,-2.37430007600982,2.17918998768938));
#67026=CARTESIAN_POINT('Ctrl Pts',(14.9996576532661,-2.37918375708191,2.17385705649335));
#67027=CARTESIAN_POINT('Ctrl Pts',(15.0006749352364,-2.39030605223147,2.16162924635957));
#67028=CARTESIAN_POINT('Ctrl Pts',(15.001248449718,-2.39653283605589,2.15472373747882));
#67029=CARTESIAN_POINT('Ctrl Pts',(15.0030142337181,-2.41556982077244,2.13342710418028));
#67030=CARTESIAN_POINT('Ctrl Pts',(15.004210648287,-2.42828074395567,2.11894817549581));
#67031=CARTESIAN_POINT('Ctrl Pts',(15.0212721603102,-2.60686763581553,1.91180372236777));
#67032=CARTESIAN_POINT('Ctrl Pts',(15.0381290141231,-2.74947143401784,1.70032551873446));
#67033=CARTESIAN_POINT('Ctrl Pts',(15.0653273647175,-2.93348460514272,1.34265383993753));
#67034=CARTESIAN_POINT('Ctrl Pts',(15.0753954484817,-2.99208155291536,1.20644206339538));
#67035=CARTESIAN_POINT('Ctrl Pts',(15.088938678542,-3.05985094226806,1.0132313997135));
#67036=CARTESIAN_POINT('Ctrl Pts',(15.0926420034621,-3.07718681979923,0.959295432964452));
#67037=CARTESIAN_POINT('Ctrl Pts',(15.0982656059838,-3.10177403119091,0.875254955112782));
#67038=CARTESIAN_POINT('Ctrl Pts',(15.1002314095604,-3.1100280791091,0.845457801342096));
#67039=CARTESIAN_POINT('Ctrl Pts',(15.1026617548289,-3.11981850414629,0.808028728741279));
#67040=CARTESIAN_POINT('Ctrl Pts',(15.1031483212269,-3.12175744311823,0.800505087169984));
#67041=CARTESIAN_POINT('Ctrl Pts',(15.1039175880348,-3.12478959995272,0.788560874766613));
#67042=CARTESIAN_POINT('Ctrl Pts',(15.1042013076125,-3.1259006740415,0.784144931645784));
#67043=CARTESIAN_POINT('Ctrl Pts',(15.10473541078,-3.12797866879361,0.775811376743137));
#67044=CARTESIAN_POINT('Ctrl Pts',(15.1049859044795,-3.12894757979536,0.771894350149719));
#67045=CARTESIAN_POINT('Ctrl Pts',(15.1055593084457,-3.1311524458972,0.762908345985083));
#67046=CARTESIAN_POINT('Ctrl Pts',(15.1058819296038,-3.13238344779115,0.757838189019702));
#67047=CARTESIAN_POINT('Ctrl Pts',(15.1068781614429,-3.13615483938944,0.742138680627024));
#67048=CARTESIAN_POINT('Ctrl Pts',(15.1075494038975,-3.13865351086278,0.731499244486191));
#67049=CARTESIAN_POINT('Ctrl Pts',(15.1131260617385,-3.15905091643544,0.642617359995613));
#67050=CARTESIAN_POINT('Ctrl Pts',(15.1178758687404,-3.17407673875217,0.563736680675645));
#67051=CARTESIAN_POINT('Ctrl Pts',(15.1242663352804,-3.19064097886558,0.454778629523579));
#67052=CARTESIAN_POINT('Ctrl Pts',(15.1259883526809,-3.19472723681376,0.425125184903111));
#67053=CARTESIAN_POINT('Ctrl Pts',(15.1352016288248,-3.21449585385841,0.265223841976268));
#67054=CARTESIAN_POINT('Ctrl Pts',(15.1424995742806,-3.22262790300222,0.134162465310681));
#67055=CARTESIAN_POINT('Ctrl Pts',(15.1553204624045,-3.22283895868667,-0.0951862285488035));
#67056=CARTESIAN_POINT('Ctrl Pts',(15.1608197253378,-3.21844527033867,-0.193288392988242));
#67057=CARTESIAN_POINT('Ctrl Pts',(15.1698768604655,-3.20407840080513,-0.35172904129138));
#67058=CARTESIAN_POINT('Ctrl Pts',(15.1733781283162,-3.19685446179728,-0.412253244994023));
#67059=CARTESIAN_POINT('Ctrl Pts',(15.1820158470909,-3.17508980198272,-0.559087030677871));
#67060=CARTESIAN_POINT('Ctrl Pts',(15.1871969743326,-3.158741832144,-0.645074818197823));
#67061=CARTESIAN_POINT('Ctrl Pts',(15.1934149677491,-3.13545869355486,-0.745150498364081));
#67062=CARTESIAN_POINT('Ctrl Pts',(15.1943418804486,-3.13189482547814,-0.759990311719795));
#67063=CARTESIAN_POINT('Ctrl Pts',(15.1958391620589,-3.12598957568767,-0.78383240986947));
#67064=CARTESIAN_POINT('Ctrl Pts',(15.1964073931163,-3.12371436250361,-0.792850964999574));
#67065=CARTESIAN_POINT('Ctrl Pts',(15.197420962456,-3.11959561171698,-0.808884035419884));
#67066=CARTESIAN_POINT('Ctrl Pts',(15.1978658025011,-3.11776736885509,-0.815902442536883));
#67067=CARTESIAN_POINT('Ctrl Pts',(15.1987960983281,-3.11390116040694,-0.830541603241341));
#67068=CARTESIAN_POINT('Ctrl Pts',(15.1992816918438,-3.11185887609818,-0.838161156926052));
#67069=CARTESIAN_POINT('Ctrl Pts',(15.200547766653,-3.10647135981199,-0.857970296477163));
#67070=CARTESIAN_POINT('Ctrl Pts',(15.2013296676057,-3.10308237571739,-0.870147746745694));
#67071=CARTESIAN_POINT('Ctrl Pts',(15.204729019631,-3.08808269305092,-0.922843078558261));
#67072=CARTESIAN_POINT('Ctrl Pts',(15.2073699464865,-3.07574982212357,-0.96314943106514));
#67073=CARTESIAN_POINT('Ctrl Pts',(15.2143482361777,-3.04141714958041,-1.06796223163581));
#67074=CARTESIAN_POINT('Ctrl Pts',(15.2187255700755,-3.01815637667191,-1.13203029760212));
#67075=CARTESIAN_POINT('Ctrl Pts',(15.2328222448072,-2.9378529266205,-1.33309865482892));
#67076=CARTESIAN_POINT('Ctrl Pts',(15.2427558789215,-2.8733776754647,-1.46690988692199));
#67077=CARTESIAN_POINT('Ctrl Pts',(15.255315224363,-2.78135503792632,-1.62836966183403));
#67078=CARTESIAN_POINT('Ctrl Pts',(15.257853505674,-2.76222066299254,-1.66062054375748));
#67079=CARTESIAN_POINT('Ctrl Pts',(15.2738409268937,-2.63817479943112,-1.86162096321881));
#67080=CARTESIAN_POINT('Ctrl Pts',(15.2872793758239,-2.51839415295489,-2.02071989769385));
#67081=CARTESIAN_POINT('Ctrl Pts',(15.3004851134808,-2.37768012851168,-2.17551462653088));
#67082=CARTESIAN_POINT('Ctrl Pts',(15.3011419386871,-2.37061588937,-2.18321025003884));
#67083=CARTESIAN_POINT('Ctrl Pts',(15.302122791084,-2.35996619158621,-2.19469915400406));
#67084=CARTESIAN_POINT('Ctrl Pts',(15.3024488831076,-2.35640881691023,-2.198518203362));
#67085=CARTESIAN_POINT('Ctrl Pts',(15.303010798871,-2.35024944718996,-2.20509852227101));
#67086=CARTESIAN_POINT('Ctrl Pts',(15.3032469556684,-2.34765183821192,-2.20786385536685));
#67087=CARTESIAN_POINT('Ctrl Pts',(15.3037389346192,-2.34222135147988,-2.21362456174629));
#67088=CARTESIAN_POINT('Ctrl Pts',(15.3039946846047,-2.33938760754884,-2.21661908805895));
#67089=CARTESIAN_POINT('Ctrl Pts',(15.3046078462457,-2.3325680496375,-2.22379793399773));
#67090=CARTESIAN_POINT('Ctrl Pts',(15.3049648293645,-2.32857668705824,-2.22797701315815));
#67091=CARTESIAN_POINT('Ctrl Pts',(15.3061862429921,-2.31484911027079,-2.24227302157284));
#67092=CARTESIAN_POINT('Ctrl Pts',(15.3070464946323,-2.30505786383752,-2.25233722334539));
#67093=CARTESIAN_POINT('Ctrl Pts',(15.3091041753893,-2.28135148221348,-2.27638797342363));
#67094=CARTESIAN_POINT('Ctrl Pts',(15.3102969940665,-2.26737291084877,-2.29031153256187));
#67095=CARTESIAN_POINT('Ctrl Pts',(15.3147081530182,-2.21484036184344,-2.34168497068751));
#67096=CARTESIAN_POINT('Ctrl Pts',(15.3178722262048,-2.17547738976182,-2.37829878942329));
#67097=CARTESIAN_POINT('Ctrl Pts',(15.3256834473043,-2.07469185987813,-2.46744813403822));
#67098=CARTESIAN_POINT('Ctrl Pts',(15.3302731419139,-2.01217375151787,-2.51869107470802));
#67099=CARTESIAN_POINT('Ctrl Pts',(15.3458566208664,-1.79165955667816,-2.68597853535667));
#67100=CARTESIAN_POINT('Ctrl Pts',(15.3566468053936,-1.62505228326975,-2.78993353290938));
#67101=CARTESIAN_POINT('Ctrl Pts',(15.3703716835656,-1.41079657455153,-2.89787870123314));
#67102=CARTESIAN_POINT('Ctrl Pts',(15.372903387189,-1.37115997513711,-2.91684213785507));
#67103=CARTESIAN_POINT('Ctrl Pts',(15.376288466089,-1.31814348395038,-2.94088749506775));
#67104=CARTESIAN_POINT('Ctrl Pts',(15.3771212493929,-1.3050989191316,-2.94669956156003));
#67105=CARTESIAN_POINT('Ctrl Pts',(15.3824145608504,-1.22219410977495,-2.98297969580263));
#67106=CARTESIAN_POINT('Ctrl Pts',(15.386943377462,-1.151314763883,-3.01104619992293));
#67107=CARTESIAN_POINT('Ctrl Pts',(15.3924426477417,-1.06574143531627,-3.04146779143902));
#67108=CARTESIAN_POINT('Ctrl Pts',(15.3933305980832,-1.05193866599805,-3.046269220761));
#67109=CARTESIAN_POINT('Ctrl Pts',(15.3947829677527,-1.02938884784141,-3.05394186381261));
#67110=CARTESIAN_POINT('Ctrl Pts',(15.395345505136,-1.02066121084517,-3.05686980382081));
#67111=CARTESIAN_POINT('Ctrl Pts',(15.3963514560325,-1.00506633998423,-3.06202732573919));
#67112=CARTESIAN_POINT('Ctrl Pts',(15.3967943901735,-0.998203906188465,
-3.06427130842962));
#67113=CARTESIAN_POINT('Ctrl Pts',(15.3977308002374,-0.983705241246241,
-3.06895842943831));
#67114=CARTESIAN_POINT('Ctrl Pts',(15.3982244507343,-0.976067327852589,
-3.07139616671605));
#67115=CARTESIAN_POINT('Ctrl Pts',(15.3995345521572,-0.9558119294269,-3.07777774908896));
#67116=CARTESIAN_POINT('Ctrl Pts',(15.400352611083,-0.943179238304977,-3.08167247339529));
#67117=CARTESIAN_POINT('Ctrl Pts',(15.4041416232694,-0.884742878128455,
-3.09929573406158));
#67118=CARTESIAN_POINT('Ctrl Pts',(15.4071432244256,-0.838663184494064,
-3.11208092343156));
#67119=CARTESIAN_POINT('Ctrl Pts',(15.4153111159994,-0.713913224274812,
-3.14372203765289));
#67120=CARTESIAN_POINT('Ctrl Pts',(15.4205363034389,-0.634793459361312,
-3.16064800500406));
#67121=CARTESIAN_POINT('Ctrl Pts',(15.4485974163442,-0.213283363532098,
-3.23435579154359));
#67122=CARTESIAN_POINT('Ctrl Pts',(15.4729307886101,0.135909696031122,-3.23852275724333));
#67123=CARTESIAN_POINT('Ctrl Pts',(15.4967462405727,0.504058717654823,-3.18318763662073));
#67124=CARTESIAN_POINT('Ctrl Pts',(15.4983523187759,0.529054262969654,-3.17912887477608));
#67125=CARTESIAN_POINT('Ctrl Pts',(15.5004172824748,0.561446927873938,-3.17347633531926));
#67126=CARTESIAN_POINT('Ctrl Pts',(15.5008905744842,0.56888907210638,-3.17215067895932));
#67127=CARTESIAN_POINT('Ctrl Pts',(15.5016436787339,0.580760578997237,-3.16999290572147));
#67128=CARTESIAN_POINT('Ctrl Pts',(15.5019244391387,0.585192923528332,-3.16917767177688));
#67129=CARTESIAN_POINT('Ctrl Pts',(15.5024310026801,0.593202241155556,-3.16768715531785));
#67130=CARTESIAN_POINT('Ctrl Pts',(15.5026569863704,0.596779740329687,-3.1670151175114));
#67131=CARTESIAN_POINT('Ctrl Pts',(15.5031975247657,0.605347415102063,-3.16539063591076));
#67132=CARTESIAN_POINT('Ctrl Pts',(15.5035117477796,0.610336479364641,-3.16443245364495));
#67133=CARTESIAN_POINT('Ctrl Pts',(15.5044571775658,0.625372430026128,-3.16150781937738));
#67134=CARTESIAN_POINT('Ctrl Pts',(15.5050863520346,0.635412350050198,-3.15950526510695));
#67135=CARTESIAN_POINT('Ctrl Pts',(15.5110795427846,0.731346983542837,-3.13989443523806));
#67136=CARTESIAN_POINT('Ctrl Pts',(15.5162558297956,0.816507745941176,-3.11883370608293));
#67137=CARTESIAN_POINT('Ctrl Pts',(15.5304697659594,1.05263149988107,-3.05010159669894));
#67138=CARTESIAN_POINT('Ctrl Pts',(15.5392525652299,1.20109819810997,-2.99474911639553));
#67139=CARTESIAN_POINT('Ctrl Pts',(15.561470987037,1.56222477878012,-2.82891467766525));
#67140=CARTESIAN_POINT('Ctrl Pts',(15.5749707882375,1.76772718792067,-2.70525833464536));
#67141=CARTESIAN_POINT('Ctrl Pts',(15.5905959944686,1.97324424675203,-2.54809929497118));
#67142=CARTESIAN_POINT('Ctrl Pts',(15.591786958381,1.98872748382345,-2.53603348619014));
#67143=CARTESIAN_POINT('Ctrl Pts',(15.593548556136,2.01135777207077,-2.51806341900508));
#67144=CARTESIAN_POINT('Ctrl Pts',(15.5941148185644,2.01859131530457,-2.51226841088885));
#67145=CARTESIAN_POINT('Ctrl Pts',(15.5951261357562,2.03143668054732,-2.50188631001886));
#67146=CARTESIAN_POINT('Ctrl Pts',(15.595570700121,2.03705823804988,-2.49731131995249));
#67147=CARTESIAN_POINT('Ctrl Pts',(15.5965017063793,2.04877813077054,-2.48770742106146));
#67148=CARTESIAN_POINT('Ctrl Pts',(15.5969882906561,2.05487348657019,-2.48267496751795));
#67149=CARTESIAN_POINT('Ctrl Pts',(15.5982597846743,2.07072277277213,-2.46949111058253));
#67150=CARTESIAN_POINT('Ctrl Pts',(15.5990461367697,2.08044702611454,-2.4613043921902));
#67151=CARTESIAN_POINT('Ctrl Pts',(15.6024911951489,2.12270832461477,-2.42529578505876));
#67152=CARTESIAN_POINT('Ctrl Pts',(15.6051741656447,2.1547363615124,-2.39688573025646));
#67153=CARTESIAN_POINT('Ctrl Pts',(15.6122881886908,2.23731771231515,-2.32063995671971));
#67154=CARTESIAN_POINT('Ctrl Pts',(15.6167611636337,2.28690180192743,-2.27179209815806));
#67155=CARTESIAN_POINT('Ctrl Pts',(15.6373150395803,2.50431372361843,-2.04327334661744));
#67156=CARTESIAN_POINT('Ctrl Pts',(15.6541170110741,2.65281417726106,-1.84637534088398));
#67157=CARTESIAN_POINT('Ctrl Pts',(15.6797977590894,2.84648061589473,-1.51729306187853));
#67158=CARTESIAN_POINT('Ctrl Pts',(15.6888201663959,2.90800355561298,-1.39576313229773));
#67159=CARTESIAN_POINT('Ctrl Pts',(15.6980958187008,2.96591460070476,-1.2607871936792));
#67160=CARTESIAN_POINT('Ctrl Pts',(15.698773833461,2.97011529001045,-1.25085927992975));
#67161=CARTESIAN_POINT('Ctrl Pts',(15.6997809665278,2.97630779311625,-1.23601682739945));
#67162=CARTESIAN_POINT('Ctrl Pts',(15.7001123034902,2.9783373689397,-1.23111826999285));
#67163=CARTESIAN_POINT('Ctrl Pts',(15.700680832198,2.98180674810264,-1.22268583055916));
#67164=CARTESIAN_POINT('Ctrl Pts',(15.7009183751292,2.98325237358707,-1.21915437871109));
#67165=CARTESIAN_POINT('Ctrl Pts',(15.7014107207519,2.98624052192831,-1.21181762946941));
#67166=CARTESIAN_POINT('Ctrl Pts',(15.7016654588692,2.98778204406975,-1.20801195325481));
#67167=CARTESIAN_POINT('Ctrl Pts',(15.7022719817961,2.99144138693292,-1.19892799457506));
#67168=CARTESIAN_POINT('Ctrl Pts',(15.7026233617654,2.99355252982742,-1.19364699973163));
#67169=CARTESIAN_POINT('Ctrl Pts',(15.7038059384463,3.00062718525627,-1.17581302487944));
#67170=CARTESIAN_POINT('Ctrl Pts',(15.7046333068759,3.00552588949837,-1.16323424847324));
#67171=CARTESIAN_POINT('Ctrl Pts',(15.7066001968583,3.01704402313385,-1.13309969751068));
#67172=CARTESIAN_POINT('Ctrl Pts',(15.7077356284515,3.02358954148022,-1.11551597171177));
#67173=CARTESIAN_POINT('Ctrl Pts',(15.7235587087532,3.11326505178351,-0.868024261195266));
#67174=CARTESIAN_POINT('Ctrl Pts',(15.736949543964,3.1701366631343,-0.629408072058027));
#67175=CARTESIAN_POINT('Ctrl Pts',(15.7627845220379,3.22545553185205,-0.171624807649652));
#67176=CARTESIAN_POINT('Ctrl Pts',(15.7751026879613,3.22969604652536,0.0454146241689535));
#67177=CARTESIAN_POINT('Ctrl Pts',(15.7892592668255,3.21069222996387,0.279095864381373));
#67178=CARTESIAN_POINT('Ctrl Pts',(15.7903465476792,3.20908966795408,0.296955518588385));
#67179=CARTESIAN_POINT('Ctrl Pts',(15.7919966615134,3.20644288773968,0.323922174146647));
#67180=CARTESIAN_POINT('Ctrl Pts',(15.7925560324063,3.20550870291503,0.333039817511544));
#67181=CARTESIAN_POINT('Ctrl Pts',(15.7935303797795,3.20381747362355,0.348879515359437));
#67182=CARTESIAN_POINT('Ctrl Pts',(15.7939447958039,3.2030781316616,0.355603433474069));
#67183=CARTESIAN_POINT('Ctrl Pts',(15.7948103564142,3.20149228802624,0.369619512855863));
#67184=CARTESIAN_POINT('Ctrl Pts',(15.7952616173622,3.20064202917643,0.376911202039747));
#67185=CARTESIAN_POINT('Ctrl Pts',(15.7963302239336,3.19857323153404,0.394140958194536));
#67186=CARTESIAN_POINT('Ctrl Pts',(15.796948243093,3.19733328341281,0.404076333835586));
#67187=CARTESIAN_POINT('Ctrl Pts',(15.798997581415,3.19307834974241,0.436923632570207));
#67188=CARTESIAN_POINT('Ctrl Pts',(15.8004352130785,3.18986327516766,0.45980849184632));
#67189=CARTESIAN_POINT('Ctrl Pts',(15.8038381076063,3.18171570045026,0.513597182729975));
#67190=CARTESIAN_POINT('Ctrl Pts',(15.805809715637,3.17657869430164,0.544467218981702));
#67191=CARTESIAN_POINT('Ctrl Pts',(15.8128778197582,3.15669554481401,0.654069296796966));
#67192=CARTESIAN_POINT('Ctrl Pts',(15.8180503151655,3.13946581219031,0.732315558280276));
#67193=CARTESIAN_POINT('Ctrl Pts',(15.8455858022309,3.03390834483839,1.13890478421955));
#67194=CARTESIAN_POINT('Ctrl Pts',(15.8693825382955,2.89696416664439,1.45232811371252));
#67195=CARTESIAN_POINT('Ctrl Pts',(15.8933141668011,2.69622765946527,1.76564732350463));
#67196=CARTESIAN_POINT('Ctrl Pts',(15.8953636228226,2.67845390515615,1.79249516892775));
#67197=CARTESIAN_POINT('Ctrl Pts',(15.8979019589517,2.65566267829451,1.82582590032601));
#67198=CARTESIAN_POINT('Ctrl Pts',(15.8984145599822,2.65101959655277,1.8325609352295));
#67199=CARTESIAN_POINT('Ctrl Pts',(15.8992185662069,2.64367214466132,1.84313243797375));
#67200=CARTESIAN_POINT('Ctrl Pts',(15.8995111226179,2.64098499098507,1.84698074446687));
#67201=CARTESIAN_POINT('Ctrl Pts',(15.900052949987,2.63598276068994,1.85411126416736));
#67202=CARTESIAN_POINT('Ctrl Pts',(15.9003023695789,2.63366997724544,1.85739498917685));
#67203=CARTESIAN_POINT('Ctrl Pts',(15.9008619838766,2.62845818105451,1.86476546996866));
#67204=CARTESIAN_POINT('Ctrl Pts',(15.9011719409318,2.6255557822597,1.86884978063817));
#67205=CARTESIAN_POINT('Ctrl Pts',(15.9020921042403,2.6168931604609,1.88097997452616));
#67206=CARTESIAN_POINT('Ctrl Pts',(15.9027004356467,2.61110532934405,1.88900620509603));
#67207=CARTESIAN_POINT('Ctrl Pts',(15.9078416680229,2.56168290411548,1.95688121330853));
#67208=CARTESIAN_POINT('Ctrl Pts',(15.912241021053,2.516030131726,2.01524135599555));
#67209=CARTESIAN_POINT('Ctrl Pts',(15.923829090987,2.38808002716268,2.16767149428997));
#67210=CARTESIAN_POINT('Ctrl Pts',(15.9308516713183,2.30225526879232,2.25861703209239));
#67211=CARTESIAN_POINT('Ctrl Pts',(15.9436357222225,2.13604899462007,2.41539455626853));
#67212=CARTESIAN_POINT('Ctrl Pts',(15.9493991598353,2.05735765213357,2.48276364463649));
#67213=CARTESIAN_POINT('Ctrl Pts',(15.9595464858926,1.91510056143496,2.59313777271369));
#67214=CARTESIAN_POINT('Ctrl Pts',(15.9638922988872,1.85301808146851,2.63785635465237));
#67215=CARTESIAN_POINT('Ctrl Pts',(15.9683010644095,1.78943598014216,2.68030528773732));
#67216=CARTESIAN_POINT('Origin',(-1.72497344927317,0.,0.));
#67217=CARTESIAN_POINT('',(17.4669156580687,1.78943621037803,2.68030513402633));
#67218=CARTESIAN_POINT('',(17.218344821656,1.78943620926209,2.68030513477136));
#67219=CARTESIAN_POINT('',(-1.72497344927317,1.78943621037804,2.68030513402633));
#67220=CARTESIAN_POINT('',(16.646573449236,-3.2227488963424,-0.00266713776262383));
#67221=CARTESIAN_POINT('Ctrl Pts',(16.6465734492731,-3.2227488963419,-0.0026671383622827));
#67222=CARTESIAN_POINT('Ctrl Pts',(16.6563207021309,-3.22261856278451,-0.160151404718748));
#67223=CARTESIAN_POINT('Ctrl Pts',(16.6660679549888,-3.21094182220305,-0.317172978826481));
#67224=CARTESIAN_POINT('Ctrl Pts',(16.6758152078467,-3.18793726157565,-0.472412509103579));
#67225=CARTESIAN_POINT('Ctrl Pts',(16.6772288474639,-3.18460092068508,-0.494926827072348));
#67226=CARTESIAN_POINT('Ctrl Pts',(16.6786424870812,-3.18102638060837,-0.517403721746265));
#67227=CARTESIAN_POINT('Ctrl Pts',(16.6800561266984,-3.17721437437539,-0.539839218436775));
#67228=CARTESIAN_POINT('Ctrl Pts',(16.6862283747912,-3.16057035286246,-0.637797318908653));
#67229=CARTESIAN_POINT('Ctrl Pts',(16.692400622884,-3.13936250720821,-0.735157376286323));
#67230=CARTESIAN_POINT('Ctrl Pts',(16.6985728709767,-3.11364577400216,-0.831461097429376));
#67231=CARTESIAN_POINT('Ctrl Pts',(16.7047367596294,-3.08796387048676,-0.92763438875508));
#67232=CARTESIAN_POINT('Ctrl Pts',(16.710900648282,-3.05778532814494,-1.02275377146286));
#67233=CARTESIAN_POINT('Ctrl Pts',(16.7170645369346,-3.02321645072212,-1.11636904945593));
#67234=CARTESIAN_POINT('Ctrl Pts',(16.7232218985932,-2.98868417857741,-1.20988519743548));
#67235=CARTESIAN_POINT('Ctrl Pts',(16.7293792602517,-2.94977096356845,-1.30190000192231));
#67236=CARTESIAN_POINT('Ctrl Pts',(16.7355366219103,-2.9066332198159,-1.39197733026175));
#67237=CARTESIAN_POINT('Ctrl Pts',(16.7416894860566,-2.86352698509944,-1.48198886355627));
#67238=CARTESIAN_POINT('Ctrl Pts',(16.7478423502029,-2.81620254362144,-1.57006534375197));
#67239=CARTESIAN_POINT('Ctrl Pts',(16.7539952143492,-2.7648644811798,-1.65579043456904));
#67240=CARTESIAN_POINT('Ctrl Pts',(16.7601457474857,-2.71354586813964,-1.74148304847468));
#67241=CARTESIAN_POINT('Ctrl Pts',(16.7662962806223,-2.65821687840365,-1.82482567081586));
#67242=CARTESIAN_POINT('Ctrl Pts',(16.7724468137588,-2.59912768898054,-1.90542720114799));
#67243=CARTESIAN_POINT('Ctrl Pts',(16.778596661974,-2.54004507970996,-1.98601975572046));
#67244=CARTESIAN_POINT('Ctrl Pts',(16.7847465101892,-2.47720336007928,-2.06387147483843));
#67245=CARTESIAN_POINT('Ctrl Pts',(16.7908963584045,-2.41089502801246,-2.13862168847247));
#67246=CARTESIAN_POINT('Ctrl Pts',(16.7970471667836,-2.34457634335384,-2.21338357271296));
#67247=CARTESIAN_POINT('Ctrl Pts',(16.8031979751627,-2.27479025950479,-2.2850426646788));
#67248=CARTESIAN_POINT('Ctrl Pts',(16.8093487835419,-2.20186772104511,-2.35327348634187));
#67249=CARTESIAN_POINT('Ctrl Pts',(16.815506169908,-2.128867195517,-2.421577277513));
#67250=CARTESIAN_POINT('Ctrl Pts',(16.8216635562742,-2.0527238350218,-2.48644517967099));
#67251=CARTESIAN_POINT('Ctrl Pts',(16.8278209426404,-1.97380332741507,-2.54759062393965));
#67252=CARTESIAN_POINT('Ctrl Pts',(16.8339817653774,-1.89483877512612,-2.60877019281981));
#67253=CARTESIAN_POINT('Ctrl Pts',(16.8401425881143,-1.81309434452169,-2.66622291678952));
#67254=CARTESIAN_POINT('Ctrl Pts',(16.8463034108513,-1.72896476084045,-2.71970557565923));
#67255=CARTESIAN_POINT('Ctrl Pts',(16.852474533768,-1.64469452227114,-2.7732776513199));
#67256=CARTESIAN_POINT('Ctrl Pts',(16.8586456566847,-1.55803154251315,-2.82286618787387));
#67257=CARTESIAN_POINT('Ctrl Pts',(16.8648167796014,-1.46939530811457,-2.86827386959316));
#67258=CARTESIAN_POINT('Ctrl Pts',(16.8695123015469,-1.40195322514026,-2.90282394563104));
#67259=CARTESIAN_POINT('Ctrl Pts',(16.8742078234925,-1.33336924323071,-2.93495447708597));
#67260=CARTESIAN_POINT('Ctrl Pts',(16.8789033454381,-1.2638347816207,-2.96459764677532));
#67261=CARTESIAN_POINT('Ctrl Pts',(16.8850755935309,-1.1724319614384,-3.00356349544968));
#67262=CARTESIAN_POINT('Ctrl Pts',(16.8912478416236,-1.07906451399484,-3.03836684654929));
#67263=CARTESIAN_POINT('Ctrl Pts',(16.8974200897164,-0.98414766434149,-3.0688061094294));
#67264=CARTESIAN_POINT('Ctrl Pts',(16.903583978369,-0.889359366183593,-3.09920414661798));
#67265=CARTESIAN_POINT('Ctrl Pts',(16.9097478670217,-0.793026246694331,
-3.12524971196125));
#67266=CARTESIAN_POINT('Ctrl Pts',(16.9159117556743,-0.695584494367052,
-3.14678880347826));
#67267=CARTESIAN_POINT('Ctrl Pts',(16.9220691173328,-0.598245923939434,
-3.16830508706821));
#67268=CARTESIAN_POINT('Ctrl Pts',(16.9282264789914,-0.499801476377009,
-3.18532429066935));
#67269=CARTESIAN_POINT('Ctrl Pts',(16.93438384065,-0.400702605073226,-3.19774216984227));
#67270=CARTESIAN_POINT('Ctrl Pts',(16.9405367047963,-0.301676118406173,
-3.21015097864273));
#67271=CARTESIAN_POINT('Ctrl Pts',(16.9466895689426,-0.201996588068138,
-3.21796509128979));
#67272=CARTESIAN_POINT('Ctrl Pts',(16.9528424330889,-0.102124861484679,
-3.2211314898909));
#67273=CARTESIAN_POINT('Ctrl Pts',(16.9589929662254,-0.00229097125920541,
-3.22429668890334));
#67274=CARTESIAN_POINT('Ctrl Pts',(16.965143499362,0.0977345368565912,-3.22281765878928));
#67275=CARTESIAN_POINT('Ctrl Pts',(16.9712940324985,0.197487392412191,-3.2166933786636));
#67276=CARTESIAN_POINT('Ctrl Pts',(16.9774438807137,0.297229139522876,-3.21056978053573));
#67277=CARTESIAN_POINT('Ctrl Pts',(16.9835937289289,0.396697860879073,-3.1998019874695));
#67278=CARTESIAN_POINT('Ctrl Pts',(16.9897435771441,0.495432001014504,-3.18444103334805));
#67279=CARTESIAN_POINT('Ctrl Pts',(16.9958943855233,0.594181556320692,-3.16907768095047));
#67280=CARTESIAN_POINT('Ctrl Pts',(17.0020451939024,0.692195873352404,-3.14911980989199));
#67281=CARTESIAN_POINT('Ctrl Pts',(17.0081960022815,0.789022211968121,-3.1246698244008));
#67282=CARTESIAN_POINT('Ctrl Pts',(17.0143533886477,0.885952101590818,-3.10019369085265));
#67283=CARTESIAN_POINT('Ctrl Pts',(17.0205107750139,0.981691053794507,-3.07121595614433));
#67284=CARTESIAN_POINT('Ctrl Pts',(17.0266681613801,1.07580027311818,-3.03788928943417));
#67285=CARTESIAN_POINT('Ctrl Pts',(17.0328289841171,1.16996201377982,-3.00454402347158));
#67286=CARTESIAN_POINT('Ctrl Pts',(17.038989806854,1.26249180795012,-2.9668451558868));
#67287=CARTESIAN_POINT('Ctrl Pts',(17.045150629591,1.35297162465931,-2.92499322142236));
#67288=CARTESIAN_POINT('Ctrl Pts',(17.0513217525077,1.44360271310833,-2.88307131538666));
#67289=CARTESIAN_POINT('Ctrl Pts',(17.0574928754244,1.53217659261148,-2.83698267375057));
#67290=CARTESIAN_POINT('Ctrl Pts',(17.063663998341,1.61830045874771,-2.78697348170322));
#67291=CARTESIAN_POINT('Ctrl Pts',(17.0683595202866,1.68383091551223,-2.74892218019634));
#67292=CARTESIAN_POINT('Ctrl Pts',(17.0730550422322,1.74794346625185,-2.70860203059588));
#67293=CARTESIAN_POINT('Ctrl Pts',(17.0777505641778,1.81047756020777,-2.66613738702343));
#67294=CARTESIAN_POINT('Ctrl Pts',(17.0839228122705,1.89267842022412,-2.61031775326647));
#67295=CARTESIAN_POINT('Ctrl Pts',(17.0900950603633,1.9724400442519,-2.55059475248506));
#67296=CARTESIAN_POINT('Ctrl Pts',(17.0962673084561,2.04936833600685,-2.48720867356813));
#67297=CARTESIAN_POINT('Ctrl Pts',(17.1024311971087,2.12619243923277,-2.42390844216154));
#67298=CARTESIAN_POINT('Ctrl Pts',(17.1085950857613,2.2001905050555,-2.35695526718765));
#67299=CARTESIAN_POINT('Ctrl Pts',(17.114758974414,2.27099713405129,-2.28663280384736));
#67300=CARTESIAN_POINT('Ctrl Pts',(17.1209163360725,2.34172878530586,-2.21638480556116));
#67301=CARTESIAN_POINT('Ctrl Pts',(17.1270736977311,2.40927541187636,-2.14277491637476));
#67302=CARTESIAN_POINT('Ctrl Pts',(17.1332310593896,2.47330521693873,-2.06612653687127));
#67303=CARTESIAN_POINT('Ctrl Pts',(17.1393839235359,2.53728825280869,-1.98953414352619));
#67304=CARTESIAN_POINT('Ctrl Pts',(17.1455367876822,2.59775929671622,-1.90990800476759));
#67305=CARTESIAN_POINT('Ctrl Pts',(17.1516896518285,2.65442456461577,-1.82760712224055));
#67306=CARTESIAN_POINT('Ctrl Pts',(17.1578401849651,2.71106836490448,-1.74533741936523));
#67307=CARTESIAN_POINT('Ctrl Pts',(17.1639907181016,2.763909008008,-1.66039534357055));
#67308=CARTESIAN_POINT('Ctrl Pts',(17.1701412512381,2.81269459936232,-1.57317089129504));
#67309=CARTESIAN_POINT('Ctrl Pts',(17.1762910994534,2.86147475796937,-1.4859561523056));
#67310=CARTESIAN_POINT('Ctrl Pts',(17.1824409476686,2.90620055057427,-1.39645992125861));
#67311=CARTESIAN_POINT('Ctrl Pts',(17.1885907958838,2.94666533956786,-1.30509805726981));
#67312=CARTESIAN_POINT('Ctrl Pts',(17.1947416042629,2.98713644625085,-1.21372192912952));
#67313=CARTESIAN_POINT('Ctrl Pts',(17.200892412642,3.02334505201687,-1.12047998669558));
#67314=CARTESIAN_POINT('Ctrl Pts',(17.2070432210212,3.05513249898531,-1.02580845002554));
#67315=CARTESIAN_POINT('Ctrl Pts',(17.2132006073874,3.08695394106489,-0.931035666803198));
#67316=CARTESIAN_POINT('Ctrl Pts',(17.2193579937535,3.11434464406396,-0.834830648913799));
#67317=CARTESIAN_POINT('Ctrl Pts',(17.2255153801197,3.13719577344072,-0.737645064787729));
#67318=CARTESIAN_POINT('Ctrl Pts',(17.2316762028567,3.16005965578577,-0.640405242437708));
#67319=CARTESIAN_POINT('Ctrl Pts',(17.2378370255936,3.17837883945993,-0.542184191049059));
#67320=CARTESIAN_POINT('Ctrl Pts',(17.2439978483306,3.19209598245055,-0.443441993188545));
#67321=CARTESIAN_POINT('Ctrl Pts',(17.2501689712473,3.20583605891033,-0.344534709847042));
#67322=CARTESIAN_POINT('Ctrl Pts',(17.256340094164,3.214958686299,-0.245104972405858));
#67323=CARTESIAN_POINT('Ctrl Pts',(17.2625112170807,3.21945856441972,-0.145616326297994));
#67324=CARTESIAN_POINT('Ctrl Pts',(17.2672067390262,3.22288245934995,-0.0699167935805051));
#67325=CARTESIAN_POINT('Ctrl Pts',(17.2719022609718,3.22363110273314,0.00581677334481895));
#67326=CARTESIAN_POINT('Ctrl Pts',(17.2765977829174,3.22172229092571,0.0813820782016825));
#67327=CARTESIAN_POINT('Ctrl Pts',(17.2827702109138,3.21921309097379,0.180715317117513));
#67328=CARTESIAN_POINT('Ctrl Pts',(17.2889426389102,3.21210115545655,0.280107242932961));
#67329=CARTESIAN_POINT('Ctrl Pts',(17.2951150669066,3.20037552543264,0.379096371272234));
#67330=CARTESIAN_POINT('Ctrl Pts',(17.3012790891514,3.18866586363608,0.477950693984469));
#67331=CARTESIAN_POINT('Ctrl Pts',(17.3074431113961,3.172355046599,0.576402881916098));
#67332=CARTESIAN_POINT('Ctrl Pts',(17.3136071336409,3.15148411714757,0.673992152674372));
#67333=CARTESIAN_POINT('Ctrl Pts',(17.3199949888254,3.12985530569827,0.775125163622305));
#67334=CARTESIAN_POINT('Ctrl Pts',(17.3263828440099,3.10332887786078,0.875330920908748));
#67335=CARTESIAN_POINT('Ctrl Pts',(17.3327706991944,3.07200934862504,0.974102727878518));
#67336=CARTESIAN_POINT('Ctrl Pts',(17.3389233296928,3.04184312143185,1.06923738801037));
#67337=CARTESIAN_POINT('Ctrl Pts',(17.3450759601912,3.00723071574878,1.16304138810687));
#67338=CARTESIAN_POINT('Ctrl Pts',(17.3512285906897,2.96831713035872,1.25507409188422));
#67339=CARTESIAN_POINT('Ctrl Pts',(17.3573788863308,2.929418312257,1.34707187023743));
#67340=CARTESIAN_POINT('Ctrl Pts',(17.363529181972,2.88622172737016,1.43729928857426));
#67341=CARTESIAN_POINT('Ctrl Pts',(17.3696794776131,2.83892100630479,1.52533441659899));
#67342=CARTESIAN_POINT('Ctrl Pts',(17.3758290844128,2.79162558298445,1.61335968456978));
#67343=CARTESIAN_POINT('Ctrl Pts',(17.3819786912125,2.74022714357916,1.69919276816272));
#67344=CARTESIAN_POINT('Ctrl Pts',(17.3881282980121,2.68496542556838,1.78243603700172));
#67345=CARTESIAN_POINT('Ctrl Pts',(17.394278860962,2.62969511538211,1.86569224863005));
#67346=CARTESIAN_POINT('Ctrl Pts',(17.4004294239118,2.57056057432557,1.94635748428125));
#67347=CARTESIAN_POINT('Ctrl Pts',(17.4065799868617,2.5078444643747,2.02406366130248));
#67348=CARTESIAN_POINT('Ctrl Pts',(17.412736350793,2.44506920292928,2.10184312789014));
#67349=CARTESIAN_POINT('Ctrl Pts',(17.4188927147243,2.37870590385022,2.17665762742585));
#67350=CARTESIAN_POINT('Ctrl Pts',(17.4250490786555,2.30907687291099,2.24817293762904));
#67351=CARTESIAN_POINT('Ctrl Pts',(17.4312089072886,2.23940865588232,2.31972849548906));
#67352=CARTESIAN_POINT('Ctrl Pts',(17.4373687359217,2.16647136398159,2.38798087018275));
#67353=CARTESIAN_POINT('Ctrl Pts',(17.4435285645548,2.09062202041369,2.4526347323361));
#67354=CARTESIAN_POINT('Ctrl Pts',(17.4496967946728,2.01466922476066,2.51737677688546));
#67355=CARTESIAN_POINT('Ctrl Pts',(17.4558650247908,1.93579679350734,2.57851024843153));
#67356=CARTESIAN_POINT('Ctrl Pts',(17.4620332549088,1.85439222095044,2.6357820572609));
#67357=CARTESIAN_POINT('Ctrl Pts',(17.4636607226287,1.83291388574586,2.65089304020906));
#67358=CARTESIAN_POINT('Ctrl Pts',(17.4652881903487,1.81125941470005,2.66573543763448));
#67359=CARTESIAN_POINT('Ctrl Pts',(17.4669156580687,1.78943621037803,2.68030513402633));
#67360=CARTESIAN_POINT('Ctrl Pts',(16.2168686787502,1.78943621037802,2.68030513402634));
#67361=CARTESIAN_POINT('Ctrl Pts',(16.2230266939213,1.70630275993286,2.73580702619216));
#67362=CARTESIAN_POINT('Ctrl Pts',(16.2291847090924,1.62063435401742,2.78740441593627));
#67363=CARTESIAN_POINT('Ctrl Pts',(16.2353427242635,1.53283923964877,2.8348759104929));
#67364=CARTESIAN_POINT('Ctrl Pts',(16.2415045012076,1.44499049350348,2.88237640416426));
#67365=CARTESIAN_POINT('Ctrl Pts',(16.2476662781518,1.35501284322985,2.92574579597347));
#67366=CARTESIAN_POINT('Ctrl Pts',(16.2538280550959,1.26333585366192,2.96481029466512));
#67367=CARTESIAN_POINT('Ctrl Pts',(16.2599997290293,1.17151161335968,3.00393753839395));
#67368=CARTESIAN_POINT('Ctrl Pts',(16.2661714029626,1.07798299073099,3.03874593220572));
#67369=CARTESIAN_POINT('Ctrl Pts',(16.272343076896,0.983196062854421,3.06911111960574));
#67370=CARTESIAN_POINT('Ctrl Pts',(16.2756826143371,0.931906170033793,3.08554194231637));
#67371=CARTESIAN_POINT('Ctrl Pts',(16.2790221517781,0.880248060733309,3.10067268616429));
#67372=CARTESIAN_POINT('Ctrl Pts',(16.2823616892192,0.828293496285961,3.11448991754836));
#67373=CARTESIAN_POINT('Ctrl Pts',(16.288533937312,0.732269281262086,3.14002740037728));
#67374=CARTESIAN_POINT('Ctrl Pts',(16.2947061854047,0.634893910508744,3.1611648236009));
#67375=CARTESIAN_POINT('Ctrl Pts',(16.3008784334975,0.536607106782113,3.17776185002132));
#67376=CARTESIAN_POINT('Ctrl Pts',(16.3070423221501,0.438453418678726,3.19433639810862));
#67377=CARTESIAN_POINT('Ctrl Pts',(16.3132062108028,0.339391175663221,3.20638270016883));
#67378=CARTESIAN_POINT('Ctrl Pts',(16.3193700994554,0.23987406558232,3.21381051015162));
#67379=CARTESIAN_POINT('Ctrl Pts',(16.3255274611139,0.140462335015088,3.22123045476329));
#67380=CARTESIAN_POINT('Ctrl Pts',(16.3316848227725,0.0405971257550134,
3.22404159804077));
#67381=CARTESIAN_POINT('Ctrl Pts',(16.337842184431,-0.0592598587934908,
3.222205119423));
#67382=CARTESIAN_POINT('Ctrl Pts',(16.3439950485773,-0.159043904957785,
3.22036998222149));
#67383=CARTESIAN_POINT('Ctrl Pts',(16.3501479127236,-0.258819305362028,
3.21389398044223));
#67384=CARTESIAN_POINT('Ctrl Pts',(16.35630077687,-0.358122361369344,3.20279033606436));
#67385=CARTESIAN_POINT('Ctrl Pts',(16.3624513100065,-0.457387796459263,
3.19169089829709));
#67386=CARTESIAN_POINT('Ctrl Pts',(16.368601843143,-0.556180811514087,3.17596734970656));
#67387=CARTESIAN_POINT('Ctrl Pts',(16.3747523762796,-0.654041732521595,
3.15568486617725));
#67388=CARTESIAN_POINT('Ctrl Pts',(16.3809022244948,-0.751891755769422,
3.13540464129858));
#67389=CARTESIAN_POINT('Ctrl Pts',(16.38705207271,-0.848809465998504,3.11056657898061));
#67390=CARTESIAN_POINT('Ctrl Pts',(16.3932019209252,-0.944345297372316,
3.08128699115009));
#67391=CARTESIAN_POINT('Ctrl Pts',(16.3993527293043,-1.03989604457104,3.05200283195405));
#67392=CARTESIAN_POINT('Ctrl Pts',(16.4055035376835,-1.1340640690317,3.01827589717565));
#67393=CARTESIAN_POINT('Ctrl Pts',(16.4116543460626,-1.22641585355492,2.98027208768749));
#67394=CARTESIAN_POINT('Ctrl Pts',(16.4178117324288,-1.31886640376962,2.9422276349942));
#67395=CARTESIAN_POINT('Ctrl Pts',(16.423969118795,-1.4094964328398,2.89989733959456));
#67396=CARTESIAN_POINT('Ctrl Pts',(16.4301265051612,-1.49789339158082,2.8534948659422));
#67397=CARTESIAN_POINT('Ctrl Pts',(16.4362873278981,-1.58633968370895,2.80706649557091));
#67398=CARTESIAN_POINT('Ctrl Pts',(16.4424481506351,-1.67255004880547,2.7565616405934));
#67399=CARTESIAN_POINT('Ctrl Pts',(16.448608973372,-1.7561393138044,2.70223838197347));
#67400=CARTESIAN_POINT('Ctrl Pts',(16.4547800962887,-1.83986833034136,2.64782430117748));
#67401=CARTESIAN_POINT('Ctrl Pts',(16.4609512192054,-1.92096714054579,2.58957931854786));
#67402=CARTESIAN_POINT('Ctrl Pts',(16.4671223421221,-1.99908204816339,2.5278031029356));
#67403=CARTESIAN_POINT('Ctrl Pts',(16.4718178640677,-2.05851859933026,2.48079843619378));
#67404=CARTESIAN_POINT('Ctrl Pts',(16.4765133860133,-2.11622827998603,2.43175023148924));
#67405=CARTESIAN_POINT('Ctrl Pts',(16.4812089079588,-2.17206990711811,2.38080446091062));
#67406=CARTESIAN_POINT('Ctrl Pts',(16.4872889959218,-2.2443775246516,2.31483633850555));
#67407=CARTESIAN_POINT('Ctrl Pts',(16.4933690838848,-2.3138226346073,2.24543804555174));
#67408=CARTESIAN_POINT('Ctrl Pts',(16.4994491718478,-2.38005449792452,2.17289165615989));
#67409=CARTESIAN_POINT('Ctrl Pts',(16.5055793500724,-2.44683200653065,2.09974759982019));
#67410=CARTESIAN_POINT('Ctrl Pts',(16.5117095282969,-2.51034268704653,2.02340358087469));
#67411=CARTESIAN_POINT('Ctrl Pts',(16.5178397065214,-2.57026084270078,1.94419051612208));
#67412=CARTESIAN_POINT('Ctrl Pts',(16.5239044002319,-2.62953893355454,1.86582363052726));
#67413=CARTESIAN_POINT('Ctrl Pts',(16.5299690939424,-2.68530058600998,1.78464905108463));
#67414=CARTESIAN_POINT('Ctrl Pts',(16.5360337876529,-2.73726824252463,1.70102325997211));
#67415=CARTESIAN_POINT('Ctrl Pts',(16.5420946861043,-2.78920337790466,1.61744980151786));
#67416=CARTESIAN_POINT('Ctrl Pts',(16.5481555845558,-2.83734899587132,1.53142855711569));
#67417=CARTESIAN_POINT('Ctrl Pts',(16.5542164830072,-2.88147004464528,1.44334609304627));
#67418=CARTESIAN_POINT('Ctrl Pts',(16.5602753222,-2.92557610279544,1.35529355598717));
#67419=CARTESIAN_POINT('Ctrl Pts',(16.5663341613929,-2.96566010800427,1.26518159138569));
#67420=CARTESIAN_POINT('Ctrl Pts',(16.5723930005857,-3.00153287295572,1.17342148227573));
#67421=CARTESIAN_POINT('Ctrl Pts',(16.5785747046399,-3.03813308786114,1.07980060533149));
#67422=CARTESIAN_POINT('Ctrl Pts',(16.5847564086941,-3.07034918648835,0.984464442450112));
#67423=CARTESIAN_POINT('Ctrl Pts',(16.5909381127483,-3.09803229148831,0.887870195127457));
#67424=CARTESIAN_POINT('Ctrl Pts',(16.5970005632215,-3.12518135128422,0.793139383807464));
#67425=CARTESIAN_POINT('Ctrl Pts',(16.6030630136948,-3.14797068691146,0.697199052244218));
#67426=CARTESIAN_POINT('Ctrl Pts',(16.609125464168,-3.16631103188143,0.600493140581918));
#67427=CARTESIAN_POINT('Ctrl Pts',(16.6153667950127,-3.18519253223647,0.500933797048542));
#67428=CARTESIAN_POINT('Ctrl Pts',(16.6216081258573,-3.19935830376747,0.400563491805864));
#67429=CARTESIAN_POINT('Ctrl Pts',(16.627849456702,-3.20876825168828,0.299873088918141));
#67430=CARTESIAN_POINT('Ctrl Pts',(16.6340907875467,-3.2181781996091,0.199182686030418));
#67431=CARTESIAN_POINT('Ctrl Pts',(16.6403321183913,-3.22283235110456,0.0981727012668687));
#67432=CARTESIAN_POINT('Ctrl Pts',(16.646573449236,-3.2227488963424,-0.00266713776262558));
#67433=CARTESIAN_POINT('',(16.397001193014,-3.22274992098439,-0.00071364915948762));
#67434=CARTESIAN_POINT('Ctrl Pts',(15.9683010644095,1.78943598014216,2.68030528773732));
#67435=CARTESIAN_POINT('Ctrl Pts',(15.9744111699109,1.70131758392898,2.73913523872003));
#67436=CARTESIAN_POINT('Ctrl Pts',(15.9806437554029,1.61031895692001,2.79360584986089));
#67437=CARTESIAN_POINT('Ctrl Pts',(15.9881249457863,1.50100645402874,2.85191445822639));
#67438=CARTESIAN_POINT('Ctrl Pts',(15.9892077917178,1.48518103854343,2.86018770625233));
#67439=CARTESIAN_POINT('Ctrl Pts',(15.9908522949314,1.46114730347362,2.87249887356432));
#67440=CARTESIAN_POINT('Ctrl Pts',(15.991410523563,1.45298903337334,2.87663415944084));
#67441=CARTESIAN_POINT('Ctrl Pts',(15.9923834385129,1.43877101168713,2.88376511386765));
#67442=CARTESIAN_POINT('Ctrl Pts',(15.992797568485,1.43271920501153,2.8867765647031));
#67443=CARTESIAN_POINT('Ctrl Pts',(15.9936538956602,1.42020620145379,2.89295414398068));
#67444=CARTESIAN_POINT('Ctrl Pts',(15.9940961792845,1.41374379107446,2.89611771613011));
#67445=CARTESIAN_POINT('Ctrl Pts',(15.9951387239813,1.39851206812112,2.90351103827247));
#67446=CARTESIAN_POINT('Ctrl Pts',(15.9957396100857,1.38973411158864,2.90772272574307));
#67447=CARTESIAN_POINT('Ctrl Pts',(15.997012525266,1.37114198072267,2.91653986054752));
#67448=CARTESIAN_POINT('Ctrl Pts',(15.9976848798145,1.36132340055682,2.92113568393084));
#67449=CARTESIAN_POINT('Ctrl Pts',(15.9995033858335,1.33477332771783,2.93340015604154));
#67450=CARTESIAN_POINT('Ctrl Pts',(16.0006527480568,1.31799921591922,2.94097506891944));
#67451=CARTESIAN_POINT('Ctrl Pts',(16.0098667153589,1.18359436543072,3.00028929492527));
#67452=CARTESIAN_POINT('Ctrl Pts',(16.018165684055,1.06304416223038,3.04508806783611));
#67453=CARTESIAN_POINT('Ctrl Pts',(16.0445596502099,0.680859249907262,3.16165087517386));
#67454=CARTESIAN_POINT('Ctrl Pts',(16.0632944570895,0.412653181284849,3.2076944093041));
#67455=CARTESIAN_POINT('Ctrl Pts',(16.0820290354376,0.128649797679572,3.2202083437708));
#67456=CARTESIAN_POINT('Ctrl Pts',(16.0828982768621,0.115430785474178,3.22070928379955));
#67457=CARTESIAN_POINT('Ctrl Pts',(16.0877893049261,0.0407935520529635,
3.22307758054531));
#67458=CARTESIAN_POINT('Ctrl Pts',(16.0917526929636,-0.0206699549010299,
3.22326963576358));
#67459=CARTESIAN_POINT('Ctrl Pts',(16.0962603126204,-0.092171009264649,
3.22144741371853));
#67460=CARTESIAN_POINT('Ctrl Pts',(16.0968923923274,-0.10223499888431,3.22114373253747));
#67461=CARTESIAN_POINT('Ctrl Pts',(16.0978416425163,-0.117408838105377,
3.22061467490167));
#67462=CARTESIAN_POINT('Ctrl Pts',(16.0981607281436,-0.122519730306948,
3.22042429440686));
#67463=CARTESIAN_POINT('Ctrl Pts',(16.0987296716682,-0.131651506416395,
3.22006236581669));
#67464=CARTESIAN_POINT('Ctrl Pts',(16.0989797874212,-0.135672528732226,
3.21989545241152));
#67465=CARTESIAN_POINT('Ctrl Pts',(16.0995160115931,-0.144307409481603,
3.21952081281911));
#67466=CARTESIAN_POINT('Ctrl Pts',(16.0998019837475,-0.148921120330165,
3.21931070155764));
#67467=CARTESIAN_POINT('Ctrl Pts',(16.1005856181057,-0.161587044799179,
3.21870660080785));
#67468=CARTESIAN_POINT('Ctrl Pts',(16.1010821495033,-0.169638323574166,
3.21829231077317));
#67469=CARTESIAN_POINT('Ctrl Pts',(16.1037011887418,-0.212236766076815,
3.21594004452639));
#67470=CARTESIAN_POINT('Ctrl Pts',(16.1057953492502,-0.246754167624729,
3.21347591017222));
#67471=CARTESIAN_POINT('Ctrl Pts',(16.1118446440377,-0.347528374177671,
3.20464837686346));
#67472=CARTESIAN_POINT('Ctrl Pts',(16.1157313326968,-0.413638642460783,
3.19678767576636));
#67473=CARTESIAN_POINT('Ctrl Pts',(16.1249567225218,-0.572218270836931,
3.17292960036643));
#67474=CARTESIAN_POINT('Ctrl Pts',(16.1302349329642,-0.664325252683203,
3.15493098941956));
#67475=CARTESIAN_POINT('Ctrl Pts',(16.1426761042349,-0.880317490871748,
3.10284368921993));
#67476=CARTESIAN_POINT('Ctrl Pts',(16.1498085647131,-1.00320497091956,3.06531840584928));
#67477=CARTESIAN_POINT('Ctrl Pts',(16.1664215780302,-1.27833215820242,2.96298256846807));
#67478=CARTESIAN_POINT('Ctrl Pts',(16.1759724715495,-1.42846375938282,2.89359274938661));
#67479=CARTESIAN_POINT('Ctrl Pts',(16.1871324931095,-1.58975921206449,2.80342102454104));
#67480=CARTESIAN_POINT('Ctrl Pts',(16.1883248621219,-1.60682493959801,2.7936745301117));
#67481=CARTESIAN_POINT('Ctrl Pts',(16.1900881480807,-1.63181014318447,2.77910043163032));
#67482=CARTESIAN_POINT('Ctrl Pts',(16.1906546814246,-1.63979984697515,2.77439362951903));
#67483=CARTESIAN_POINT('Ctrl Pts',(16.1916566786765,-1.65386339416463,2.76602670321143));
#67484=CARTESIAN_POINT('Ctrl Pts',(16.1920916183248,-1.659945705292,2.76238087591891));
#67485=CARTESIAN_POINT('Ctrl Pts',(16.1929999880696,-1.67260185712784,2.75473769787025));
#67486=CARTESIAN_POINT('Ctrl Pts',(16.1934735455634,-1.67917350871398,2.75073682538486));
#67487=CARTESIAN_POINT('Ctrl Pts',(16.1944407235126,-1.69254124746841,2.74253268750756));
#67488=CARTESIAN_POINT('Ctrl Pts',(16.1949344088852,-1.69933615025632,2.73832760330379));
#67489=CARTESIAN_POINT('Ctrl Pts',(16.1961445497975,-1.71592198604141,2.72797780782076));
#67490=CARTESIAN_POINT('Ctrl Pts',(16.1968620200333,-1.72569557740239,2.72180564160397));
#67491=CARTESIAN_POINT('Ctrl Pts',(16.1988370017323,-1.75243412638133,2.70471794303886));
#67492=CARTESIAN_POINT('Ctrl Pts',(16.2000984769707,-1.76932990841859,2.69369563314341));
#67493=CARTESIAN_POINT('Ctrl Pts',(16.2109888188054,-1.91360957536704,2.59762875079558));
#67494=CARTESIAN_POINT('Ctrl Pts',(16.2209531248965,-2.03486617573846,2.50377403991726));
#67495=CARTESIAN_POINT('Ctrl Pts',(16.2424460007868,-2.27532453105108,2.28861532452761));
#67496=CARTESIAN_POINT('Ctrl Pts',(16.25399747391,-2.39254884207164,2.1657716825991));
#67497=CARTESIAN_POINT('Ctrl Pts',(16.2751706692155,-2.59094393291775,1.9220006607759));
#67498=CARTESIAN_POINT('Ctrl Pts',(16.2847988289659,-2.67467119925028,1.80366893425787));
#67499=CARTESIAN_POINT('Ctrl Pts',(16.2947029690045,-2.75642449651405,1.66984602855923));
#67500=CARTESIAN_POINT('Ctrl Pts',(16.2954579452262,-2.76262754158888,1.65956344899287));
#67501=CARTESIAN_POINT('Ctrl Pts',(16.2965448542827,-2.77151808681189,1.64463790205908));
#67502=CARTESIAN_POINT('Ctrl Pts',(16.296879712477,-2.77425160688929,1.64002266968465));
#67503=CARTESIAN_POINT('Ctrl Pts',(16.2974671813133,-2.77903778234854,1.63189555819161));
#67504=CARTESIAN_POINT('Ctrl Pts',(16.297720110279,-2.78109532785786,1.62838659005661));
#67505=CARTESIAN_POINT('Ctrl Pts',(16.2982476052231,-2.78538004415174,1.62104756289266));
#67506=CARTESIAN_POINT('Ctrl Pts',(16.2985220893806,-2.78760595761773,1.61721681203778));
#67507=CARTESIAN_POINT('Ctrl Pts',(16.2992424369652,-2.7934376760502,1.60713273187644));
#67508=CARTESIAN_POINT('Ctrl Pts',(16.2996874564643,-2.79703040851733,1.60087181374437));
#67509=CARTESIAN_POINT('Ctrl Pts',(16.301668906611,-2.8129802530347,1.57285901948052));
#67510=CARTESIAN_POINT('Ctrl Pts',(16.3031908843387,-2.82510528331116,1.55097505698315));
#67511=CARTESIAN_POINT('Ctrl Pts',(16.3160153682931,-2.92603551018716,1.36369866004603));
#67512=CARTESIAN_POINT('Ctrl Pts',(16.3265401636377,-3.00050002832363,1.19095625801945));
#67513=CARTESIAN_POINT('Ctrl Pts',(16.3514993649324,-3.14077162809572,0.7671733290003));
#67514=CARTESIAN_POINT('Ctrl Pts',(16.3658858189897,-3.19218097387089,0.512799416071989));
#67515=CARTESIAN_POINT('Ctrl Pts',(16.3833188965377,-3.21522846088223,0.222464671532063));
#67516=CARTESIAN_POINT('Ctrl Pts',(16.3852888400579,-3.21731807968137,0.189865322853617));
#67517=CARTESIAN_POINT('Ctrl Pts',(16.3879966107665,-3.21949151182315,0.14537248388479));
#67518=CARTESIAN_POINT('Ctrl Pts',(16.3887209270774,-3.22000561539516,0.133501253434329));
#67519=CARTESIAN_POINT('Ctrl Pts',(16.3898721200999,-3.22071631611739,0.114683324781635));
#67520=CARTESIAN_POINT('Ctrl Pts',(16.3902976382364,-3.22095611797239,0.107738288395413));
#67521=CARTESIAN_POINT('Ctrl Pts',(16.3911517513287,-3.22139163868266,0.0938197257307931));
#67522=CARTESIAN_POINT('Ctrl Pts',(16.3915803494882,-3.22158718048736,0.0868462319927856));
#67523=CARTESIAN_POINT('Ctrl Pts',(16.3924407430093,-3.22193368692295,0.0728693967865503));
#67524=CARTESIAN_POINT('Ctrl Pts',(16.3928725419104,-3.22208446335216,0.065866089161238));
#67525=CARTESIAN_POINT('Ctrl Pts',(16.3939263155754,-3.22239617563137,0.04880250781653));
#67526=CARTESIAN_POINT('Ctrl Pts',(16.394549049548,-3.22253283271506,0.0387419136726294));
#67527=CARTESIAN_POINT('Ctrl Pts',(16.3957811749886,-3.22270957562087,0.0188828806645124));
#67528=CARTESIAN_POINT('Ctrl Pts',(16.3963904821978,-3.22275209071569,0.00908458474906739));
#67529=CARTESIAN_POINT('Ctrl Pts',(16.397001193014,-3.22274992098439,-0.00071364915948762));
#67530=CARTESIAN_POINT('Ctrl Pts',(16.3970011089261,-3.22274992128285,-0.000712300053586545));
#67531=CARTESIAN_POINT('Ctrl Pts',(16.4000499952323,-3.222739109685,-0.0496285902397631));
#67532=CARTESIAN_POINT('Ctrl Pts',(16.4031335870394,-3.22161459570378,-0.0985365305315511));
#67533=CARTESIAN_POINT('Ctrl Pts',(16.4185052177376,-3.21058390395279,-0.339461510791843));
#67534=CARTESIAN_POINT('Ctrl Pts',(16.4312857109541,-3.18462237739346,-0.53032325674288));
#67535=CARTESIAN_POINT('Ctrl Pts',(16.4561576032861,-3.10259562993228,-0.889401700762396));
#67536=CARTESIAN_POINT('Ctrl Pts',(16.4681680705531,-3.049364880723,-1.0575979878311));
#67537=CARTESIAN_POINT('Ctrl Pts',(16.4828813413233,-2.96463328870021,-1.26464671447841));
#67538=CARTESIAN_POINT('Ctrl Pts',(16.4859767176357,-2.94563659456967,-1.3082841445284));
#67539=CARTESIAN_POINT('Ctrl Pts',(16.4907729904448,-2.91423179777867,-1.37626878528022));
#67540=CARTESIAN_POINT('Ctrl Pts',(16.4925055193836,-2.90246931044543,-1.40090497920624));
#67541=CARTESIAN_POINT('Ctrl Pts',(16.4946871106681,-2.88710181709131,-1.43206706930084));
#67542=CARTESIAN_POINT('Ctrl Pts',(16.4951532041314,-2.88378572056338,-1.43873309328605));
#67543=CARTESIAN_POINT('Ctrl Pts',(16.4958975389548,-2.87843672747348,-1.44939285543799));
#67544=CARTESIAN_POINT('Ctrl Pts',(16.4961766908395,-2.87641857442559,-1.45339390006555));
#67545=CARTESIAN_POINT('Ctrl Pts',(16.4967072451973,-2.87255968088809,-1.461004743599));
#67546=CARTESIAN_POINT('Ctrl Pts',(16.4969587370425,-2.87072049997563,-1.46461523693213));
#67547=CARTESIAN_POINT('Ctrl Pts',(16.4975357192614,-2.86647807306831,-1.4729048469192));
#67548=CARTESIAN_POINT('Ctrl Pts',(16.4978609126101,-2.86407017960254,-1.47758155061002));
#67549=CARTESIAN_POINT('Ctrl Pts',(16.4988915053716,-2.85638611900982,-1.49241647257229));
#67550=CARTESIAN_POINT('Ctrl Pts',(16.4995942536309,-2.85106720501054,-1.50255262475929));
#67551=CARTESIAN_POINT('Ctrl Pts',(16.506352429903,-2.79916285360483,-1.60019775203507));
#67552=CARTESIAN_POINT('Ctrl Pts',(16.5121696974556,-2.74861177364789,-1.68555128366764));
#67553=CARTESIAN_POINT('Ctrl Pts',(16.5262668709858,-2.61392722851102,-1.89074104311305));
#67554=CARTESIAN_POINT('Ctrl Pts',(16.5343913260252,-2.52541670116867,-2.00743420474199));
#67555=CARTESIAN_POINT('Ctrl Pts',(16.5559208039694,-2.2724097377441,-2.29766441150014));
#67556=CARTESIAN_POINT('Ctrl Pts',(16.5694050719756,-2.09605762214324,-2.45959907477577));
#67557=CARTESIAN_POINT('Ctrl Pts',(16.5846280695142,-1.8927551213189,-2.60840401901072));
#67558=CARTESIAN_POINT('Ctrl Pts',(16.5854319686233,-1.8820043438503,-2.61617146175146));
#67559=CARTESIAN_POINT('Ctrl Pts',(16.5867674645548,-1.86412210903003,-2.62892412003284));
#67560=CARTESIAN_POINT('Ctrl Pts',(16.58729760397,-1.85701779562866,-2.63394726041709));
#67561=CARTESIAN_POINT('Ctrl Pts',(16.5883294362001,-1.84317982421048,-2.64364765356918));
#67562=CARTESIAN_POINT('Ctrl Pts',(16.588831001631,-1.83644848195097,-2.64832810500794));
#67563=CARTESIAN_POINT('Ctrl Pts',(16.5893362927831,-1.82966255946109,-2.65300819505124));
#67564=CARTESIAN_POINT('Ctrl Pts',(16.589339036157,-1.82962571656205,-2.65303360359336));
#67565=CARTESIAN_POINT('Ctrl Pts',(16.5893440699943,-1.82955811300148,-2.65308022401251));
#67566=CARTESIAN_POINT('Ctrl Pts',(16.5893463611346,-1.82952734329172,-2.65310144247141));
#67567=CARTESIAN_POINT('Ctrl Pts',(16.589351015401,-1.82946483691802,-2.65314454458581));
#67568=CARTESIAN_POINT('Ctrl Pts',(16.5893533784737,-1.82943310096691,-2.65316642769948));
#67569=CARTESIAN_POINT('Ctrl Pts',(16.5893581796194,-1.82936862161112,-2.65321088689635));
#67570=CARTESIAN_POINT('Ctrl Pts',(16.5893606176394,-1.82933587890988,-2.65323346244046));
#67571=CARTESIAN_POINT('Ctrl Pts',(16.5893655718598,-1.82926934332688,-2.65327933579337));
#67572=CARTESIAN_POINT('Ctrl Pts',(16.5893680880116,-1.82923555108999,-2.65330263309941));
#67573=CARTESIAN_POINT('Ctrl Pts',(16.5893732018518,-1.82916687133701,-2.65334998089165));
#67574=CARTESIAN_POINT('Ctrl Pts',(16.5893757994974,-1.82913198438932,-2.65337403092339));
#67575=CARTESIAN_POINT('Ctrl Pts',(16.5893810799027,-1.82906106714463,-2.65342291711476));
#67576=CARTESIAN_POINT('Ctrl Pts',(16.5893837626122,-1.82902503751554,-2.6534477527465));
#67577=CARTESIAN_POINT('Ctrl Pts',(16.589389216898,-1.82895178448462,-2.6534982446901));
#67578=CARTESIAN_POINT('Ctrl Pts',(16.5893919884389,-1.82891456155067,-2.6535239006067));
#67579=CARTESIAN_POINT('Ctrl Pts',(16.5893976243923,-1.82883886809789,-2.65357606998867));
#67580=CARTESIAN_POINT('Ctrl Pts',(16.5894004887657,-1.82880039809474,-2.65360258302006));
#67581=CARTESIAN_POINT('Ctrl Pts',(16.5894063146363,-1.82872215336613,-2.65365650577095));
#67582=CARTESIAN_POINT('Ctrl Pts',(16.5894092760919,-1.82868237919014,-2.65368391502683));
#67583=CARTESIAN_POINT('Ctrl Pts',(16.5894153006245,-1.82860146567853,-2.65373967161695));
#67584=CARTESIAN_POINT('Ctrl Pts',(16.5894183636691,-1.82856032676909,-2.65376801856559));
#67585=CARTESIAN_POINT('Ctrl Pts',(16.5894245961762,-1.82847661933577,-2.6538256946744));
#67586=CARTESIAN_POINT('Ctrl Pts',(16.5894277656057,-1.82843405124559,-2.65385502343617));
#67587=CARTESIAN_POINT('Ctrl Pts',(16.5894342159882,-1.8283474168431,-2.65391471013784));
#67588=CARTESIAN_POINT('Ctrl Pts',(16.5894374969081,-1.82830335096306,-2.65394506767194));
#67589=CARTESIAN_POINT('Ctrl Pts',(16.5894441757122,-1.8282136478684,-2.65400686195763));
#67590=CARTESIAN_POINT('Ctrl Pts',(16.5894475735653,-1.82816801105835,-2.65403829831325));
#67591=CARTESIAN_POINT('Ctrl Pts',(16.589454492026,-1.82807508829159,-2.65410230348491));
#67592=CARTESIAN_POINT('Ctrl Pts',(16.5894580126124,-1.82802780260412,-2.65413487198798));
#67593=CARTESIAN_POINT('Ctrl Pts',(16.5894651827376,-1.82793149879386,-2.65420119843224));
#67594=CARTESIAN_POINT('Ctrl Pts',(16.5894688322551,-1.82788248094004,-2.65423495604939));
#67595=CARTESIAN_POINT('Ctrl Pts',(16.5894762668778,-1.82778262362344,-2.65430372171122));
#67596=CARTESIAN_POINT('Ctrl Pts',(16.589480051958,-1.82773178447891,-2.65433872938543));
#67597=CARTESIAN_POINT('Ctrl Pts',(16.5894877648009,-1.82762818923377,-2.65441006035623));
#67598=CARTESIAN_POINT('Ctrl Pts',(16.5894916925427,-1.82757543339558,-2.65444638330694));
#67599=CARTESIAN_POINT('Ctrl Pts',(16.5894996983117,-1.82746790258163,-2.65452041468055));
#67600=CARTESIAN_POINT('Ctrl Pts',(16.5895037763236,-1.82741312779065,-2.65455812279566));
#67601=CARTESIAN_POINT('Ctrl Pts',(16.5895120908056,-1.82730144923561,-2.65463499956085));
#67602=CARTESIAN_POINT('Ctrl Pts',(16.5895163272605,-1.8272445456507,-2.65467416788987));
#67603=CARTESIAN_POINT('Ctrl Pts',(16.5895249674066,-1.82712849152999,-2.6547540456877));
#67604=CARTESIAN_POINT('Ctrl Pts',(16.5895293710878,-1.82706934110019,-2.65479475486668));
#67605=CARTESIAN_POINT('Ctrl Pts',(16.5895383551484,-1.82694866611953,-2.65487780122581));
#67606=CARTESIAN_POINT('Ctrl Pts',(16.5895429355172,-1.82688714168104,-2.65492013809043));
#67607=CARTESIAN_POINT('Ctrl Pts',(16.5895522831516,-1.82676158160453,-2.65500653342234));
#67608=CARTESIAN_POINT('Ctrl Pts',(16.5895570504099,-1.82669754603437,-2.65505059158082));
#67609=CARTESIAN_POINT('Ctrl Pts',(16.5895667828414,-1.82656681559989,-2.6551405305939));
#67610=CARTESIAN_POINT('Ctrl Pts',(16.5895717480099,-1.82650012076539,-2.655186411139));
#67611=CARTESIAN_POINT('Ctrl Pts',(16.5895818881815,-1.82636391158558,-2.65528010425945));
#67612=CARTESIAN_POINT('Ctrl Pts',(16.5895870631839,-1.82629439721301,-2.65532791653434));
#67613=CARTESIAN_POINT('Ctrl Pts',(16.5895976359233,-1.82615237556289,-2.65542559140141));
#67614=CARTESIAN_POINT('Ctrl Pts',(16.5896030336617,-1.82607986822302,-2.65547545368331));
#67615=CARTESIAN_POINT('Ctrl Pts',(16.5896138302346,-1.82593483778435,-2.65557518033504));
#67616=CARTESIAN_POINT('Ctrl Pts',(16.5896192289933,-1.82586231570136,-2.65562504400514));
#67617=CARTESIAN_POINT('Ctrl Pts',(16.5900599168791,-1.81994246762946,-2.65969496919288));
#67618=CARTESIAN_POINT('Ctrl Pts',(16.5904959396648,-1.81408191918375,-2.66369568529113));
#67619=CARTESIAN_POINT('Ctrl Pts',(16.591504967565,-1.80051223134995,-2.67289350852866));
#67620=CARTESIAN_POINT('Ctrl Pts',(16.5920784966523,-1.79279374769735,-2.67807665657474));
#67621=CARTESIAN_POINT('Ctrl Pts',(16.5938094626318,-1.76948300733419,-2.69358444559813));
#67622=CARTESIAN_POINT('Ctrl Pts',(16.5949707319381,-1.75382341528902,-2.70380670223369));
#67623=CARTESIAN_POINT('Ctrl Pts',(16.6123839859193,-1.51872855643692,-2.85437007948953));
#67624=CARTESIAN_POINT('Ctrl Pts',(16.6296819605777,-1.2832067758928,-2.96770774649493));
#67625=CARTESIAN_POINT('Ctrl Pts',(16.6572047251047,-0.897963175961086,
-3.09858713093773));
#67626=CARTESIAN_POINT('Ctrl Pts',(16.6671559738335,-0.756191328804278,
-3.13620125858548));
#67627=CARTESIAN_POINT('Ctrl Pts',(16.6803723668195,-0.559670177165497,
-3.17423465839397));
#67628=CARTESIAN_POINT('Ctrl Pts',(16.6838747666673,-0.506743431103136,
-3.18311296651785));
#67629=CARTESIAN_POINT('Ctrl Pts',(16.6885824578689,-0.43410785577902,-3.19343955929563));
#67630=CARTESIAN_POINT('Ctrl Pts',(16.6898387962672,-0.41457346000359,-3.19603422049542));
#67631=CARTESIAN_POINT('Ctrl Pts',(16.6919739475725,-0.381094225339752,
-3.20016898380726));
#67632=CARTESIAN_POINT('Ctrl Pts',(16.692857204112,-0.36716110907499,-3.20179747491863));
#67633=CARTESIAN_POINT('Ctrl Pts',(16.6940971675271,-0.347475687395216,
-3.20396809886131));
#67634=CARTESIAN_POINT('Ctrl Pts',(16.6944579947098,-0.341732121548773,
-3.20458579073638));
#67635=CARTESIAN_POINT('Ctrl Pts',(16.695074822161,-0.331887015517989,-3.20561781330294));
#67636=CARTESIAN_POINT('Ctrl Pts',(16.6953312488285,-0.327786298622197,
-3.20603972202199));
#67637=CARTESIAN_POINT('Ctrl Pts',(16.6958228403389,-0.319909419738118,
-3.20683487631056));
#67638=CARTESIAN_POINT('Ctrl Pts',(16.6960580739086,-0.316133409862919,
-3.20720932093361));
#67639=CARTESIAN_POINT('Ctrl Pts',(16.6966160841305,-0.307160224968528,
-3.20808313769721));
#67640=CARTESIAN_POINT('Ctrl Pts',(16.6969385249232,-0.301962460593134,
-3.20857655284675));
#67641=CARTESIAN_POINT('Ctrl Pts',(16.6979044748694,-0.286354080106295,
-3.2100199665271));
#67642=CARTESIAN_POINT('Ctrl Pts',(16.6985458919845,-0.275939895179967,
-3.21093195597616));
#67643=CARTESIAN_POINT('Ctrl Pts',(16.7113012782673,-0.0678953651523029,
-3.22813114898002));
#67644=CARTESIAN_POINT('Ctrl Pts',(16.7224514374401,0.130850733931946,-3.22619652195971));
#67645=CARTESIAN_POINT('Ctrl Pts',(16.7426345563512,0.489757196123863,-3.18945684997258));
#67646=CARTESIAN_POINT('Ctrl Pts',(16.7516572405222,0.649845765068287,-3.16072692886614));
#67647=CARTESIAN_POINT('Ctrl Pts',(16.7674877532071,0.917119915435433,-3.09158984444052));
#67648=CARTESIAN_POINT('Ctrl Pts',(16.774132776632,1.02556697036692,-3.05732644301238));
#67649=CARTESIAN_POINT('Ctrl Pts',(16.782007587846,1.14813590376406,-3.0113451500305));
#67650=CARTESIAN_POINT('Ctrl Pts',(16.7830503796093,1.16425224123502,-3.00515097244806));
#67651=CARTESIAN_POINT('Ctrl Pts',(16.7847265393173,1.18996952152383,-2.99502882916147));
#67652=CARTESIAN_POINT('Ctrl Pts',(16.7853571466778,1.19960276526942,-2.99118343658588));
#67653=CARTESIAN_POINT('Ctrl Pts',(16.7865622845142,1.21793122413258,-2.98376431244321));
#67654=CARTESIAN_POINT('Ctrl Pts',(16.7871365299466,1.22662970818898,-2.98019890191331));
#67655=CARTESIAN_POINT('Ctrl Pts',(16.7881491865587,1.24190691290999,-2.97385873231898));
#67656=CARTESIAN_POINT('Ctrl Pts',(16.7885870486961,1.24849227439157,-2.97110006220009));
#67657=CARTESIAN_POINT('Ctrl Pts',(16.7894464887863,1.26137794841352,-2.96565172631269));
#67658=CARTESIAN_POINT('Ctrl Pts',(16.789868005233,1.2676789628405,-2.96296380952248));
#67659=CARTESIAN_POINT('Ctrl Pts',(16.7909912595639,1.2844194801497,-2.95575938527642));
#67660=CARTESIAN_POINT('Ctrl Pts',(16.7916941982392,1.29484365182372,-2.95120769459627));
#67661=CARTESIAN_POINT('Ctrl Pts',(16.7942180094451,1.3320820077969,-2.93471237707476));
#67662=CARTESIAN_POINT('Ctrl Pts',(16.7960495278954,1.35875618585592,-2.9224579974887));
#67663=CARTESIAN_POINT('Ctrl Pts',(16.7981705747803,1.38923904778023,-2.90794633130796));
#67664=CARTESIAN_POINT('Ctrl Pts',(16.7984478243401,1.39321562963116,-2.90604322175106));
#67665=CARTESIAN_POINT('Ctrl Pts',(16.8161358892818,1.64640819996547,-2.78423137039711));
#67666=CARTESIAN_POINT('Ctrl Pts',(16.8347287356816,1.87911001732313,-2.63277178333459));
#67667=CARTESIAN_POINT('Ctrl Pts',(16.8614757591024,2.18003477909586,-2.37648569884837));
#67668=CARTESIAN_POINT('Ctrl Pts',(16.8694943973193,2.26617002311396,-2.2944961337676));
#67669=CARTESIAN_POINT('Ctrl Pts',(16.8804727589352,2.38049713103802,-2.17293784162986));
#67670=CARTESIAN_POINT('Ctrl Pts',(16.88359864053,2.41262537835953,-2.1372095714432));
#67671=CARTESIAN_POINT('Ctrl Pts',(16.8884369192417,2.46186179003618,-2.07993019144936));
#67672=CARTESIAN_POINT('Ctrl Pts',(16.8901815919505,2.4795124529342,-2.05885676796523));
#67673=CARTESIAN_POINT('Ctrl Pts',(16.8923762140806,2.50161051591836,-2.03177707613838));
#67674=CARTESIAN_POINT('Ctrl Pts',(16.8928434394751,2.50630896560232,-2.02597843819934));
#67675=CARTESIAN_POINT('Ctrl Pts',(16.8935891534087,2.51379879986591,-2.01666885561076));
#67676=CARTESIAN_POINT('Ctrl Pts',(16.8938685583511,2.51660303700085,-2.0131683571283));
#67677=CARTESIAN_POINT('Ctrl Pts',(16.894399299443,2.52192605618841,-2.00649518796544));
#67678=CARTESIAN_POINT('Ctrl Pts',(16.8946507261324,2.52444613381322,-2.00332366077946));
#67679=CARTESIAN_POINT('Ctrl Pts',(16.8952271715592,2.53022011442161,-1.99602888840464));
#67680=CARTESIAN_POINT('Ctrl Pts',(16.8955518951387,2.53346991844349,-1.99190243838388));
#67681=CARTESIAN_POINT('Ctrl Pts',(16.8964161244271,2.5421110088815,-1.98087502614272));
#67682=CARTESIAN_POINT('Ctrl Pts',(16.8969543704657,2.54748432576062,-1.97395994508968));
#67683=CARTESIAN_POINT('Ctrl Pts',(16.9006970477109,2.58478198210128,-1.92555453338215));
#67684=CARTESIAN_POINT('Ctrl Pts',(16.9038355291246,2.61572151822829,-1.88331087098912));
#67685=CARTESIAN_POINT('Ctrl Pts',(16.9206036247207,2.77805219641848,-1.64994758631482));
#67686=CARTESIAN_POINT('Ctrl Pts',(16.9332885187166,2.88956170917061,-1.44580705464937));
#67687=CARTESIAN_POINT('Ctrl Pts',(16.9575267891894,3.05449517460461,-1.04692249901461));
#67688=CARTESIAN_POINT('Ctrl Pts',(16.9689398215512,3.11346845739485,-0.855736560816484));
#67689=CARTESIAN_POINT('Ctrl Pts',(16.9822474294151,3.15865912079881,-0.6398653513746));
#67690=CARTESIAN_POINT('Ctrl Pts',(16.9835157488638,3.16274561271978,-0.619350681485886));
#67691=CARTESIAN_POINT('Ctrl Pts',(16.985376381522,3.16841850936224,-0.589350623475699));
#67692=CARTESIAN_POINT('Ctrl Pts',(16.9859636565608,3.17016267878636,-0.579895330844444));
#67693=CARTESIAN_POINT('Ctrl Pts',(16.9869976991082,3.17315227420335,-0.563271817436396));
#67694=CARTESIAN_POINT('Ctrl Pts',(16.9874438865121,3.17441579262071,-0.556106887011703));
#67695=CARTESIAN_POINT('Ctrl Pts',(16.9883128596609,3.17682508852709,-0.542168891009394));
#67696=CARTESIAN_POINT('Ctrl Pts',(16.9887355590261,3.17797349491455,-0.535396314824354));
#67697=CARTESIAN_POINT('Ctrl Pts',(16.9897487539236,3.18066983177097,-0.519180654185753));
#67698=CARTESIAN_POINT('Ctrl Pts',(16.9903398949484,3.18219736723143,-0.509734286893273));
#67699=CARTESIAN_POINT('Ctrl Pts',(16.9924778336904,3.18755743055467,-0.475623997131077));
#67700=CARTESIAN_POINT('Ctrl Pts',(16.9940323649592,3.19114539014042,-0.450923055724328));
#67701=CARTESIAN_POINT('Ctrl Pts',(16.9963249230625,3.19598463621889,-0.414650626003227));
#67702=CARTESIAN_POINT('Ctrl Pts',(16.9970558038624,3.19746079580874,-0.403109650266346));
#67703=CARTESIAN_POINT('Ctrl Pts',(17.0139876568164,3.23012185742507,-0.136283741417817));
#67704=CARTESIAN_POINT('Ctrl Pts',(17.0311949611847,3.23069377974112,0.121767434515482));
#67705=CARTESIAN_POINT('Ctrl Pts',(17.061322455295,3.17861375631521,0.563810703728457));
#67706=CARTESIAN_POINT('Ctrl Pts',(17.0740619293645,3.14031391012763,0.748271657561799));
#67707=CARTESIAN_POINT('Ctrl Pts',(17.0876849085203,3.07893068489434,0.952328818867472));
#67708=CARTESIAN_POINT('Ctrl Pts',(17.0892719388212,3.07143948521891,0.976219197871528));
#67709=CARTESIAN_POINT('Ctrl Pts',(17.0912966405999,3.06142989123675,1.00688465927331));
#67710=CARTESIAN_POINT('Ctrl Pts',(17.0917485395012,3.05916632499223,1.01374113779552));
#67711=CARTESIAN_POINT('Ctrl Pts',(17.0924755768789,3.05547651792626,1.02479287848273));
#67712=CARTESIAN_POINT('Ctrl Pts',(17.0927515534256,3.05406465063036,1.02899285989948));
#67713=CARTESIAN_POINT('Ctrl Pts',(17.0932798781394,3.05134008239275,1.03704281937484));
#67714=CARTESIAN_POINT('Ctrl Pts',(17.0935323031022,3.05002875780627,1.0408932146617));
#67715=CARTESIAN_POINT('Ctrl Pts',(17.0941165369165,3.04697158040114,1.04981451335244));
#67716=CARTESIAN_POINT('Ctrl Pts',(17.0944480259587,3.04522034503873,1.05488358379804));
#67717=CARTESIAN_POINT('Ctrl Pts',(17.0955190451632,3.03950865609358,1.07128370115698));
#67718=CARTESIAN_POINT('Ctrl Pts',(17.0962556210477,3.03549749315963,1.08259716349494));
#67719=CARTESIAN_POINT('Ctrl Pts',(17.1057476315043,2.98274381406795,1.22879010151195));
#67720=CARTESIAN_POINT('Ctrl Pts',(17.1140021921056,2.92510673743358,1.36031157830405));
#67721=CARTESIAN_POINT('Ctrl Pts',(17.1243731128257,2.8403807253697,1.52314243035026));
#67722=CARTESIAN_POINT('Ctrl Pts',(17.1266258691787,2.82120889966688,1.55836643903213));
#67723=CARTESIAN_POINT('Ctrl Pts',(17.1408324359696,2.69586295771963,1.77876369311601));
#67724=CARTESIAN_POINT('Ctrl Pts',(17.1526309064463,2.57217792746988,1.95334893858489));
#67725=CARTESIAN_POINT('Ctrl Pts',(17.1703307977481,2.37244900266836,2.18309005397934));
#67726=CARTESIAN_POINT('Ctrl Pts',(17.1757172272911,2.30987577937546,2.24919274636321));
#67727=CARTESIAN_POINT('Ctrl Pts',(17.1822011779251,2.23304559841401,2.32376503428086));
#67728=CARTESIAN_POINT('Ctrl Pts',(17.1831795005784,2.22141335862531,2.33488741798036));
#67729=CARTESIAN_POINT('Ctrl Pts',(17.1846893319437,2.20340342271436,2.35185154839321));
#67730=CARTESIAN_POINT('Ctrl Pts',(17.185218148771,2.19708459330411,2.35775563544508));
#67731=CARTESIAN_POINT('Ctrl Pts',(17.1861836763199,2.18552823061081,2.36846668830334));
#67732=CARTESIAN_POINT('Ctrl Pts',(17.1866200299798,2.1802983940587,2.37328190739672));
#67733=CARTESIAN_POINT('Ctrl Pts',(17.1875726947395,2.16886517728149,2.38373902053944));
#67734=CARTESIAN_POINT('Ctrl Pts',(17.1880892917213,2.16265563699862,2.3893740747106));
#67735=CARTESIAN_POINT('Ctrl Pts',(17.1895012111658,2.14565839384658,2.40467824992613));
#67736=CARTESIAN_POINT('Ctrl Pts',(17.1903985651119,2.1348274720379,2.41429888008091));
#67737=CARTESIAN_POINT('Ctrl Pts',(17.1948030728425,2.08153279899714,2.46099915322595));
#67738=CARTESIAN_POINT('Ctrl Pts',(17.1983532666532,2.03816818752887,2.49703132074851));
#67739=CARTESIAN_POINT('Ctrl Pts',(17.2025512209128,1.98645892302093,2.53775251143482));
#67740=CARTESIAN_POINT('Ctrl Pts',(17.203155178146,1.97900917220977,2.54356630648374));
#67741=CARTESIAN_POINT('Ctrl Pts',(17.2052627443095,1.95297666163645,2.56369851136851));
#67742=CARTESIAN_POINT('Ctrl Pts',(17.2067726140065,1.93426354186359,2.57784646640258));
#67743=CARTESIAN_POINT('Ctrl Pts',(17.2116091374084,1.87411874636929,2.62229500740112));
#67744=CARTESIAN_POINT('Ctrl Pts',(17.2149624125329,1.83211947298785,2.65180876073935));
#67745=CARTESIAN_POINT('Ctrl Pts',(17.218344821656,1.78943620926209,2.68030513477136));
#67746=CARTESIAN_POINT('Origin',(-1.72497344927317,0.,0.));
#67747=CARTESIAN_POINT('',(18.7170794495574,1.78943621037806,2.68030513402632));
#67748=CARTESIAN_POINT('',(18.4731355395702,1.78943620771753,2.68030513580255));
#67749=CARTESIAN_POINT('',(-1.72497344927317,1.78943621037804,2.68030513402633));
#67750=CARTESIAN_POINT('',(17.8965734493264,-3.22274931384398,0.00210300217175629));
#67751=CARTESIAN_POINT('Ctrl Pts',(17.8965734493264,-3.22274931384398,0.002103002171752));
#67752=CARTESIAN_POINT('Ctrl Pts',(17.9026568563018,-3.22281334652089,-0.0960239842600718));
#67753=CARTESIAN_POINT('Ctrl Pts',(17.9087402632772,-3.21839149416545,-0.194328558742725));
#67754=CARTESIAN_POINT('Ctrl Pts',(17.9148236702526,-3.20946154458654,-0.292359635244282));
#67755=CARTESIAN_POINT('Ctrl Pts',(17.9208998680669,-3.2005421774732,-0.390274539702337));
#67756=CARTESIAN_POINT('Ctrl Pts',(17.9269760658813,-3.1871253663105,-0.487916147950806));
#67757=CARTESIAN_POINT('Ctrl Pts',(17.9330522636956,-3.16924092933091,-0.584832877285252));
#67758=CARTESIAN_POINT('Ctrl Pts',(17.9391231590748,-3.15137209932627,-0.681665031580054));
#67759=CARTESIAN_POINT('Ctrl Pts',(17.945194054454,-3.12904347202547,-0.777773125995886));
#67760=CARTESIAN_POINT('Ctrl Pts',(17.9512649498332,-3.10233661305032,-0.872711350807052));
#67761=CARTESIAN_POINT('Ctrl Pts',(17.9573330655231,-3.07564198238142,-0.967606106122657));
#67762=CARTESIAN_POINT('Ctrl Pts',(17.9634011812131,-3.04457322120995,-1.06133162549463));
#67763=CARTESIAN_POINT('Ctrl Pts',(17.9694692969031,-3.00926263391265,-1.15345392740113));
#67764=CARTESIAN_POINT('Ctrl Pts',(17.9755363610955,-2.97395816531805,-1.24556026613567));
#67765=CARTESIAN_POINT('Ctrl Pts',(17.9816034252879,-2.93441349103862,-1.33606352173451));
#67766=CARTESIAN_POINT('Ctrl Pts',(17.9876704894804,-2.89080986879401,-1.42454760011141));
#67767=CARTESIAN_POINT('Ctrl Pts',(17.99373822901,-2.84720139294191,-1.51304152783025));
#67768=CARTESIAN_POINT('Ctrl Pts',(17.9998059685396,-2.79953327099698,-1.5995154313789));
#67769=CARTESIAN_POINT('Ctrl Pts',(18.0058737080692,-2.74803318804049,-1.68357689456942));
#67770=CARTESIAN_POINT('Ctrl Pts',(18.0119476112746,-2.6964807907403,-1.7677237483074));
#67771=CARTESIAN_POINT('Ctrl Pts',(18.01802151448,-2.64108889635926,-1.84945288785606));
#67772=CARTESIAN_POINT('Ctrl Pts',(18.0240954176853,-2.58212890738195,-1.92840033918336));
#67773=CARTESIAN_POINT('Ctrl Pts',(18.03017265551,-2.52313654891948,-2.00739113326562));
#67774=CARTESIAN_POINT('Ctrl Pts',(18.0362498933347,-2.46057248211144,-2.08359685528342));
#67775=CARTESIAN_POINT('Ctrl Pts',(18.0423271311594,-2.3947474046535,-2.15668783796018));
#67776=CARTESIAN_POINT('Ctrl Pts',(18.0484141616522,-2.32881625875608,-2.22989659712535));
#67777=CARTESIAN_POINT('Ctrl Pts',(18.0545011921449,-2.25961392689952,-2.29998028044469));
#67778=CARTESIAN_POINT('Ctrl Pts',(18.0605882226376,-2.18748671269529,-2.36664730035584));
#67779=CARTESIAN_POINT('Ctrl Pts',(18.0643877010504,-2.14246545090453,-2.40826035015047));
#67780=CARTESIAN_POINT('Ctrl Pts',(18.0681871794632,-2.09630526690075,-2.44854301873974));
#67781=CARTESIAN_POINT('Ctrl Pts',(18.071986657876,-2.04909615611315,-2.48743291477425));
#67782=CARTESIAN_POINT('Ctrl Pts',(18.0781589059687,-1.972405012655,-2.55060950391345));
#67783=CARTESIAN_POINT('Ctrl Pts',(18.0843311540615,-1.89265440894733,-2.61034721978994));
#67784=CARTESIAN_POINT('Ctrl Pts',(18.0905034021542,-1.81018580212359,-2.66633548607263));
#67785=CARTESIAN_POINT('Ctrl Pts',(18.0966672908069,-1.72782888740473,-2.72224792413959));
#67786=CARTESIAN_POINT('Ctrl Pts',(18.1028311794595,-1.6427616424801,-2.77442076406159));
#67787=CARTESIAN_POINT('Ctrl Pts',(18.1089950681121,-1.55535906571456,-2.82258316780915));
#67788=CARTESIAN_POINT('Ctrl Pts',(18.1151524297707,-1.46804904028062,-2.87069457197792));
#67789=CARTESIAN_POINT('Ctrl Pts',(18.1213097914292,-1.37840897771133,-2.91480377430139));
#67790=CARTESIAN_POINT('Ctrl Pts',(18.1274671530877,-1.28684256276156,-2.95468336394363));
#67791=CARTESIAN_POINT('Ctrl Pts',(18.133620017234,-1.19534303052784,-2.99453382439838));
#67792=CARTESIAN_POINT('Ctrl Pts',(18.1397728813803,-1.10192034043838,-3.03016064156325));
#67793=CARTESIAN_POINT('Ctrl Pts',(18.1459257455266,-1.00700164596564,-3.06138289789476));
#67794=CARTESIAN_POINT('Ctrl Pts',(18.1520762786632,-0.912118911396808,
-3.09259332568876));
#67795=CARTESIAN_POINT('Ctrl Pts',(18.1582268117997,-0.815741710762389,
-3.11940237270234));
#67796=CARTESIAN_POINT('Ctrl Pts',(18.1643773449362,-0.718315155376485,
-3.14167803889203));
#67797=CARTESIAN_POINT('Ctrl Pts',(18.1705271931515,-0.62089944937957,-3.16395122447089));
#67798=CARTESIAN_POINT('Ctrl Pts',(18.1766770413667,-0.522435044406073,
-3.18169193609567));
#67799=CARTESIAN_POINT('Ctrl Pts',(18.1828268895819,-0.423379137392556,
-3.19481887882877));
#67800=CARTESIAN_POINT('Ctrl Pts',(18.188977697961,-0.324307764971698,-3.20794787104608));
#67801=CARTESIAN_POINT('Ctrl Pts',(18.1951285063401,-0.224645137730853,
-3.21646160652262));
#67802=CARTESIAN_POINT('Ctrl Pts',(18.2012793147192,-0.124854492697445,
-3.22033056038557));
#67803=CARTESIAN_POINT('Ctrl Pts',(18.2074367010854,-0.0249571264768749,
-3.22420365190441));
#67804=CARTESIAN_POINT('Ctrl Pts',(18.2135940874516,0.075068096033463,-3.22342202563264));
#67805=CARTESIAN_POINT('Ctrl Pts',(18.2197514738178,0.174757130536443,-3.21800831382187));
#67806=CARTESIAN_POINT('Ctrl Pts',(18.2259122965547,0.274501800412089,-3.21259158067705));
#67807=CARTESIAN_POINT('Ctrl Pts',(18.2320731192917,0.373909476447318,-3.20253765747931));
#67808=CARTESIAN_POINT('Ctrl Pts',(18.2382339420287,0.472522526797308,-3.18792095638664));
#67809=CARTESIAN_POINT('Ctrl Pts',(18.2444050649454,0.571300446708627,-3.1732798178682));
#67810=CARTESIAN_POINT('Ctrl Pts',(18.2505761878621,0.66928066080252,-3.15406074754169));
#67811=CARTESIAN_POINT('Ctrl Pts',(18.2567473107787,0.766016855504997,-3.13038907159833));
#67812=CARTESIAN_POINT('Ctrl Pts',(18.2614428327244,0.839622086075572,-3.11237762127033));
#67813=CARTESIAN_POINT('Ctrl Pts',(18.26613835467,0.912507329936493,-3.09178940003567));
#67814=CARTESIAN_POINT('Ctrl Pts',(18.2708338766156,0.98448346849884,-3.06869839879264));
#67815=CARTESIAN_POINT('Ctrl Pts',(18.2770061247084,1.07909586497143,-3.03834535390593));
#67816=CARTESIAN_POINT('Ctrl Pts',(18.2831783728012,1.1724697320842,-3.0035592298004));
#67817=CARTESIAN_POINT('Ctrl Pts',(18.2893506208939,1.26415918089062,-2.96445933145826));
#67818=CARTESIAN_POINT('Ctrl Pts',(18.2955145095465,1.35572444926094,-2.92541238841785));
#67819=CARTESIAN_POINT('Ctrl Pts',(18.3016783981991,1.44560943763035,-2.88206345244063));
#67820=CARTESIAN_POINT('Ctrl Pts',(18.3078422868518,1.53338354917857,-2.83458153059822));
#67821=CARTESIAN_POINT('Ctrl Pts',(18.3139996485103,1.6210647159745,-2.78714988776617));
#67822=CARTESIAN_POINT('Ctrl Pts',(18.3201570101689,1.70663906983877,-2.73559416540845));
#67823=CARTESIAN_POINT('Ctrl Pts',(18.3263143718274,1.78969703426868,-2.68013098337187));
#67824=CARTESIAN_POINT('Ctrl Pts',(18.3324672359738,1.87269433079679,-2.62470831322245));
#67825=CARTESIAN_POINT('Ctrl Pts',(18.3386201001201,1.95317853208352,-2.56538409836791));
#67826=CARTESIAN_POINT('Ctrl Pts',(18.3447729642664,2.0307664824223,-2.50241984014876));
#67827=CARTESIAN_POINT('Ctrl Pts',(18.3509234974029,2.10832503860151,-2.4394794359101));
#67828=CARTESIAN_POINT('Ctrl Pts',(18.3570740305394,2.18298918713755,-2.37290200184059));
#67829=CARTESIAN_POINT('Ctrl Pts',(18.363224563676,2.25440721217204,-2.30299059577036));
#67830=CARTESIAN_POINT('Ctrl Pts',(18.3693744118912,2.32581728411885,-2.23308697501121));
#67831=CARTESIAN_POINT('Ctrl Pts',(18.3755242601064,2.39398164084689,-2.15985042424882));
#67832=CARTESIAN_POINT('Ctrl Pts',(18.3816741083216,2.45858468526504,-2.0836215846166));
#67833=CARTESIAN_POINT('Ctrl Pts',(18.3878249167007,2.52319781603173,-2.0073808435229));
#67834=CARTESIAN_POINT('Ctrl Pts',(18.3939757250798,2.58424824922221,-1.92814721702782));
#67835=CARTESIAN_POINT('Ctrl Pts',(18.4001265334589,2.64146067124637,-1.84629441984713));
#67836=CARTESIAN_POINT('Ctrl Pts',(18.4062839198251,2.69873427914218,-1.76435408512538));
#67837=CARTESIAN_POINT('Ctrl Pts',(18.4124413061913,2.75216143014478,-1.67978934298297));
#67838=CARTESIAN_POINT('Ctrl Pts',(18.4185986925575,2.80151024920306,-1.59300278910937));
#67839=CARTESIAN_POINT('Ctrl Pts',(18.4247595152944,2.85088660930384,-1.50616780059813));
#67840=CARTESIAN_POINT('Ctrl Pts',(18.4309203380314,2.89617990777551,-1.4171089181667));
#67841=CARTESIAN_POINT('Ctrl Pts',(18.4370811607683,2.9372052945644,-1.32625134121811));
#67842=CARTESIAN_POINT('Ctrl Pts',(18.443252283685,2.97829927103286,-1.23524186095851));
#67843=CARTESIAN_POINT('Ctrl Pts',(18.4494234066017,3.01511092275271,-1.14242808334039));
#67844=CARTESIAN_POINT('Ctrl Pts',(18.4555945295184,3.04750434891383,-1.04825321647552));
#67845=CARTESIAN_POINT('Ctrl Pts',(18.460290051464,3.07215205816974,-0.976596864777705));
#67846=CARTESIAN_POINT('Ctrl Pts',(18.4649855734096,3.0942428605833,-0.904152885904801));
#67847=CARTESIAN_POINT('Ctrl Pts',(18.4696810953552,3.11373673960027,-0.831120375735952));
#67848=CARTESIAN_POINT('Ctrl Pts',(18.475853343448,3.1393613791988,-0.735119382274197));
#67849=CARTESIAN_POINT('Ctrl Pts',(18.4820255915408,3.16058718753498,-0.637763239425528));
#67850=CARTESIAN_POINT('Ctrl Pts',(18.4881978396335,3.17727342830439,-0.539491542371941));
#67851=CARTESIAN_POINT('Ctrl Pts',(18.4943617282861,3.19393706991237,-0.441352940482053));
#67852=CARTESIAN_POINT('Ctrl Pts',(18.5005256169388,3.20607329211211,-0.342301673477271));
#67853=CARTESIAN_POINT('Ctrl Pts',(18.5066895055914,3.21359143704915,-0.242791347095304));
#67854=CARTESIAN_POINT('Ctrl Pts',(18.5128468672499,3.22110162095865,-0.14338639304334));
#67855=CARTESIAN_POINT('Ctrl Pts',(18.5190042289085,3.22400341708432,-0.0435237767830685));
#67856=CARTESIAN_POINT('Ctrl Pts',(18.525161590567,3.22225758576355,0.0563348337112121));
#67857=CARTESIAN_POINT('Ctrl Pts',(18.5313144547133,3.22051302964767,0.156120504633599));
#67858=CARTESIAN_POINT('Ctrl Pts',(18.5374673188597,3.21412760301785,0.255901742607642));
#67859=CARTESIAN_POINT('Ctrl Pts',(18.543620183006,3.20311410691901,0.355214837185091));
#67860=CARTESIAN_POINT('Ctrl Pts',(18.5497707161425,3.19210478327815,0.454490307041912));
#67861=CARTESIAN_POINT('Ctrl Pts',(18.555921249279,3.17647092187352,0.553297554657986));
#67862=CARTESIAN_POINT('Ctrl Pts',(18.5620717824156,3.1562772812874,0.651176847046182));
#67863=CARTESIAN_POINT('Ctrl Pts',(18.5682216306308,3.13608588945837,0.749045239628971));
#67864=CARTESIAN_POINT('Ctrl Pts',(18.574371478846,3.11133581574808,0.845985457016277));
#67865=CARTESIAN_POINT('Ctrl Pts',(18.5805213270612,3.08214296393584,0.941547827973059));
#67866=CARTESIAN_POINT('Ctrl Pts',(18.5866721354403,3.05294555430002,1.03712511889828));
#67867=CARTESIAN_POINT('Ctrl Pts',(18.5928229438194,3.01930411572692,1.13132372064531));
#67868=CARTESIAN_POINT('Ctrl Pts',(18.5989737521986,2.98138415548961,1.22370996559459));
#67869=CARTESIAN_POINT('Ctrl Pts',(18.6051311385648,2.94342364171983,1.31619501308906));
#67870=CARTESIAN_POINT('Ctrl Pts',(18.6112885249309,2.90117563440664,1.40686343072131));
#67871=CARTESIAN_POINT('Ctrl Pts',(18.6174459112971,2.85485342341849,1.49530247551983));
#67872=CARTESIAN_POINT('Ctrl Pts',(18.6236067340341,2.8085053605051,1.58379087719327));
#67873=CARTESIAN_POINT('Ctrl Pts',(18.629767556771,2.75807878497181,1.67004705324089));
#67874=CARTESIAN_POINT('Ctrl Pts',(18.635928379508,2.70383142802998,1.75368559647885));
#67875=CARTESIAN_POINT('Ctrl Pts',(18.6420995024247,2.64949337581088,1.8374639736423));
#67876=CARTESIAN_POINT('Ctrl Pts',(18.6482706253414,2.59132203573088,1.91861562311033));
#67877=CARTESIAN_POINT('Ctrl Pts',(18.6544417482581,2.52961675544487,1.99678657674589));
#67878=CARTESIAN_POINT('Ctrl Pts',(18.6591372702037,2.48266606240976,2.05626577255204));
#67879=CARTESIAN_POINT('Ctrl Pts',(18.6638327921493,2.4336702646636,2.11401995360804));
#67880=CARTESIAN_POINT('Ctrl Pts',(18.6685283140949,2.38277520607407,2.1699078044513));
#67881=CARTESIAN_POINT('Ctrl Pts',(18.6747006593625,2.31587276633024,2.24337335645331));
#67882=CARTESIAN_POINT('Ctrl Pts',(18.6808730046302,2.24545175883948,2.31387122200969));
#67883=CARTESIAN_POINT('Ctrl Pts',(18.6870453498979,2.1718058916275,2.38104530229731));
#67884=CARTESIAN_POINT('Ctrl Pts',(18.6932084687882,2.09827010972772,2.44811897125324));
#67885=CARTESIAN_POINT('Ctrl Pts',(18.6993715876786,2.021519372625,2.51187844534637));
#67886=CARTESIAN_POINT('Ctrl Pts',(18.705534706569,1.94188611155576,2.57200231186654));
#67887=CARTESIAN_POINT('Ctrl Pts',(18.7093829542318,1.89216315208627,2.60954361732096));
#67888=CARTESIAN_POINT('Ctrl Pts',(18.7132312018946,1.84131715179318,2.64566816899642));
#67889=CARTESIAN_POINT('Ctrl Pts',(18.7170794495574,1.78943621037806,2.68030513402632));
#67890=CARTESIAN_POINT('Ctrl Pts',(17.4669156580687,1.78943621037803,2.68030513402633));
#67891=CARTESIAN_POINT('Ctrl Pts',(17.4697587725981,1.75131203222926,2.70575775283613));
#67892=CARTESIAN_POINT('Ctrl Pts',(17.4726018871276,1.7126728546953,2.73037800620175));
#67893=CARTESIAN_POINT('Ctrl Pts',(17.475445001657,1.67355890093987,2.75414563296586));
#67894=CARTESIAN_POINT('Ctrl Pts',(17.4816172497498,1.58864461979969,2.80574386703093));
#67895=CARTESIAN_POINT('Ctrl Pts',(17.4877894978425,1.50119237257124,2.85350219556718));
#67896=CARTESIAN_POINT('Ctrl Pts',(17.4939617459353,1.41158440453206,2.89716189250478));
#67897=CARTESIAN_POINT('Ctrl Pts',(17.5001256345879,1.32209779785631,2.94076245853624));
#67898=CARTESIAN_POINT('Ctrl Pts',(17.5062895232406,1.23046166048895,2.98027523764615));
#67899=CARTESIAN_POINT('Ctrl Pts',(17.5124534118932,1.13708577126703,3.01548561782046));
#67900=CARTESIAN_POINT('Ctrl Pts',(17.5186107735517,1.04380875856788,3.05065871342394));
#67901=CARTESIAN_POINT('Ctrl Pts',(17.5247681352103,0.948796060755513,3.08153831512958));
#67902=CARTESIAN_POINT('Ctrl Pts',(17.5309254968688,0.852479659083573,3.1079568840878));
#67903=CARTESIAN_POINT('Ctrl Pts',(17.5370783610152,0.756233609653304,3.13435615617118));
#67904=CARTESIAN_POINT('Ctrl Pts',(17.5432312251615,0.658686167264141,3.15630075933928));
#67905=CARTESIAN_POINT('Ctrl Pts',(17.5493840893078,0.560285914103534,3.17367251885842));
#67906=CARTESIAN_POINT('Ctrl Pts',(17.5555346224443,0.461922939833879,3.19103769709441));
#67907=CARTESIAN_POINT('Ctrl Pts',(17.5616851555809,0.362708224050383,3.20383339855629));
#67908=CARTESIAN_POINT('Ctrl Pts',(17.5678356887174,0.26310114969074,3.21199242644366));
#67909=CARTESIAN_POINT('Ctrl Pts',(17.5739855369326,0.163505167541867,3.22015054574438));
#67910=CARTESIAN_POINT('Ctrl Pts',(17.5801353851478,0.063517346610522,3.22367298256498));
#67911=CARTESIAN_POINT('Ctrl Pts',(17.586285233363,-0.036398196497658,3.22254445024296));
#67912=CARTESIAN_POINT('Ctrl Pts',(17.5924360417421,-0.136329339226623,
3.22141574172538));
#67913=CARTESIAN_POINT('Ctrl Pts',(17.5985868501213,-0.236187747329852,
3.21563462665637));
#67914=CARTESIAN_POINT('Ctrl Pts',(17.6047376585004,-0.335510706137782,
3.20523792074269));
#67915=CARTESIAN_POINT('Ctrl Pts',(17.6108950448666,-0.434939885965303,
3.19483009606336));
#67916=CARTESIAN_POINT('Ctrl Pts',(17.6170524312328,-0.533832040144026,
3.17979686887251));
#67917=CARTESIAN_POINT('Ctrl Pts',(17.623209817599,-0.631731090493708,3.16022679436202));
#67918=CARTESIAN_POINT('Ctrl Pts',(17.6293706403359,-0.729684777245112,
3.1406457980045));
#67919=CARTESIAN_POINT('Ctrl Pts',(17.6355314630729,-0.826643834866129,
3.11652301682949));
#67920=CARTESIAN_POINT('Ctrl Pts',(17.6416922858098,-0.92216591387072,3.08799734290608));
#67921=CARTESIAN_POINT('Ctrl Pts',(17.6478634087265,-1.01784769469178,3.05942397737054));
#67922=CARTESIAN_POINT('Ctrl Pts',(17.6540345316432,-1.11208728788402,3.02643315905609));
#67923=CARTESIAN_POINT('Ctrl Pts',(17.6602056545599,-1.20446080492819,2.98921256050682));
#67924=CARTESIAN_POINT('Ctrl Pts',(17.6649011765055,-1.27474653449925,2.96089192264634));
#67925=CARTESIAN_POINT('Ctrl Pts',(17.6695966984511,-1.34395228700999,2.9301234737808));
#67926=CARTESIAN_POINT('Ctrl Pts',(17.6742922203967,-1.41190142362904,2.89700740980314));
#67927=CARTESIAN_POINT('Ctrl Pts',(17.6804644684894,-1.50122033934532,2.85347645305443));
#67928=CARTESIAN_POINT('Ctrl Pts',(17.6866367165822,-1.588681396552,2.8057342603715));
#67929=CARTESIAN_POINT('Ctrl Pts',(17.692808964675,-1.67386026863737,2.75396248405407));
#67930=CARTESIAN_POINT('Ctrl Pts',(17.6989728533276,-1.75892377794558,2.70226082531096));
#67931=CARTESIAN_POINT('Ctrl Pts',(17.7051367419802,-1.84171087771072,2.6465406539447));
#67932=CARTESIAN_POINT('Ctrl Pts',(17.7113006306329,-1.92181946278051,2.58703063665238));
#67933=CARTESIAN_POINT('Ctrl Pts',(17.7174579922914,-2.00184322018855,2.52758363502328));
#67934=CARTESIAN_POINT('Ctrl Pts',(17.72361535395,-2.0791937549697,2.46435502349232));
#67935=CARTESIAN_POINT('Ctrl Pts',(17.7297727156085,-2.15349655526324,2.39761759856933));
#67936=CARTESIAN_POINT('Ctrl Pts',(17.7359255797548,-2.2277450826763,2.33092892056129));
#67937=CARTESIAN_POINT('Ctrl Pts',(17.7420784439011,-2.29894997938641,2.26073681410068));
#67938=CARTESIAN_POINT('Ctrl Pts',(17.7482313080474,-2.36676928277229,2.18735473223379));
#67939=CARTESIAN_POINT('Ctrl Pts',(17.754381841184,-2.43456289284608,2.11400045113507));
#67940=CARTESIAN_POINT('Ctrl Pts',(17.7605323743205,-2.49897316368225,2.03745891460282));
#67941=CARTESIAN_POINT('Ctrl Pts',(17.766682907457,-2.55969517567515,1.95808022566118));
#67942=CARTESIAN_POINT('Ctrl Pts',(17.7728327556722,-2.62041042568495,1.87871037630401));
#67943=CARTESIAN_POINT('Ctrl Pts',(17.7789826038874,-2.67743796951116,1.79650434768742));
#67944=CARTESIAN_POINT('Ctrl Pts',(17.7851324521027,-2.73051399527618,1.71184429318233));
#67945=CARTESIAN_POINT('Ctrl Pts',(17.7912832604818,-2.78359830769865,1.62717102086636));
#67946=CARTESIAN_POINT('Ctrl Pts',(17.7974340688609,-2.83272964590099,1.54004332970663));
#67947=CARTESIAN_POINT('Ctrl Pts',(17.8035848772401,-2.87768878502424,1.45087036603747));
#67948=CARTESIAN_POINT('Ctrl Pts',(17.8097422636063,-2.92269600573557,1.36160203626944));
#67949=CARTESIAN_POINT('Ctrl Pts',(17.8158996499724,-2.96352192135572,1.27028445476588));
#67950=CARTESIAN_POINT('Ctrl Pts',(17.8220570363386,-2.99999441915956,1.17734916125654));
#67951=CARTESIAN_POINT('Ctrl Pts',(17.8282178590756,-3.03648727187019,1.08436200156448));
#67952=CARTESIAN_POINT('Ctrl Pts',(17.8343786818125,-3.06862172855124,0.989755743208075));
#67953=CARTESIAN_POINT('Ctrl Pts',(17.8405395045495,-3.09627544355293,0.893977594882056));
#67954=CARTESIAN_POINT('Ctrl Pts',(17.8467106274662,-3.12397539235274,0.798039316621462));
#67955=CARTESIAN_POINT('Ctrl Pts',(17.8528817503829,-3.14717953487941,0.700925657501339));
#67956=CARTESIAN_POINT('Ctrl Pts',(17.8590528732996,-3.16581654208732,0.603094672788866));
#67957=CARTESIAN_POINT('Ctrl Pts',(17.8637483952451,-3.17999718271397,0.52865643166556));
#67958=CARTESIAN_POINT('Ctrl Pts',(17.8684439171907,-3.19153474824845,0.453803120398392));
#67959=CARTESIAN_POINT('Ctrl Pts',(17.8731394391363,-3.20041801394429,0.378737506092117));
#67960=CARTESIAN_POINT('Ctrl Pts',(17.8809507758485,-3.21519596201036,0.253860485889424));
#67961=CARTESIAN_POINT('Ctrl Pts',(17.8887621125608,-3.22266709330376,0.128101959648026));
#67962=CARTESIAN_POINT('Ctrl Pts',(17.8965734492731,-3.22274931384342,0.00210300303191614));
#67963=CARTESIAN_POINT('Ctrl Pts',(17.218344821656,1.78943620926209,2.68030513477136));
#67964=CARTESIAN_POINT('Ctrl Pts',(17.218996255307,1.78121564418187,2.68579338184603));
#67965=CARTESIAN_POINT('Ctrl Pts',(17.2196487630733,1.77296970763706,2.69124389172866));
#67966=CARTESIAN_POINT('Ctrl Pts',(17.236471424427,1.56006568899324,2.83056880659984));
#67967=CARTESIAN_POINT('Ctrl Pts',(17.2532926280998,1.34087819022421,2.94074052014517));
#67968=CARTESIAN_POINT('Ctrl Pts',(17.2740174238738,1.0484075159506,3.04818902544994));
#67969=CARTESIAN_POINT('Ctrl Pts',(17.2784255491868,0.984749776020059,3.06934581850393));
#67970=CARTESIAN_POINT('Ctrl Pts',(17.2849851458498,0.887141057238322,3.0984363953252));
#67971=CARTESIAN_POINT('Ctrl Pts',(17.2872009426343,0.853647615099221,3.10783097013015));
#67972=CARTESIAN_POINT('Ctrl Pts',(17.2898945850584,0.812197532181473,3.11873659378563));
#67973=CARTESIAN_POINT('Ctrl Pts',(17.2904004797907,0.804380230094272,3.12076196167777));
#67974=CARTESIAN_POINT('Ctrl Pts',(17.2911932523726,0.79207725323583,3.12390021368537));
#67975=CARTESIAN_POINT('Ctrl Pts',(17.2914812564977,0.787596722164427,3.12503285167271));
#67976=CARTESIAN_POINT('Ctrl Pts',(17.2920189834721,0.779210243314774,3.12713369599776));
#67977=CARTESIAN_POINT('Ctrl Pts',(17.2922688353303,0.775304960996747,3.12810421399642));
#67978=CARTESIAN_POINT('Ctrl Pts',(17.2928349951901,0.766436372916174,3.13029055529922));
#67979=CARTESIAN_POINT('Ctrl Pts',(17.2931510407565,0.761471999657033,3.1315018871014));
#67980=CARTESIAN_POINT('Ctrl Pts',(17.29410737286,0.746409457751866,3.13513928582453));
#67981=CARTESIAN_POINT('Ctrl Pts',(17.29474555719,0.736302303227153,3.13752838159355));
#67982=CARTESIAN_POINT('Ctrl Pts',(17.2994078367798,0.662073595017321,3.15469587434005));
#67983=CARTESIAN_POINT('Ctrl Pts',(17.303327763258,0.597519209537753,3.1675573717906));
#67984=CARTESIAN_POINT('Ctrl Pts',(17.3106504595164,0.474009369588108,3.18825395626274));
#67985=CARTESIAN_POINT('Ctrl Pts',(17.3140650369906,0.41514433878044,3.19645178341192));
#67986=CARTESIAN_POINT('Ctrl Pts',(17.3254168135382,0.216768991329332,3.21850543603342));
#67987=CARTESIAN_POINT('Ctrl Pts',(17.3331875647572,0.0765881523064569,
3.22488802704263));
#67988=CARTESIAN_POINT('Ctrl Pts',(17.3530210348043,-0.277439556604902,
3.21790371907984));
#67989=CARTESIAN_POINT('Ctrl Pts',(17.3651732031636,-0.490328704767302,
3.19240293092688));
#67990=CARTESIAN_POINT('Ctrl Pts',(17.3794578096054,-0.721809880852266,
3.14096305293035));
#67991=CARTESIAN_POINT('Ctrl Pts',(17.380866369542,-0.744456347208361,3.13567267224105));
#67992=CARTESIAN_POINT('Ctrl Pts',(17.3828942238259,-0.776792857861574,
3.12774858067602));
#67993=CARTESIAN_POINT('Ctrl Pts',(17.3835070945248,-0.786531285234542,
3.12531388210939));
#67994=CARTESIAN_POINT('Ctrl Pts',(17.3845710019956,-0.803376015042545,
3.1210188239924));
#67995=CARTESIAN_POINT('Ctrl Pts',(17.3850213521265,-0.810487663876386,
3.11917958228552));
#67996=CARTESIAN_POINT('Ctrl Pts',(17.3858875844682,-0.824130441794685,
3.11560142774978));
#67997=CARTESIAN_POINT('Ctrl Pts',(17.3863033433176,-0.830662517449225,
3.11386624996699));
#67998=CARTESIAN_POINT('Ctrl Pts',(17.3872830738975,-0.846017478948949,
3.10973561084354));
#67999=CARTESIAN_POINT('Ctrl Pts',(17.3878475966572,-0.854835691112436,
3.10732313776235));
#68000=CARTESIAN_POINT('Ctrl Pts',(17.3895174142792,-0.880831918339204,
3.10009209486116));
#68001=CARTESIAN_POINT('Ctrl Pts',(17.3906261259373,-0.897980105891992,
3.09516842413682));
#68002=CARTESIAN_POINT('Ctrl Pts',(17.402967686621,-1.08759881269832,3.03901576874802));
#68003=CARTESIAN_POINT('Ctrl Pts',(17.4146758129753,-1.25550035156639,2.97358157797115));
#68004=CARTESIAN_POINT('Ctrl Pts',(17.433466353701,-1.5080701036121,2.84993223668737));
#68005=CARTESIAN_POINT('Ctrl Pts',(17.4403206066947,-1.59694044066333,2.80110140496957));
#68006=CARTESIAN_POINT('Ctrl Pts',(17.460474393217,-1.85083920250379,2.64557851648796));
#68007=CARTESIAN_POINT('Ctrl Pts',(17.4737674548813,-2.00861045809417,2.52788313360291));
#68008=CARTESIAN_POINT('Ctrl Pts',(17.4871655174868,-2.16586164017598,2.38650087129517));
#68009=CARTESIAN_POINT('Ctrl Pts',(17.4881116942534,-2.17695822764668,2.37638295499818));
#68010=CARTESIAN_POINT('Ctrl Pts',(17.489424054336,-2.19234333798265,2.36215653691083));
#68011=CARTESIAN_POINT('Ctrl Pts',(17.4897950241741,-2.19669162946884,2.35811337785725));
#68012=CARTESIAN_POINT('Ctrl Pts',(17.4904239228963,-2.20406251590948,2.35122164800931));
#68013=CARTESIAN_POINT('Ctrl Pts',(17.4906823200298,-2.20709080965138,2.3483792220818));
#68014=CARTESIAN_POINT('Ctrl Pts',(17.4911738297685,-2.21285086271516,2.34295172092911));
#68015=CARTESIAN_POINT('Ctrl Pts',(17.4914070246026,-2.2155835956161,2.34036771435768));
#68016=CARTESIAN_POINT('Ctrl Pts',(17.491954954221,-2.22200415097917,2.33427526748916));
#68017=CARTESIAN_POINT('Ctrl Pts',(17.4922693814721,-2.2256882105153,2.33076284975408));
#68018=CARTESIAN_POINT('Ctrl Pts',(17.4931956853666,-2.2365397688213,2.32036767974182));
#68019=CARTESIAN_POINT('Ctrl Pts',(17.4938057013579,-2.24368385258729,2.3134604129694));
#68020=CARTESIAN_POINT('Ctrl Pts',(17.4995103242819,-2.31045621059005,2.24830123459879));
#68021=CARTESIAN_POINT('Ctrl Pts',(17.5044364285496,-2.36784105968864,2.18778375211872));
#68022=CARTESIAN_POINT('Ctrl Pts',(17.5115345959294,-2.44869744046942,2.09559980242966));
#68023=CARTESIAN_POINT('Ctrl Pts',(17.5137836070429,-2.47403515419072,2.0656253087844));
#68024=CARTESIAN_POINT('Ctrl Pts',(17.5239945856777,-2.58734981215462,1.92649714339337));
#68025=CARTESIAN_POINT('Ctrl Pts',(17.5317672934675,-2.66869582655016,1.81213560991748));
#68026=CARTESIAN_POINT('Ctrl Pts',(17.5519599646978,-2.85809864132709,1.50530953802706));
#68027=CARTESIAN_POINT('Ctrl Pts',(17.5644783940036,-2.95430152447993,1.30643300124577));
#68028=CARTESIAN_POINT('Ctrl Pts',(17.5789888136548,-3.03627896164313,1.08052175918995));
#68029=CARTESIAN_POINT('Ctrl Pts',(17.5802015031873,-3.0429229984093,1.0616669924705));
#68030=CARTESIAN_POINT('Ctrl Pts',(17.5819953737513,-3.05244517678235,1.03382063303629));
#68031=CARTESIAN_POINT('Ctrl Pts',(17.5825720206181,-3.05546000049047,1.02487601248616));
#68032=CARTESIAN_POINT('Ctrl Pts',(17.5835938814549,-3.06072086425352,1.00903811343204));
#68033=CARTESIAN_POINT('Ctrl Pts',(17.5840385588038,-3.06298302973659,1.0021502289661));
#68034=CARTESIAN_POINT('Ctrl Pts',(17.5849095589254,-3.06736082280074,0.988667342908383));
#68035=CARTESIAN_POINT('Ctrl Pts',(17.5853358121773,-3.0694784711606,0.982073034998844));
#68036=CARTESIAN_POINT('Ctrl Pts',(17.5864879909021,-3.07513568388318,0.964259553575727));
#68037=CARTESIAN_POINT('Ctrl Pts',(17.5872152334363,-3.07863507505134,0.953027822114359));
#68038=CARTESIAN_POINT('Ctrl Pts',(17.5899197131768,-3.09138392002294,0.911305783384572));
#68039=CARTESIAN_POINT('Ctrl Pts',(17.5919096936923,-3.10024229841894,0.880698782386737));
#68040=CARTESIAN_POINT('Ctrl Pts',(17.6120433145843,-3.18463193221272,0.572054289843209));
#68041=CARTESIAN_POINT('Ctrl Pts',(17.6314669497433,-3.22299288741503,0.285259651166556));
#68042=CARTESIAN_POINT('Ctrl Pts',(17.6596739779669,-3.22263943885347,-0.131835884447859));
#68043=CARTESIAN_POINT('Ctrl Pts',(17.6683619514602,-3.21477208702586,-0.260827695952668));
#68044=CARTESIAN_POINT('Ctrl Pts',(17.6800887164683,-3.19303344089445,-0.439605475919181));
#68045=CARTESIAN_POINT('Ctrl Pts',(17.68336176788,-3.18568105890001,-0.490053491736329));
#68046=CARTESIAN_POINT('Ctrl Pts',(17.6871192593359,-3.17567832006897,-0.54887176034701));
#68047=CARTESIAN_POINT('Ctrl Pts',(17.6876644348986,-3.17418751190498,-0.557428601003604));
#68048=CARTESIAN_POINT('Ctrl Pts',(17.6885348904489,-3.17174337731699,-0.571129475717084));
#68049=CARTESIAN_POINT('Ctrl Pts',(17.6888613910862,-3.17081210024894,-0.576277325099635));
#68050=CARTESIAN_POINT('Ctrl Pts',(17.6894392563615,-3.1691379969091,-0.585404393940074));
#68051=CARTESIAN_POINT('Ctrl Pts',(17.6896909064771,-3.16840020426217,-0.589384504583058));
#68052=CARTESIAN_POINT('Ctrl Pts',(17.6902211700118,-3.16682703890943,-0.597782808165955));
#68053=CARTESIAN_POINT('Ctrl Pts',(17.6904996817189,-3.16598992070272,-0.602200633265005));
#68054=CARTESIAN_POINT('Ctrl Pts',(17.6912421688003,-3.16372933332074,-0.613995698080348));
#68055=CARTESIAN_POINT('Ctrl Pts',(17.6917052038299,-3.16228929689642,-0.621369791003705));
#68056=CARTESIAN_POINT('Ctrl Pts',(17.6938884455929,-3.15535668754718,-0.656221707228936));
#68057=CARTESIAN_POINT('Ctrl Pts',(17.6955903359931,-3.14953148252711,-0.683633176718141));
#68058=CARTESIAN_POINT('Ctrl Pts',(17.7116371207942,-3.09065237982463,-0.943951555649504));
#68059=CARTESIAN_POINT('Ctrl Pts',(17.7247500515091,-3.01220774887604,-1.17039091274974));
#68060=CARTESIAN_POINT('Ctrl Pts',(17.7505932821299,-2.81368186425124,-1.58709819479223));
#68061=CARTESIAN_POINT('Ctrl Pts',(17.7632318171866,-2.6973706685749,-1.77759879206017));
#68062=CARTESIAN_POINT('Ctrl Pts',(17.7777512614815,-2.55154090473208,-1.96877506872042));
#68063=CARTESIAN_POINT('Ctrl Pts',(17.778833784184,-2.54059612375943,-1.98287860845329));
#68064=CARTESIAN_POINT('Ctrl Pts',(17.7804778784141,-2.52386836668892,-2.00406827814829));
#68065=CARTESIAN_POINT('Ctrl Pts',(17.781036023722,-2.51817135367504,-2.01122207293809));
#68066=CARTESIAN_POINT('Ctrl Pts',(17.7820088342172,-2.50821075188735,-2.0236210305915));
#68067=CARTESIAN_POINT('Ctrl Pts',(17.7824229433581,-2.50396094698811,-2.02887723290264));
#68068=CARTESIAN_POINT('Ctrl Pts',(17.7832884468379,-2.49505861724397,-2.03981715100268));
#68069=CARTESIAN_POINT('Ctrl Pts',(17.7837399594041,-2.49040313894979,-2.04549840310207));
#68070=CARTESIAN_POINT('Ctrl Pts',(17.7848102166945,-2.47934137779691,-2.05890373661293));
#68071=CARTESIAN_POINT('Ctrl Pts',(17.7854296406917,-2.47291838758104,-2.06661387516059));
#68072=CARTESIAN_POINT('Ctrl Pts',(17.7874883783825,-2.45150268554474,-2.09207842713798));
#68073=CARTESIAN_POINT('Ctrl Pts',(17.7889340845569,-2.43635422972455,-2.10970035413202));
#68074=CARTESIAN_POINT('Ctrl Pts',(17.8034796649227,-2.28288025927146,-2.28437629246379));
#68075=CARTESIAN_POINT('Ctrl Pts',(17.8172282167309,-2.12978444742709,-2.42773677416274));
#68076=CARTESIAN_POINT('Ctrl Pts',(17.8407842890914,-1.85225478291416,-2.64104135461136));
#68077=CARTESIAN_POINT('Ctrl Pts',(17.8503726521199,-1.73510142564146,-2.71944293848149));
#68078=CARTESIAN_POINT('Ctrl Pts',(17.8649765268354,-1.54674434223661,-2.82835497076971));
#68079=CARTESIAN_POINT('Ctrl Pts',(17.8700817997819,-1.47893606540631,-2.86439513020792));
#68080=CARTESIAN_POINT('Ctrl Pts',(17.8785730916323,-1.36184144777993,-2.9213630241878));
#68081=CARTESIAN_POINT('Ctrl Pts',(17.8820088150027,-1.31320361822395,-2.94354736842773));
#68082=CARTESIAN_POINT('Ctrl Pts',(17.8859309811665,-1.25592658562948,-2.96796961556646));
#68083=CARTESIAN_POINT('Ctrl Pts',(17.886484214146,-1.24780572141544,-2.9713929584096));
#68084=CARTESIAN_POINT('Ctrl Pts',(17.8873650411718,-1.23480740621754,-2.97680970037566));
#68085=CARTESIAN_POINT('Ctrl Pts',(17.887693901688,-1.22993900229697,-2.97882449537912));
#68086=CARTESIAN_POINT('Ctrl Pts',(17.8882744608355,-1.22131671303639,-2.98236809888988));
#68087=CARTESIAN_POINT('Ctrl Pts',(17.8885264542168,-1.21756486051184,-2.9839017748561));
#68088=CARTESIAN_POINT('Ctrl Pts',(17.8890558515707,-1.20966302881378,-2.98711448726941));
#68089=CARTESIAN_POINT('Ctrl Pts',(17.8893331596651,-1.20551245278582,-2.98879195162424));
#68090=CARTESIAN_POINT('Ctrl Pts',(17.8900690302999,-1.19446840769231,-2.99322867792044));
#68091=CARTESIAN_POINT('Ctrl Pts',(17.8905266817445,-1.187568825033,-2.99597279421586));
#68092=CARTESIAN_POINT('Ctrl Pts',(17.8926474999511,-1.15545440166465,-3.00861703816584));
#68093=CARTESIAN_POINT('Ctrl Pts',(17.894293597801,-1.13012396598836,-3.01822320108332));
#68094=CARTESIAN_POINT('Ctrl Pts',(17.8987566630976,-1.06044611590274,-3.04364718355415));
#68095=CARTESIAN_POINT('Ctrl Pts',(17.9015407890691,-1.01586705930184,-3.05881492316037));
#68096=CARTESIAN_POINT('Ctrl Pts',(17.9110170677043,-0.861047873108858,
-3.10773279739154));
#68097=CARTESIAN_POINT('Ctrl Pts',(17.9175241502935,-0.74933407218692,-3.13654407024733));
#68098=CARTESIAN_POINT('Ctrl Pts',(17.9397888966039,-0.359881347184209,
-3.21498294552861));
#68099=CARTESIAN_POINT('Ctrl Pts',(17.9553426193508,-0.077377678183578,
-3.23413448481953));
#68100=CARTESIAN_POINT('Ctrl Pts',(17.9728184250106,0.213937365374667,-3.2156566024651));
#68101=CARTESIAN_POINT('Ctrl Pts',(17.9734155425346,0.223865171433876,-3.21498070958324));
#68102=CARTESIAN_POINT('Ctrl Pts',(17.9755188615752,0.25874186052237,-3.21244394830643));
#68103=CARTESIAN_POINT('Ctrl Pts',(17.9770324388021,0.283671575761402,-3.2103385887447));
#68104=CARTESIAN_POINT('Ctrl Pts',(17.9791381362927,0.318108239451829,-3.2070261081837));
#68105=CARTESIAN_POINT('Ctrl Pts',(17.9797224667968,0.327638535033711,-3.20606648368826));
#68106=CARTESIAN_POINT('Ctrl Pts',(17.9807283100963,0.343998398663553,-3.2043454691331));
#68107=CARTESIAN_POINT('Ctrl Pts',(17.9811491708191,0.350830107200836,-3.20360469136875));
#68108=CARTESIAN_POINT('Ctrl Pts',(17.9820169687281,0.364888676387711,-3.20203477982202));
#68109=CARTESIAN_POINT('Ctrl Pts',(17.9824639866112,0.372115198423704,-3.20120301684624));
#68110=CARTESIAN_POINT('Ctrl Pts',(17.983503156922,0.388878623196843,-3.19921603925885));
#68111=CARTESIAN_POINT('Ctrl Pts',(17.9840958810206,0.398413263188915,-3.19804263854369));
#68112=CARTESIAN_POINT('Ctrl Pts',(17.9859808196012,0.428648153774528,-3.1941844078));
#68113=CARTESIAN_POINT('Ctrl Pts',(17.9872780326044,0.449327311523937,-3.19134112950069));
#68114=CARTESIAN_POINT('Ctrl Pts',(18.0009472029659,0.665854576657254,-3.15942351688875));
#68115=CARTESIAN_POINT('Ctrl Pts',(18.0138982512026,0.858618047448988,-3.11256626904443));
#68116=CARTESIAN_POINT('Ctrl Pts',(18.0426237318469,1.26347051668131,-2.97366774463613));
#68117=CARTESIAN_POINT('Ctrl Pts',(18.0584422536356,1.47248204088198,-2.87590981722368));
#68118=CARTESIAN_POINT('Ctrl Pts',(18.077098668881,1.71690593136426,-2.72790185009183));
#68119=CARTESIAN_POINT('Ctrl Pts',(18.0806794503136,1.7637576385851,-2.69784624742659));
#68120=CARTESIAN_POINT('Ctrl Pts',(18.0847479701244,1.81719289233825,-2.66157982333475));
#68121=CARTESIAN_POINT('Ctrl Pts',(18.0853081217614,1.82455443092031,-2.6565387813808));
#68122=CARTESIAN_POINT('Ctrl Pts',(18.0861978441412,1.83625618219817,-2.64845405740705));
#68123=CARTESIAN_POINT('Ctrl Pts',(18.0865287212972,1.84060991958709,-2.6454301702621));
#68124=CARTESIAN_POINT('Ctrl Pts',(18.087111594041,1.84828336680693,-2.64007246587258));
#68125=CARTESIAN_POINT('Ctrl Pts',(18.0873638923026,1.85160615270468,-2.63774310444972));
#68126=CARTESIAN_POINT('Ctrl Pts',(18.0878926039503,1.85857221079515,-2.63284006281744));
#68127=CARTESIAN_POINT('Ctrl Pts',(18.0881689263029,1.86221453292502,-2.63026509938734));
#68128=CARTESIAN_POINT('Ctrl Pts',(18.088899379119,1.87184681421547,-2.62342545788328));
#68129=CARTESIAN_POINT('Ctrl Pts',(18.0893526221596,1.87782758714492,-2.61914779735983));
#68130=CARTESIAN_POINT('Ctrl Pts',(18.0914237025256,1.90517138709063,-2.59944873781665));
#68131=CARTESIAN_POINT('Ctrl Pts',(18.0930254312597,1.92636017694078,-2.58378565830548));
#68132=CARTESIAN_POINT('Ctrl Pts',(18.107186686904,2.11376046229517,-2.44166950653747));
#68133=CARTESIAN_POINT('Ctrl Pts',(18.1187919837638,2.26752971679767,-2.29957975580011));
#68134=CARTESIAN_POINT('Ctrl Pts',(18.1447488558559,2.5764955199715,-1.95272209802431));
#68135=CARTESIAN_POINT('Ctrl Pts',(18.1590974014191,2.72317476170245,-1.74233981235439));
#68136=CARTESIAN_POINT('Ctrl Pts',(18.1756981063697,2.85251160315852,-1.49988831870937));
#68137=CARTESIAN_POINT('Ctrl Pts',(18.1768651687894,2.86141111983531,-1.48283977327762));
#68138=CARTESIAN_POINT('Ctrl Pts',(18.1786040933243,2.87438314414717,-1.45743796932309));
#68139=CARTESIAN_POINT('Ctrl Pts',(18.1791718154387,2.87857307825575,-1.44914489409222));
#68140=CARTESIAN_POINT('Ctrl Pts',(18.1801835738701,2.88595962933506,-1.43436636140056));
#68141=CARTESIAN_POINT('Ctrl Pts',(18.1806271098279,2.88917040657127,-1.42788802127776));
#68142=CARTESIAN_POINT('Ctrl Pts',(18.1815612363618,2.89587500817863,-1.41424504177749));
#68143=CARTESIAN_POINT('Ctrl Pts',(18.1820519884977,2.89936410202991,-1.40707814396426));
#68144=CARTESIAN_POINT('Ctrl Pts',(18.1833462586601,2.90847836808413,-1.38817882030668));
#68145=CARTESIAN_POINT('Ctrl Pts',(18.1841513159129,2.91405909671061,-1.37642523504178));
#68146=CARTESIAN_POINT('Ctrl Pts',(18.1877952441244,2.93891924628962,-1.32323831571081));
#68147=CARTESIAN_POINT('Ctrl Pts',(18.1906619729058,2.95738642937206,-1.28143323564138));
#68148=CARTESIAN_POINT('Ctrl Pts',(18.1983782706955,3.00419238989113,-1.16907042778489));
#68149=CARTESIAN_POINT('Ctrl Pts',(18.2032790627917,3.03093237427858,-1.09788206104661));
#68150=CARTESIAN_POINT('Ctrl Pts',(18.2287185772952,3.15473996469066,-0.729154204719931));
#68151=CARTESIAN_POINT('Ctrl Pts',(18.2504686754304,3.21059606269129,-0.419618568786852));
#68152=CARTESIAN_POINT('Ctrl Pts',(18.2750292354069,3.22303290713635,-0.0449510719625321));
#68153=CARTESIAN_POINT('Ctrl Pts',(18.2790293408244,3.22330135641951,0.0170675943606899));
#68154=CARTESIAN_POINT('Ctrl Pts',(18.2835736626479,3.22153250228033,0.0891502898599032));
#68155=CARTESIAN_POINT('Ctrl Pts',(18.2842073232337,3.2212374896472,0.0992395038693905));
#68156=CARTESIAN_POINT('Ctrl Pts',(18.2851584794236,3.22072139776817,0.114444100032095));
#68157=CARTESIAN_POINT('Ctrl Pts',(18.2854779014298,3.2205355241234,0.119560498489084));
#68158=CARTESIAN_POINT('Ctrl Pts',(18.2860472125515,3.22018174616714,0.128698424547651));
#68159=CARTESIAN_POINT('Ctrl Pts',(18.2862973608781,3.22001850022707,0.132720087590041));
#68160=CARTESIAN_POINT('Ctrl Pts',(18.2868333976551,3.21965190815539,0.141352219116043));
#68161=CARTESIAN_POINT('Ctrl Pts',(18.287119150823,3.21944619402374,0.14596254300184));
#68162=CARTESIAN_POINT('Ctrl Pts',(18.2879015721003,3.2188546711652,0.158609269246529));
#68163=CARTESIAN_POINT('Ctrl Pts',(18.2883971152335,3.21844866690736,0.166644760228525));
#68164=CARTESIAN_POINT('Ctrl Pts',(18.2910019841578,3.21614880508485,0.209013877060418));
#68165=CARTESIAN_POINT('Ctrl Pts',(18.2930833254905,3.21373555381913,0.243318624275949));
#68166=CARTESIAN_POINT('Ctrl Pts',(18.2990848569302,3.20509277813615,0.343289866775975));
#68167=CARTESIAN_POINT('Ctrl Pts',(18.3029378835285,3.19739573311508,0.408814539826498));
#68168=CARTESIAN_POINT('Ctrl Pts',(18.3211497671374,3.15084616686602,0.721824333985837));
#68169=CARTESIAN_POINT('Ctrl Pts',(18.3347468557573,3.08523952595941,0.96445501732195));
#68170=CARTESIAN_POINT('Ctrl Pts',(18.3492148114757,2.99102920573645,1.19994649356021));
#68171=CARTESIAN_POINT('Ctrl Pts',(18.3493928710357,2.9898661101187,1.20284161073554));
#68172=CARTESIAN_POINT('Ctrl Pts',(18.3498882776976,2.98662003149034,1.21088778266241));
#68173=CARTESIAN_POINT('Ctrl Pts',(18.3502058185659,2.98452793305053,1.21603513566622));
#68174=CARTESIAN_POINT('Ctrl Pts',(18.3530717558043,2.96554348532392,1.26239994852628));
#68175=CARTESIAN_POINT('Ctrl Pts',(18.3556385441123,2.94781206785718,1.30326727496762));
#68176=CARTESIAN_POINT('Ctrl Pts',(18.3586692120556,2.92608353283526,1.35063319291652));
#68177=CARTESIAN_POINT('Ctrl Pts',(18.3591101126738,2.92290306504024,1.3575023146057));
#68178=CARTESIAN_POINT('Ctrl Pts',(18.364329719472,2.88502450850945,1.43856153043603));
#68179=CARTESIAN_POINT('Ctrl Pts',(18.3691878440013,2.84753709651971,1.51140876445932));
#68180=CARTESIAN_POINT('Ctrl Pts',(18.3750511455947,2.79996631707882,1.59578516216952));
#68181=CARTESIAN_POINT('Ctrl Pts',(18.3759605039468,2.79252368158289,1.60877379908814));
#68182=CARTESIAN_POINT('Ctrl Pts',(18.3774409514536,2.78030406481381,1.62975876121442));
#68183=CARTESIAN_POINT('Ctrl Pts',(18.3780100345254,2.77558237895084,1.63778715569596));
#68184=CARTESIAN_POINT('Ctrl Pts',(18.3790233251997,2.76713213321772,1.65201381328183));
#68185=CARTESIAN_POINT('Ctrl Pts',(18.3794670269255,2.76341736857454,1.65822022893991));
#68186=CARTESIAN_POINT('Ctrl Pts',(18.3804005919381,2.75557106268429,1.67122979668467));
#68187=CARTESIAN_POINT('Ctrl Pts',(18.3808906134647,2.75143515417554,1.67803024566919));
#68188=CARTESIAN_POINT('Ctrl Pts',(18.3821808926254,2.7404994530043,1.6958620932737));
#68189=CARTESIAN_POINT('Ctrl Pts',(18.382982672336,2.73365829417609,1.70686783733203));
#68190=CARTESIAN_POINT('Ctrl Pts',(18.3865909356843,2.70266866321686,1.75605833624521));
#68191=CARTESIAN_POINT('Ctrl Pts',(18.3894246130884,2.67778617344998,1.79377246550688));
#68192=CARTESIAN_POINT('Ctrl Pts',(18.3970314882563,2.60959364588803,1.89254895481142));
#68193=CARTESIAN_POINT('Ctrl Pts',(18.4018541406598,2.56493699668418,1.95264367164623));
#68194=CARTESIAN_POINT('Ctrl Pts',(18.4267506066009,2.32723677743884,2.25028006525773));
#68195=CARTESIAN_POINT('Ctrl Pts',(18.4479831610657,2.10318708427647,2.46096588443852));
#68196=CARTESIAN_POINT('Ctrl Pts',(18.4697976226025,1.83186531289969,2.65161139403311));
#68197=CARTESIAN_POINT('Ctrl Pts',(18.4714725545752,1.81073557249715,2.66608516732623));
#68198=CARTESIAN_POINT('Ctrl Pts',(18.4731355395702,1.78943620771753,2.68030513580255));
#68199=CARTESIAN_POINT('Origin',(-1.72497344927317,0.,0.));
#68200=CARTESIAN_POINT('',(19.9669438677106,1.78943621037804,2.68030513402633));
#68201=CARTESIAN_POINT('',(19.7206814315572,1.78943602647606,2.6803052568037));
#68202=CARTESIAN_POINT('',(-1.72497344927317,1.78943621037804,2.68030513402633));
#68203=CARTESIAN_POINT('',(19.146573449238,-3.22274959114088,0.00162336111893835));
#68204=CARTESIAN_POINT('Ctrl Pts',(19.1465734492731,-3.22274959114116,0.00162336054795465));
#68205=CARTESIAN_POINT('Ctrl Pts',(19.1528129930212,-3.22280074318622,-0.0999253881336108));
#68206=CARTESIAN_POINT('Ctrl Pts',(19.1590525367692,-3.21804785151634,-0.201467213136769));
#68207=CARTESIAN_POINT('Ctrl Pts',(19.1652920805173,-3.2085193226538,-0.302524905846155));
#68208=CARTESIAN_POINT('Ctrl Pts',(19.1715337357476,-3.19898756930556,-0.403616796813063));
#68209=CARTESIAN_POINT('Ctrl Pts',(19.1777753909778,-3.18467700214314,-0.504223814665632));
#68210=CARTESIAN_POINT('Ctrl Pts',(19.1840170462081,-3.16566779601905,-0.603874960358412));
#68211=CARTESIAN_POINT('Ctrl Pts',(19.1902622883947,-3.14664766567892,-0.703583373600274));
#68212=CARTESIAN_POINT('Ctrl Pts',(19.1965075305812,-3.12292360146622,-0.802334412752572));
#68213=CARTESIAN_POINT('Ctrl Pts',(19.2027527727677,-3.09462648393053,-0.89966909886679));
#68214=CARTESIAN_POINT('Ctrl Pts',(19.2090073720642,-3.0662869694417,-0.997149619415189));
#68215=CARTESIAN_POINT('Ctrl Pts',(19.2152619713607,-3.03336083914884,-1.09320914994683));
#68216=CARTESIAN_POINT('Ctrl Pts',(19.2215165706571,-2.99602833737228,-1.18740547588526));
#68217=CARTESIAN_POINT('Ctrl Pts',(19.2277765972731,-2.95866344096807,-1.28168353904353));
#68218=CARTESIAN_POINT('Ctrl Pts',(19.2340366238891,-2.9168847279077,-1.37409479835277));
#68219=CARTESIAN_POINT('Ctrl Pts',(19.2402966505051,-2.87091904732102,-1.46422040220363));
#68220=CARTESIAN_POINT('Ctrl Pts',(19.2465677868719,-2.82487179084231,-1.55450595313753));
#68221=CARTESIAN_POINT('Ctrl Pts',(19.2528389232386,-2.77462293690911,-1.64249738896081));
#68222=CARTESIAN_POINT('Ctrl Pts',(19.2591100596054,-2.72044345063527,-1.7278035173004));
#68223=CARTESIAN_POINT('Ctrl Pts',(19.2610966965082,-2.70327989996263,-1.75482769484693));
#68224=CARTESIAN_POINT('Ctrl Pts',(19.263083333411,-2.68572219265785,-1.78158262996471));
#68225=CARTESIAN_POINT('Ctrl Pts',(19.2650699703137,-2.66777977423865,-1.80805659166497));
#68226=CARTESIAN_POINT('Ctrl Pts',(19.2712422184065,-2.6120347824327,-1.89030808884741));
#68227=CARTESIAN_POINT('Ctrl Pts',(19.2774144664993,-2.5523842109608,-1.97012389438097));
#68228=CARTESIAN_POINT('Ctrl Pts',(19.283586714592,-2.48906799086659,-2.04710969401822));
#68229=CARTESIAN_POINT('Ctrl Pts',(19.2897506032447,-2.42583752366879,-2.12399122724014));
#68230=CARTESIAN_POINT('Ctrl Pts',(19.2959144918973,-2.35895154903475,-2.1980500402326));
#68231=CARTESIAN_POINT('Ctrl Pts',(19.30207838055,-2.28869339035218,-2.26892047623054));
#68232=CARTESIAN_POINT('Ctrl Pts',(19.3082357422085,-2.21850962863106,-2.33971586692139));
#68233=CARTESIAN_POINT('Ctrl Pts',(19.314393103867,-2.14496108614528,-2.40732928604279));
#68234=CARTESIAN_POINT('Ctrl Pts',(19.3205504655256,-2.06837086215162,-2.47142864333611));
#68235=CARTESIAN_POINT('Ctrl Pts',(19.3267033296719,-1.99183658183785,-2.53548118063415));
#68236=CARTESIAN_POINT('Ctrl Pts',(19.3328561938182,-1.91226536930191,-2.59602448134056));
#68237=CARTESIAN_POINT('Ctrl Pts',(19.3390090579645,-1.83001595935445,-2.65276443564219));
#68238=CARTESIAN_POINT('Ctrl Pts',(19.345159591101,-1.74779770955839,-2.70948289403805));
#68239=CARTESIAN_POINT('Ctrl Pts',(19.3513101242376,-1.66290363557621,-2.76240062269866));
#68240=CARTESIAN_POINT('Ctrl Pts',(19.3574606573741,-1.57572350502502,-2.81126537313923));
#68241=CARTESIAN_POINT('Ctrl Pts',(19.3636105055893,-1.48855308282425,-2.8601246820174));
#68242=CARTESIAN_POINT('Ctrl Pts',(19.3697603538045,-1.39909748909988,-2.90493169761945));
#68243=CARTESIAN_POINT('Ctrl Pts',(19.3759102020197,-1.30777239521821,-2.94547940491955));
#68244=CARTESIAN_POINT('Ctrl Pts',(19.3820610103988,-1.21643304292602,-2.98603344285488));
#68245=CARTESIAN_POINT('Ctrl Pts',(19.388211818778,-1.12322400776556,-3.02232667534786));
#68246=CARTESIAN_POINT('Ctrl Pts',(19.3943626271571,-1.0285813655908,-3.05420004859855));
#68247=CARTESIAN_POINT('Ctrl Pts',(19.4005200135233,-0.933837507764791,
-3.08610750885438));
#68248=CARTESIAN_POINT('Ctrl Pts',(19.4066773998895,-0.837657393797968,
-3.1135855319858));
#68249=CARTESIAN_POINT('Ctrl Pts',(19.4128347862557,-0.740492593138584,
-3.13652487348768));
#68250=CARTESIAN_POINT('Ctrl Pts',(19.4189956089926,-0.643273565854203,
-3.1594770171881));
#68251=CARTESIAN_POINT('Ctrl Pts',(19.4251564317296,-0.545069184423238,
-3.17788535481417));
#68252=CARTESIAN_POINT('Ctrl Pts',(19.4313172544666,-0.446339479169904,
-3.19169212673064));
#68253=CARTESIAN_POINT('Ctrl Pts',(19.4374883773832,-0.347444709321798,
-3.20552198196541));
#68254=CARTESIAN_POINT('Ctrl Pts',(19.4436595002999,-0.248023294036869,
-3.21473486429637));
#68255=CARTESIAN_POINT('Ctrl Pts',(19.4498306232166,-0.148538773745802,
-3.21932505273918));
#68256=CARTESIAN_POINT('Ctrl Pts',(19.4545261451622,-0.0728423803045645,
-3.22281766354254));
#68257=CARTESIAN_POINT('Ctrl Pts',(19.4592216671079,0.00289047582658457,
-3.22363505479609));
#68258=CARTESIAN_POINT('Ctrl Pts',(19.4639171890535,0.0784574822998072,
-3.22179483921171));
#68259=CARTESIAN_POINT('Ctrl Pts',(19.4700894371462,0.177790062784492,-3.21937588190247));
#68260=CARTESIAN_POINT('Ctrl Pts',(19.476261685239,0.277185504657452,-3.21235451274927));
#68261=CARTESIAN_POINT('Ctrl Pts',(19.4824339333318,0.376182374086792,-3.20071935413376));
#68262=CARTESIAN_POINT('Ctrl Pts',(19.4885978219844,0.475045166208819,-3.18909995370077));
#68263=CARTESIAN_POINT('Ctrl Pts',(19.494761710637,0.573510031211977,-3.17287923409625));
#68264=CARTESIAN_POINT('Ctrl Pts',(19.5009255992897,0.671116179509239,-3.15209781512264));
#68265=CARTESIAN_POINT('Ctrl Pts',(19.5070829609482,0.768618971826402,-3.13133840177023));
#68266=CARTESIAN_POINT('Ctrl Pts',(19.5132403226067,0.865264432706953,-3.10602798023603));
#68267=CARTESIAN_POINT('Ctrl Pts',(19.5193976842653,0.960598501788612,-3.07625877989181));
#68268=CARTESIAN_POINT('Ctrl Pts',(19.5255505484116,1.05586293615248,-3.04651132381893));
#68269=CARTESIAN_POINT('Ctrl Pts',(19.5317034125579,1.14981746976196,-3.01231169313222));
#68270=CARTESIAN_POINT('Ctrl Pts',(19.5378562767042,1.24202072323521,-2.97380263056483));
#68271=CARTESIAN_POINT('Ctrl Pts',(19.5440068098408,1.33418904554799,-2.9353081571382));
#68272=CARTESIAN_POINT('Ctrl Pts',(19.5501573429773,1.42460700566302,-2.89250766306926));
#68273=CARTESIAN_POINT('Ctrl Pts',(19.5563078761138,1.5128516585648,-2.84559263101339));
#68274=CARTESIAN_POINT('Ctrl Pts',(19.562457724329,1.60108648457133,-2.79868282339992));
#68275=CARTESIAN_POINT('Ctrl Pts',(19.5686075725443,1.68714810099244,-2.7476595926638));
#68276=CARTESIAN_POINT('Ctrl Pts',(19.5747574207595,1.77063760717915,-2.69276067011959));
#68277=CARTESIAN_POINT('Ctrl Pts',(19.5809082291386,1.85414014842151,-2.63785317631243));
#68278=CARTESIAN_POINT('Ctrl Pts',(19.5870590375178,1.93506941881528,-2.57906902747991));
#68279=CARTESIAN_POINT('Ctrl Pts',(19.5932098458969,2.01305583020682,-2.5166890524994));
#68280=CARTESIAN_POINT('Ctrl Pts',(19.5993672322631,2.09112564422955,-2.45424236520383));
#68281=CARTESIAN_POINT('Ctrl Pts',(19.6055246186293,2.16624597466008,-2.38819244443255));
#68282=CARTESIAN_POINT('Ctrl Pts',(19.6116820049955,2.23808075582248,-2.31886008480828));
#68283=CARTESIAN_POINT('Ctrl Pts',(19.6178428277325,2.30995562719977,-2.24948903154353));
#68284=CARTESIAN_POINT('Ctrl Pts',(19.6240036504694,2.37854099947952,-2.17683220711775));
#68285=CARTESIAN_POINT('Ctrl Pts',(19.6301644732064,2.44353954163502,-2.10124536191424));
#68286=CARTESIAN_POINT('Ctrl Pts',(19.6363355961231,2.50864675380018,-2.02553214428875));
#68287=CARTESIAN_POINT('Ctrl Pts',(19.6425067190398,2.57015488978245,-1.946879463304));
#68288=CARTESIAN_POINT('Ctrl Pts',(19.6486778419564,2.62780849598165,-1.86567415990753));
#68289=CARTESIAN_POINT('Ctrl Pts',(19.653373363902,2.67167632632685,-1.80388616940059));
#68290=CARTESIAN_POINT('Ctrl Pts',(19.6580688858476,2.71331345388933,-1.74062098755121));
#68291=CARTESIAN_POINT('Ctrl Pts',(19.6627644077931,2.75262530228131,-1.67605832468346));
#68292=CARTESIAN_POINT('Ctrl Pts',(19.6689366558859,2.80430059718442,-1.59119091753042));
#68293=CARTESIAN_POINT('Ctrl Pts',(19.6751089039787,2.85213829201417,-1.50378205960815));
#68294=CARTESIAN_POINT('Ctrl Pts',(19.6812811520714,2.89587931381894,-1.41421376117458));
#68295=CARTESIAN_POINT('Ctrl Pts',(19.6874450407241,2.93956109457451,-1.32476677037754));
#68296=CARTESIAN_POINT('Ctrl Pts',(19.6936089293767,2.97915704135858,-1.23316653903017));
#68297=CARTESIAN_POINT('Ctrl Pts',(19.6997728180293,3.01445217026319,-1.13982265098371));
#68298=CARTESIAN_POINT('Ctrl Pts',(19.7059301796879,3.04970992485577,-1.04657760557381));
#68299=CARTESIAN_POINT('Ctrl Pts',(19.7120875413464,3.08067576291136,-0.951592978288173));
#68300=CARTESIAN_POINT('Ctrl Pts',(19.718244903005,3.10718175351252,-0.855300598116752));
#68301=CARTESIAN_POINT('Ctrl Pts',(19.7243977671513,3.13366838338359,-0.759078552640999));
#68302=CARTESIAN_POINT('Ctrl Pts',(19.7305506312976,3.15570152753199,-0.661551070956055));
#68303=CARTESIAN_POINT('Ctrl Pts',(19.7367034954439,3.17316260406615,-0.563166627789823));
#68304=CARTESIAN_POINT('Ctrl Pts',(19.7428540285804,3.19061706547943,-0.464819457524949));
#68305=CARTESIAN_POINT('Ctrl Pts',(19.749004561717,3.2035028251813,-0.365616398092275));
#68306=CARTESIAN_POINT('Ctrl Pts',(19.7551550948535,3.2117522693879,-0.266016771241406));
#68307=CARTESIAN_POINT('Ctrl Pts',(19.7613049430687,3.22000079493912,-0.166428235771939));
#68308=CARTESIAN_POINT('Ctrl Pts',(19.7674547912839,3.2236139956172,-0.0664436535774133));
#68309=CARTESIAN_POINT('Ctrl Pts',(19.7736046394991,3.22257616345777,0.0334728728044253));
#68310=CARTESIAN_POINT('Ctrl Pts',(19.7797554478783,3.22153816926361,0.13340499896078));
#68311=CARTESIAN_POINT('Ctrl Pts',(19.7859062562574,3.21584770440904,0.233268613806891));
#68312=CARTESIAN_POINT('Ctrl Pts',(19.7920570646366,3.20554116455006,0.33260096944389));
#68313=CARTESIAN_POINT('Ctrl Pts',(19.7982144510028,3.19522360235362,0.43203955614976));
#68314=CARTESIAN_POINT('Ctrl Pts',(19.804371837369,3.18028015205904,0.530945316200336));
#68315=CARTESIAN_POINT('Ctrl Pts',(19.8105292237351,3.16079895481053,0.628862091216109));
#68316=CARTESIAN_POINT('Ctrl Pts',(19.8166900464721,3.14130688531643,0.726833512525474));
#68317=CARTESIAN_POINT('Ctrl Pts',(19.8228508692091,3.11727212998798,0.823814427981407));
#68318=CARTESIAN_POINT('Ctrl Pts',(19.829011691946,3.08883317928826,0.919362362198937));
#68319=CARTESIAN_POINT('Ctrl Pts',(19.8351828148627,3.06034668196753,1.01507004145994));
#68320=CARTESIAN_POINT('Ctrl Pts',(19.8413539377794,3.02744142452246,1.10933954368935));
#68321=CARTESIAN_POINT('Ctrl Pts',(19.8475250606961,2.99030469462921,1.20174681018029));
#68322=CARTESIAN_POINT('Ctrl Pts',(19.8522205826417,2.96204787126753,1.27205821923747));
#68323=CARTESIAN_POINT('Ctrl Pts',(19.8569161045872,2.93134225754545,1.34129187371315));
#68324=CARTESIAN_POINT('Ctrl Pts',(19.8616116265328,2.8982878889683,1.40927104389456));
#68325=CARTESIAN_POINT('Ctrl Pts',(19.8677836353661,2.85483971489893,1.49862597476367));
#68326=CARTESIAN_POINT('Ctrl Pts',(19.8739556441994,2.80717894706068,1.58612701454832));
#68327=CARTESIAN_POINT('Ctrl Pts',(19.8801276530327,2.75548683046381,1.67134972092632));
#68328=CARTESIAN_POINT('Ctrl Pts',(19.8862916465573,2.70386184408032,1.75646175243086));
#68329=CARTESIAN_POINT('Ctrl Pts',(19.892455640082,2.6482161353862,1.83930096185228));
#68330=CARTESIAN_POINT('Ctrl Pts',(19.8986196336066,2.58877801620846,1.91946501538731));
#68331=CARTESIAN_POINT('Ctrl Pts',(19.9047764049644,2.5294095388971,1.99953514309861));
#68332=CARTESIAN_POINT('Ctrl Pts',(19.9109331763222,2.46625774731003,2.07693600293512));
#68333=CARTESIAN_POINT('Ctrl Pts',(19.91708994768,2.39959501652406,2.15129294127343));
#68334=CARTESIAN_POINT('Ctrl Pts',(19.9232424841021,2.33297813970292,2.22559873318562));
#68335=CARTESIAN_POINT('Ctrl Pts',(19.9293950205242,2.26285541225963,2.29686444243887));
#68336=CARTESIAN_POINT('Ctrl Pts',(19.9355475569464,2.18953992099314,2.36474787173545));
#68337=CARTESIAN_POINT('Ctrl Pts',(19.941698105571,2.11624811692488,2.43260936885619));
#68338=CARTESIAN_POINT('Ctrl Pts',(19.9478486541956,2.03976591450839,2.49709045991259));
#68339=CARTESIAN_POINT('Ctrl Pts',(19.9539992028202,1.96044313657274,2.55788589869932));
#68340=CARTESIAN_POINT('Ctrl Pts',(19.958314091117,1.904794616892,2.60053665123055));
#68341=CARTESIAN_POINT('Ctrl Pts',(19.9626289794138,1.84774884604552,2.64137421513157));
#68342=CARTESIAN_POINT('Ctrl Pts',(19.9669438677106,1.78943621037804,2.68030513402633));
#68343=CARTESIAN_POINT('Ctrl Pts',(18.7170794495574,1.78943621037806,2.68030513402632));
#68344=CARTESIAN_POINT('Ctrl Pts',(18.7233417863607,1.70500923028825,2.73667061771235));
#68345=CARTESIAN_POINT('Ctrl Pts',(18.7296041231639,1.61783995710172,2.78909426977908));
#68346=CARTESIAN_POINT('Ctrl Pts',(18.7358664599671,1.52833574574161,2.83730636533816));
#68347=CARTESIAN_POINT('Ctrl Pts',(18.7420176376459,1.44042027195277,2.88466267582925));
#68348=CARTESIAN_POINT('Ctrl Pts',(18.7481688153247,1.35025247487346,2.92795551133685));
#68349=CARTESIAN_POINT('Ctrl Pts',(18.7543199930036,1.25824587160605,2.96697402905491));
#68350=CARTESIAN_POINT('Ctrl Pts',(18.7604698971959,1.16625831658886,3.00598446871703));
#68351=CARTESIAN_POINT('Ctrl Pts',(18.7666198013881,1.07243311178441,3.04072217979505));
#68352=CARTESIAN_POINT('Ctrl Pts',(18.7727697055804,0.977204988616989,3.07102392903769));
#68353=CARTESIAN_POINT('Ctrl Pts',(18.7789199815786,0.881971108225357,3.10132751023877));
#68354=CARTESIAN_POINT('Ctrl Pts',(18.7850702575768,0.785334555129725,3.12719446558737));
#68355=CARTESIAN_POINT('Ctrl Pts',(18.7912205335749,0.68774553153598,3.14851133813304));
#68356=CARTESIAN_POINT('Ctrl Pts',(18.7975667835132,0.587046906767896,3.17050745686296));
#68357=CARTESIAN_POINT('Ctrl Pts',(18.8039130334515,0.485334571628309,3.18765853116547));
#68358=CARTESIAN_POINT('Ctrl Pts',(18.8102592833898,0.383113188613054,3.19989716197423));
#68359=CARTESIAN_POINT('Ctrl Pts',(18.8164188211197,0.283899247844779,3.21177572158992));
#68360=CARTESIAN_POINT('Ctrl Pts',(18.8225783588495,0.184206240647182,3.21902689963705));
#68361=CARTESIAN_POINT('Ctrl Pts',(18.8287378965794,0.0844980762081079,
3.22164207161769));
#68362=CARTESIAN_POINT('Ctrl Pts',(18.8351775026219,-0.0197437234809175,
3.22437615297694));
#68363=CARTESIAN_POINT('Ctrl Pts',(18.8416171086644,-0.124001549914439,
3.22204267337145));
#68364=CARTESIAN_POINT('Ctrl Pts',(18.8480567147069,-0.227750211563248,
3.2146924275322));
#68365=CARTESIAN_POINT('Ctrl Pts',(18.8544963207495,-0.331498873212073,
3.20734218169296));
#68366=CARTESIAN_POINT('Ctrl Pts',(18.860935926792,-0.434737848062131,3.1949753062194));
#68367=CARTESIAN_POINT('Ctrl Pts',(18.8673755328345,-0.536954836311479,
3.17770311172421));
#68368=CARTESIAN_POINT('Ctrl Pts',(18.8735477809273,-0.634928005260677,
3.16114801987125));
#68369=CARTESIAN_POINT('Ctrl Pts',(18.8797200290201,-0.732307274235706,
3.14002856287555));
#68370=CARTESIAN_POINT('Ctrl Pts',(18.8858922771128,-0.828634300415547,
3.11439926128216));
#68371=CARTESIAN_POINT('Ctrl Pts',(18.8920561657655,-0.924830865214518,
3.08880467096564));
#68372=CARTESIAN_POINT('Ctrl Pts',(18.8982200544181,-1.01997760371505,3.05871248697548));
#68373=CARTESIAN_POINT('Ctrl Pts',(18.9043839430707,-1.11362422350716,3.02422860434162));
#68374=CARTESIAN_POINT('Ctrl Pts',(18.9105413047293,-1.20717168009763,2.98978123698418));
#68375=CARTESIAN_POINT('Ctrl Pts',(18.9166986663878,-1.29922177067461,2.95095156570248));
#68376=CARTESIAN_POINT('Ctrl Pts',(18.9228560280464,-1.3893382207761,2.90789560864738));
#68377=CARTESIAN_POINT('Ctrl Pts',(18.9290088921927,-1.47938884725696,2.86487110088904));
#68378=CARTESIAN_POINT('Ctrl Pts',(18.935161756339,-1.56750825057104,2.81762663153629));
#68379=CARTESIAN_POINT('Ctrl Pts',(18.9413146204853,-1.6532799088945,2.76636640836781));
#68380=CARTESIAN_POINT('Ctrl Pts',(18.9474651536218,-1.73901907266471,2.71512560511125));
#68381=CARTESIAN_POINT('Ctrl Pts',(18.9536156867584,-1.82241188631285,2.65987229357431));
#68382=CARTESIAN_POINT('Ctrl Pts',(18.9597662198949,-1.9030670224539,2.60085629563582));
#68383=CARTESIAN_POINT('Ctrl Pts',(18.9659160681101,-1.9837131768653,2.5418468696996));
#68384=CARTESIAN_POINT('Ctrl Pts',(18.9720659163253,-2.06162190933523,2.47907584692133));
#68385=CARTESIAN_POINT('Ctrl Pts',(18.9782157645405,-2.13643228446384,2.41283539770134));
#68386=CARTESIAN_POINT('Ctrl Pts',(18.9843665729197,-2.21125433959241,2.34658460648745));
#68387=CARTESIAN_POINT('Ctrl Pts',(18.9905173812988,-2.28297675130363,2.27686360090969));
#68388=CARTESIAN_POINT('Ctrl Pts',(18.996668189678,-2.35127374128403,2.2040030299544));
#68389=CARTESIAN_POINT('Ctrl Pts',(19.0028255760442,-2.41964377153594,2.13106453820222));
#68390=CARTESIAN_POINT('Ctrl Pts',(19.0089829624104,-2.48458076714167,2.05498009380272));
#68391=CARTESIAN_POINT('Ctrl Pts',(19.0151403487766,-2.54579782738497,1.97611512432397));
#68392=CARTESIAN_POINT('Ctrl Pts',(19.0213011715135,-2.607049052208,1.89720614115809));
#68393=CARTESIAN_POINT('Ctrl Pts',(19.0274619942505,-2.66457595712857,1.81551389772774));
#68394=CARTESIAN_POINT('Ctrl Pts',(19.0336228169875,-2.71813496374011,1.73143289832253));
#68395=CARTESIAN_POINT('Ctrl Pts',(19.0397939399042,-2.77178351478708,1.64721132525664));
#68396=CARTESIAN_POINT('Ctrl Pts',(19.0459650628209,-2.8214507004121,1.56059339587594));
#68397=CARTESIAN_POINT('Ctrl Pts',(19.0521361857376,-2.86693882417383,1.47199841743963));
#68398=CARTESIAN_POINT('Ctrl Pts',(19.0568317076831,-2.90155010744723,1.40458772555615));
#68399=CARTESIAN_POINT('Ctrl Pts',(19.0615272296287,-2.93374288370895,1.33603293883333));
#68400=CARTESIAN_POINT('Ctrl Pts',(19.0662227515742,-2.96344916204088,1.26652541486509));
#68401=CARTESIAN_POINT('Ctrl Pts',(19.0730622090646,-3.00671907541927,1.16528134424656));
#68402=CARTESIAN_POINT('Ctrl Pts',(19.079901666555,-3.04484207353096,1.06171188840576));
#68403=CARTESIAN_POINT('Ctrl Pts',(19.0867411240455,-3.07758863484432,0.956329314188925));
#68404=CARTESIAN_POINT('Ctrl Pts',(19.093561136033,-3.11024209325389,0.851246356886852));
#68405=CARTESIAN_POINT('Ctrl Pts',(19.1003811480205,-3.13754949825345,0.744360810177043));
#68406=CARTESIAN_POINT('Ctrl Pts',(19.107201160008,-3.15932940831118,0.63620378203852));
#68407=CARTESIAN_POINT('Ctrl Pts',(19.1139862885523,-3.18099791706078,0.528599962539821));
#68408=CARTESIAN_POINT('Ctrl Pts',(19.1207714170965,-3.197195216958,0.419737885761649));
#68409=CARTESIAN_POINT('Ctrl Pts',(19.1275565456408,-3.20779026533691,0.310159920218187));
#68410=CARTESIAN_POINT('Ctrl Pts',(19.1338955135065,-3.21768862920311,0.207787327297706));
#68411=CARTESIAN_POINT('Ctrl Pts',(19.1402344813723,-3.22269762399439,0.104790240090867));
#68412=CARTESIAN_POINT('Ctrl Pts',(19.146573449238,-3.22274959114088,0.00162336111892945));
#68413=CARTESIAN_POINT('',(18.9023069674493,-3.22275003535735,0.00201018136784693));
#68414=CARTESIAN_POINT('Ctrl Pts',(18.4731355395702,1.78943620771753,2.68030513580255));
#68415=CARTESIAN_POINT('Ctrl Pts',(18.476024270916,1.75243759205303,2.70500630195752));
#68416=CARTESIAN_POINT('Ctrl Pts',(18.4788769810994,1.71492714727499,2.72894162742002));
#68417=CARTESIAN_POINT('Ctrl Pts',(18.4823483894815,1.66791014521011,2.75759040523856));
#68418=CARTESIAN_POINT('Ctrl Pts',(18.4830115716966,1.65886444919064,2.76304141157852));
#68419=CARTESIAN_POINT('Ctrl Pts',(18.4839936041243,1.64537225142197,2.77108177211625));
#68420=CARTESIAN_POINT('Ctrl Pts',(18.4843146191607,1.64094619178575,2.77370503659756));
#68421=CARTESIAN_POINT('Ctrl Pts',(18.4848856768894,1.63304435144863,2.77836281440048));
#68422=CARTESIAN_POINT('Ctrl Pts',(18.4851359852072,1.6295710310706,2.78040141662612));
#68423=CARTESIAN_POINT('Ctrl Pts',(18.4856654291219,1.62220359998114,2.78470704841974));
#68424=CARTESIAN_POINT('Ctrl Pts',(18.4859444562345,1.6183085690645,2.78697241486077));
#68425=CARTESIAN_POINT('Ctrl Pts',(18.4866981320776,1.60775503423643,2.79308081090891));
#68426=CARTESIAN_POINT('Ctrl Pts',(18.4871717751755,1.60108745759378,2.7969082255881));
#68427=CARTESIAN_POINT('Ctrl Pts',(18.4882198329573,1.58625721943527,2.80535087337655));
#68428=CARTESIAN_POINT('Ctrl Pts',(18.488793523456,1.57808794804422,2.80995443417332));
#68429=CARTESIAN_POINT('Ctrl Pts',(18.4905286388476,1.5532285548915,2.82382063293728));
#68430=CARTESIAN_POINT('Ctrl Pts',(18.4916834377403,1.5364758044674,2.83297088783571));
#68431=CARTESIAN_POINT('Ctrl Pts',(18.50896109981,1.28289343695959,2.96856493832906));
#68432=CARTESIAN_POINT('Ctrl Pts',(18.5235323797865,1.03121843864519,3.06509810180271));
#68433=CARTESIAN_POINT('Ctrl Pts',(18.5494369907781,0.584023003599997,3.17520044154092));
#68434=CARTESIAN_POINT('Ctrl Pts',(18.5604454691664,0.393891621412011,3.20434308689518));
#68435=CARTESIAN_POINT('Ctrl Pts',(18.5731190962936,0.18441182878952,3.21751947184798));
#68436=CARTESIAN_POINT('Ctrl Pts',(18.5742066736896,0.166502078349412,3.21849597050111));
#68437=CARTESIAN_POINT('Ctrl Pts',(18.575857162619,0.139428459714096,3.2197455326491));
#68438=CARTESIAN_POINT('Ctrl Pts',(18.5764166098233,0.130269848601947,3.22012908968073));
#68439=CARTESIAN_POINT('Ctrl Pts',(18.5773910529248,0.114349790326214,3.22072778270735));
#68440=CARTESIAN_POINT('Ctrl Pts',(18.5778054880914,0.107589038748581,3.22096071421027));
#68441=CARTESIAN_POINT('Ctrl Pts',(18.5786710524421,0.0934903612106258,
3.22140202448157));
#68442=CARTESIAN_POINT('Ctrl Pts',(18.5791222978726,0.0861523635538499,
3.22160662089677));
#68443=CARTESIAN_POINT('Ctrl Pts',(18.5801908023742,0.0688056796694947,
3.22203096864952));
#68444=CARTESIAN_POINT('Ctrl Pts',(18.5808087346269,0.0587965857734008,
3.22222915733301));
#68445=CARTESIAN_POINT('Ctrl Pts',(18.5828574924463,0.0256879690323781,
3.22273042155132));
#68446=CARTESIAN_POINT('Ctrl Pts',(18.5842946255916,0.00258652631420823,
3.22283175279419));
#68447=CARTESIAN_POINT('Ctrl Pts',(18.6010332299844,-0.26501048133997,3.22112840264514));
#68448=CARTESIAN_POINT('Ctrl Pts',(18.61724099708,-0.508485757515415,3.19175419317788));
#68449=CARTESIAN_POINT('Ctrl Pts',(18.6418861061547,-0.863162548035848,
3.10733177933052));
#68450=CARTESIAN_POINT('Ctrl Pts',(18.6500494271499,-0.978428136077582,
3.07298548146399));
#68451=CARTESIAN_POINT('Ctrl Pts',(18.6656380460207,-1.19776200678344,2.99403350077649));
#68452=CARTESIAN_POINT('Ctrl Pts',(18.673066719152,-1.30194566601167,2.95022268005662));
#68453=CARTESIAN_POINT('Ctrl Pts',(18.6809368654072,-1.41415793606447,2.89593021724134));
#68454=CARTESIAN_POINT('Ctrl Pts',(18.6816723772746,-1.42466378610514,2.89077629673106));
#68455=CARTESIAN_POINT('Ctrl Pts',(18.6827364387447,-1.4398938282097,2.88320160531408));
#68456=CARTESIAN_POINT('Ctrl Pts',(18.6830677469511,-1.44464033144697,2.88082627853905));
#68457=CARTESIAN_POINT('Ctrl Pts',(18.6836511155358,-1.45300627108334,2.87661377553958));
#68458=CARTESIAN_POINT('Ctrl Pts',(18.683903480282,-1.45662813050576,2.87478147475325));
#68459=CARTESIAN_POINT('Ctrl Pts',(18.6841558598204,-1.46025304276704,2.87293902017468));
#68460=CARTESIAN_POINT('Ctrl Pts',(18.6841563102148,-1.46025951176447,2.87293573211349));
#68461=CARTESIAN_POINT('Ctrl Pts',(18.6841572108481,-1.46027244754318,2.87292915706233));
#68462=CARTESIAN_POINT('Ctrl Pts',(18.6841576602452,-1.46027890223328,2.87292587621836));
#68463=CARTESIAN_POINT('Ctrl Pts',(18.684158557766,-1.46029179334282,2.8729193237625));
#68464=CARTESIAN_POINT('Ctrl Pts',(18.6841590058816,-1.46029822964437,2.87291605221069));
#68465=CARTESIAN_POINT('Ctrl Pts',(18.684159900896,-1.46031108479031,2.87290951792614));
#68466=CARTESIAN_POINT('Ctrl Pts',(18.6841603477541,-1.46031750304842,2.87290625549155));
#68467=CARTESIAN_POINT('Ctrl Pts',(18.6841612402268,-1.46033032172228,2.87289973963768));
#68468=CARTESIAN_POINT('Ctrl Pts',(18.6841616858266,-1.46033672192511,2.87289648632678));
#68469=CARTESIAN_POINT('Ctrl Pts',(18.6841625757727,-1.46034950434424,2.87288998879404));
#68470=CARTESIAN_POINT('Ctrl Pts',(18.6841630201143,-1.46035588649246,2.87288674460695));
#68471=CARTESIAN_POINT('Ctrl Pts',(18.6841639075422,-1.4603686327767,2.87288026533531));
#68472=CARTESIAN_POINT('Ctrl Pts',(18.6841643506206,-1.4603749967993,2.87287703030858));
#68473=CARTESIAN_POINT('Ctrl Pts',(18.6841652355712,-1.46038770753736,2.8728705689997));
#68474=CARTESIAN_POINT('Ctrl Pts',(18.6841656774042,-1.46039405368954,2.87286734300405));
#68475=CARTESIAN_POINT('Ctrl Pts',(18.6841665598646,-1.46040672869427,2.87286089975396));
#68476=CARTESIAN_POINT('Ctrl Pts',(18.6841670004615,-1.46041305710831,2.87285768272259));
#68477=CARTESIAN_POINT('Ctrl Pts',(18.6841678804205,-1.46042569621865,2.87285125761405));
#68478=CARTESIAN_POINT('Ctrl Pts',(18.6841683197752,-1.46043200680808,2.87284804959136));
#68479=CARTESIAN_POINT('Ctrl Pts',(18.6841691972552,-1.46044461034698,2.87284164246109));
#68480=CARTESIAN_POINT('Ctrl Pts',(18.684169635365,-1.4604509030723,2.87283844346761));
#68481=CARTESIAN_POINT('Ctrl Pts',(18.6841705104098,-1.46046347166695,2.87283205399764));
#68482=CARTESIAN_POINT('Ctrl Pts',(18.6841709472997,-1.46046974688777,2.87282886385099));
#68483=CARTESIAN_POINT('Ctrl Pts',(18.6841718198684,-1.46048227995116,2.87282249234063));
#68484=CARTESIAN_POINT('Ctrl Pts',(18.6841722555346,-1.46048853761152,2.87281931106969));
#68485=CARTESIAN_POINT('Ctrl Pts',(18.684173125644,-1.46050103538487,2.87281295739716));
#68486=CARTESIAN_POINT('Ctrl Pts',(18.6841735600824,-1.46050727542684,2.87280978503182));
#68487=CARTESIAN_POINT('Ctrl Pts',(18.6841744277575,-1.46051973826814,2.87280344901599));
#68488=CARTESIAN_POINT('Ctrl Pts',(18.684174860972,-1.46052596074721,2.87280028552847));
#68489=CARTESIAN_POINT('Ctrl Pts',(18.6841757262361,-1.46053838899034,2.87279396700046));
#68490=CARTESIAN_POINT('Ctrl Pts',(18.6841761582447,-1.46054459416561,2.87279081225946));
#68491=CARTESIAN_POINT('Ctrl Pts',(18.6841770210724,-1.46055698744658,2.87278451140517));
#68492=CARTESIAN_POINT('Ctrl Pts',(18.6841774518729,-1.46056317528688,2.87278136542696));
#68493=CARTESIAN_POINT('Ctrl Pts',(18.6841783122832,-1.46057553387815,2.87277508210872));
#68494=CARTESIAN_POINT('Ctrl Pts',(18.6841787418776,-1.46058170440909,2.8727719448807));
#68495=CARTESIAN_POINT('Ctrl Pts',(18.6841795998783,-1.46059402842215,2.87276567904267));
#68496=CARTESIAN_POINT('Ctrl Pts',(18.684180028265,-1.46060018162263,2.87276255057599));
#68497=CARTESIAN_POINT('Ctrl Pts',(18.6841808838898,-1.46061247154269,2.87275630197232));
#68498=CARTESIAN_POINT('Ctrl Pts',(18.6841813110869,-1.46061860767264,2.87275318213524));
#68499=CARTESIAN_POINT('Ctrl Pts',(18.6841821643033,-1.46063086303052,2.87274695100528));
#68500=CARTESIAN_POINT('Ctrl Pts',(18.6841825903017,-1.46063698195809,2.87274383986526));
#68501=CARTESIAN_POINT('Ctrl Pts',(18.6841834411658,-1.46064920356114,2.87273762579936));
#68502=CARTESIAN_POINT('Ctrl Pts',(18.6841838659907,-1.46065530564827,2.87273452317278));
#68503=CARTESIAN_POINT('Ctrl Pts',(18.6841847144447,-1.4606674926646,2.87272832659474));
#68504=CARTESIAN_POINT('Ctrl Pts',(18.6841851380758,-1.46067357762199,2.8727252326291));
#68505=CARTESIAN_POINT('Ctrl Pts',(18.6841859841906,-1.46068573106895,2.87271905302245));
#68506=CARTESIAN_POINT('Ctrl Pts',(18.6841864066461,-1.46069179915524,2.87271596758665));
#68507=CARTESIAN_POINT('Ctrl Pts',(18.6841872503922,-1.46070391861135,2.87270980516652));
#68508=CARTESIAN_POINT('Ctrl Pts',(18.6841876716662,-1.4607099697425,2.87270672830369));
#68509=CARTESIAN_POINT('Ctrl Pts',(18.6841885130783,-1.46072205570476,2.87270058281817));
#68510=CARTESIAN_POINT('Ctrl Pts',(18.6841889331813,-1.46072809003067,2.87269751445249));
#68511=CARTESIAN_POINT('Ctrl Pts',(18.6841897722531,-1.46074014240808,2.87269138594864));
#68512=CARTESIAN_POINT('Ctrl Pts',(18.6841901911871,-1.46074615995923,2.87268832606503));
#68513=CARTESIAN_POINT('Ctrl Pts',(18.6841910279453,-1.46075817913488,2.87268221434885));
#68514=CARTESIAN_POINT('Ctrl Pts',(18.684191445729,-1.46076418017749,2.87267916281231));
#68515=CARTESIAN_POINT('Ctrl Pts',(18.6841922801366,-1.46077616561937,2.87267306815513));
#68516=CARTESIAN_POINT('Ctrl Pts',(18.6841926967576,-1.46078214997686,2.87267002505586));
#68517=CARTESIAN_POINT('Ctrl Pts',(18.6841935288435,-1.46079410210191,2.87266394724643));
#68518=CARTESIAN_POINT('Ctrl Pts',(18.684193944294,-1.4608000696619,2.87266091264197));
#68519=CARTESIAN_POINT('Ctrl Pts',(18.6841947741202,-1.46081198935764,2.87265485122977));
#68520=CARTESIAN_POINT('Ctrl Pts',(18.6841951884342,-1.46081794060716,2.87265182487283));
#68521=CARTESIAN_POINT('Ctrl Pts',(18.6844709114871,-1.46477846073263,2.87063778736576));
#68522=CARTESIAN_POINT('Ctrl Pts',(18.68474569995,-1.46872890091856,2.86861859811481));
#68523=CARTESIAN_POINT('Ctrl Pts',(18.6854750564779,-1.47922277631883,2.86322750164909));
#68524=CARTESIAN_POINT('Ctrl Pts',(18.6859287292191,-1.48575889714807,2.85984129808454));
#68525=CARTESIAN_POINT('Ctrl Pts',(18.6869281793814,-1.50017565401075,2.8523095654072));
#68526=CARTESIAN_POINT('Ctrl Pts',(18.6874733243851,-1.50805085773481,2.8481536939787));
#68527=CARTESIAN_POINT('Ctrl Pts',(18.6891006642262,-1.5315901730399,2.83560661484554));
#68528=CARTESIAN_POINT('Ctrl Pts',(18.6901771619395,-1.54720249322364,2.82711828696506));
#68529=CARTESIAN_POINT('Ctrl Pts',(18.694036143216,-1.60327516571804,2.79602827086923));
#68530=CARTESIAN_POINT('Ctrl Pts',(18.696778131406,-1.64331885159899,2.77268262778019));
#68531=CARTESIAN_POINT('Ctrl Pts',(18.7062765686993,-1.78202583038118,2.68775473309759));
#68532=CARTESIAN_POINT('Ctrl Pts',(18.7128414671115,-1.87785225682153,2.62170102572494));
#68533=CARTESIAN_POINT('Ctrl Pts',(18.7351687553292,-2.19314880293415,2.37818887708171));
#68534=CARTESIAN_POINT('Ctrl Pts',(18.7507272520347,-2.39276519082314,2.17723264891625));
#68535=CARTESIAN_POINT('Ctrl Pts',(18.7682333897745,-2.56995237866755,1.9446258434106));
#68536=CARTESIAN_POINT('Ctrl Pts',(18.7688551435811,-2.57619053772006,1.93635410220001));
#68537=CARTESIAN_POINT('Ctrl Pts',(18.7709658706776,-2.59718065100408,1.90824043289281));
#68538=CARTESIAN_POINT('Ctrl Pts',(18.772461901902,-2.61174383850366,1.88825923894307));
#68539=CARTESIAN_POINT('Ctrl Pts',(18.7745469773166,-2.63160009617297,1.86034656300099));
#68540=CARTESIAN_POINT('Ctrl Pts',(18.7751284311644,-2.63709029435138,1.85255584990574));
#68541=CARTESIAN_POINT('Ctrl Pts',(18.7761306277284,-2.64647206549712,1.83911669475803));
#68542=CARTESIAN_POINT('Ctrl Pts',(18.7765507291151,-2.65038033389599,1.83347994124274));
#68543=CARTESIAN_POINT('Ctrl Pts',(18.7774181756086,-2.65839992538469,1.82183435255886));
#68544=CARTESIAN_POINT('Ctrl Pts',(18.7778656053226,-2.66250893744366,1.81582398048249));
#68545=CARTESIAN_POINT('Ctrl Pts',(18.7789078034674,-2.67201597139271,1.80181611425027));
#68546=CARTESIAN_POINT('Ctrl Pts',(18.7795031540309,-2.67739849299595,1.79380823038807));
#68547=CARTESIAN_POINT('Ctrl Pts',(18.7814047516953,-2.69443632822417,1.76821254724416));
#68548=CARTESIAN_POINT('Ctrl Pts',(18.7827161232096,-2.70595473348776,1.7505346855386));
#68549=CARTESIAN_POINT('Ctrl Pts',(18.796955438228,-2.82851975276614,1.55832770704123));
#68550=CARTESIAN_POINT('Ctrl Pts',(18.810518611536,-2.92266862332685,1.37364057529463));
#68551=CARTESIAN_POINT('Ctrl Pts',(18.8362270285434,-3.06282551573948,1.01786593336279));
#68552=CARTESIAN_POINT('Ctrl Pts',(18.8482228433012,-3.11372614614363,0.84950627088044));
#68553=CARTESIAN_POINT('Ctrl Pts',(18.8618745076466,-3.15686347303331,0.648999801147239));
#68554=CARTESIAN_POINT('Ctrl Pts',(18.8638281707892,-3.16267180529422,0.620076502959375));
#68555=CARTESIAN_POINT('Ctrl Pts',(18.8703929424111,-3.1809727708513,0.521986097404746));
#68556=CARTESIAN_POINT('Ctrl Pts',(18.874942651001,-3.1916007672669,0.452485929125252));
#68557=CARTESIAN_POINT('Ctrl Pts',(18.8800411533158,-3.2012029426253,0.372194797411296));
#68558=CARTESIAN_POINT('Ctrl Pts',(18.8807047899899,-3.2024062579273,0.361695194360419));
#68559=CARTESIAN_POINT('Ctrl Pts',(18.8816873632619,-3.20411873890622,0.346073915746262));
#68560=CARTESIAN_POINT('Ctrl Pts',(18.8820084681183,-3.20466730495548,0.34095676206605));
#68561=CARTESIAN_POINT('Ctrl Pts',(18.8825796246021,-3.20562331706386,0.331832687463649));
#68562=CARTESIAN_POINT('Ctrl Pts',(18.8828299422166,-3.20603551076065,0.32782630729504));
#68563=CARTESIAN_POINT('Ctrl Pts',(18.8833145048134,-3.20682024522696,0.320055906575915));
#68564=CARTESIAN_POINT('Ctrl Pts',(18.8835487997507,-3.20719366770239,0.316292027614158));
#68565=CARTESIAN_POINT('Ctrl Pts',(18.8840630801918,-3.20800007045058,0.308015681483374));
#68566=CARTESIAN_POINT('Ctrl Pts',(18.8843429031406,-3.20843015872852,0.303502931127059));
#68567=CARTESIAN_POINT('Ctrl Pts',(18.8850316171246,-3.2094672166819,0.29237288514179));
#68568=CARTESIAN_POINT('Ctrl Pts',(18.885439906633,-3.21006324774873,0.2857545558346));
#68569=CARTESIAN_POINT('Ctrl Pts',(18.8874029618911,-3.21283794034375,0.253839690028737));
#68570=CARTESIAN_POINT('Ctrl Pts',(18.8889428689628,-3.21473815024191,0.228519006920698));
#68571=CARTESIAN_POINT('Ctrl Pts',(18.8945016334168,-3.22056952438101,0.136207284159294));
#68572=CARTESIAN_POINT('Ctrl Pts',(18.8984358349785,-3.22270761219489,0.0691171422643548));
#68573=CARTESIAN_POINT('Ctrl Pts',(18.9023083833077,-3.22274937597677,0.00200552769956143));
#68574=CARTESIAN_POINT('Ctrl Pts',(18.9023081109937,-3.22274937303652,0.0020102469239669));
#68575=CARTESIAN_POINT('Ctrl Pts',(18.9195468469855,-3.22293572278098,-0.29673838686921));
#68576=CARTESIAN_POINT('Ctrl Pts',(18.9355977504742,-3.18158379616016,-0.594088851345514));
#68577=CARTESIAN_POINT('Ctrl Pts',(18.9567435757215,-3.08170305669619,-0.945316117520925));
#68578=CARTESIAN_POINT('Ctrl Pts',(18.9606333022897,-3.061597713524,-1.00853105112119));
#68579=CARTESIAN_POINT('Ctrl Pts',(18.9670453919786,-3.02582990050013,-1.11003470961203));
#68580=CARTESIAN_POINT('Ctrl Pts',(18.9695294300397,-3.01135515118264,-1.14872257692395));
#68581=CARTESIAN_POINT('Ctrl Pts',(18.9728006031635,-2.99151929683866,-1.19878576325663));
#68582=CARTESIAN_POINT('Ctrl Pts',(18.9735650997096,-2.98682920126305,-1.2104240269658));
#68583=CARTESIAN_POINT('Ctrl Pts',(18.9748127150365,-2.97908784689376,-1.22931487759577));
#68584=CARTESIAN_POINT('Ctrl Pts',(18.9752944357453,-2.97607775321187,-1.2365842765004));
#68585=CARTESIAN_POINT('Ctrl Pts',(18.9762223411069,-2.97023941000974,-1.25053912515274));
#68586=CARTESIAN_POINT('Ctrl Pts',(18.9766683883441,-2.96741513051169,-1.25722619211876));
#68587=CARTESIAN_POINT('Ctrl Pts',(18.9776904036008,-2.96090354187435,-1.27249954762327));
#68588=CARTESIAN_POINT('Ctrl Pts',(18.9782668740921,-2.95720144507192,-1.28107942505656));
#68589=CARTESIAN_POINT('Ctrl Pts',(18.9797972805776,-2.9472963411418,-1.30376349268296));
#68590=CARTESIAN_POINT('Ctrl Pts',(18.9807533998814,-2.94102946844005,-1.31783937558592));
#68591=CARTESIAN_POINT('Ctrl Pts',(18.9873378469139,-2.89733798955403,-1.41410985412766));
#68592=CARTESIAN_POINT('Ctrl Pts',(18.9930810500932,-2.85657687981357,-1.49473743890401));
#68593=CARTESIAN_POINT('Ctrl Pts',(19.0016449537475,-2.79205539432489,-1.6100606741569));
#68594=CARTESIAN_POINT('Ctrl Pts',(19.0043791285299,-2.7709147162206,-1.64617742202777));
#68595=CARTESIAN_POINT('Ctrl Pts',(19.0200950127406,-2.64629319190259,-1.8498756819759));
#68596=CARTESIAN_POINT('Ctrl Pts',(19.0334970490938,-2.52833077215714,-2.008093287704));
#68597=CARTESIAN_POINT('Ctrl Pts',(19.0536628440086,-2.32858226792262,-2.23029106093209));
#68598=CARTESIAN_POINT('Ctrl Pts',(19.0604898934677,-2.2569249137759,-2.30277794456624));
#68599=CARTESIAN_POINT('Ctrl Pts',(19.0697388502625,-2.15282297989842,-2.39854897784718));
#68600=CARTESIAN_POINT('Ctrl Pts',(19.072300640028,-2.12320330959228,-2.42480761971353));
#68601=CARTESIAN_POINT('Ctrl Pts',(19.0758429349648,-2.08103133123277,-2.46082878928617));
#68602=CARTESIAN_POINT('Ctrl Pts',(19.0768516905573,-2.0688802740121,-2.47105325047359));
#68603=CARTESIAN_POINT('Ctrl Pts',(19.0785936213724,-2.04764146121901,-2.48865807989506));
#68604=CARTESIAN_POINT('Ctrl Pts',(19.0793295196284,-2.03858826010307,-2.49607942742557));
#68605=CARTESIAN_POINT('Ctrl Pts',(19.0803980093954,-2.02532215566365,-2.50683397531472));
#68606=CARTESIAN_POINT('Ctrl Pts',(19.080733341867,-2.02114116458665,-2.51020612855282));
#68607=CARTESIAN_POINT('Ctrl Pts',(19.0813068557279,-2.0139599064157,-2.51596855549932));
#68608=CARTESIAN_POINT('Ctrl Pts',(19.0815454059082,-2.01096377745318,-2.51836394575818));
#68609=CARTESIAN_POINT('Ctrl Pts',(19.0820210370105,-2.00497159709823,-2.52313715188626));
#68610=CARTESIAN_POINT('Ctrl Pts',(19.0822581199902,-2.00197559359882,-2.52551498023637));
#68611=CARTESIAN_POINT('Ctrl Pts',(19.0828250551498,-1.99478957741151,-2.53119745988811));
#68612=CARTESIAN_POINT('Ctrl Pts',(19.0831545460625,-1.99059555934513,-2.53449706237245));
#68613=CARTESIAN_POINT('Ctrl Pts',(19.0843382355519,-1.97546592575178,-2.54633943212475));
#68614=CARTESIAN_POINT('Ctrl Pts',(19.0851882538767,-1.96448316397013,-2.55482211552728));
#68615=CARTESIAN_POINT('Ctrl Pts',(19.0872300856562,-1.93782671200865,-2.57513705235195));
#68616=CARTESIAN_POINT('Ctrl Pts',(19.0884172700055,-1.92209880590669,-2.58689764505222));
#68617=CARTESIAN_POINT('Ctrl Pts',(19.1033631089563,-1.72135179479103,-2.73416519312427));
#68618=CARTESIAN_POINT('Ctrl Pts',(19.1159908096351,-1.52246130869292,-2.84971101512472));
#68619=CARTESIAN_POINT('Ctrl Pts',(19.1414042041509,-1.10763575568693,-3.03476691685052));
#68620=CARTESIAN_POINT('Ctrl Pts',(19.1541295882859,-0.893318733522047,
-3.10461415695245));
#68621=CARTESIAN_POINT('Ctrl Pts',(19.1690739985333,-0.650708539150723,
-3.15645985714619));
#68622=CARTESIAN_POINT('Ctrl Pts',(19.1704851698305,-0.627871768440136,
-3.16108168689464));
#68623=CARTESIAN_POINT('Ctrl Pts',(19.1725161237013,-0.595120116044307,
-3.16734123967173));
#68624=CARTESIAN_POINT('Ctrl Pts',(19.1731294552611,-0.585244215527582,
-3.16918091715226));
#68625=CARTESIAN_POINT('Ctrl Pts',(19.1741939060691,-0.568130981929209,
-3.17228604140608));
#68626=CARTESIAN_POINT('Ctrl Pts',(19.1746443367307,-0.560897585502903,
-3.17357297667568));
#68627=CARTESIAN_POINT('Ctrl Pts',(19.1755105428876,-0.547003429586606,
-3.1759959802576));
#68628=CARTESIAN_POINT('Ctrl Pts',(19.1759261943944,-0.540343366909256,
-3.17713585849257));
#68629=CARTESIAN_POINT('Ctrl Pts',(19.1769053955744,-0.524670437350793,
-3.1797675940332));
#68630=CARTESIAN_POINT('Ctrl Pts',(19.1774694948035,-0.515654749329727,
-3.18124208393997));
#68631=CARTESIAN_POINT('Ctrl Pts',(19.1791372364645,-0.489039973718108,
-3.1854787432568));
#68632=CARTESIAN_POINT('Ctrl Pts',(19.180244283749,-0.47142433346498,-3.1881333091497));
#68633=CARTESIAN_POINT('Ctrl Pts',(19.1955012724945,-0.229380358965879,
-3.22255792709559));
#68634=CARTESIAN_POINT('Ctrl Pts',(19.2104259549474,-0.00227779418153801,
-3.23070457876806));
#68635=CARTESIAN_POINT('Ctrl Pts',(19.2383467692494,0.410827569834983,-3.20195296405217));
#68636=CARTESIAN_POINT('Ctrl Pts',(19.25116025723,0.59640741267276,-3.17263051532355));
#68637=CARTESIAN_POINT('Ctrl Pts',(19.2666534464151,0.824945988472334,-3.11574767733978));
#68638=CARTESIAN_POINT('Ctrl Pts',(19.2697751598095,0.871241837265544,-3.10312063028053));
#68639=CARTESIAN_POINT('Ctrl Pts',(19.2740152450062,0.934699273685092,-3.08428054678533));
#68640=CARTESIAN_POINT('Ctrl Pts',(19.2751747590292,0.952113850784152,-3.07894924819312));
#68641=CARTESIAN_POINT('Ctrl Pts',(19.2768996563874,0.97812655918964,-3.0707439076663));
#68642=CARTESIAN_POINT('Ctrl Pts',(19.2774708904556,0.986758955563268,-3.06798084746457));
#68643=CARTESIAN_POINT('Ctrl Pts',(19.2785067135553,1.00244681280718,-3.06288641005989));
#68644=CARTESIAN_POINT('Ctrl Pts',(19.2789719660595,1.00950605243815,-3.06056699095498));
#68645=CARTESIAN_POINT('Ctrl Pts',(19.2797148610513,1.02079966756017,-3.05681297883345));
#68646=CARTESIAN_POINT('Ctrl Pts',(19.2799934097384,1.02503913751544,-3.05539397066856));
#68647=CARTESIAN_POINT('Ctrl Pts',(19.2805222645747,1.03309790130835,-3.0526779321963));
#68648=CARTESIAN_POINT('Ctrl Pts',(19.2807726614675,1.03691766787931,-3.05138256887592));
#68649=CARTESIAN_POINT('Ctrl Pts',(19.2813450695905,1.04565907643052,-3.04839986341412));
#68650=CARTESIAN_POINT('Ctrl Pts',(19.2816667953427,1.05057906152651,-3.04670777525024));
#68651=CARTESIAN_POINT('Ctrl Pts',(19.2826575403915,1.06575014572033,-3.04144899586515));
#68652=CARTESIAN_POINT('Ctrl Pts',(19.283324228998,1.07598747053171,-3.03784238213104));
#68653=CARTESIAN_POINT('Ctrl Pts',(19.2887631296341,1.15971543410778,-3.0078686360866));
#68654=CARTESIAN_POINT('Ctrl Pts',(19.2933881634955,1.23225066000184,-2.9788880777403));
#68655=CARTESIAN_POINT('Ctrl Pts',(19.3152928300221,1.57731349268273,-2.82625769550204));
#68656=CARTESIAN_POINT('Ctrl Pts',(19.331344018382,1.83278134337235,-2.66769432609381));
#68657=CARTESIAN_POINT('Ctrl Pts',(19.3528508765832,2.11938731689852,-2.42894099797097));
#68658=CARTESIAN_POINT('Ctrl Pts',(19.3571607082895,2.17441326483933,-2.37980730101956));
#68659=CARTESIAN_POINT('Ctrl Pts',(19.363300864777,2.24902466230523,-2.30843588754094));
#68660=CARTESIAN_POINT('Ctrl Pts',(19.3650672573436,2.27006485408745,-2.28774859884894));
#68661=CARTESIAN_POINT('Ctrl Pts',(19.3681756822099,2.30632898732159,-2.25109984372946));
#68662=CARTESIAN_POINT('Ctrl Pts',(19.3695121309953,2.32167882765504,-2.23526537309219));
#68663=CARTESIAN_POINT('Ctrl Pts',(19.3714541900308,2.34362972834558,-2.21215138939556));
#68664=CARTESIAN_POINT('Ctrl Pts',(19.3720541096453,2.35036212944019,-2.20499703635156));
#68665=CARTESIAN_POINT('Ctrl Pts',(19.37310282391,2.36204606663375,-2.19246650170605));
#68666=CARTESIAN_POINT('Ctrl Pts',(19.3735509861827,2.36701224562379,-2.18710402351447));
#68667=CARTESIAN_POINT('Ctrl Pts',(19.3744182691767,2.37657066735608,-2.17671215569577));
#68668=CARTESIAN_POINT('Ctrl Pts',(19.3748372846858,2.38116529759328,-2.17168500710666));
#68669=CARTESIAN_POINT('Ctrl Pts',(19.3759450511905,2.39325038769828,-2.15837781919581));
#68670=CARTESIAN_POINT('Ctrl Pts',(19.3766349421564,2.4007137627231,-2.15007340643303));
#68671=CARTESIAN_POINT('Ctrl Pts',(19.379066644222,2.42679829357903,-2.12074430061063));
#68672=CARTESIAN_POINT('Ctrl Pts',(19.3808181120334,2.44518720365318,-2.09951561195235));
#68673=CARTESIAN_POINT('Ctrl Pts',(19.38306372346,2.46825332616384,-2.07217330125616));
#68674=CARTESIAN_POINT('Ctrl Pts',(19.3835472137446,2.47318971572936,-2.06627909560131));
#68675=CARTESIAN_POINT('Ctrl Pts',(19.3992427125922,2.6324713538276,-1.87470324959702));
#68676=CARTESIAN_POINT('Ctrl Pts',(19.4153336306336,2.76545452620205,-1.67231467599055));
#68677=CARTESIAN_POINT('Ctrl Pts',(19.43978351188,2.92884217398956,-1.34996569972591));
#68678=CARTESIAN_POINT('Ctrl Pts',(19.4479275172098,2.9770849851421,-1.23995583202116));
#68679=CARTESIAN_POINT('Ctrl Pts',(19.4606189171491,3.04373297815114,-1.06149547851009));
#68680=CARTESIAN_POINT('Ctrl Pts',(19.4652585351681,3.06621638360191,-0.99468666545364));
#68681=CARTESIAN_POINT('Ctrl Pts',(19.4721207848168,3.09684534732681,-0.89272691668536));
#68682=CARTESIAN_POINT('Ctrl Pts',(19.4744145080525,3.10662076315755,-0.858090991551482));
#68683=CARTESIAN_POINT('Ctrl Pts',(19.4771896088989,3.11789985002776,-0.815404638342351));
#68684=CARTESIAN_POINT('Ctrl Pts',(19.4777010542599,3.11995526729352,-0.807504385468357));
#68685=CARTESIAN_POINT('Ctrl Pts',(19.4785005696449,3.12313210721124,-0.795100585288707));
#68686=CARTESIAN_POINT('Ctrl Pts',(19.4787897975237,3.12427384015181,-0.790602347714645));
#68687=CARTESIAN_POINT('Ctrl Pts',(19.4793286036165,3.12638683920144,-0.782201424224416));
#68688=CARTESIAN_POINT('Ctrl Pts',(19.4795783161567,3.12736050650948,-0.7782994275778));
#68689=CARTESIAN_POINT('Ctrl Pts',(19.4801426100491,3.12954800968427,-0.769462567671047));
#68690=CARTESIAN_POINT('Ctrl Pts',(19.4804569359534,3.1307574754239,-0.76452666329324));
#68691=CARTESIAN_POINT('Ctrl Pts',(19.4813826829569,3.13429265157615,-0.749950320125462));
#68692=CARTESIAN_POINT('Ctrl Pts',(19.4819922384185,3.13658557119324,-0.740301876927223));
#68693=CARTESIAN_POINT('Ctrl Pts',(19.4861618193415,3.15202629402446,-0.673968695595575));
#68694=CARTESIAN_POINT('Ctrl Pts',(19.489640590406,3.16368225291094,-0.616943401790247));
#68695=CARTESIAN_POINT('Ctrl Pts',(19.5116329106778,3.22867951346079,-0.248329020418671));
#68696=CARTESIAN_POINT('Ctrl Pts',(19.5284918153321,3.23747933245778,0.0693773877777829));
#68697=CARTESIAN_POINT('Ctrl Pts',(19.551101347747,3.19076258393137,0.459368671516029));
#68698=CARTESIAN_POINT('Ctrl Pts',(19.5555716426548,3.17894332183028,0.53507340137765));
#68699=CARTESIAN_POINT('Ctrl Pts',(19.5628542757283,3.15573701976109,0.655403009036923));
#68700=CARTESIAN_POINT('Ctrl Pts',(19.5656134022081,3.14607132942601,0.700331426457077));
#68701=CARTESIAN_POINT('Ctrl Pts',(19.569194947626,3.13243489022064,0.757719721663582));
#68702=CARTESIAN_POINT('Ctrl Pts',(19.5699889557391,3.12934416400893,0.770384717814093));
#68703=CARTESIAN_POINT('Ctrl Pts',(19.5712728017207,3.12423859589389,0.790768226232197));
#68704=CARTESIAN_POINT('Ctrl Pts',(19.5717610841462,3.12227177021382,0.798498705576408));
#68705=CARTESIAN_POINT('Ctrl Pts',(19.5726936563804,3.11846782146986,0.813220921952253));
#68706=CARTESIAN_POINT('Ctrl Pts',(19.5731377772321,3.11663583132536,0.820213944642812));
#68707=CARTESIAN_POINT('Ctrl Pts',(19.5741538189433,3.11239821819931,0.836170452012708));
#68708=CARTESIAN_POINT('Ctrl Pts',(19.5747262312626,3.10997738204567,0.84512979698253));
#68709=CARTESIAN_POINT('Ctrl Pts',(19.5762184919233,3.10357971890653,0.868407344718188));
#68710=CARTESIAN_POINT('Ctrl Pts',(19.577140299399,3.0995425324689,0.88270859601125));
#68711=CARTESIAN_POINT('Ctrl Pts',(19.5830607740857,3.07307198648957,0.97405622009607));
#68712=CARTESIAN_POINT('Ctrl Pts',(19.5881496000922,3.04786821438571,1.05026399134539));
#68713=CARTESIAN_POINT('Ctrl Pts',(19.5973198522107,2.99823172025703,1.18345083601292));
#68714=CARTESIAN_POINT('Ctrl Pts',(19.6013635934688,2.97494905316397,1.24081695350646));
#68715=CARTESIAN_POINT('Ctrl Pts',(19.6055919894123,2.94915916808336,1.29945467172816));
#68716=CARTESIAN_POINT('Ctrl Pts',(19.6057348377648,2.94828621570922,1.30143406777099));
#68717=CARTESIAN_POINT('Ctrl Pts',(19.6223122847033,2.84678458359205,1.53096005240015));
#68718=CARTESIAN_POINT('Ctrl Pts',(19.6394337723317,2.72015890655008,1.74606403498391));
#68719=CARTESIAN_POINT('Ctrl Pts',(19.660372700055,2.53013896625822,1.99722129746198));
#68720=CARTESIAN_POINT('Ctrl Pts',(19.6647204357496,2.48859631533556,2.04875222008995));
#68721=CARTESIAN_POINT('Ctrl Pts',(19.6712007096994,2.42304801360427,2.12512201853792));
#68722=CARTESIAN_POINT('Ctrl Pts',(19.6733958550939,2.40018308930761,2.15091297820777));
#68723=CARTESIAN_POINT('Ctrl Pts',(19.6760678633841,2.37147058838699,2.18227166883929));
#68724=CARTESIAN_POINT('Ctrl Pts',(19.676572251571,2.36601112074458,2.18818960970238));
#68725=CARTESIAN_POINT('Ctrl Pts',(19.6773631934099,2.35738672497007,2.19746824786598));
#68726=CARTESIAN_POINT('Ctrl Pts',(19.6776508648295,2.35423670217204,2.20084266185227));
#68727=CARTESIAN_POINT('Ctrl Pts',(19.6781883015933,2.34832662894692,2.20714653012446));
#68728=CARTESIAN_POINT('Ctrl Pts',(19.6784381944949,2.34556837135872,2.2100775500367));
#68729=CARTESIAN_POINT('Ctrl Pts',(19.6790048762536,2.33929028446925,2.21672387079241));
#68730=CARTESIAN_POINT('Ctrl Pts',(19.679321400731,2.33576710040752,2.22043594995841));
#68731=CARTESIAN_POINT('Ctrl Pts',(19.6802806086358,2.3250407105294,2.23168365309842));
#68732=CARTESIAN_POINT('Ctrl Pts',(19.6809211712189,2.31780968464217,2.2391928246317));
#68733=CARTESIAN_POINT('Ctrl Pts',(19.6856426191976,2.26402018096327,2.2945116260712));
#68734=CARTESIAN_POINT('Ctrl Pts',(19.6896163296568,2.21601937774936,2.34090379121807));
#68735=CARTESIAN_POINT('Ctrl Pts',(19.7028634509873,2.04821004438332,2.49329749758059));
#68736=CARTESIAN_POINT('Ctrl Pts',(19.7117666141936,1.92212096769904,2.59172161007445));
#68737=CARTESIAN_POINT('Ctrl Pts',(19.7206814315572,1.78943602647606,2.6803052568037));
#68738=CARTESIAN_POINT('Origin',(-1.72497344927317,0.,0.));
#68739=CARTESIAN_POINT('',(21.2168443958857,1.78943621037803,2.68030513402633));
#68740=CARTESIAN_POINT('',(20.9673281879432,1.78943621037181,2.68030513403048));
#68741=CARTESIAN_POINT('',(-1.72497344927317,1.78943621037804,2.68030513402633));
#68742=CARTESIAN_POINT('',(20.3965734493048,-3.22274885406294,-0.00271774465727977));
#68743=CARTESIAN_POINT('Ctrl Pts',(20.3965734493048,-3.22274885406294,-0.0027177446573006));
#68744=CARTESIAN_POINT('Ctrl Pts',(20.4039084698346,-3.22264841945202,-0.121814852024652));
#68745=CARTESIAN_POINT('Ctrl Pts',(20.4112434903643,-3.21594228569994,-0.24062621396647));
#68746=CARTESIAN_POINT('Ctrl Pts',(20.4185785108941,-3.20274814338226,-0.358499501480124));
#68747=CARTESIAN_POINT('Ctrl Pts',(20.4260054409484,-3.18938867537232,-0.477849768882879));
#68748=CARTESIAN_POINT('Ctrl Pts',(20.4334323710027,-3.16937766417932,-0.596238263840522));
#68749=CARTESIAN_POINT('Ctrl Pts',(20.4408593010569,-3.14288643768406,-0.713009398480532));
#68750=CARTESIAN_POINT('Ctrl Pts',(20.4466239616218,-3.12232438477968,-0.803645226482011));
#68751=CARTESIAN_POINT('Ctrl Pts',(20.4523886221867,-3.09785925306823,-0.893307093579976));
#68752=CARTESIAN_POINT('Ctrl Pts',(20.4581532827517,-3.06959081273735,-0.981697410029416));
#68753=CARTESIAN_POINT('Ctrl Pts',(20.4643255308444,-3.03932366605053,-1.07633732091077));
#68754=CARTESIAN_POINT('Ctrl Pts',(20.4704977789372,-3.00462231767946,-1.16974272713076));
#68755=CARTESIAN_POINT('Ctrl Pts',(20.47667002703,-2.96560566779542,-1.26146763162582));
#68756=CARTESIAN_POINT('Ctrl Pts',(20.4828339156826,-2.92664186046469,-1.35306830766535));
#68757=CARTESIAN_POINT('Ctrl Pts',(20.4889978043352,-2.88337453667252,-1.44299260958903));
#68758=CARTESIAN_POINT('Ctrl Pts',(20.4951616929879,-2.83597231254074,-1.53080978733556));
#68759=CARTESIAN_POINT('Ctrl Pts',(20.5013190546464,-2.78862028302699,-1.61853397472617));
#68760=CARTESIAN_POINT('Ctrl Pts',(20.507476416305,-2.73714226319858,-1.70415509374264));
#68761=CARTESIAN_POINT('Ctrl Pts',(20.5136337779635,-2.68175450101443,-1.7872633714114));
#68762=CARTESIAN_POINT('Ctrl Pts',(20.5197866421098,-2.62640719562852,-1.87031094442828));
#68763=CARTESIAN_POINT('Ctrl Pts',(20.5259395062561,-2.5671560658485,-1.95084896491966));
#68764=CARTESIAN_POINT('Ctrl Pts',(20.5320923704024,-2.50426226509231,-2.02849403995544));
#68765=CARTESIAN_POINT('Ctrl Pts',(20.538242903539,-2.44139229162379,-2.10610969919003));
#68766=CARTESIAN_POINT('Ctrl Pts',(20.5443934366755,-2.37488266238489,-2.18083425353745));
#68767=CARTESIAN_POINT('Ctrl Pts',(20.5505439698121,-2.30503611580601,-2.25231571217934));
#68768=CARTESIAN_POINT('Ctrl Pts',(20.5566938180273,-2.23519734731543,-2.32378921066968));
#68769=CARTESIAN_POINT('Ctrl Pts',(20.5628436662425,-2.16202270385255,-2.3920200207912));
#68770=CARTESIAN_POINT('Ctrl Pts',(20.5689935144577,-2.08585253992285,-2.4566922363612));
#68771=CARTESIAN_POINT('Ctrl Pts',(20.5751443228368,-2.00967048369248,-2.52137454907939));
#68772=CARTESIAN_POINT('Ctrl Pts',(20.581295131216,-1.93049230920649,-2.5824968825218));
#68773=CARTESIAN_POINT('Ctrl Pts',(20.5874459395951,-1.84869148110703,-2.63978358396712));
#68774=CARTESIAN_POINT('Ctrl Pts',(20.5936033259613,-1.76680317104507,-2.69713155072214));
#68775=CARTESIAN_POINT('Ctrl Pts',(20.5997607123275,-1.68228696297001,-2.75063544451039));
#68776=CARTESIAN_POINT('Ctrl Pts',(20.6059180986937,-1.59554524191772,-2.80006302491457));
#68777=CARTESIAN_POINT('Ctrl Pts',(20.6120789214306,-1.50875511124853,-2.84951819031709));
#68778=CARTESIAN_POINT('Ctrl Pts',(20.6182397441676,-1.41973738112053,-2.89489231454284));
#68779=CARTESIAN_POINT('Ctrl Pts',(20.6244005669046,-1.32891708296139,-2.93600016163375));
#68780=CARTESIAN_POINT('Ctrl Pts',(20.6305716898213,-1.23794494381707,-2.97717673626825));
#68781=CARTESIAN_POINT('Ctrl Pts',(20.636742812738,-1.1451646207189,-3.01407262579408));
#68782=CARTESIAN_POINT('Ctrl Pts',(20.6429139356546,-1.05101919823025,-3.0465515271289));
#68783=CARTESIAN_POINT('Ctrl Pts',(20.6476094576002,-0.979385250351234,
-3.07126427326021));
#68784=CARTESIAN_POINT('Ctrl Pts',(20.6523049795458,-0.906961354554591,
-3.09342082858202));
#68785=CARTESIAN_POINT('Ctrl Pts',(20.6570005014913,-0.833946570311851,
-3.1129809958246));
#68786=CARTESIAN_POINT('Ctrl Pts',(20.6631727495841,-0.737968877520492,
-3.13869277107705));
#68787=CARTESIAN_POINT('Ctrl Pts',(20.6693449976769,-0.640632042801461,
-3.1600069470349));
#68788=CARTESIAN_POINT('Ctrl Pts',(20.6755172457696,-0.542375533400338,
-3.17678238840319));
#68789=CARTESIAN_POINT('Ctrl Pts',(20.6816811344222,-0.44425209859308,-3.19353510980046));
#68790=CARTESIAN_POINT('Ctrl Pts',(20.6878450230749,-0.345211889220213,
-3.20576124213907));
#68791=CARTESIAN_POINT('Ctrl Pts',(20.6940089117275,-0.245708428536648,
-3.21336971583508));
#68792=CARTESIAN_POINT('Ctrl Pts',(20.7001662733861,-0.14631033291329,-3.22097013285364));
#68793=CARTESIAN_POINT('Ctrl Pts',(20.7063236350446,-0.0464503919433015,
-3.22396257943623));
#68794=CARTESIAN_POINT('Ctrl Pts',(20.7124809967031,0.053409762209582,-3.22230739685101));
#68795=CARTESIAN_POINT('Ctrl Pts',(20.7186338608495,0.153196975663071,-3.22065342325826));
#68796=CARTESIAN_POINT('Ctrl Pts',(20.7247867249958,0.25298396898358,-3.21435857703962));
#68797=CARTESIAN_POINT('Ctrl Pts',(20.7309395891421,0.352307020293586,-3.20343523829527));
#68798=CARTESIAN_POINT('Ctrl Pts',(20.7370901222786,0.451592443111013,-3.1925160378528));
#68799=CARTESIAN_POINT('Ctrl Pts',(20.7432406554151,0.550413841867864,-3.17697187651682));
#68800=CARTESIAN_POINT('Ctrl Pts',(20.7493911885517,0.648311424980942,-3.15686709551403));
#68801=CARTESIAN_POINT('Ctrl Pts',(20.7555410367669,0.746198106251643,-3.13676455337298));
#68802=CARTESIAN_POINT('Ctrl Pts',(20.7616908849821,0.843160750914965,-3.11210248866523));
#68803=CARTESIAN_POINT('Ctrl Pts',(20.7678407331973,0.938749582707908,-3.08299639692714));
#68804=CARTESIAN_POINT('Ctrl Pts',(20.7739915415764,1.03435333860067,-3.05388576091112));
#68805=CARTESIAN_POINT('Ctrl Pts',(20.7801423499556,1.12858244001119,-3.02032984626491));
#68806=CARTESIAN_POINT('Ctrl Pts',(20.7862931583347,1.22100306925711,-2.98249376652571));
#68807=CARTESIAN_POINT('Ctrl Pts',(20.7924505447009,1.31352253782048,-2.94461722296012));
#68808=CARTESIAN_POINT('Ctrl Pts',(20.7986079310671,1.40422926930088,-2.9024515385471));
#68809=CARTESIAN_POINT('Ctrl Pts',(20.8047653174333,1.49271032728007,-2.85620962839414));
#68810=CARTESIAN_POINT('Ctrl Pts',(20.8109261401702,1.58124076558128,-2.80994191113099));
#68811=CARTESIAN_POINT('Ctrl Pts',(20.8170869629072,1.66754268150185,-2.75959365659507));
#68812=CARTESIAN_POINT('Ctrl Pts',(20.8232477856442,1.75123043405774,-2.70542224603295));
#68813=CARTESIAN_POINT('Ctrl Pts',(20.8294189085608,1.8350581028114,-2.65116026716706));
#68814=CARTESIAN_POINT('Ctrl Pts',(20.8355900314775,1.91626252467126,-2.59306261757174));
#68815=CARTESIAN_POINT('Ctrl Pts',(20.8417611543942,1.99448945990918,-2.53142832345915));
#68816=CARTESIAN_POINT('Ctrl Pts',(20.8464566763398,2.054011251341,-2.48453164282019));
#68817=CARTESIAN_POINT('Ctrl Pts',(20.8511521982854,2.11180988520511,-2.43558829240713));
#68818=CARTESIAN_POINT('Ctrl Pts',(20.855847720231,2.1677439137054,-2.38474398774653));
#68819=CARTESIAN_POINT('Ctrl Pts',(20.8620199683238,2.24126900947336,-2.31790931715942));
#68820=CARTESIAN_POINT('Ctrl Pts',(20.8681922164166,2.31182970747074,-2.24755349730068));
#68821=CARTESIAN_POINT('Ctrl Pts',(20.8743644645093,2.37906965898984,-2.17396989863567));
#68822=CARTESIAN_POINT('Ctrl Pts',(20.880528353162,2.44621854347132,-2.10048595858426));
#68823=CARTESIAN_POINT('Ctrl Pts',(20.8866922418146,2.5100553302807,-2.02378324654332));
#68824=CARTESIAN_POINT('Ctrl Pts',(20.8928561304672,2.57025818620453,-1.94419402806114));
#68825=CARTESIAN_POINT('Ctrl Pts',(20.8990134921258,2.63039729281253,-1.86468908727887));
#68826=CARTESIAN_POINT('Ctrl Pts',(20.9051708537843,2.68690985812159,-1.78230406127739));
#68827=CARTESIAN_POINT('Ctrl Pts',(20.9113282154429,2.73951291161525,-1.69740583526549));
#68828=CARTESIAN_POINT('Ctrl Pts',(20.9174810795892,2.79207754234115,-1.61256962133473));
#68829=CARTESIAN_POINT('Ctrl Pts',(20.9236339437355,2.84073811061664,-1.52522422523414));
#68830=CARTESIAN_POINT('Ctrl Pts',(20.9297868078818,2.88525429152501,-1.43576642798769));
#68831=CARTESIAN_POINT('Ctrl Pts',(20.9359373410183,2.92975360749858,-1.34634252178686));
#68832=CARTESIAN_POINT('Ctrl Pts',(20.9420878741548,2.9701114625802,-1.25480819305112));
#68833=CARTESIAN_POINT('Ctrl Pts',(20.9482384072914,3.00613336716641,-1.16158501251899));
#68834=CARTESIAN_POINT('Ctrl Pts',(20.9543882555066,3.04215126036528,-1.0683722132893));
#68835=CARTESIAN_POINT('Ctrl Pts',(20.9605381037218,3.07383400648183,-0.97347134135303));
#68836=CARTESIAN_POINT('Ctrl Pts',(20.966687951937,3.10103556276004,-0.877323202131077));
#68837=CARTESIAN_POINT('Ctrl Pts',(20.9728387603161,3.12824136596472,-0.781160051485772));
#68838=CARTESIAN_POINT('Ctrl Pts',(20.9789895686952,3.15096447140595,-0.683749664773333));
#68839=CARTESIAN_POINT('Ctrl Pts',(20.9851403770744,3.16910920440028,-0.58554625187546));
#68840=CARTESIAN_POINT('Ctrl Pts',(20.9912977634406,3.18727334229416,-0.487237815257345));
#68841=CARTESIAN_POINT('Ctrl Pts',(20.9974551498068,3.20084925117145,-0.388135086858821));
#68842=CARTESIAN_POINT('Ctrl Pts',(21.0036125361729,3.20979275816905,-0.288700557854578));
#68843=CARTESIAN_POINT('Ctrl Pts',(21.0097733589099,3.21874125644122,-0.189210535514574));
#68844=CARTESIAN_POINT('Ctrl Pts',(21.0159341816469,3.22305218551559,-0.0893887777816784));
#68845=CARTESIAN_POINT('Ctrl Pts',(21.0220950043838,3.22273353676235,0.0103011420352819));
#68846=CARTESIAN_POINT('Ctrl Pts',(21.0282661273005,3.22241435526542,0.110157731814233));
#68847=CARTESIAN_POINT('Ctrl Pts',(21.0344372502172,3.21745015690376,0.209881609359754));
#68848=CARTESIAN_POINT('Ctrl Pts',(21.0406083731339,3.20790094414447,0.309013098520099));
#68849=CARTESIAN_POINT('Ctrl Pts',(21.0453038950794,3.20063508043062,0.384440875463251));
#68850=CARTESIAN_POINT('Ctrl Pts',(21.049999417025,3.19071581091794,0.459525772203122));
#68851=CARTESIAN_POINT('Ctrl Pts',(21.0546949389705,3.17818923053461,0.534070011715522));
#68852=CARTESIAN_POINT('Ctrl Pts',(21.0608680040607,3.16172090242125,0.63207113873379));
#68853=CARTESIAN_POINT('Ctrl Pts',(21.0670410691508,3.14068646221925,0.729482353170679));
#68854=CARTESIAN_POINT('Ctrl Pts',(21.0732141342409,3.11514003931512,0.82584508108713));
#68855=CARTESIAN_POINT('Ctrl Pts',(21.0793768581294,3.08963641212206,0.922046380866371));
#68856=CARTESIAN_POINT('Ctrl Pts',(21.0855395820179,3.05963595228572,1.01720227274774));
#68857=CARTESIAN_POINT('Ctrl Pts',(21.0917023059064,3.02524408820333,1.11086262395076));
#68858=CARTESIAN_POINT('Ctrl Pts',(21.0978591145962,2.99088523463951,1.2044330766605));
#68859=CARTESIAN_POINT('Ctrl Pts',(21.104015923286,2.9521435003847,1.29651043561477));
#68860=CARTESIAN_POINT('Ctrl Pts',(21.1101727319757,2.90917446053823,1.38665840085153));
#68861=CARTESIAN_POINT('Ctrl Pts',(21.1163252782469,2.86623516857617,1.47674395577471));
#68862=CARTESIAN_POINT('Ctrl Pts',(21.1224778245181,2.8190745739082,1.56490238096836));
#68863=CARTESIAN_POINT('Ctrl Pts',(21.1286303707893,2.76789646638622,1.65071703022253));
#68864=CARTESIAN_POINT('Ctrl Pts',(21.1347803034177,2.7167400996667,1.73649522483959));
#68865=CARTESIAN_POINT('Ctrl Pts',(21.140930236046,2.66156983598659,1.81993125087876));
#68866=CARTESIAN_POINT('Ctrl Pts',(21.1470801686744,2.60263505790736,1.90063366219047));
#68867=CARTESIAN_POINT('Ctrl Pts',(21.1532311967123,2.54368978252358,1.98135044799916));
#68868=CARTESIAN_POINT('Ctrl Pts',(21.1593822247501,2.48097890090506,2.0593322891714));
#68869=CARTESIAN_POINT('Ctrl Pts',(21.165533252788,2.4147944155433,2.13421777079118));
#68870=CARTESIAN_POINT('Ctrl Pts',(21.1716846498006,2.3486059600478,2.20910774448151));
#68871=CARTESIAN_POINT('Ctrl Pts',(21.1778360468132,2.27894378007838,2.28090066870694));
#68872=CARTESIAN_POINT('Ctrl Pts',(21.1839874438259,2.20613832156088,2.34927036942122));
#68873=CARTESIAN_POINT('Ctrl Pts',(21.1901443124187,2.13326810362314,2.41770088401225));
#68874=CARTESIAN_POINT('Ctrl Pts',(21.1963011810115,2.05724934509148,2.48270180114223));
#68875=CARTESIAN_POINT('Ctrl Pts',(21.2024580496043,1.97844711928728,2.54398595882207));
#68876=CARTESIAN_POINT('Ctrl Pts',(21.2072534983648,1.91706980866938,2.59171883366774));
#68877=CARTESIAN_POINT('Ctrl Pts',(21.2120489471252,1.85400463589929,2.63719769927644));
#68878=CARTESIAN_POINT('Ctrl Pts',(21.2168443958857,1.78943621037803,2.68030513402633));
#68879=CARTESIAN_POINT('Ctrl Pts',(19.9669438677106,1.78943621037804,2.68030513402633));
#68880=CARTESIAN_POINT('Ctrl Pts',(19.9730942171982,1.70631862674015,2.73579643312977));
#68881=CARTESIAN_POINT('Ctrl Pts',(19.9792445666858,1.62062618941371,2.78741199000142));
#68882=CARTESIAN_POINT('Ctrl Pts',(19.9853949161734,1.53276032849706,2.83491857694107));
#68883=CARTESIAN_POINT('Ctrl Pts',(19.9916502435984,1.44339471917444,2.88323603544441));
#68884=CARTESIAN_POINT('Ctrl Pts',(19.9979055710233,1.35178120773494,2.92730272350199));
#68885=CARTESIAN_POINT('Ctrl Pts',(20.0041608984482,1.25836630716031,2.9669229513932));
#68886=CARTESIAN_POINT('Ctrl Pts',(20.0103206012078,1.16637943233011,3.0059375081861));
#68887=CARTESIAN_POINT('Ctrl Pts',(20.0164803039674,1.07264629273122,3.04064050720801));
#68888=CARTESIAN_POINT('Ctrl Pts',(20.022640006727,0.977610152184573,3.07089497587359));
#68889=CARTESIAN_POINT('Ctrl Pts',(20.0289431464846,0.880360966750745,3.10185396070333));
#68890=CARTESIAN_POINT('Ctrl Pts',(20.0352462862422,0.781747811513302,3.12815453582589));
#68891=CARTESIAN_POINT('Ctrl Pts',(20.0415494259997,0.682256880388447,3.14970524202863));
#68892=CARTESIAN_POINT('Ctrl Pts',(20.0478525657573,0.582765949263606,3.17125594823137));
#68893=CARTESIAN_POINT('Ctrl Pts',(20.0541557055149,0.482397726816721,3.18805677235531));
#68894=CARTESIAN_POINT('Ctrl Pts',(20.0604588452725,0.381642573167133,3.20007289117707));
#68895=CARTESIAN_POINT('Ctrl Pts',(20.0666310933652,0.282979711661953,3.21183948200839));
#68896=CARTESIAN_POINT('Ctrl Pts',(20.072803341458,0.183598511516072,3.21905963072166));
#68897=CARTESIAN_POINT('Ctrl Pts',(20.0789755895508,0.0839540715665517,
3.22165629395307));
#68898=CARTESIAN_POINT('Ctrl Pts',(20.0851394782034,-0.0155554140324681,
3.22424944037008));
#68899=CARTESIAN_POINT('Ctrl Pts',(20.091303366856,-0.115327000405413,3.22223153622414));
#68900=CARTESIAN_POINT('Ctrl Pts',(20.0974672555086,-0.21489881363349,3.21557709632329));
#68901=CARTESIAN_POINT('Ctrl Pts',(20.1036246171672,-0.314365189423047,
3.20892970286535));
#68902=CARTESIAN_POINT('Ctrl Pts',(20.1097819788257,-0.413631781613563,
3.19765556333951));
#68903=CARTESIAN_POINT('Ctrl Pts',(20.1159393404843,-0.512236019325593,
3.18178123430972));
#68904=CARTESIAN_POINT('Ctrl Pts',(20.1220922046306,-0.610768233694957,
3.16591850034182));
#68905=CARTESIAN_POINT('Ctrl Pts',(20.1282450687769,-0.708638627907619,
3.14546232617529));
#68906=CARTESIAN_POINT('Ctrl Pts',(20.1343979329232,-0.805389981364252,
3.12049107360013));
#68907=CARTESIAN_POINT('Ctrl Pts',(20.1405484660597,-0.902104680614698,
3.09552928137263));
#68908=CARTESIAN_POINT('Ctrl Pts',(20.1466989991963,-0.997700761366174,
3.0660559179943));
#68909=CARTESIAN_POINT('Ctrl Pts',(20.1528495323328,-1.09173230074264,3.03220021535768));
#68910=CARTESIAN_POINT('Ctrl Pts',(20.158999380548,-1.18575336879797,2.99834828288092));
#68911=CARTESIAN_POINT('Ctrl Pts',(20.1651492287632,-1.27820983317403,2.96011512854095));
#68912=CARTESIAN_POINT('Ctrl Pts',(20.1712990769784,-1.36867297657283,2.91767918827607));
#68913=CARTESIAN_POINT('Ctrl Pts',(20.1774498853575,-1.4591502438078,2.87523662256964));
#68914=CARTESIAN_POINT('Ctrl Pts',(20.1836006937367,-1.54763317862179,2.82859015210215));
#68915=CARTESIAN_POINT('Ctrl Pts',(20.1897515021158,-1.63371593283588,2.77796504896987));
#68916=CARTESIAN_POINT('Ctrl Pts',(20.195908888482,-1.7198907483218,2.72728580477969));
#68917=CARTESIAN_POINT('Ctrl Pts',(20.2020662748482,-1.80365988226804,2.67261965185332));
#68918=CARTESIAN_POINT('Ctrl Pts',(20.2082236612143,-1.88464496906871,2.61423619879));
#68919=CARTESIAN_POINT('Ctrl Pts',(20.2143844839513,-1.96567525277091,2.55582016255263));
#68920=CARTESIAN_POINT('Ctrl Pts',(20.2205453066883,-2.04391805489442,2.49368296481865));
#68921=CARTESIAN_POINT('Ctrl Pts',(20.2267061294252,-2.11902836556457,2.42813433492316));
#68922=CARTESIAN_POINT('Ctrl Pts',(20.2328772523419,-2.19426425194636,2.36247611533522));
#68923=CARTESIAN_POINT('Ctrl Pts',(20.2390483752586,-2.26635687202856,2.29339537165235));
#68924=CARTESIAN_POINT('Ctrl Pts',(20.2452194981753,-2.33499823336709,2.22123857626158));
#68925=CARTESIAN_POINT('Ctrl Pts',(20.2499150201208,-2.38722649439675,2.166335470157));
#68926=CARTESIAN_POINT('Ctrl Pts',(20.2546105420664,-2.43745742487321,2.1096522517446));
#68927=CARTESIAN_POINT('Ctrl Pts',(20.259306064012,-2.48557179491179,2.0513533130202));
#68928=CARTESIAN_POINT('Ctrl Pts',(20.2654494495405,-2.5485222247117,1.97507790410108));
#68929=CARTESIAN_POINT('Ctrl Pts',(20.271592835069,-2.60807636476049,1.89575905697603));
#68930=CARTESIAN_POINT('Ctrl Pts',(20.2777362205975,-2.66392368938818,1.81373320519211));
#68931=CARTESIAN_POINT('Ctrl Pts',(20.2838716717915,-2.71969888581354,1.73181329182643));
#68932=CARTESIAN_POINT('Ctrl Pts',(20.2900071229855,-2.77177653159852,1.64719367652906));
#68933=CARTESIAN_POINT('Ctrl Pts',(20.2961425741796,-2.81988544742911,1.560244732687));
#68934=CARTESIAN_POINT('Ctrl Pts',(20.3022717794618,-2.86794538820766,1.47338430318737));
#68935=CARTESIAN_POINT('Ctrl Pts',(20.3084009847441,-2.91204441515768,1.3841996375125));
#68936=CARTESIAN_POINT('Ctrl Pts',(20.3145301900264,-2.95195450045975,1.29309017075973));
#68937=CARTESIAN_POINT('Ctrl Pts',(20.3206548317614,-2.99183487039829,1.20204854026701));
#68938=CARTESIAN_POINT('Ctrl Pts',(20.3267794734963,-3.02753232243455,1.10908535734209));
#68939=CARTESIAN_POINT('Ctrl Pts',(20.3329041152313,-3.05886516307952,1.01462381038419));
#68940=CARTESIAN_POINT('Ctrl Pts',(20.3390266838001,-3.09018739768616,0.92019423827334));
#68941=CARTESIAN_POINT('Ctrl Pts',(20.3451492523689,-3.11714781439698,0.824267724102018));
#68942=CARTESIAN_POINT('Ctrl Pts',(20.3512718209377,-3.13961351635457,0.727285728186446));
#68943=CARTESIAN_POINT('Ctrl Pts',(20.3573931590532,-3.16207470337753,0.630323222753389));
#68944=CARTESIAN_POINT('Ctrl Pts',(20.3635144971687,-3.180042877248,0.532306085458401));
#68945=CARTESIAN_POINT('Ctrl Pts',(20.3696358352842,-3.19343581795904,0.433687951269458));
#68946=CARTESIAN_POINT('Ctrl Pts',(20.3757593834993,-3.20683359417032,0.335034211157722));
#68947=CARTESIAN_POINT('Ctrl Pts',(20.3818829317143,-3.21565278223615,0.235779475920398));
#68948=CARTESIAN_POINT('Ctrl Pts',(20.3880064799293,-3.21986288635336,0.136383853825077));
#68949=CARTESIAN_POINT('Ctrl Pts',(20.3908621363773,-3.22182622697657,0.0900316836186007));
#68950=CARTESIAN_POINT('Ctrl Pts',(20.3937177928252,-3.22278795507048,0.0436489185283968));
#68951=CARTESIAN_POINT('Ctrl Pts',(20.3965734492731,-3.22274885406337,-0.00271774414203127));
#68952=CARTESIAN_POINT('Ctrl Pts',(19.7206814315572,1.78943602647607,2.6803052568037));
#68953=CARTESIAN_POINT('Ctrl Pts',(19.7289802291916,1.66591970175143,2.76276771542073));
#68954=CARTESIAN_POINT('Ctrl Pts',(19.7372902951155,1.53668781520546,2.8367029284314));
#68955=CARTESIAN_POINT('Ctrl Pts',(19.7502089053106,1.33477329037264,2.93431017825189));
#68956=CARTESIAN_POINT('Ctrl Pts',(19.7546090323161,1.26580402635902,2.96471498196429));
#68957=CARTESIAN_POINT('Ctrl Pts',(19.7617870253068,1.15367465474395,3.00952051990762));
#68958=CARTESIAN_POINT('Ctrl Pts',(19.7645136235498,1.11116371598277,3.02547415306848));
#68959=CARTESIAN_POINT('Ctrl Pts',(19.7680585821135,1.05608417200107,3.04482713786495));
#68960=CARTESIAN_POINT('Ctrl Pts',(19.7688492493658,1.04381109360894,3.04905632466441));
#68961=CARTESIAN_POINT('Ctrl Pts',(19.7701289921938,1.02396746701611,3.05576039989184));
#68962=CARTESIAN_POINT('Ctrl Pts',(19.7706165304726,1.01641262672995,3.05828160336431));
#68963=CARTESIAN_POINT('Ctrl Pts',(19.7715485451682,1.00198006699373,3.06303865620979));
#68964=CARTESIAN_POINT('Ctrl Pts',(19.7719928561243,0.995104006507827,3.06527941286962));
#68965=CARTESIAN_POINT('Ctrl Pts',(19.7730105501088,0.979364497026078,3.07035003105503));
#68966=CARTESIAN_POINT('Ctrl Pts',(19.7735844303595,0.970496249378194,3.07316468128043));
#68967=CARTESIAN_POINT('Ctrl Pts',(19.7753524407012,0.943198439125302,3.08169865919526));
#68968=CARTESIAN_POINT('Ctrl Pts',(19.7765507310396,0.924729857029722,3.08729081673171));
#68969=CARTESIAN_POINT('Ctrl Pts',(19.7935404217358,0.663376023866606,3.16387141920115));
#68970=CARTESIAN_POINT('Ctrl Pts',(19.8103135050892,0.413056312934985,3.20616328004224));
#68971=CARTESIAN_POINT('Ctrl Pts',(19.8374924096142,0.0115765992932028,
3.22617335865394));
#68972=CARTESIAN_POINT('Ctrl Pts',(19.8476256850581,-0.137612394891393,
3.22325837963423));
#68973=CARTESIAN_POINT('Ctrl Pts',(19.8612410909834,-0.342625340216841,
3.2049882277363));
#68974=CARTESIAN_POINT('Ctrl Pts',(19.8649539245169,-0.399042914708731,
3.1984538787418));
#68975=CARTESIAN_POINT('Ctrl Pts',(19.8705903113331,-0.485921673878087,
3.18605663299165));
#68976=CARTESIAN_POINT('Ctrl Pts',(19.8725596254666,-0.516518440073175,
3.18123963469908));
#68977=CARTESIAN_POINT('Ctrl Pts',(19.8749936903938,-0.554703442397623,
3.17466251550715));
#68978=CARTESIAN_POINT('Ctrl Pts',(19.8754805456949,-0.562359846195949,
3.17331520696098));
#68979=CARTESIAN_POINT('Ctrl Pts',(19.8762501641119,-0.574494140235761,
3.17113462175542));
#68980=CARTESIAN_POINT('Ctrl Pts',(19.8765339479639,-0.578975207605876,
3.1703195447861));
#68981=CARTESIAN_POINT('Ctrl Pts',(19.877068103554,-0.587422814508041,3.16876447217507));
#68982=CARTESIAN_POINT('Ctrl Pts',(19.8773185856887,-0.591389645411858,
3.16802653565467));
#68983=CARTESIAN_POINT('Ctrl Pts',(19.877891872028,-0.600481055493412,3.16631761954002));
#68984=CARTESIAN_POINT('Ctrl Pts',(19.8782143875523,-0.605604661108876,
3.16534164999124));
#68985=CARTESIAN_POINT('Ctrl Pts',(19.8792099711976,-0.62144785500857,3.16228388481651));
#68986=CARTESIAN_POINT('Ctrl Pts',(19.8798806755426,-0.63215938533121,3.16016001560192));
#68987=CARTESIAN_POINT('Ctrl Pts',(19.8854409268335,-0.721255145672709,
3.14202308066662));
#68988=CARTESIAN_POINT('Ctrl Pts',(19.8901758818645,-0.79903630007227,3.12314927901672));
#68989=CARTESIAN_POINT('Ctrl Pts',(19.8966037168646,-0.905701274256411,
3.0930199931721));
#68990=CARTESIAN_POINT('Ctrl Pts',(19.8983766981551,-0.935240404890352,
3.08421674845799));
#68991=CARTESIAN_POINT('Ctrl Pts',(19.9085320212259,-1.10473346694555,3.03104541172181));
#68992=CARTESIAN_POINT('Ctrl Pts',(19.9166721877592,-1.24165650023627,2.97757705066822));
#68993=CARTESIAN_POINT('Ctrl Pts',(19.9372657866948,-1.57446099334369,2.82065298361735));
#68994=CARTESIAN_POINT('Ctrl Pts',(19.9497983535513,-1.76419422005291,2.70603216277327));
#68995=CARTESIAN_POINT('Ctrl Pts',(19.9645078303311,-1.95911381884285,2.5590082354429));
#68996=CARTESIAN_POINT('Ctrl Pts',(19.9659056548041,-1.97738722001914,2.54491450616881));
#68997=CARTESIAN_POINT('Ctrl Pts',(19.9679207611938,-2.00336502004563,2.52442989490071));
#68998=CARTESIAN_POINT('Ctrl Pts',(19.9685317313592,-2.01119373941462,2.51819725931001));
#68999=CARTESIAN_POINT('Ctrl Pts',(19.9695934000173,-2.02471438806824,2.50732987190517));
#69000=CARTESIAN_POINT('Ctrl Pts',(19.970043419882,-2.0304197759055,2.50271192349335));
#69001=CARTESIAN_POINT('Ctrl Pts',(19.9709097679311,-2.04135371104809,2.49379998489755));
#69002=CARTESIAN_POINT('Ctrl Pts',(19.9713259753534,-2.04658461538731,2.48950893736709));
#69003=CARTESIAN_POINT('Ctrl Pts',(19.9723079135283,-2.05887378256289,2.47936290403284));
#69004=CARTESIAN_POINT('Ctrl Pts',(19.9728742014607,-2.06592061540058,2.47349422285426));
#69005=CARTESIAN_POINT('Ctrl Pts',(19.974552682025,-2.08668751057707,2.45604866797816));
#69006=CARTESIAN_POINT('Ctrl Pts',(19.9756683415232,-2.10033582563484,2.44438729026499));
#69007=CARTESIAN_POINT('Ctrl Pts',(19.9897993108338,-2.27123683098548,2.29587815510908));
#69008=CARTESIAN_POINT('Ctrl Pts',(20.0034626767976,-2.41491979028521,2.14422619535186));
#69009=CARTESIAN_POINT('Ctrl Pts',(20.0290237173945,-2.64848716836799,1.84422184490517));
#69010=CARTESIAN_POINT('Ctrl Pts',(20.0407569811577,-2.74302531105695,1.70042660936587));
#69011=CARTESIAN_POINT('Ctrl Pts',(20.0569667380699,-2.85998108597723,1.48718609848464));
#69012=CARTESIAN_POINT('Ctrl Pts',(20.0616693071054,-2.8922254505176,1.42346326695561));
#69013=CARTESIAN_POINT('Ctrl Pts',(20.0686134800997,-2.93763525762032,1.32579591356883));
#69014=CARTESIAN_POINT('Ctrl Pts',(20.0709280640983,-2.95238544904572,1.29261600684481));
#69015=CARTESIAN_POINT('Ctrl Pts',(20.0737249249903,-2.96977096124173,1.25165690673077));
#69016=CARTESIAN_POINT('Ctrl Pts',(20.0742378213022,-2.97294074380799,1.24410928445468));
#69017=CARTESIAN_POINT('Ctrl Pts',(20.0750390986676,-2.97786437509233,1.23225927076503));
#69018=CARTESIAN_POINT('Ctrl Pts',(20.0753286458914,-2.9796377104106,1.22796508996803));
#69019=CARTESIAN_POINT('Ctrl Pts',(20.0758677365172,-2.98292856148737,1.21994710079582));
#69020=CARTESIAN_POINT('Ctrl Pts',(20.0761174156275,-2.98444837802755,1.21622432586366));
#69021=CARTESIAN_POINT('Ctrl Pts',(20.0766812360623,-2.98787051527878,1.20779679547853));
#69022=CARTESIAN_POINT('Ctrl Pts',(20.0769951237206,-2.9897686881931,1.20309039859039));
#69023=CARTESIAN_POINT('Ctrl Pts',(20.0779183954819,-2.99533102130554,1.1892044919493));
#69024=CARTESIAN_POINT('Ctrl Pts',(20.0785259288192,-2.99896411953153,1.18001248577706));
#69025=CARTESIAN_POINT('Ctrl Pts',(20.0826545463061,-3.02346264146662,1.11718542665454));
#69026=CARTESIAN_POINT('Ctrl Pts',(20.0860961727694,-3.04293190898718,1.06301269342243));
#69027=CARTESIAN_POINT('Ctrl Pts',(20.0968283827786,-3.1000585176466,0.889598430721381));
#69028=CARTESIAN_POINT('Ctrl Pts',(20.1038951214382,-3.13223623259125,0.768667320473749));
#69029=CARTESIAN_POINT('Ctrl Pts',(20.1230422021435,-3.20071234172113,0.434076982630533));
#69030=CARTESIAN_POINT('Ctrl Pts',(20.1349950551912,-3.22263527377611,0.218170968691717));
#69031=CARTESIAN_POINT('Ctrl Pts',(20.1476543523149,-3.22275026120138,0.00035588477229578));
#69032=CARTESIAN_POINT('Ctrl Pts',(20.1477325700598,-3.2227501289256,-0.000989561080740707));
#69033=CARTESIAN_POINT('Ctrl Pts',(20.1484713113117,-3.22274092450776,-0.0136933996024656));
#69034=CARTESIAN_POINT('Ctrl Pts',(20.1491333204908,-3.22267264703738,-0.0250515796886401));
#69035=CARTESIAN_POINT('Ctrl Pts',(20.1543970996916,-3.22165477417427,-0.115142872878734));
#69036=CARTESIAN_POINT('Ctrl Pts',(20.1590721954234,-3.21788015495692,-0.193812107968267));
#69037=CARTESIAN_POINT('Ctrl Pts',(20.1647327461069,-3.20998153677356,-0.286974158346346));
#69038=CARTESIAN_POINT('Ctrl Pts',(20.1656299128291,-3.20863288654313,-0.301679668029256));
#69039=CARTESIAN_POINT('Ctrl Pts',(20.1670943754145,-3.2062749307442,-0.325582920431327));
#69040=CARTESIAN_POINT('Ctrl Pts',(20.1676597363297,-3.2053269870437,-0.33478660802144));
#69041=CARTESIAN_POINT('Ctrl Pts',(20.1686688439573,-3.20356819642222,-0.351170303752988));
#69042=CARTESIAN_POINT('Ctrl Pts',(20.1691120998742,-3.20277280809544,-0.358351935587643));
#69043=CARTESIAN_POINT('Ctrl Pts',(20.1700472373982,-3.20104682461974,-0.373471095635817));
#69044=CARTESIAN_POINT('Ctrl Pts',(20.1705392864184,-3.20011084302665,-0.381407948512044));
#69045=CARTESIAN_POINT('Ctrl Pts',(20.171840640307,-3.19756220801141,-0.402349616818439));
#69046=CARTESIAN_POINT('Ctrl Pts',(20.1726515150272,-3.19589975139659,-0.415348118001118));
#69047=CARTESIAN_POINT('Ctrl Pts',(20.1763596372003,-3.18795980514592,-0.47455734979508));
#69048=CARTESIAN_POINT('Ctrl Pts',(20.1792859593834,-3.1807592640557,-0.520636661804334));
#69049=CARTESIAN_POINT('Ctrl Pts',(20.1872007832742,-3.15882170635153,-0.643484217162877));
#69050=CARTESIAN_POINT('Ctrl Pts',(20.1922438068385,-3.14228815791712,-0.719895836793292));
#69051=CARTESIAN_POINT('Ctrl Pts',(20.2187049725916,-3.04252396783887,-1.11149059445214));
#69052=CARTESIAN_POINT('Ctrl Pts',(20.2414377149087,-2.91461933617843,-1.41326324249615));
#69053=CARTESIAN_POINT('Ctrl Pts',(20.2656694398784,-2.71893518199291,-1.73081753219396));
#69054=CARTESIAN_POINT('Ctrl Pts',(20.2686901346675,-2.6933369219396,-1.7703882746673));
#69055=CARTESIAN_POINT('Ctrl Pts',(20.2721911217662,-2.66211734992872,-1.81640322903893));
#69056=CARTESIAN_POINT('Ctrl Pts',(20.2727232850044,-2.65732850491791,-1.82340195678699));
#69057=CARTESIAN_POINT('Ctrl Pts',(20.2735769640072,-2.64957541455836,-1.8346374080525));
#69058=CARTESIAN_POINT('Ctrl Pts',(20.2738996280088,-2.64662854003478,-1.83888598570491));
#69059=CARTESIAN_POINT('Ctrl Pts',(20.2744731473428,-2.6413610066962,-1.84644141932421));
#69060=CARTESIAN_POINT('Ctrl Pts',(20.274724273071,-2.63904434414623,-1.84975101919495));
#69061=CARTESIAN_POINT('Ctrl Pts',(20.2752561030354,-2.63411645134774,-1.85676293808298));
#69062=CARTESIAN_POINT('Ctrl Pts',(20.2755366956653,-2.63150364402591,-1.86046409790142));
#69063=CARTESIAN_POINT('Ctrl Pts',(20.2762906304546,-2.62444884506474,-1.87041294540837));
#69064=CARTESIAN_POINT('Ctrl Pts',(20.2767629807737,-2.6199923182591,-1.87665036216145));
#69065=CARTESIAN_POINT('Ctrl Pts',(20.2790588566986,-2.5981551552206,-1.90698455296931));
#69066=CARTESIAN_POINT('Ctrl Pts',(20.2808616958443,-2.58046343998206,-1.93085703221845));
#69067=CARTESIAN_POINT('Ctrl Pts',(20.2858606978108,-2.52996707990865,-1.99706078127216));
#69068=CARTESIAN_POINT('Ctrl Pts',(20.2890135809553,-2.49643265780358,-2.03882560381484));
#69069=CARTESIAN_POINT('Ctrl Pts',(20.2946949604353,-2.4332854770754,-2.11357552274144));
#69070=CARTESIAN_POINT('Ctrl Pts',(20.2972365192397,-2.40400433104826,-2.14682163602927));
#69071=CARTESIAN_POINT('Ctrl Pts',(20.3189265061937,-2.14630771085541,-2.42752658386254));
#69072=CARTESIAN_POINT('Ctrl Pts',(20.3370540436743,-1.88111474928892,-2.63835918022059));
#69073=CARTESIAN_POINT('Ctrl Pts',(20.3575307933085,-1.58254420988207,-2.80743864052252));
#69074=CARTESIAN_POINT('Ctrl Pts',(20.3579103545594,-1.57700869249403,-2.81055181049625));
#69075=CARTESIAN_POINT('Ctrl Pts',(20.3602499104094,-1.54288268837285,-2.82961168477673));
#69076=CARTESIAN_POINT('Ctrl Pts',(20.3622241201737,-1.51406060524487,-2.84513789481262));
#69077=CARTESIAN_POINT('Ctrl Pts',(20.3649369693509,-1.47445105212665,-2.86570290559432));
#69078=CARTESIAN_POINT('Ctrl Pts',(20.3656620336859,-1.46386417026199,-2.87112534267082));
#69079=CARTESIAN_POINT('Ctrl Pts',(20.3668141252229,-1.44704288754362,-2.87962372010225));
#69080=CARTESIAN_POINT('Ctrl Pts',(20.3672397900481,-1.44082806517103,-2.88273834629208));
#69081=CARTESIAN_POINT('Ctrl Pts',(20.3681102278696,-1.42812009576557,-2.88905572341396));
#69082=CARTESIAN_POINT('Ctrl Pts',(20.3685550581731,-1.42162613950074,-2.89225674846581));
#69083=CARTESIAN_POINT('Ctrl Pts',(20.3695771448402,-1.40670617221827,-2.89954876511996));
#69084=CARTESIAN_POINT('Ctrl Pts',(20.3701549137137,-1.39827303206734,-2.90362494497681));
#69085=CARTESIAN_POINT('Ctrl Pts',(20.371946692167,-1.37212390766454,-2.91612385585074));
#69086=CARTESIAN_POINT('Ctrl Pts',(20.3731650260043,-1.35434895817158,-2.92442152104124));
#69087=CARTESIAN_POINT('Ctrl Pts',(20.383894223218,-1.19788448912377,-2.99572951795048));
#69088=CARTESIAN_POINT('Ctrl Pts',(20.3937400599149,-1.05498574185414,-3.04898599680294));
#69089=CARTESIAN_POINT('Ctrl Pts',(20.4239484558779,-0.61796845565421,-3.17744732993056));
#69090=CARTESIAN_POINT('Ctrl Pts',(20.4450494585192,-0.316476177380199,
-3.22147259843938));
#69091=CARTESIAN_POINT('Ctrl Pts',(20.4666801482623,0.0196649616159529,
-3.22285846637663));
#69092=CARTESIAN_POINT('Ctrl Pts',(20.4687786128436,0.0526185201255753,
-3.22248892931092));
#69093=CARTESIAN_POINT('Ctrl Pts',(20.4713690994219,0.0938075203182971,
-3.22139500005276));
#69094=CARTESIAN_POINT('Ctrl Pts',(20.471886002397,0.102052166157655,-3.22114435506224));
#69095=CARTESIAN_POINT('Ctrl Pts',(20.4726952759532,0.115002400335194,-3.22070088456942));
#69096=CARTESIAN_POINT('Ctrl Pts',(20.4729888222946,0.119708612528294,-3.22052939572251));
#69097=CARTESIAN_POINT('Ctrl Pts',(20.4735315705697,0.128426765546993,-3.2201925797929));
#69098=CARTESIAN_POINT('Ctrl Pts',(20.4737809253533,0.132438737043239,-3.22003007226678));
#69099=CARTESIAN_POINT('Ctrl Pts',(20.4743392504605,0.141436559095113,-3.21964876469827));
#69100=CARTESIAN_POINT('Ctrl Pts',(20.4746479881176,0.146422194650503,-3.21942588204558));
#69101=CARTESIAN_POINT('Ctrl Pts',(20.4755609918976,0.161194930861298,-3.2187310800625));
#69102=CARTESIAN_POINT('Ctrl Pts',(20.4761634266426,0.170980527275454,-3.21822610091376));
#69103=CARTESIAN_POINT('Ctrl Pts',(20.4810991872886,0.251449724622588,-3.21370547268204));
#69104=CARTESIAN_POINT('Ctrl Pts',(20.4853106083577,0.321991810443162,-3.20740593565496));
#69105=CARTESIAN_POINT('Ctrl Pts',(20.496282031536,0.508658250010303,-3.18451458339333));
#69106=CARTESIAN_POINT('Ctrl Pts',(20.5028950739508,0.624184381902098,-3.1639001265023));
#69107=CARTESIAN_POINT('Ctrl Pts',(20.5250913678361,1.00984891359085,-3.07312955714131));
#69108=CARTESIAN_POINT('Ctrl Pts',(20.5404931395569,1.27188178392693,-2.97425952398424));
#69109=CARTESIAN_POINT('Ctrl Pts',(20.557596185019,1.52391608826407,-2.83969077283677));
#69110=CARTESIAN_POINT('Ctrl Pts',(20.558004444565,1.52991261219465,-2.83646458243286));
#69111=CARTESIAN_POINT('Ctrl Pts',(20.5600625132314,1.56004156827878,-2.82013156283506));
#69112=CARTESIAN_POINT('Ctrl Pts',(20.5617221892684,1.5840154347542,-2.80673596150411));
#69113=CARTESIAN_POINT('Ctrl Pts',(20.5640657474983,1.61740036562644,-2.78751788422871));
#69114=CARTESIAN_POINT('Ctrl Pts',(20.5647404113197,1.62695753629128,-2.78195058689767));
#69115=CARTESIAN_POINT('Ctrl Pts',(20.5658321843213,1.64233587426611,-2.77288596107061));
#69116=CARTESIAN_POINT('Ctrl Pts',(20.5662481782628,1.64817503308301,-2.76941920557493));
#69117=CARTESIAN_POINT('Ctrl Pts',(20.5671141131238,1.66028724804923,-2.76217621225702));
#69118=CARTESIAN_POINT('Ctrl Pts',(20.5675641610904,1.6665584735681,-2.75839700303662));
#69119=CARTESIAN_POINT('Ctrl Pts',(20.5686246873165,1.68128017980863,-2.74945677654805));
#69120=CARTESIAN_POINT('Ctrl Pts',(20.5692358110827,1.68971982560838,-2.74427814125343));
#69121=CARTESIAN_POINT('Ctrl Pts',(20.571239436272,1.71724622852086,-2.72721259814539));
#69122=CARTESIAN_POINT('Ctrl Pts',(20.5726378687498,1.73623213424713,-2.71516502252512));
#69123=CARTESIAN_POINT('Ctrl Pts',(20.5759341089152,1.78044797794668,-2.68645429978394));
#69124=CARTESIAN_POINT('Ctrl Pts',(20.5778377420047,1.80557222550908,-2.66963303570567));
#69125=CARTESIAN_POINT('Ctrl Pts',(20.584592689814,1.89326706555523,-2.60911509350287));
#69126=CARTESIAN_POINT('Ctrl Pts',(20.5895128009219,1.95451471701099,-2.56355465203845));
#69127=CARTESIAN_POINT('Ctrl Pts',(20.6150868324603,2.25971459528024,-2.31922602001072));
#69128=CARTESIAN_POINT('Ctrl Pts',(20.6369653338288,2.47518190792737,-2.08771416490546));
#69129=CARTESIAN_POINT('Ctrl Pts',(20.6614812495578,2.68773441454902,-1.77927026347234));
#69130=CARTESIAN_POINT('Ctrl Pts',(20.6653497931549,2.72040261424747,-1.7289099694471));
#69131=CARTESIAN_POINT('Ctrl Pts',(20.6697624388816,2.75685443694016,-1.66912288949575));
#69132=CARTESIAN_POINT('Ctrl Pts',(20.6703903284589,2.76202157072408,-1.6605584770816));
#69133=CARTESIAN_POINT('Ctrl Pts',(20.6713345247138,2.7697631777192,-1.6475908211724));
#69134=CARTESIAN_POINT('Ctrl Pts',(20.6716527168457,2.77236715022545,-1.64320539186909));
#69135=CARTESIAN_POINT('Ctrl Pts',(20.6722206860638,2.77700658079784,-1.63534956474592));
#69136=CARTESIAN_POINT('Ctrl Pts',(20.6724707174041,2.7790459537,-1.63188153263245));
#69137=CARTESIAN_POINT('Ctrl Pts',(20.6730074491048,2.78341737050781,-1.62441580984607));
#69138=CARTESIAN_POINT('Ctrl Pts',(20.6732940105666,2.78574729038131,-1.62041692674965));
#69139=CARTESIAN_POINT('Ctrl Pts',(20.674080911474,2.7921339761048,-1.60940085730269));
#69140=CARTESIAN_POINT('Ctrl Pts',(20.6745801043479,2.79617292994234,-1.60237330519178));
#69141=CARTESIAN_POINT('Ctrl Pts',(20.6772377495427,2.81760488859402,-1.56475510807865));
#69142=CARTESIAN_POINT('Ctrl Pts',(20.6793668532931,2.83452329994665,-1.53389496366684));
#69143=CARTESIAN_POINT('Ctrl Pts',(20.6855470925973,2.88273761755558,-1.44242619997023));
#69144=CARTESIAN_POINT('Ctrl Pts',(20.6895261996228,2.91262036829977,-1.3810913659796));
#69145=CARTESIAN_POINT('Ctrl Pts',(20.7072058812553,3.03852030736128,-1.10038229044601));
#69146=CARTESIAN_POINT('Ctrl Pts',(20.7202345232669,3.11185683159875,-0.871668655335678));
#69147=CARTESIAN_POINT('Ctrl Pts',(20.7421869196752,3.18810132597748,-0.493495222717645));
#69148=CARTESIAN_POINT('Ctrl Pts',(20.7506972944325,3.2072144095353,-0.348274410371027));
#69149=CARTESIAN_POINT('Ctrl Pts',(20.7606998438942,3.21760665767313,-0.183021589053609));
#69150=CARTESIAN_POINT('Ctrl Pts',(20.761870168043,3.21864427205975,-0.163763642078358));
#69151=CARTESIAN_POINT('Ctrl Pts',(20.763613026169,3.2199260354401,-0.135205096803927));
#69152=CARTESIAN_POINT('Ctrl Pts',(20.7641813925414,3.22030287357123,-0.125910648938842));
#69153=CARTESIAN_POINT('Ctrl Pts',(20.7651938759245,3.22090114261816,-0.109387795067659));
#69154=CARTESIAN_POINT('Ctrl Pts',(20.7656374899645,3.22113849330376,-0.102160001131859));
#69155=CARTESIAN_POINT('Ctrl Pts',(20.7665713487827,3.22158615168371,-0.0869694189091101));
#69156=CARTESIAN_POINT('Ctrl Pts',(20.7670617535443,3.22179126850761,-0.0790065370297626));
#69157=CARTESIAN_POINT('Ctrl Pts',(20.7683541261965,3.22225313285796,-0.0580599140718856));
#69158=CARTESIAN_POINT('Ctrl Pts',(20.7691576251502,3.22246092477963,-0.0450753388185116));
#69159=CARTESIAN_POINT('Ctrl Pts',(20.7727845520275,3.22304280702763,0.0133592911564714));
#69160=CARTESIAN_POINT('Ctrl Pts',(20.7756355201495,3.22253383567223,0.0588110855641397));
#69161=CARTESIAN_POINT('Ctrl Pts',(20.7832995788939,3.2186230549001,0.17966166966234));
#69162=CARTESIAN_POINT('Ctrl Pts',(20.788163043942,3.21353380909361,0.254973863837604));
#69163=CARTESIAN_POINT('Ctrl Pts',(20.8133436301556,3.17409469394364,0.638068899788148));
#69164=CARTESIAN_POINT('Ctrl Pts',(20.8348469237467,3.09816268723872,0.939869210308037));
#69165=CARTESIAN_POINT('Ctrl Pts',(20.8594938006782,2.95531436473915,1.28707849822721));
#69166=CARTESIAN_POINT('Ctrl Pts',(20.8637490556735,2.92839638292575,1.34720084527485));
#69167=CARTESIAN_POINT('Ctrl Pts',(20.8685556706488,2.89511940848214,1.41580686341731));
#69168=CARTESIAN_POINT('Ctrl Pts',(20.8692078684748,2.89054087453619,1.4251311951832));
#69169=CARTESIAN_POINT('Ctrl Pts',(20.870176817732,2.88364264668812,1.43900964723685));
#69170=CARTESIAN_POINT('Ctrl Pts',(20.8704956517355,2.88135712920066,1.44358053932054));
#69171=CARTESIAN_POINT('Ctrl Pts',(20.8710643205662,2.87725249090699,1.45174097536426));
#69172=CARTESIAN_POINT('Ctrl Pts',(20.8713144122351,2.87543751686951,1.45533255415432));
#69173=CARTESIAN_POINT('Ctrl Pts',(20.8718507778918,2.87152382092332,1.46304130611008));
#69174=CARTESIAN_POINT('Ctrl Pts',(20.8721369148771,2.86942297704463,1.46715735248848));
#69175=CARTESIAN_POINT('Ctrl Pts',(20.872921462592,2.86362728553628,1.47845240753759));
#69176=CARTESIAN_POINT('Ctrl Pts',(20.8734187381169,2.85991427077189,1.48562213195255));
#69177=CARTESIAN_POINT('Ctrl Pts',(20.8760485056602,2.84007130371609,1.52358824330249));
#69178=CARTESIAN_POINT('Ctrl Pts',(20.878152373962,2.82347003969167,1.55413748202821));
#69179=CARTESIAN_POINT('Ctrl Pts',(20.8842379371014,2.77343162072368,1.64276753906209));
#69180=CARTESIAN_POINT('Ctrl Pts',(20.8881502039223,2.7386720319103,1.70008377590273));
#69181=CARTESIAN_POINT('Ctrl Pts',(20.9060935679682,2.56864360571242,1.96168359448551));
#69182=CARTESIAN_POINT('Ctrl Pts',(20.9194077657512,2.41215017058785,2.15120372201841));
#69183=CARTESIAN_POINT('Ctrl Pts',(20.9368538966456,2.19158867555922,2.36364232977687));
#69184=CARTESIAN_POINT('Ctrl Pts',(20.9403743784684,2.14629248909059,2.40484801886621));
#69185=CARTESIAN_POINT('Ctrl Pts',(20.9449700440704,2.08644489735947,2.45625275717279));
#69186=CARTESIAN_POINT('Ctrl Pts',(20.9460032546528,2.07294364156569,2.46765770720606));
#69187=CARTESIAN_POINT('Ctrl Pts',(20.9511075231225,2.00604131422766,2.52323576253808));
#69188=CARTESIAN_POINT('Ctrl Pts',(20.9552345537638,1.95132190911437,2.56578685885222));
#69189=CARTESIAN_POINT('Ctrl Pts',(20.9602906969076,1.88381310537646,2.61487411319555));
#69190=CARTESIAN_POINT('Ctrl Pts',(20.9611521193032,1.87229514930295,2.62313349026753));
#69191=CARTESIAN_POINT('Ctrl Pts',(20.9625696396051,1.85331729892081,2.63655358881213));
#69192=CARTESIAN_POINT('Ctrl Pts',(20.9631240044374,1.84588935405468,2.64175932421788));
#69193=CARTESIAN_POINT('Ctrl Pts',(20.9641209057462,1.83252160072759,2.65104395721525));
#69194=CARTESIAN_POINT('Ctrl Pts',(20.9645629958561,1.82658988094671,2.65513443834842));
#69195=CARTESIAN_POINT('Ctrl Pts',(20.9654935220019,1.81409738667375,2.66368751780943));
#69196=CARTESIAN_POINT('Ctrl Pts',(20.9659821164421,1.80753375719032,2.66814584228224));
#69197=CARTESIAN_POINT('Ctrl Pts',(20.9667568400117,1.79712010867691,2.67516321900054));
#69198=CARTESIAN_POINT('Ctrl Pts',(20.9670423576727,1.79328091100523,2.67773831936296));
#69199=CARTESIAN_POINT('Ctrl Pts',(20.9673281879432,1.78943621037185,2.68030513403046));
#69200=CARTESIAN_POINT('Origin',(-1.72497344927317,0.,0.));
#69201=CARTESIAN_POINT('',(22.4670531482195,1.78943621037803,2.68030513402633));
#69202=CARTESIAN_POINT('',(22.2208495079139,1.78943601979592,2.68030526126352));
#69203=CARTESIAN_POINT('',(-1.72497344927317,1.78943621037804,2.68030513402633));
#69204=CARTESIAN_POINT('',(21.6465734492304,-3.22274996585741,-0.000469111987035887));
#69205=CARTESIAN_POINT('Ctrl Pts',(21.6465734492731,-3.22274996585731,-0.000469112675110201));
#69206=CARTESIAN_POINT('Ctrl Pts',(21.6481278312453,-3.22274632312903,-0.0254942357564947));
#69207=CARTESIAN_POINT('Ctrl Pts',(21.6496822132174,-3.22245120008828,-0.0505169572527867));
#69208=CARTESIAN_POINT('Ctrl Pts',(21.6512365951896,-3.22186473262596,-0.0755328217469976));
#69209=CARTESIAN_POINT('Ctrl Pts',(21.6574088432824,-3.21953594681871,-0.174867557146353));
#69210=CARTESIAN_POINT('Ctrl Pts',(21.6635810913751,-3.21260480812707,-0.274269331810238));
#69211=CARTESIAN_POINT('Ctrl Pts',(21.6697533394679,-3.20105952006451,-0.373276722425059));
#69212=CARTESIAN_POINT('Ctrl Pts',(21.6759172281205,-3.18952986846744,-0.47215002148327));
#69213=CARTESIAN_POINT('Ctrl Pts',(21.6820811167731,-3.17339853837091,-0.570629570496825));
#69214=CARTESIAN_POINT('Ctrl Pts',(21.6882450054258,-3.15270573127254,-0.668254543195374));
#69215=CARTESIAN_POINT('Ctrl Pts',(21.6944023670843,-3.13203483596349,-0.765776139980608));
#69216=CARTESIAN_POINT('Ctrl Pts',(21.7005597287429,-3.10681215609342,-0.862444536922237));
#69217=CARTESIAN_POINT('Ctrl Pts',(21.7067170904014,-3.07712950881661,-0.95780559012259));
#69218=CARTESIAN_POINT('Ctrl Pts',(21.7128699545477,-3.04746854259035,-1.05309698889499));
#69219=CARTESIAN_POINT('Ctrl Pts',(21.719022818694,-3.01335421450438,-1.14708252897496));
#69220=CARTESIAN_POINT('Ctrl Pts',(21.7251756828403,-2.97492886656484,-1.23932070158585));
#69221=CARTESIAN_POINT('Ctrl Pts',(21.7313262159769,-2.93651807605081,-1.3315239298072));
#69222=CARTESIAN_POINT('Ctrl Pts',(21.7374767491134,-2.89379967775345,-1.42198070540096));
#69223=CARTESIAN_POINT('Ctrl Pts',(21.7436272822499,-2.84696477031514,-1.51026790970492));
#69224=CARTESIAN_POINT('Ctrl Pts',(21.7497771304652,-2.80013507839656,-1.59854528237514));
#69225=CARTESIAN_POINT('Ctrl Pts',(21.7559269786804,-2.74918999228949,-1.68465318037131));
#69226=CARTESIAN_POINT('Ctrl Pts',(21.7620768268956,-2.694366881103,-1.76819248740495));
#69227=CARTESIAN_POINT('Ctrl Pts',(21.7682276352747,-2.63953521049007,-1.85174483726922));
#69228=CARTESIAN_POINT('Ctrl Pts',(21.7743784436539,-2.58082455052733,-1.93272743643165));
#69229=CARTESIAN_POINT('Ctrl Pts',(21.780529252033,-2.51851539447775,-2.01077044196462));
#69230=CARTESIAN_POINT('Ctrl Pts',(21.7866866383992,-2.45613960185024,-2.08889691065372));
#69231=CARTESIAN_POINT('Ctrl Pts',(21.7928440247654,-2.39015789979764,-2.16407716785023));
#69232=CARTESIAN_POINT('Ctrl Pts',(21.7990014111316,-2.32089077774229,-2.23597485681096));
#69233=CARTESIAN_POINT('Ctrl Pts',(21.8051622338685,-2.25158499845486,-2.30791267109472));
#69234=CARTESIAN_POINT('Ctrl Pts',(21.8113230566055,-2.17899046327251,-2.37656397033987));
#69235=CARTESIAN_POINT('Ctrl Pts',(21.8174838793425,-2.10346265252566,-2.44163110070496));
#69236=CARTESIAN_POINT('Ctrl Pts',(21.8236550022592,-2.02780856805557,-2.50680701575122));
#69237=CARTESIAN_POINT('Ctrl Pts',(21.8298261251758,-1.94921175432683,-2.56838652443545));
#69238=CARTESIAN_POINT('Ctrl Pts',(21.8359972480925,-1.8680588202361,-2.62611382210256));
#69239=CARTESIAN_POINT('Ctrl Pts',(21.8406927700381,-1.80631067680886,-2.67003772326466));
#69240=CARTESIAN_POINT('Ctrl Pts',(21.8453882919836,-1.74308331769695,-2.71173226350374));
#69241=CARTESIAN_POINT('Ctrl Pts',(21.8500838139291,-1.67855636729737,-2.75110270333651));
#69242=CARTESIAN_POINT('Ctrl Pts',(21.8562560620219,-1.59373590406534,-2.80285501649537));
#69243=CARTESIAN_POINT('Ctrl Pts',(21.8624283101147,-1.50637050747736,-2.85077203819863));
#69244=CARTESIAN_POINT('Ctrl Pts',(21.8686005582074,-1.41684195245698,-2.89459434882643));
#69245=CARTESIAN_POINT('Ctrl Pts',(21.87476444686,-1.32743465124642,-2.93835730831069));
#69246=CARTESIAN_POINT('Ctrl Pts',(21.8809283355127,-1.23587040140118,-2.9780363901404));
#69247=CARTESIAN_POINT('Ctrl Pts',(21.8870922241653,-1.14255859144916,-3.01341623869085));
#69248=CARTESIAN_POINT('Ctrl Pts',(21.8932495858238,-1.0493455901658,-3.04875862321896));
#69249=CARTESIAN_POINT('Ctrl Pts',(21.8994069474824,-0.954389111677636,
-3.07981067210762));
#69250=CARTESIAN_POINT('Ctrl Pts',(21.9055643091409,-0.85812083235513,-3.10640406250992));
#69251=CARTESIAN_POINT('Ctrl Pts',(21.9117171732872,-0.761922870124273,
-3.13297802834285));
#69252=CARTESIAN_POINT('Ctrl Pts',(21.9178700374335,-0.664415429509654,
-3.15509969531556));
#69253=CARTESIAN_POINT('Ctrl Pts',(21.9240229015799,-0.566046877410062,
-3.17265007447628));
#69254=CARTESIAN_POINT('Ctrl Pts',(21.9301734347164,-0.467715592191445,
-3.19019380468387));
#69255=CARTESIAN_POINT('Ctrl Pts',(21.9363239678529,-0.368524270856346,
-3.20316961200751));
#69256=CARTESIAN_POINT('Ctrl Pts',(21.9424745009895,-0.268932173587789,
-3.2115094657356));
#69257=CARTESIAN_POINT('Ctrl Pts',(21.9486243492047,-0.169351166862188,
-3.21984839074034));
#69258=CARTESIAN_POINT('Ctrl Pts',(21.9547741974199,-0.0693699057953061,
-3.22355235229859));
#69259=CARTESIAN_POINT('Ctrl Pts',(21.9609240456351,0.030547521525458,-3.22260522115705));
#69260=CARTESIAN_POINT('Ctrl Pts',(21.9670748540142,0.130480548761247,-3.22165794214175));
#69261=CARTESIAN_POINT('Ctrl Pts',(21.9732256623934,0.230349288058754,-3.21605813219087));
#69262=CARTESIAN_POINT('Ctrl Pts',(21.9793764707725,0.329690958671108,-3.20584176687973));
#69263=CARTESIAN_POINT('Ctrl Pts',(21.9855338571387,0.429138870314394,-3.19561447566834));
#69264=CARTESIAN_POINT('Ctrl Pts',(21.9916912435049,0.528058154734965,-3.18076081458409));
#69265=CARTESIAN_POINT('Ctrl Pts',(21.9978486298711,0.625992573729931,-3.16136851065088));
#69266=CARTESIAN_POINT('Ctrl Pts',(22.004009452608,0.723981648865477,-3.14196538408248));
#69267=CARTESIAN_POINT('Ctrl Pts',(22.010170275345,0.820984342240742,-3.11801867440618));
#69268=CARTESIAN_POINT('Ctrl Pts',(22.0163310980819,0.916558052936471,-3.08966647036493));
#69269=CARTESIAN_POINT('Ctrl Pts',(22.0225022209986,1.01229155177081,-3.06126686473306));
#69270=CARTESIAN_POINT('Ctrl Pts',(22.0286733439153,1.10659088535593,-3.02844719527263));
#69271=CARTESIAN_POINT('Ctrl Pts',(22.034844466832,1.1990318251467,-2.99139436463756));
#69272=CARTESIAN_POINT('Ctrl Pts',(22.0395399887776,1.26936885575224,-2.96320137905889));
#69273=CARTESIAN_POINT('Ctrl Pts',(22.0442355107232,1.33863035514316,-2.93255862578227));
#69274=CARTESIAN_POINT('Ctrl Pts',(22.0489310326689,1.40663950287093,-2.89956597984302));
#69275=CARTESIAN_POINT('Ctrl Pts',(22.0551032807616,1.49603730299087,-2.85619725569856));
#69276=CARTESIAN_POINT('Ctrl Pts',(22.0612755288544,1.58358489327371,-2.80861392956884));
#69277=CARTESIAN_POINT('Ctrl Pts',(22.0674477769472,1.66885761801247,-2.75699688307799));
#69278=CARTESIAN_POINT('Ctrl Pts',(22.0736116655998,1.75401485286383,-2.70544974460175));
#69279=CARTESIAN_POINT('Ctrl Pts',(22.0797755542524,1.83690297764013,-2.6498799672432));
#69280=CARTESIAN_POINT('Ctrl Pts',(22.0859394429051,1.91711947270133,-2.59051548729));
#69281=CARTESIAN_POINT('Ctrl Pts',(22.0920968045636,1.99725102583408,-2.53121386888922));
#69282=CARTESIAN_POINT('Ctrl Pts',(22.0982541662222,2.07471622635874,-2.46812579351227));
#69283=CARTESIAN_POINT('Ctrl Pts',(22.1044115278807,2.1491400677625,-2.40152337728322));
#69284=CARTESIAN_POINT('Ctrl Pts',(22.110564392027,2.22350954787386,-2.33496960935496));
#69285=CARTESIAN_POINT('Ctrl Pts',(22.1167172561734,2.29484176286572,-2.2649068929557));
#69286=CARTESIAN_POINT('Ctrl Pts',(22.1228701203197,2.36279418159805,-2.19164805977292));
#69287=CARTESIAN_POINT('Ctrl Pts',(22.1290206534562,2.43072085658761,-2.1184169806656));
#69288=CARTESIAN_POINT('Ctrl Pts',(22.1351711865928,2.49526998446236,-2.04199250883538));
#69289=CARTESIAN_POINT('Ctrl Pts',(22.1413217197293,2.55613601049785,-1.96272419313976));
#69290=CARTESIAN_POINT('Ctrl Pts',(22.1474715679445,2.61699525851286,-1.88346470473751));
#69291=CARTESIAN_POINT('Ctrl Pts',(22.1536214161597,2.67417195558059,-1.8013623466216));
#69292=CARTESIAN_POINT('Ctrl Pts',(22.1597712643749,2.72740159644865,-1.71679879257569));
#69293=CARTESIAN_POINT('Ctrl Pts',(22.1659220727541,2.78063954795779,-1.63222203578531));
#69294=CARTESIAN_POINT('Ctrl Pts',(22.1720728811332,2.82992898782414,-1.54518368746661));
#69295=CARTESIAN_POINT('Ctrl Pts',(22.1782236895124,2.87504994873398,-1.45609249527107));
#69296=CARTESIAN_POINT('Ctrl Pts',(22.1843810758785,2.92021916429237,-1.36690602442718));
#69297=CARTESIAN_POINT('Ctrl Pts',(22.1905384622447,2.96121080212157,-1.2756627139547));
#69298=CARTESIAN_POINT('Ctrl Pts',(22.1966958486109,2.99785196630828,-1.18279379039694));
#69299=CARTESIAN_POINT('Ctrl Pts',(22.2028566713479,3.03451357953265,-1.08987303769683));
#69300=CARTESIAN_POINT('Ctrl Pts',(22.2090174940849,3.06681974342698,-0.995325276217104));
#69301=CARTESIAN_POINT('Ctrl Pts',(22.2151783168218,3.09464730062386,-0.899597491793666));
#69302=CARTESIAN_POINT('Ctrl Pts',(22.2213494397385,3.12252138226282,-0.80370966163823));
#69303=CARTESIAN_POINT('Ctrl Pts',(22.2275205626552,3.14590179897318,-0.706638290304755));
#69304=CARTESIAN_POINT('Ctrl Pts',(22.2336916855719,3.16471639021537,-0.60884130280574));
#69305=CARTESIAN_POINT('Ctrl Pts',(22.2383872075174,3.17903215207373,-0.534428929691776));
#69306=CARTESIAN_POINT('Ctrl Pts',(22.243082729463,3.1907055967668,-0.459596688545039));
#69307=CARTESIAN_POINT('Ctrl Pts',(22.2477782514085,3.19972513143753,-0.384547325757277));
#69308=CARTESIAN_POINT('Ctrl Pts',(22.2539504995013,3.21158127997964,-0.285895186186295));
#69309=CARTESIAN_POINT('Ctrl Pts',(22.260122747594,3.21889164035863,-0.186520581175701));
#69310=CARTESIAN_POINT('Ctrl Pts',(22.2662949956868,3.22157875612023,-0.0868785394378976));
#69311=CARTESIAN_POINT('Ctrl Pts',(22.2724588843394,3.22426223256224,0.0126285511977798));
#69312=CARTESIAN_POINT('Ctrl Pts',(22.278622772992,3.22233489826665,0.112401928243455));
#69313=CARTESIAN_POINT('Ctrl Pts',(22.2847866616447,3.21577084877965,0.211979741105177));
#69314=CARTESIAN_POINT('Ctrl Pts',(22.2909440233032,3.20921375002044,0.311452110174464));
#69315=CARTESIAN_POINT('Ctrl Pts',(22.2971013849618,3.19802972574339,0.410728895718908));
#69316=CARTESIAN_POINT('Ctrl Pts',(22.3032587466203,3.18224491259648,0.509347502942561));
#69317=CARTESIAN_POINT('Ctrl Pts',(22.3094116107666,3.16647162912644,0.607894076328115));
#69318=CARTESIAN_POINT('Ctrl Pts',(22.3155644749129,3.14610430657407,0.705782999587667));
#69319=CARTESIAN_POINT('Ctrl Pts',(22.3217173390592,3.12122089164884,0.802556981176296));
#69320=CARTESIAN_POINT('Ctrl Pts',(22.3278678721958,3.096346903794,0.899294299986199));
#69321=CARTESIAN_POINT('Ctrl Pts',(22.3340184053323,3.06696033120595,0.994917096198299));
#69322=CARTESIAN_POINT('Ctrl Pts',(22.3401689384688,3.03319000093142,1.08897932980826));
#69323=CARTESIAN_POINT('Ctrl Pts',(22.346318786684,2.99942343130967,1.1830310886791));
#69324=CARTESIAN_POINT('Ctrl Pts',(22.3524686348992,2.96127422133949,1.27552222162924));
#69325=CARTESIAN_POINT('Ctrl Pts',(22.3586184831144,2.91892041771169,1.36602384955966));
#69326=CARTESIAN_POINT('Ctrl Pts',(22.3647692914936,2.87656000146629,1.45653960733456));
#69327=CARTESIAN_POINT('Ctrl Pts',(22.3709200998727,2.82999387180943,1.54506484966208));
#69328=CARTESIAN_POINT('Ctrl Pts',(22.3770709082518,2.77944693233037,1.63119352403671));
#69329=CARTESIAN_POINT('Ctrl Pts',(22.383228294618,2.72884593538555,1.71741430879258));
#69330=CARTESIAN_POINT('Ctrl Pts',(22.3893856809842,2.67425584755697,1.80123303217076));
#69331=CARTESIAN_POINT('Ctrl Pts',(22.3955430673504,2.61594593386626,1.88227108398036));
#69332=CARTESIAN_POINT('Ctrl Pts',(22.4017038900874,2.55760347804303,1.96335436225068));
#69333=CARTESIAN_POINT('Ctrl Pts',(22.4078647128243,2.49553733188193,2.04165353802593));
#69334=CARTESIAN_POINT('Ctrl Pts',(22.4140255355613,2.43005691140302,2.11682332041255));
#69335=CARTESIAN_POINT('Ctrl Pts',(22.420196658478,2.36446701526989,2.19211877794061));
#69336=CARTESIAN_POINT('Ctrl Pts',(22.4263677813946,2.2954517431091,2.26427407730709));
#69337=CARTESIAN_POINT('Ctrl Pts',(22.4325389043113,2.22335728758057,2.33298091167981));
#69338=CARTESIAN_POINT('Ctrl Pts',(22.4372344262569,2.16850161501311,2.38525899023476));
#69339=CARTESIAN_POINT('Ctrl Pts',(22.4419299482026,2.11186401776716,2.43554135498066));
#69340=CARTESIAN_POINT('Ctrl Pts',(22.4466254701482,2.05360877953829,2.48370862685285));
#69341=CARTESIAN_POINT('Ctrl Pts',(22.4527985050484,1.97702269967905,2.5470324178519));
#69342=CARTESIAN_POINT('Ctrl Pts',(22.4589715399486,1.89737013881085,2.60692201962735));
#69343=CARTESIAN_POINT('Ctrl Pts',(22.4651445748488,1.81499212238597,2.66306611975311));
#69344=CARTESIAN_POINT('Ctrl Pts',(22.4657807659724,1.80650226874485,2.66885231385642));
#69345=CARTESIAN_POINT('Ctrl Pts',(22.4664169570959,1.79798349964587,2.67459875801627));
#69346=CARTESIAN_POINT('Ctrl Pts',(22.4670531482195,1.78943621037803,2.68030513402633));
#69347=CARTESIAN_POINT('Ctrl Pts',(21.2168443958857,1.78943621037803,2.68030513402633));
#69348=CARTESIAN_POINT('Ctrl Pts',(21.2230150525931,1.70635126714696,2.73577464160868));
#69349=CARTESIAN_POINT('Ctrl Pts',(21.2291857093005,1.62077675188503,2.7873158961107));
#69350=CARTESIAN_POINT('Ctrl Pts',(21.2353563660079,1.53312715272033,2.83472021478164));
#69351=CARTESIAN_POINT('Ctrl Pts',(21.2414182965754,1.44702192768618,2.88128927574313));
#69352=CARTESIAN_POINT('Ctrl Pts',(21.2474802271428,1.3589145411085,2.92386591393451));
#69353=CARTESIAN_POINT('Ctrl Pts',(21.2535421577103,1.26921500444823,2.96229823532059));
#69354=CARTESIAN_POINT('Ctrl Pts',(21.259714405803,1.1778830784366,3.00142996402264));
#69355=CARTESIAN_POINT('Ctrl Pts',(21.2658866538958,1.08457897127673,3.03640276884295));
#69356=CARTESIAN_POINT('Ctrl Pts',(21.2720589019886,0.989717541342602,3.06701430561691));
#69357=CARTESIAN_POINT('Ctrl Pts',(21.2782227906412,0.89498458784571,3.09758438337864));
#69358=CARTESIAN_POINT('Ctrl Pts',(21.2843866792939,0.798698913535267,3.12380480113236));
#69359=CARTESIAN_POINT('Ctrl Pts',(21.2905505679465,0.701296426591066,3.14552076523914));
#69360=CARTESIAN_POINT('Ctrl Pts',(21.296707929605,0.603997079968211,3.16721373412693));
#69361=CARTESIAN_POINT('Ctrl Pts',(21.3028652912636,0.505583693465033,3.18441163818673));
#69362=CARTESIAN_POINT('Ctrl Pts',(21.3090226529221,0.406507530472406,3.19700941352528));
#69363=CARTESIAN_POINT('Ctrl Pts',(21.3151755170684,0.307503735529606,3.2095979870901));
#69364=CARTESIAN_POINT('Ctrl Pts',(21.3213283812148,0.207838556199264,3.21759305769202));
#69365=CARTESIAN_POINT('Ctrl Pts',(21.3274812453611,0.107972742892041,3.22094077084512));
#69366=CARTESIAN_POINT('Ctrl Pts',(21.3336317784976,0.00814476370253209,
3.22428721571863));
#69367=CARTESIAN_POINT('Ctrl Pts',(21.3397823116341,-0.0918832647827476,
3.222989787007));
#69368=CARTESIAN_POINT('Ctrl Pts',(21.3459328447707,-0.191647074731872,
3.21704662093149));
#69369=CARTESIAN_POINT('Ctrl Pts',(21.3520826929859,-0.291399775016203,
3.21110411668498));
#69370=CARTESIAN_POINT('Ctrl Pts',(21.3582325412011,-0.390887881655189,
3.20051692946857));
#69371=CARTESIAN_POINT('Ctrl Pts',(21.3643823894163,-0.489649747289857,
3.18533525511507));
#69372=CARTESIAN_POINT('Ctrl Pts',(21.3705331977954,-0.588427032423949,
3.17015121047606));
#69373=CARTESIAN_POINT('Ctrl Pts',(21.3766840061746,-0.686477421965865,
3.15037131990363));
#69374=CARTESIAN_POINT('Ctrl Pts',(21.3828348145537,-0.783347990602642,
3.12609716549547));
#69375=CARTESIAN_POINT('Ctrl Pts',(21.3889922009199,-0.880322157548261,
3.10179705107303));
#69376=CARTESIAN_POINT('Ctrl Pts',(21.3951495872861,-0.976113561814008,
3.07299318073088));
#69377=CARTESIAN_POINT('Ctrl Pts',(21.4013069736523,-1.07028313148713,3.03983742673093));
#69378=CARTESIAN_POINT('Ctrl Pts',(21.4074677963893,-1.16450525617911,3.00666316886308));
#69379=CARTESIAN_POINT('Ctrl Pts',(21.4136286191262,-1.25710334114861,2.9691323537059));
#69380=CARTESIAN_POINT('Ctrl Pts',(21.4197894418632,-1.34765899203866,2.92744475672511));
#69381=CARTESIAN_POINT('Ctrl Pts',(21.4259605647799,-1.43836604145444,2.88568746292626));
#69382=CARTESIAN_POINT('Ctrl Pts',(21.4321316876966,-1.52702345013386,2.83975970547664));
#69383=CARTESIAN_POINT('Ctrl Pts',(21.4383028106132,-1.61323796734748,2.7899069560128));
#69384=CARTESIAN_POINT('Ctrl Pts',(21.4429983325588,-1.67883739926089,2.7519746895008));
#69385=CARTESIAN_POINT('Ctrl Pts',(21.4476938545044,-1.74302304664015,2.71177100438844));
#69386=CARTESIAN_POINT('Ctrl Pts',(21.4523893764499,-1.80563413322286,2.66941996310819));
#69387=CARTESIAN_POINT('Ctrl Pts',(21.4585372899088,-1.88761171661731,2.61396914428544));
#69388=CARTESIAN_POINT('Ctrl Pts',(21.4646852033676,-1.96718249968798,2.55463705375598));
#69389=CARTESIAN_POINT('Ctrl Pts',(21.4708331168264,-2.04395372661063,2.49166023485838));
#69390=CARTESIAN_POINT('Ctrl Pts',(21.4769726892617,-2.12062079614558,2.42876885814016));
#69391=CARTESIAN_POINT('Ctrl Pts',(21.4831122616971,-2.1944955217772,2.36224285512097));
#69392=CARTESIAN_POINT('Ctrl Pts',(21.4892518341324,-2.26521360153258,2.29236229726712));
#69393=CARTESIAN_POINT('Ctrl Pts',(21.4953849289502,-2.33585706946764,2.2225554675977));
#69394=CARTESIAN_POINT('Ctrl Pts',(21.501518023768,-2.40335020165196,2.14940142452263));
#69395=CARTESIAN_POINT('Ctrl Pts',(21.5076511185858,-2.46736211538117,2.0732201412493));
#69396=CARTESIAN_POINT('Ctrl Pts',(21.5137798105395,-2.53132807584215,1.99709354746641));
#69397=CARTESIAN_POINT('Ctrl Pts',(21.5199085024933,-2.59181750451994,1.91794436790151));
#69398=CARTESIAN_POINT('Ctrl Pts',(21.5260371944471,-2.64853740050429,1.83612831812757));
#69399=CARTESIAN_POINT('Ctrl Pts',(21.5321636552663,-2.70523664775598,1.75434205327671));
#69400=CARTESIAN_POINT('Ctrl Pts',(21.5382901160854,-2.75816883919948,1.66989120679491));
#69401=CARTESIAN_POINT('Ctrl Pts',(21.5444165769046,-2.80708278322244,1.58316259766209));
#69402=CARTESIAN_POINT('Ctrl Pts',(21.5505424801101,-2.855992275232,1.49644188233004));
#69403=CARTESIAN_POINT('Ctrl Pts',(21.5566683833156,-2.90088403178773,1.40744419831191));
#69404=CARTESIAN_POINT('Ctrl Pts',(21.5627942865211,-2.94155207588588,1.31658229797894));
#69405=CARTESIAN_POINT('Ctrl Pts',(21.5689213047369,-2.98222752220502,1.22570385935696));
#69406=CARTESIAN_POINT('Ctrl Pts',(21.5750483229527,-3.01867755048412,1.13296093063977));
#69407=CARTESIAN_POINT('Ctrl Pts',(21.5811753411685,-3.05074414799851,1.03878665083492));
#69408=CARTESIAN_POINT('Ctrl Pts',(21.5873089114137,-3.08284503646537,0.944511664188625));
#69409=CARTESIAN_POINT('Ctrl Pts',(21.593442481659,-3.11055299542423,0.848802686451053));
#69410=CARTESIAN_POINT('Ctrl Pts',(21.5995760519042,-3.13375984553868,0.752108232230822));
#69411=CARTESIAN_POINT('Ctrl Pts',(21.6057132516376,-3.1569804281099,0.655356559887253));
#69412=CARTESIAN_POINT('Ctrl Pts',(21.611850451371,-3.17569451746197,0.557618680284896));
#69413=CARTESIAN_POINT('Ctrl Pts',(21.6179876511044,-3.18984542193015,0.459351441372813));
#69414=CARTESIAN_POINT('Ctrl Pts',(21.6241346487006,-3.20401891790996,0.36092732164257));
#69415=CARTESIAN_POINT('Ctrl Pts',(21.6302816462967,-3.21361464287684,0.261972591016499));
#69416=CARTESIAN_POINT('Ctrl Pts',(21.6364286438928,-3.21862793008776,0.16294726189478));
#69417=CARTESIAN_POINT('Ctrl Pts',(21.639810245672,-3.2213858522582,0.108471198758849));
#69418=CARTESIAN_POINT('Ctrl Pts',(21.6431918474512,-3.2227578907038,0.0539737484253642));
#69419=CARTESIAN_POINT('Ctrl Pts',(21.6465734492304,-3.22274996585741,-0.000469111987035492));
#69420=CARTESIAN_POINT('',(21.3984065856094,-3.22274887336959,-0.00269475323696564));
#69421=CARTESIAN_POINT('Ctrl Pts',(20.9673281879432,1.78943621037185,2.68030513403046));
#69422=CARTESIAN_POINT('Ctrl Pts',(20.9678519537231,1.78239104114818,2.68500865854972));
#69423=CARTESIAN_POINT('Ctrl Pts',(20.9683767692861,1.77532739395979,2.6896843611713));
#69424=CARTESIAN_POINT('Ctrl Pts',(20.9698744965502,1.75515725249851,2.70292169002813));
#69425=CARTESIAN_POINT('Ctrl Pts',(20.9708499289186,1.74200684879726,2.71141563914688));
#69426=CARTESIAN_POINT('Ctrl Pts',(20.973754948643,1.70280415933879,2.73633404933602));
#69427=CARTESIAN_POINT('Ctrl Pts',(20.9756946761167,1.67657833274058,2.75248088512964));
#69428=CARTESIAN_POINT('Ctrl Pts',(20.9826153551802,1.5828538307409,2.80834913442632));
#69429=CARTESIAN_POINT('Ctrl Pts',(20.9876688686059,1.51414740036302,2.84598087202798));
#69430=CARTESIAN_POINT('Ctrl Pts',(21.0068117095735,1.2528231808831,2.97697020993401));
#69431=CARTESIAN_POINT('Ctrl Pts',(21.0213819277774,1.05244110936447,3.05356635293571));
#69432=CARTESIAN_POINT('Ctrl Pts',(21.046228958345,0.697074829497055,3.15024077252431));
#69433=CARTESIAN_POINT('Ctrl Pts',(21.0565237049827,0.545435375082559,3.18000671247934));
#69434=CARTESIAN_POINT('Ctrl Pts',(21.0670319800635,0.380291278217971,3.20025636091708));
#69435=CARTESIAN_POINT('Ctrl Pts',(21.0677881914932,0.368344508664027,3.20165341121864));
#69436=CARTESIAN_POINT('Ctrl Pts',(21.068876548389,0.351055409271595,3.20357713689932));
#69437=CARTESIAN_POINT('Ctrl Pts',(21.0692116299518,0.345719320114563,3.20415738145569));
#69438=CARTESIAN_POINT('Ctrl Pts',(21.0697993577351,0.336336263142779,3.20515397933855));
#69439=CARTESIAN_POINT('Ctrl Pts',(21.070052323158,0.332289924608085,3.20557600439013));
#69440=CARTESIAN_POINT('Ctrl Pts',(21.0705797549374,0.323836928368797,3.20644145759184));
#69441=CARTESIAN_POINT('Ctrl Pts',(21.0708541399769,0.319430161616614,3.20688346366882));
#69442=CARTESIAN_POINT('Ctrl Pts',(21.0715739424613,0.307845857021995,3.20802127352615));
#69443=CARTESIAN_POINT('Ctrl Pts',(21.0720185183005,0.300666820944817,3.20870207844611));
#69444=CARTESIAN_POINT('Ctrl Pts',(21.0739952453701,0.26864236383407,3.2116306114496));
#69445=CARTESIAN_POINT('Ctrl Pts',(21.0755130282646,0.243772813990065,3.21361397938985));
#69446=CARTESIAN_POINT('Ctrl Pts',(21.0882704438399,0.0326447176733997,
3.2279865072295));
#69447=CARTESIAN_POINT('Ctrl Pts',(21.0987407651758,-0.154368853068181,
3.22446149910762));
#69448=CARTESIAN_POINT('Ctrl Pts',(21.1216091184046,-0.561055231750271,
3.18130941823188));
#69449=CARTESIAN_POINT('Ctrl Pts',(21.1339621701854,-0.779023881877673,
3.13506357217085));
#69450=CARTESIAN_POINT('Ctrl Pts',(21.147853582335,-1.00363680752323,3.06251881433963));
#69451=CARTESIAN_POINT('Ctrl Pts',(21.1486688813881,-1.01675257093334,3.0581894203909));
#69452=CARTESIAN_POINT('Ctrl Pts',(21.1511575286567,-1.0565769869764,3.04475923543864));
#69453=CARTESIAN_POINT('Ctrl Pts',(21.152838833581,-1.08319380441311,3.03539204063635));
#69454=CARTESIAN_POINT('Ctrl Pts',(21.156281573473,-1.13707646557409,3.01563027823277));
#69455=CARTESIAN_POINT('Ctrl Pts',(21.1580436226883,-1.16433092019963,3.00521251935973));
#69456=CARTESIAN_POINT('Ctrl Pts',(21.1605081648904,-1.20198224083631,2.99023159652657));
#69457=CARTESIAN_POINT('Ctrl Pts',(21.1612001154945,-1.21250264174925,2.98598118660121));
#69458=CARTESIAN_POINT('Ctrl Pts',(21.1623125170718,-1.22933326762929,2.97907773212496));
#69459=CARTESIAN_POINT('Ctrl Pts',(21.1627317700714,-1.23565793130111,2.97645995985338));
#69460=CARTESIAN_POINT('Ctrl Pts',(21.163598848394,-1.24869955256265,2.97101331364428));
#69461=CARTESIAN_POINT('Ctrl Pts',(21.164046762773,-1.25541534443376,2.96818176565912));
#69462=CARTESIAN_POINT('Ctrl Pts',(21.1650805506339,-1.27086616197899,2.96160549100909));
#69463=CARTESIAN_POINT('Ctrl Pts',(21.1656669641665,-1.27959431115376,2.95784487115205));
#69464=CARTESIAN_POINT('Ctrl Pts',(21.1675209926088,-1.30707422927504,2.9458604483344));
#69465=CARTESIAN_POINT('Ctrl Pts',(21.1687933954435,-1.32576404059374,2.93749663818966));
#69466=CARTESIAN_POINT('Ctrl Pts',(21.1717680491982,-1.36905842856939,2.91762478032248));
#69467=CARTESIAN_POINT('Ctrl Pts',(21.1734748522124,-1.39359945035681,2.90598276643642));
#69468=CARTESIAN_POINT('Ctrl Pts',(21.1793476837579,-1.47700437773042,2.8651168303697));
#69469=CARTESIAN_POINT('Ctrl Pts',(21.1835642172386,-1.53511703010977,2.83440489336424));
#69470=CARTESIAN_POINT('Ctrl Pts',(21.196526801783,-1.70846614002117,2.73589648621368));
#69471=CARTESIAN_POINT('Ctrl Pts',(21.2054408652303,-1.82045272536734,2.66269259696062));
#69472=CARTESIAN_POINT('Ctrl Pts',(21.2245656616602,-2.04772807408802,2.49307242815482));
#69473=CARTESIAN_POINT('Ctrl Pts',(21.2347806636282,-2.16148944811625,2.39511269166931));
#69474=CARTESIAN_POINT('Ctrl Pts',(21.2460437697052,-2.28144957758011,2.27628267483768));
#69475=CARTESIAN_POINT('Ctrl Pts',(21.2473011018671,-2.29476395691983,2.26285956118005));
#69476=CARTESIAN_POINT('Ctrl Pts',(21.2495655036409,-2.31861475270052,2.23838697522766));
#69477=CARTESIAN_POINT('Ctrl Pts',(21.2505741230767,-2.32919220031012,2.22737835338654));
#69478=CARTESIAN_POINT('Ctrl Pts',(21.2523888155589,-2.34814564999663,2.20736963520577));
#69479=CARTESIAN_POINT('Ctrl Pts',(21.2531960696954,-2.35654909979147,2.19839601705703));
#69480=CARTESIAN_POINT('Ctrl Pts',(21.2579586936655,-2.40597351979519,2.14500913908558));
#69481=CARTESIAN_POINT('Ctrl Pts',(21.2618567675184,-2.44579267031167,2.09949330414281));
#69482=CARTESIAN_POINT('Ctrl Pts',(21.2662990106982,-2.49069513289802,2.04515421901408));
#69483=CARTESIAN_POINT('Ctrl Pts',(21.2669282221285,-2.49704381946209,2.03739789794604));
#69484=CARTESIAN_POINT('Ctrl Pts',(21.2678740130633,-2.50657112729013,2.02564676194547));
#69485=CARTESIAN_POINT('Ctrl Pts',(21.2681924873658,-2.50977654069463,2.02167389481635));
#69486=CARTESIAN_POINT('Ctrl Pts',(21.2687607639403,-2.51549161722652,2.01455594996598));
#69487=CARTESIAN_POINT('Ctrl Pts',(21.2690108216041,-2.5180048335561,2.01141378405463));
#69488=CARTESIAN_POINT('Ctrl Pts',(21.2695473914765,-2.52339430252902,2.00464963206559));
#69489=CARTESIAN_POINT('Ctrl Pts',(21.2698337656224,-2.52626863434576,2.00102617202707));
#69490=CARTESIAN_POINT('Ctrl Pts',(21.2706196279006,-2.53415015079322,1.99104647075088));
#69491=CARTESIAN_POINT('Ctrl Pts',(21.2711179744844,-2.53914125479659,1.98467748688704));
#69492=CARTESIAN_POINT('Ctrl Pts',(21.2737632729568,-2.5655939469439,1.950658952562));
#69493=CARTESIAN_POINT('Ctrl Pts',(21.2758811984931,-2.58662899950123,1.92267867988402));
#69494=CARTESIAN_POINT('Ctrl Pts',(21.2820194295138,-2.64698514081654,1.83961060355968));
#69495=CARTESIAN_POINT('Ctrl Pts',(21.2859688667637,-2.68503358972743,1.78361805399187));
#69496=CARTESIAN_POINT('Ctrl Pts',(21.3025387302631,-2.8394473357266,1.5402276787012));
#69497=CARTESIAN_POINT('Ctrl Pts',(21.3145880491841,-2.93817639072103,1.34234593432749));
#69498=CARTESIAN_POINT('Ctrl Pts',(21.3296145277263,-3.03176495316452,1.09386408300306));
#69499=CARTESIAN_POINT('Ctrl Pts',(21.3321724464895,-3.0467238542468,1.0514803570573));
#69500=CARTESIAN_POINT('Ctrl Pts',(21.3417543123333,-3.09899900316382,0.892872567378146));
#69501=CARTESIAN_POINT('Ctrl Pts',(21.3489062984102,-3.13058609446599,0.77488178170674));
#69502=CARTESIAN_POINT('Ctrl Pts',(21.3573904709786,-3.15913214990817,0.637446161202819));
#69503=CARTESIAN_POINT('Ctrl Pts',(21.3585031433111,-3.16270656563304,0.61946808411316));
#69504=CARTESIAN_POINT('Ctrl Pts',(21.3601840153322,-3.16785160621631,0.592384266764949));
#69505=CARTESIAN_POINT('Ctrl Pts',(21.3607485552872,-3.16953679392388,0.583300460893615));
#69506=CARTESIAN_POINT('Ctrl Pts',(21.3617567435741,-3.17247000074863,0.567101262646638));
#69507=CARTESIAN_POINT('Ctrl Pts',(21.3621999044332,-3.17373320423832,0.559988655876658));
#69508=CARTESIAN_POINT('Ctrl Pts',(21.3630578002243,-3.17612812586379,0.546235361246301));
#69509=CARTESIAN_POINT('Ctrl Pts',(21.3634724333618,-3.17726295870149,0.539595248257126));
#69510=CARTESIAN_POINT('Ctrl Pts',(21.364371520644,-3.17967467608105,0.525212430009469));
#69511=CARTESIAN_POINT('Ctrl Pts',(21.3648562092225,-3.18094411383787,0.517468535506325));
#69512=CARTESIAN_POINT('Ctrl Pts',(21.3660354170185,-3.18395807212842,0.498652379499739));
#69513=CARTESIAN_POINT('Ctrl Pts',(21.3667308679152,-3.18567312596127,0.487575563444652));
#69514=CARTESIAN_POINT('Ctrl Pts',(21.3700816293345,-3.193636698049,0.434305762110385));
#69515=CARTESIAN_POINT('Ctrl Pts',(21.3727615068429,-3.1991047094595,0.392002079868707));
#69516=CARTESIAN_POINT('Ctrl Pts',(21.3829354073375,-3.21650014504525,0.232592244963371));
#69517=CARTESIAN_POINT('Ctrl Pts',(21.3905985113232,-3.22284727235174,0.114984002839084));
#69518=CARTESIAN_POINT('Ctrl Pts',(21.3984065856094,-3.22274887336959,-0.00269475323696564));
#69519=CARTESIAN_POINT('Ctrl Pts',(21.3984063391797,-3.22274887647301,-0.00269103919059044));
#69520=CARTESIAN_POINT('Ctrl Pts',(21.4053592522661,-3.22266137514423,-0.107481341026377));
#69521=CARTESIAN_POINT('Ctrl Pts',(21.4124178111479,-3.21746293090191,-0.212202018047763));
#69522=CARTESIAN_POINT('Ctrl Pts',(21.4333807979378,-3.18702950541372,-0.520610649471097));
#69523=CARTESIAN_POINT('Ctrl Pts',(21.4473461277154,-3.14744181193964,-0.722369300118942));
#69524=CARTESIAN_POINT('Ctrl Pts',(21.4621449334735,-3.08148942459918,-0.944045988770399));
#69525=CARTESIAN_POINT('Ctrl Pts',(21.4638017771352,-3.07373608350206,-0.968992515927787));
#69526=CARTESIAN_POINT('Ctrl Pts',(21.465901937543,-3.06341934535991,-1.000816274256));
#69527=CARTESIAN_POINT('Ctrl Pts',(21.4663607969808,-3.06113489365175,-1.007781953453));
#69528=CARTESIAN_POINT('Ctrl Pts',(21.4670963169926,-3.05742375683328,-1.01896878541024));
#69529=CARTESIAN_POINT('Ctrl Pts',(21.4673738508741,-3.05601206722791,-1.02319482994292));
#69530=CARTESIAN_POINT('Ctrl Pts',(21.4679032413032,-3.05329744066672,-1.03126562080344));
#69531=CARTESIAN_POINT('Ctrl Pts',(21.4681551819514,-3.05199600732065,-1.03511082173638));
#69532=CARTESIAN_POINT('Ctrl Pts',(21.4687357346023,-3.04897514833649,-1.04398099298263));
#69533=CARTESIAN_POINT('Ctrl Pts',(21.4690640394512,-3.04725055335986,-1.04900421109233));
#69534=CARTESIAN_POINT('Ctrl Pts',(21.4699440756777,-3.04258414664137,-1.06248741052325));
#69535=CARTESIAN_POINT('Ctrl Pts',(21.4704944734817,-3.03961944526112,-1.07093950311423));
#69536=CARTESIAN_POINT('Ctrl Pts',(21.4744941835404,-3.01774091469842,-1.13249041130505));
#69537=CARTESIAN_POINT('Ctrl Pts',(21.4778669179693,-2.99747080990373,-1.18510101524148));
#69538=CARTESIAN_POINT('Ctrl Pts',(21.4853849419586,-2.94841071924306,-1.30310910564626));
#69539=CARTESIAN_POINT('Ctrl Pts',(21.4894940635605,-2.91880527371012,-1.36813598206786));
#69540=CARTESIAN_POINT('Ctrl Pts',(21.503106851959,-2.81237145587611,-1.58269839427308));
#69541=CARTESIAN_POINT('Ctrl Pts',(21.5123779091454,-2.72601526013585,-1.72719758130089));
#69542=CARTESIAN_POINT('Ctrl Pts',(21.5285682865577,-2.55959795295014,-1.96185580795392));
#69543=CARTESIAN_POINT('Ctrl Pts',(21.5353785385709,-2.48504409037869,-2.05547375218897));
#69544=CARTESIAN_POINT('Ctrl Pts',(21.5453281150155,-2.37188541426295,-2.1823893349222));
#69545=CARTESIAN_POINT('Ctrl Pts',(21.5483117875878,-2.3374269915095,-2.21925624675754));
#69546=CARTESIAN_POINT('Ctrl Pts',(21.5533295781173,-2.27875291025246,-2.27914842658912));
#69547=CARTESIAN_POINT('Ctrl Pts',(21.5553431669906,-2.25501868789961,-2.30263391933463));
#69548=CARTESIAN_POINT('Ctrl Pts',(21.558071114558,-2.22263794113817,-2.33369449471549));
#69549=CARTESIAN_POINT('Ctrl Pts',(21.5587711233171,-2.21430903133071,-2.34159879579519));
#69550=CARTESIAN_POINT('Ctrl Pts',(21.5598848488642,-2.20102730031208,-2.35406919229624));
#69551=CARTESIAN_POINT('Ctrl Pts',(21.5602973012798,-2.196102045028,-2.35866461065801));
#69552=CARTESIAN_POINT('Ctrl Pts',(21.5611534812305,-2.18586475551129,-2.36815646142));
#69553=CARTESIAN_POINT('Ctrl Pts',(21.5615973059204,-2.18055059632253,-2.37305053689877));
#69554=CARTESIAN_POINT('Ctrl Pts',(21.562610719315,-2.16839997426379,-2.38416537789433));
#69555=CARTESIAN_POINT('Ctrl Pts',(21.5631807902965,-2.16155313789057,-2.39037466242462));
#69556=CARTESIAN_POINT('Ctrl Pts',(21.5646630183904,-2.14372099763495,-2.40640707632165));
#69557=CARTESIAN_POINT('Ctrl Pts',(21.5655770915787,-2.13269495259623,-2.41618438042822));
#69558=CARTESIAN_POINT('Ctrl Pts',(21.5713640473561,-2.06271223297147,-2.47738904126479));
#69559=CARTESIAN_POINT('Ctrl Pts',(21.5763225158118,-2.00197078159039,-2.52672703138993));
#69560=CARTESIAN_POINT('Ctrl Pts',(21.5827236467789,-1.92266092929463,-2.58649125406766));
#69561=CARTESIAN_POINT('Ctrl Pts',(21.584088477052,-1.90569947744807,-2.59901356802136));
#69562=CARTESIAN_POINT('Ctrl Pts',(21.597413646922,-1.7395978438994,-2.71914304562033));
#69563=CARTESIAN_POINT('Ctrl Pts',(21.6097998460538,-1.5816430532419,-2.81395281304634));
#69564=CARTESIAN_POINT('Ctrl Pts',(21.6357801210014,-1.23687823788911,-2.98265540883846));
#69565=CARTESIAN_POINT('Ctrl Pts',(21.6493280160898,-1.04945885391843,-3.05364621893124));
#69566=CARTESIAN_POINT('Ctrl Pts',(21.6629530217962,-0.842154040696891,
-3.11080700940444));
#69567=CARTESIAN_POINT('Ctrl Pts',(21.663900522391,-0.827629739009613,-3.11470266861203));
#69568=CARTESIAN_POINT('Ctrl Pts',(21.6652143998596,-0.807329748057601,
-3.11999543806916));
#69569=CARTESIAN_POINT('Ctrl Pts',(21.6655855777811,-0.801576934557592,
-3.12147837971032));
#69570=CARTESIAN_POINT('Ctrl Pts',(21.6662147252357,-0.791794723459764,
-3.12397117999325));
#69571=CARTESIAN_POINT('Ctrl Pts',(21.6664731638829,-0.787767432375147,
-3.12498916648727));
#69572=CARTESIAN_POINT('Ctrl Pts',(21.6669646767908,-0.78009071428097,-3.12691384275272));
#69573=CARTESIAN_POINT('Ctrl Pts',(21.6671978335483,-0.776441663359776,
-3.12782193327113));
#69574=CARTESIAN_POINT('Ctrl Pts',(21.6677455714612,-0.767851869133542,
-3.129943602204));
#69575=CARTESIAN_POINT('Ctrl Pts',(21.6680598456194,-0.762909807289574,
-3.13115187633723));
#69576=CARTESIAN_POINT('Ctrl Pts',(21.668985398497,-0.748316089810579,-3.13468326030251));
#69577=CARTESIAN_POINT('Ctrl Pts',(21.669594820813,-0.738656431600315,-3.13697350877479));
#69578=CARTESIAN_POINT('Ctrl Pts',(21.6752781307853,-0.648118679711256,
-3.15799809132386));
#69579=CARTESIAN_POINT('Ctrl Pts',(21.6801848949831,-0.566547733442373,
-3.17364712772203));
#69580=CARTESIAN_POINT('Ctrl Pts',(21.6853264511989,-0.478753255741978,
-3.18699641596907));
#69581=CARTESIAN_POINT('Ctrl Pts',(21.6856599324352,-0.473048199826224,
-3.18784821416617));
#69582=CARTESIAN_POINT('Ctrl Pts',(21.692175467515,-0.361382277423468,-3.20421422500349));
#69583=CARTESIAN_POINT('Ctrl Pts',(21.6981945660834,-0.254709649677842,
-3.21445351072554));
#69584=CARTESIAN_POINT('Ctrl Pts',(21.7146124931097,0.0383715430467452,
-3.22790152918358));
#69585=CARTESIAN_POINT('Ctrl Pts',(21.7249462362604,0.224842207452441,-3.22028912312533));
#69586=CARTESIAN_POINT('Ctrl Pts',(21.7397652402321,0.479261986454161,-3.18768834944866));
#69587=CARTESIAN_POINT('Ctrl Pts',(21.7438759175802,0.548602867573561,-3.17648909401384));
#69588=CARTESIAN_POINT('Ctrl Pts',(21.7497509569,0.645480021266316,-3.15757576336131));
#69589=CARTESIAN_POINT('Ctrl Pts',(21.7514575663761,0.67336638113102,-3.1517466267172));
#69590=CARTESIAN_POINT('Ctrl Pts',(21.7540681899878,0.715612245020734,-3.14232964290477));
#69591=CARTESIAN_POINT('Ctrl Pts',(21.7549636882121,0.730030808355567,-3.13901122609289));
#69592=CARTESIAN_POINT('Ctrl Pts',(21.756618990719,0.756545824593602,-3.1327162577687));
#69593=CARTESIAN_POINT('Ctrl Pts',(21.7573778585297,0.768648900581918,-3.12976861720062));
#69594=CARTESIAN_POINT('Ctrl Pts',(21.758616250434,0.78831260068285,-3.12485868719982));
#69595=CARTESIAN_POINT('Ctrl Pts',(21.7590943968964,0.795883792032423,-3.12293892979737));
#69596=CARTESIAN_POINT('Ctrl Pts',(21.7595741792746,0.803459624498735,-3.12098865657142));
#69597=CARTESIAN_POINT('Ctrl Pts',(21.7595749232389,0.803471371750133,-3.12098563236441));
#69598=CARTESIAN_POINT('Ctrl Pts',(21.7595764132522,0.803494899068915,-3.12097957536063));
#69599=CARTESIAN_POINT('Ctrl Pts',(21.7595771592943,0.803506679026253,-3.12097654259178));
#69600=CARTESIAN_POINT('Ctrl Pts',(21.7595786534366,0.803530271336992,-3.12097046857126));
#69601=CARTESIAN_POINT('Ctrl Pts',(21.75957940155,0.803542083896503,-3.12096742726611));
#69602=CARTESIAN_POINT('Ctrl Pts',(21.7595808998809,0.803565742136834,-3.12096133598507));
#69603=CARTESIAN_POINT('Ctrl Pts',(21.7595816500864,0.803577587626535,-3.12095828605798));
#69604=CARTESIAN_POINT('Ctrl Pts',(21.7595831525948,0.803601311620237,-3.12095217755939));
#69605=CARTESIAN_POINT('Ctrl Pts',(21.7595839048972,0.80361319011538,-3.12094911898977));
#69606=CARTESIAN_POINT('Ctrl Pts',(21.7595854116088,0.803636980266337,-3.12094299316724));
#69607=CARTESIAN_POINT('Ctrl Pts',(21.7595861660175,0.803648891915093,-3.12093992591574));
#69608=CARTESIAN_POINT('Ctrl Pts',(21.7595876769495,0.80367274849331,-3.12093378269731));
#69609=CARTESIAN_POINT('Ctrl Pts',(21.7595884334747,0.803684693453638,-3.12093070672203));
#69610=CARTESIAN_POINT('Ctrl Pts',(21.7595899486348,0.803708616578942,-3.12092454607441));
#69611=CARTESIAN_POINT('Ctrl Pts',(21.7595907072781,0.803720594876109,-3.12092146136762));
#69612=CARTESIAN_POINT('Ctrl Pts',(21.7595922267072,0.803744585193873,-3.12091528312215));
#69613=CARTESIAN_POINT('Ctrl Pts',(21.7595929874866,0.803756597111661,-3.12091218960953));
#69614=CARTESIAN_POINT('Ctrl Pts',(21.7595945111751,0.803780654466387,-3.12090599380377));
#69615=CARTESIAN_POINT('Ctrl Pts',(21.7595952740906,0.803792700002387,-3.12090289148471));
#69616=CARTESIAN_POINT('Ctrl Pts',(21.7595968020794,0.803816825039296,-3.12089667795));
#69617=CARTESIAN_POINT('Ctrl Pts',(21.7595975671451,0.803828904417523,-3.12089356676554));
#69618=CARTESIAN_POINT('Ctrl Pts',(21.7595990994428,0.803853097269881,-3.12088733546504));
#69619=CARTESIAN_POINT('Ctrl Pts',(21.7595998666691,0.8038652106532,-3.12088421537198));
#69620=CARTESIAN_POINT('Ctrl Pts',(21.7596014032889,0.803889471526135,-3.12087796625033));
#69621=CARTESIAN_POINT('Ctrl Pts',(21.7596021726829,0.803901619024839,-3.12087483721898));
#69622=CARTESIAN_POINT('Ctrl Pts',(21.7596037136399,0.803925948158126,-3.12086857021187));
#69623=CARTESIAN_POINT('Ctrl Pts',(21.759604485204,0.803938129809925,-3.12086543223125));
#69624=CARTESIAN_POINT('Ctrl Pts',(21.7600495613914,0.810965074730206,-3.11905525477811));
#69625=CARTESIAN_POINT('Ctrl Pts',(21.7604946304961,0.817973679166252,-3.11722458183839));
#69626=CARTESIAN_POINT('Ctrl Pts',(21.7615091164916,0.833907191489558,-3.11300525505727));
#69627=CARTESIAN_POINT('Ctrl Pts',(21.7620790104874,0.84282808917369,-3.11060182782758));
#69628=CARTESIAN_POINT('Ctrl Pts',(21.7638541248432,0.870521361009193,-3.10301295728822));
#69629=CARTESIAN_POINT('Ctrl Pts',(21.7650636241495,0.889256882552385,-3.0976957602508));
#69630=CARTESIAN_POINT('Ctrl Pts',(21.781616872936,1.14382190177504,-3.02294969780754));
#69631=CARTESIAN_POINT('Ctrl Pts',(21.7978824599157,1.37095191580751,-2.92694324401145));
#69632=CARTESIAN_POINT('Ctrl Pts',(21.8249089152736,1.71920285461805,-2.730245959176));
#69633=CARTESIAN_POINT('Ctrl Pts',(21.8354053101026,1.84787082567989,-2.64485876462202));
#69634=CARTESIAN_POINT('Ctrl Pts',(21.8494525463479,2.01581805469811,-2.51514541576639));
#69635=CARTESIAN_POINT('Ctrl Pts',(21.8532459968199,2.06074113995951,-2.47847245072498));
#69636=CARTESIAN_POINT('Ctrl Pts',(21.8589905919686,2.12845425816945,-2.42008012596923));
#69637=CARTESIAN_POINT('Ctrl Pts',(21.860989509979,2.15195517820215,-2.39920704279093));
#69638=CARTESIAN_POINT('Ctrl Pts',(21.8634549156649,2.18091241672148,-2.37271987872689));
#69639=CARTESIAN_POINT('Ctrl Pts',(21.8639441862554,2.18665770758032,-2.36742616890325));
#69640=CARTESIAN_POINT('Ctrl Pts',(21.8647167439107,2.19572825647193,-2.35900737764558));
#69641=CARTESIAN_POINT('Ctrl Pts',(21.8650010648622,2.19906617839444,-2.35589607744367));
#69642=CARTESIAN_POINT('Ctrl Pts',(21.8655356609689,2.20534204267046,-2.35002134139359));
#69643=CARTESIAN_POINT('Ctrl Pts',(21.8657860489154,2.20828137099089,-2.34725951204898));
#69644=CARTESIAN_POINT('Ctrl Pts',(21.8663583636742,2.21499948234717,-2.34092330295013));
#69645=CARTESIAN_POINT('Ctrl Pts',(21.8666800053496,2.21877479469742,-2.33734529507545));
#69646=CARTESIAN_POINT('Ctrl Pts',(21.8676702360857,2.2303961751003,-2.32627773867471));
#69647=CARTESIAN_POINT('Ctrl Pts',(21.8683364979593,2.23821320637653,-2.31875761260266));
#69648=CARTESIAN_POINT('Ctrl Pts',(21.8737626164917,2.30184001445535,-2.2569259064803));
#69649=CARTESIAN_POINT('Ctrl Pts',(21.8783760651636,2.35570753384216,-2.20064223518734));
#69650=CARTESIAN_POINT('Ctrl Pts',(21.8993317313724,2.59564714188433,-1.93102115601129));
#69651=CARTESIAN_POINT('Ctrl Pts',(21.9145711648951,2.75514411314558,-1.69571050814438));
#69652=CARTESIAN_POINT('Ctrl Pts',(21.9356417208119,2.91969047795385,-1.36699253364841));
#69653=CARTESIAN_POINT('Ctrl Pts',(21.9405558977839,2.95453285515125,-1.28995932363136));
#69654=CARTESIAN_POINT('Ctrl Pts',(21.9484970984594,3.00486538604206,-1.16590671629488));
#69655=CARTESIAN_POINT('Ctrl Pts',(21.9514576696479,3.02237072212546,-1.11974518355661));
#69656=CARTESIAN_POINT('Ctrl Pts',(21.9552651919248,3.04325929456467,-1.06059845378057));
#69657=CARTESIAN_POINT('Ctrl Pts',(21.9560790753018,3.04763179827958,-1.04796785629027));
#69658=CARTESIAN_POINT('Ctrl Pts',(21.9573873356767,3.05451168473078,-1.02768708078981));
#69659=CARTESIAN_POINT('Ctrl Pts',(21.9578800475144,3.05706922374543,-1.02005398266347));
#69660=CARTESIAN_POINT('Ctrl Pts',(21.9588160685933,3.06186422872117,-1.00556304778099));
#69661=CARTESIAN_POINT('Ctrl Pts',(21.9592591884258,3.06410732447876,-0.998707114680354));
#69662=CARTESIAN_POINT('Ctrl Pts',(21.9602660262477,3.06914295118856,-0.98313925939995));
#69663=CARTESIAN_POINT('Ctrl Pts',(21.9608302034348,3.07192143254615,-0.974422889562584));
#69664=CARTESIAN_POINT('Ctrl Pts',(21.9622872624879,3.07898582751733,-0.95193065886192));
#69665=CARTESIAN_POINT('Ctrl Pts',(21.9631819543838,3.08321638208288,-0.938137748782555));
#69666=CARTESIAN_POINT('Ctrl Pts',(21.9686358045789,3.10835342098128,-0.854176364949277));
#69667=CARTESIAN_POINT('Ctrl Pts',(21.973269656034,3.12695485529495,-0.783345501650713));
#69668=CARTESIAN_POINT('Ctrl Pts',(21.9788107898022,3.14598981514643,-0.699309339643838));
#69669=CARTESIAN_POINT('Ctrl Pts',(21.9796463348711,3.14877610309654,-0.686654581773746));
#69670=CARTESIAN_POINT('Ctrl Pts',(21.9844468825204,3.1643046451757,-0.614044521965889));
#69671=CARTESIAN_POINT('Ctrl Pts',(21.9884581171415,3.17541007152699,-0.553755111952784));
#69672=CARTESIAN_POINT('Ctrl Pts',(22.008738159895,3.22235970054904,-0.250575547040934));
#69673=CARTESIAN_POINT('Ctrl Pts',(22.0256265048186,3.23208200282656,-0.00449090003082506));
#69674=CARTESIAN_POINT('Ctrl Pts',(22.0463974915761,3.2087950850084,0.306951396204653));
#69675=CARTESIAN_POINT('Ctrl Pts',(22.0507906125347,3.20173862004059,0.373438183203714));
#69676=CARTESIAN_POINT('Ctrl Pts',(22.0573305152761,3.18788454131705,0.47404009468864));
#69677=CARTESIAN_POINT('Ctrl Pts',(22.0595411937401,3.18259499070741,0.508341639117178));
#69678=CARTESIAN_POINT('Ctrl Pts',(22.0622294761317,3.17539364867108,0.550506906079189));
#69679=CARTESIAN_POINT('Ctrl Pts',(22.0627349988943,3.17400527168273,0.558456100608419));
#69680=CARTESIAN_POINT('Ctrl Pts',(22.0635273194852,3.171775043753,0.570948316359138));
#69681=CARTESIAN_POINT('Ctrl Pts',(22.063815241486,3.17095326719509,0.575494818423807));
#69682=CARTESIAN_POINT('Ctrl Pts',(22.0643528966968,3.16939740910222,0.583998133990971));
#69683=CARTESIAN_POINT('Ctrl Pts',(22.0646027585577,3.16866570133185,0.587955296572799));
#69684=CARTESIAN_POINT('Ctrl Pts',(22.0651690466496,3.16698768651334,0.596936083230726));
#69685=CARTESIAN_POINT('Ctrl Pts',(22.0654852099674,3.16603684026713,0.601958819952992));
#69686=CARTESIAN_POINT('Ctrl Pts',(22.0664422487253,3.16311621407032,0.61718833097298));
#69687=CARTESIAN_POINT('Ctrl Pts',(22.0670810173864,3.16110897478543,0.627387978888903));
#69688=CARTESIAN_POINT('Ctrl Pts',(22.0717577584071,3.1459892466723,0.702302766983671));
#69689=CARTESIAN_POINT('Ctrl Pts',(22.0756908313268,3.13093891541834,0.766616229065749));
#69690=CARTESIAN_POINT('Ctrl Pts',(22.0976418193456,3.0341928164051,1.12939327786391));
#69691=CARTESIAN_POINT('Ctrl Pts',(22.1141818005735,2.91182246501187,1.41533914346475));
#69692=CARTESIAN_POINT('Ctrl Pts',(22.1363540959125,2.71122023519462,1.74387391908023));
#69693=CARTESIAN_POINT('Ctrl Pts',(22.140759990471,2.66964965918646,1.80687047149689));
#69694=CARTESIAN_POINT('Ctrl Pts',(22.1479465902253,2.5995608288089,1.90537833147084));
#69695=CARTESIAN_POINT('Ctrl Pts',(22.1506758694124,2.57243360125697,1.94184658013414));
#69696=CARTESIAN_POINT('Ctrl Pts',(22.1542238445099,2.5365761289891,1.98798081951564));
#69697=CARTESIAN_POINT('Ctrl Pts',(22.1550147885536,2.52854515486869,1.99818557421186));
#69698=CARTESIAN_POINT('Ctrl Pts',(22.1562948713178,2.51548891864918,2.01457104900422));
#69699=CARTESIAN_POINT('Ctrl Pts',(22.1567824712413,2.51050197842521,2.02078223118013));
#69700=CARTESIAN_POINT('Ctrl Pts',(22.1577145318688,2.5009436389748,2.03259705184457));
#69701=CARTESIAN_POINT('Ctrl Pts',(22.1581588268218,2.49637629883038,2.03820392350124));
#69702=CARTESIAN_POINT('Ctrl Pts',(22.159176382698,2.4858908683867,2.05098773402139));
#69703=CARTESIAN_POINT('Ctrl Pts',(22.1597501403624,2.479960519063,2.05815449265041));
#69704=CARTESIAN_POINT('Ctrl Pts',(22.1615174043752,2.46163949274802,2.08010108946757));
#69705=CARTESIAN_POINT('Ctrl Pts',(22.1627150658736,2.44914727622373,2.09479524726676));
#69706=CARTESIAN_POINT('Ctrl Pts',(22.173047063414,2.340743409629,2.22001171879596));
#69707=CARTESIAN_POINT('Ctrl Pts',(22.1824897570267,2.23755261410307,2.32397919259026));
#69708=CARTESIAN_POINT('Ctrl Pts',(22.2015996342679,2.02069801692025,2.5145936183195));
#69709=CARTESIAN_POINT('Ctrl Pts',(22.2112252674824,1.90769779717072,2.60135086481549));
#69710=CARTESIAN_POINT('Ctrl Pts',(22.2208495079139,1.78943601979592,2.68030526126353));
#69711=CARTESIAN_POINT('Origin',(-1.72497344927317,0.,0.));
#69712=CARTESIAN_POINT('',(23.7170278226866,1.78943621037803,2.68030513402633));
#69713=CARTESIAN_POINT('',(23.4730037159736,1.78943621026388,2.68030513410254));
#69714=CARTESIAN_POINT('',(-1.72497344927317,1.78943621037804,2.68030513402633));
#69715=CARTESIAN_POINT('',(22.8965734492155,-3.22274864819489,0.00295178895409686));
#69716=CARTESIAN_POINT('Ctrl Pts',(22.8965734492731,-3.22274864819574,0.00295178801954905));
#69717=CARTESIAN_POINT('Ctrl Pts',(22.902681519152,-3.22283934391745,-0.0960693857917812));
#69718=CARTESIAN_POINT('Ctrl Pts',(22.9087895890309,-3.21836201049138,-0.195199612804562));
#69719=CARTESIAN_POINT('Ctrl Pts',(22.9148976589098,-3.20931356634111,-0.293979583302786));
#69720=CARTESIAN_POINT('Ctrl Pts',(22.9209858737207,-3.20029453532421,-0.392438456781707));
#69721=CARTESIAN_POINT('Ctrl Pts',(22.9270740885317,-3.18673409406454,-0.490548902010164));
#69722=CARTESIAN_POINT('Ctrl Pts',(22.9331623033426,-3.16868130723445,-0.58785741101304));
#69723=CARTESIAN_POINT('Ctrl Pts',(22.9392490004555,-3.15063302068541,-0.685141662506981));
#69724=CARTESIAN_POINT('Ctrl Pts',(22.9453356975685,-3.12809469411758,-0.781623938282448));
#69725=CARTESIAN_POINT('Ctrl Pts',(22.9514223946814,-3.10116684275637,-0.876859039919459));
#69726=CARTESIAN_POINT('Ctrl Pts',(22.9575092842943,-3.07423813976596,-0.972097153493533));
#69727=CARTESIAN_POINT('Ctrl Pts',(22.9635961739071,-3.04291975822478,-1.06608758733206));
#69728=CARTESIAN_POINT('Ctrl Pts',(22.96968306352,-3.00736229680926,-1.15839957623875));
#69729=CARTESIAN_POINT('Ctrl Pts',(22.9758067354239,-2.9715899662277,-1.25126939462153));
#69730=CARTESIAN_POINT('Ctrl Pts',(22.9819304073279,-2.93152730548399,-1.34243998677787));
#69731=CARTESIAN_POINT('Ctrl Pts',(22.9880540792318,-2.88737644976506,-1.43149390492664));
#69732=CARTESIAN_POINT('Ctrl Pts',(22.994149852758,-2.84342673761914,-1.52014210900724));
#69733=CARTESIAN_POINT('Ctrl Pts',(23.0002456262843,-2.79542626918373,-1.60669252181169));
#69734=CARTESIAN_POINT('Ctrl Pts',(23.0063413998106,-2.74361941971756,-1.69076019655321));
#69735=CARTESIAN_POINT('Ctrl Pts',(23.0124790209033,-2.69145691553949,-1.77540499700204));
#69736=CARTESIAN_POINT('Ctrl Pts',(23.0186166419961,-2.63543583487292,-1.85753246908233));
#69737=CARTESIAN_POINT('Ctrl Pts',(23.0247542630888,-2.57584755305794,-1.93678262742762));
#69738=CARTESIAN_POINT('Ctrl Pts',(23.0308918841816,-2.51625927124294,-2.01603278577293));
#69739=CARTESIAN_POINT('Ctrl Pts',(23.0370295052743,-2.45310412858725,-2.09240532528391));
#69740=CARTESIAN_POINT('Ctrl Pts',(23.0431671263671,-2.38671080430784,-2.16557823666111));
#69741=CARTESIAN_POINT('Ctrl Pts',(23.0493393744598,-2.31994290466667,-2.23916397221976));
#69742=CARTESIAN_POINT('Ctrl Pts',(23.0555116225526,-2.24965116623211,-2.3097885076005));
#69743=CARTESIAN_POINT('Ctrl Pts',(23.0616838706454,-2.17612863586824,-2.3770952279314));
#69744=CARTESIAN_POINT('Ctrl Pts',(23.067847759298,-2.10270568140966,-2.44431079079567));
#69745=CARTESIAN_POINT('Ctrl Pts',(23.0740116479506,-2.02606094968589,-2.50821717923666));
#69746=CARTESIAN_POINT('Ctrl Pts',(23.0801755366033,-1.94652641395983,-2.56849225855494));
#69747=CARTESIAN_POINT('Ctrl Pts',(23.0863328982618,-1.86707609802975,-2.62870351207937));
#69748=CARTESIAN_POINT('Ctrl Pts',(23.0924902599203,-1.78474240602476,-2.6852908402357));
#69749=CARTESIAN_POINT('Ctrl Pts',(23.0986476215789,-1.69989196613215,-2.73797093957905));
#69750=CARTESIAN_POINT('Ctrl Pts',(23.1048004857252,-1.61510350341615,-2.79061255987827));
#69751=CARTESIAN_POINT('Ctrl Pts',(23.1109533498715,-1.52780231559818,-2.83935239707996));
#69752=CARTESIAN_POINT('Ctrl Pts',(23.1171062140178,-1.43838496538052,-2.88394976618305));
#69753=CARTESIAN_POINT('Ctrl Pts',(23.1232567471543,-1.34900149088508,-2.92853023959327));
#69754=CARTESIAN_POINT('Ctrl Pts',(23.1294072802909,-1.25750383525661,-2.96897116958274));
#69755=CARTESIAN_POINT('Ctrl Pts',(23.1355578134274,-1.16431339250936,-3.00507768394152));
#69756=CARTESIAN_POINT('Ctrl Pts',(23.1417076616426,-1.07113332741884,-3.04118017749087));
#69757=CARTESIAN_POINT('Ctrl Pts',(23.1478575098579,-0.976261255028329,
-3.07294905811508));
#69758=CARTESIAN_POINT('Ctrl Pts',(23.1540073580731,-0.880137848004802,
-3.10023788297116));
#69759=CARTESIAN_POINT('Ctrl Pts',(23.1601581664522,-0.783999433419462,
-3.12753096837873));
#69760=CARTESIAN_POINT('Ctrl Pts',(23.1663089748313,-0.686609714050804,
-3.15034249006538));
#69761=CARTESIAN_POINT('Ctrl Pts',(23.1724597832105,-0.588422812743392,
-3.16857636107182));
#69762=CARTESIAN_POINT('Ctrl Pts',(23.1786171695767,-0.490130905374042,
-3.18682973230654));
#69763=CARTESIAN_POINT('Ctrl Pts',(23.1847745559429,-0.391040541524046,
-3.20049559744429));
#69764=CARTESIAN_POINT('Ctrl Pts',(23.190931942309,-0.29161417207902,-3.20952936380752));
#69765=CARTESIAN_POINT('Ctrl Pts',(23.197092765046,-0.192132313851934,-3.21856817181809));
#69766=CARTESIAN_POINT('Ctrl Pts',(23.203253587783,-0.0923145105519143,
-3.22296971367894));
#69767=CARTESIAN_POINT('Ctrl Pts',(23.2094144105199,0.00737565744893537,
-3.22274155994197));
#69768=CARTESIAN_POINT('Ctrl Pts',(23.2155855334366,0.10723249582668,-3.22251302475846));
#69769=CARTESIAN_POINT('Ctrl Pts',(23.2217566563533,0.206960838603117,-3.2176393541527));
#69770=CARTESIAN_POINT('Ctrl Pts',(23.22792777927,0.306100955347835,-3.20818013328977));
#69771=CARTESIAN_POINT('Ctrl Pts',(23.2326233012156,0.381535296900412,-3.2009827431633));
#69772=CARTESIAN_POINT('Ctrl Pts',(23.2373188231611,0.456629167056301,-3.19113163707705));
#69773=CARTESIAN_POINT('Ctrl Pts',(23.2420143451067,0.531184747029499,-3.17867273040545));
#69774=CARTESIAN_POINT('Ctrl Pts',(23.2481865931995,0.629187810720701,-3.1622955387251));
#69775=CARTESIAN_POINT('Ctrl Pts',(23.2543588412922,0.726605262142597,-3.14135291118325));
#69776=CARTESIAN_POINT('Ctrl Pts',(23.260531089385,0.82297866024604,-3.11589853610153));
#69777=CARTESIAN_POINT('Ctrl Pts',(23.2666949780376,0.919221534164408,-3.09047863538336));
#69778=CARTESIAN_POINT('Ctrl Pts',(23.2728588666903,1.01442274901521,-3.06055924241639));
#69779=CARTESIAN_POINT('Ctrl Pts',(23.2790227553429,1.10813182087535,-3.02624543453823));
#69780=CARTESIAN_POINT('Ctrl Pts',(23.2851801170014,1.20174166340283,-2.99196796184287));
#69781=CARTESIAN_POINT('Ctrl Pts',(23.29133747866,1.29386209857369,-2.95330547393786));
#69782=CARTESIAN_POINT('Ctrl Pts',(23.2974948403185,1.38405656938981,-2.91041319664904));
#69783=CARTESIAN_POINT('Ctrl Pts',(23.3036477044648,1.4741851595969,-2.86755224910057));
#69784=CARTESIAN_POINT('Ctrl Pts',(23.3098005686111,1.56239019127225,-2.82046784072556));
#69785=CARTESIAN_POINT('Ctrl Pts',(23.3159534327574,1.64825477253389,-2.76936342275969));
#69786=CARTESIAN_POINT('Ctrl Pts',(23.322103965894,1.73408682403813,-2.71827836567922));
#69787=CARTESIAN_POINT('Ctrl Pts',(23.3282544990305,1.81757981410254,-2.66317654707034));
#69788=CARTESIAN_POINT('Ctrl Pts',(23.3344050321671,1.89834196242879,-2.60430707793494));
#69789=CARTESIAN_POINT('Ctrl Pts',(23.3405548803823,1.97909511710892,-2.54544416448414));
#69790=CARTESIAN_POINT('Ctrl Pts',(23.3467047285975,2.05711768363793,-2.48281469052846));
#69791=CARTESIAN_POINT('Ctrl Pts',(23.3528545768127,2.13204819676772,-2.4167101706989));
#69792=CARTESIAN_POINT('Ctrl Pts',(23.3590053851918,2.20699040865387,-2.35059533009829));
#69793=CARTESIAN_POINT('Ctrl Pts',(23.3651561935709,2.27883928249741,-2.2810046533681));
#69794=CARTESIAN_POINT('Ctrl Pts',(23.3713070019501,2.34726844021977,-2.20826819749057));
#69795=CARTESIAN_POINT('Ctrl Pts',(23.3774643883162,2.41577077956085,-2.13545395355079));
#69796=CARTESIAN_POINT('Ctrl Pts',(23.3836217746824,2.48084580147416,-2.05948752938292));
#69797=CARTESIAN_POINT('Ctrl Pts',(23.3897791610486,2.54220594227285,-1.98073383107691));
#69798=CARTESIAN_POINT('Ctrl Pts',(23.3959399837856,2.60360032750285,-1.90193618118317));
#69799=CARTESIAN_POINT('Ctrl Pts',(23.4021008065225,2.66127545205123,-1.82034851401034));
#69800=CARTESIAN_POINT('Ctrl Pts',(23.4082616292595,2.71498702167986,-1.73636489097481));
#69801=CARTESIAN_POINT('Ctrl Pts',(23.4144327521762,2.7687883908116,-1.65224085708047));
#69802=CARTESIAN_POINT('Ctrl Pts',(23.4206038750928,2.81861275173148,-1.56571324254608));
#69803=CARTESIAN_POINT('Ctrl Pts',(23.4267749980095,2.8642616470605,-1.47720099501668));
#69804=CARTESIAN_POINT('Ctrl Pts',(23.4314705199551,2.89899525919308,-1.40985325193308));
#69805=CARTESIAN_POINT('Ctrl Pts',(23.4361660419008,2.93131244543431,-1.34135702503197));
#69806=CARTESIAN_POINT('Ctrl Pts',(23.4408615638464,2.96114486756336,-1.27190354815261));
#69807=CARTESIAN_POINT('Ctrl Pts',(23.4470338119391,3.00035948794444,-1.18060718213213));
#69808=CARTESIAN_POINT('Ctrl Pts',(23.4532060600319,3.0354169764317,-1.08733486045608));
#69809=CARTESIAN_POINT('Ctrl Pts',(23.4593783081247,3.06611461235053,-0.99250125764683));
#69810=CARTESIAN_POINT('Ctrl Pts',(23.4655421967773,3.0967706726479,-0.897796093587165));
#69811=CARTESIAN_POINT('Ctrl Pts',(23.4717060854299,3.12307848423293,-0.801534260890484));
#69812=CARTESIAN_POINT('Ctrl Pts',(23.4778699740825,3.14488285782888,-0.704151527040935));
#69813=CARTESIAN_POINT('Ctrl Pts',(23.484027335741,3.16666414258838,-0.606871912595596));
#69814=CARTESIAN_POINT('Ctrl Pts',(23.4901846973996,3.18395137565682,-0.508474178272502));
#69815=CARTESIAN_POINT('Ctrl Pts',(23.4963420590581,3.19663908354375,-0.409409491903414));
#69816=CARTESIAN_POINT('Ctrl Pts',(23.5024949232044,3.20931752396765,-0.31041716520136));
#69817=CARTESIAN_POINT('Ctrl Pts',(23.5086477873508,3.21740306370195,-0.210759284569266));
#69818=CARTESIAN_POINT('Ctrl Pts',(23.5148006514971,3.22084143003047,-0.110896551340821));
#69819=CARTESIAN_POINT('Ctrl Pts',(23.5209511846336,3.22427849373547,-0.0110716510632181));
#69820=CARTESIAN_POINT('Ctrl Pts',(23.5271017177701,3.22307186736618,0.0889575139673457));
#69821=CARTESIAN_POINT('Ctrl Pts',(23.5332522509067,3.21721926569915,0.188726677802104));
#69822=CARTESIAN_POINT('Ctrl Pts',(23.5394020991219,3.21136731577591,0.288484731375786));
#69823=CARTESIAN_POINT('Ctrl Pts',(23.5455519473371,3.20087044460797,0.387982407687484));
#69824=CARTESIAN_POINT('Ctrl Pts',(23.5517017955523,3.18577842894078,0.486758014002484));
#69825=CARTESIAN_POINT('Ctrl Pts',(23.5578526039314,3.1706840569863,0.58554904196229));
#69826=CARTESIAN_POINT('Ctrl Pts',(23.5640034123106,3.15099318114259,0.68361734657127));
#69827=CARTESIAN_POINT('Ctrl Pts',(23.5701542206897,3.12680697231633,0.780509910490545));
#69828=CARTESIAN_POINT('Ctrl Pts',(23.5763116070559,3.1025948975293,0.877506096241446));
#69829=CARTESIAN_POINT('Ctrl Pts',(23.5824689934221,3.07387799500923,0.973323608145693));
#69830=CARTESIAN_POINT('Ctrl Pts',(23.5886263797883,3.04080773838193,1.06752323660731));
#69831=CARTESIAN_POINT('Ctrl Pts',(23.5947872025252,3.00771902560189,1.16177543686332));
#69832=CARTESIAN_POINT('Ctrl Pts',(23.6009480252622,2.97027228308328,1.25440755279031));
#69833=CARTESIAN_POINT('Ctrl Pts',(23.6071088479991,2.92866690640633,1.34500100885479));
#69834=CARTESIAN_POINT('Ctrl Pts',(23.6132799709158,2.88699197037412,1.43574592665084));
#69835=CARTESIAN_POINT('Ctrl Pts',(23.6194510938325,2.8411447118201,1.5244449903503));
#69836=CARTESIAN_POINT('Ctrl Pts',(23.6256222167492,2.79137024530098,1.61070472655554));
#69837=CARTESIAN_POINT('Ctrl Pts',(23.6303177386948,2.75349754319713,1.67633856497353));
#69838=CARTESIAN_POINT('Ctrl Pts',(23.6350132606403,2.71335214004656,1.74056068135109));
#69839=CARTESIAN_POINT('Ctrl Pts',(23.6397087825859,2.6710579522838,1.8032101868727));
#69840=CARTESIAN_POINT('Ctrl Pts',(23.6461520359276,2.61302134425669,1.88917861391627));
#69841=CARTESIAN_POINT('Ctrl Pts',(23.6525952892694,2.55072347699362,1.97250029428709));
#69842=CARTESIAN_POINT('Ctrl Pts',(23.6590385426111,2.4844376228156,2.05272678670065));
#69843=CARTESIAN_POINT('Ctrl Pts',(23.6652014287937,2.42103608431474,2.12946236038559));
#69844=CARTESIAN_POINT('Ctrl Pts',(23.6713643149763,2.35398663560209,2.20336605360624));
#69845=CARTESIAN_POINT('Ctrl Pts',(23.6775272011589,2.28357367016464,2.27407318603223));
#69846=CARTESIAN_POINT('Ctrl Pts',(23.6836843482758,2.21322627540712,2.34471447384112));
#69847=CARTESIAN_POINT('Ctrl Pts',(23.6898414953927,2.1395218913356,2.41216480861059));
#69848=CARTESIAN_POINT('Ctrl Pts',(23.6959986425095,2.0627846731223,2.47609308282862));
#69849=CARTESIAN_POINT('Ctrl Pts',(23.7021510548996,1.98610646434281,2.53997219744256));
#69850=CARTESIAN_POINT('Ctrl Pts',(23.7083034672896,1.90640039290316,2.60033436134496));
#69851=CARTESIAN_POINT('Ctrl Pts',(23.7144558796797,1.82402606814533,2.65688661128515));
#69852=CARTESIAN_POINT('Ctrl Pts',(23.7153131940153,1.81254753175562,2.66476694366744));
#69853=CARTESIAN_POINT('Ctrl Pts',(23.716170508351,1.80101723805182,2.67257336124801));
#69854=CARTESIAN_POINT('Ctrl Pts',(23.7170278226866,1.78943621037803,2.68030513402633));
#69855=CARTESIAN_POINT('Ctrl Pts',(22.4670531482195,1.78943621037803,2.68030513402633));
#69856=CARTESIAN_POINT('Ctrl Pts',(22.4732162780277,1.70663396539659,2.73558590545395));
#69857=CARTESIAN_POINT('Ctrl Pts',(22.479379407836,1.62115245987748,2.7871029884318));
#69858=CARTESIAN_POINT('Ctrl Pts',(22.4855425376442,1.53336940281544,2.83458918311092));
#69859=CARTESIAN_POINT('Ctrl Pts',(22.4916993292816,1.44567662196684,2.88202654292384));
#69860=CARTESIAN_POINT('Ctrl Pts',(22.4978561209189,1.35568737542522,2.92544105046133));
#69861=CARTESIAN_POINT('Ctrl Pts',(22.5040129125562,1.26380761221948,2.96460922918959));
#69862=CARTESIAN_POINT('Ctrl Pts',(22.5101654596615,1.17199119151748,3.00375040512179));
#69863=CARTESIAN_POINT('Ctrl Pts',(22.5163180067668,1.07828724369721,3.03865090225139));
#69864=CARTESIAN_POINT('Ctrl Pts',(22.5224705538721,0.98312472179743,3.06913397294591));
#69865=CARTESIAN_POINT('Ctrl Pts',(22.5286209400674,0.887995623069388,3.09960633731522));
#69866=CARTESIAN_POINT('Ctrl Pts',(22.5347713262628,0.791409381473145,3.12566422577062));
#69867=CARTESIAN_POINT('Ctrl Pts',(22.5409217124581,0.69381240116912,3.14717999397619));
#69868=CARTESIAN_POINT('Ctrl Pts',(22.5470715836672,0.59622359288879,3.1686939606161));
#69869=CARTESIAN_POINT('Ctrl Pts',(22.5532214548764,0.497624638411956,3.18566646979002));
#69870=CARTESIAN_POINT('Ctrl Pts',(22.5593713260855,0.398473501923653,3.19802070518074));
#69871=CARTESIAN_POINT('Ctrl Pts',(22.5655223273652,0.299304145901022,3.21037721072613));
#69872=CARTESIAN_POINT('Ctrl Pts',(22.571673328645,0.199582837374169,3.21811370303971));
#69873=CARTESIAN_POINT('Ctrl Pts',(22.5778243299248,0.0997730440188858,
3.22120519405194));
#69874=CARTESIAN_POINT('Ctrl Pts',(22.5839820025074,-0.000145001850732199,
3.22430003805854));
#69875=CARTESIAN_POINT('Ctrl Pts',(22.5901396750899,-0.100151289225844,
3.22273980851612));
#69876=CARTESIAN_POINT('Ctrl Pts',(22.5962973476725,-0.199782100852666,
3.21655167449225));
#69877=CARTESIAN_POINT('Ctrl Pts',(22.6024586093376,-0.299470983641893,
3.210359933631));
#69878=CARTESIAN_POINT('Ctrl Pts',(22.6086198710027,-0.398783523223655,
3.19953496402935));
#69879=CARTESIAN_POINT('Ctrl Pts',(22.6147811326678,-0.497262953691921,
3.18415563648914));
#69880=CARTESIAN_POINT('Ctrl Pts',(22.6209525032228,-0.59590396108603,3.16875107581697));
#69881=CARTESIAN_POINT('Ctrl Pts',(22.6271238737778,-0.69370870411311,3.14877732116875));
#69882=CARTESIAN_POINT('Ctrl Pts',(22.6332952443328,-0.790232337502041,
3.12436400172356));
#69883=CARTESIAN_POINT('Ctrl Pts',(22.6373543925178,-0.853719650050794,
3.10830642092649));
#69884=CARTESIAN_POINT('Ctrl Pts',(22.6414135407027,-0.91665303363912,3.09032922842104));
#69885=CARTESIAN_POINT('Ctrl Pts',(22.6454726888877,-0.978910542606468,
3.07048069723194));
#69886=CARTESIAN_POINT('Ctrl Pts',(22.6516449369805,-1.07357788990984,3.04029947368625));
#69887=CARTESIAN_POINT('Ctrl Pts',(22.6578171850732,-1.16701475826756,3.00568292964486));
#69888=CARTESIAN_POINT('Ctrl Pts',(22.663989433166,-1.2587750428666,2.9667495603701));
#69889=CARTESIAN_POINT('Ctrl Pts',(22.6701533218186,-1.35041105109282,2.92786892085677));
#69890=CARTESIAN_POINT('Ctrl Pts',(22.6763172104713,-1.44037459246968,2.88468324490364));
#69891=CARTESIAN_POINT('Ctrl Pts',(22.6824810991239,-1.52823476404977,2.83736075754384));
#69892=CARTESIAN_POINT('Ctrl Pts',(22.6886384607824,-1.61600189974735,2.79008838036815));
#69893=CARTESIAN_POINT('Ctrl Pts',(22.694795822441,-1.70166971336131,2.73868810548877));
#69894=CARTESIAN_POINT('Ctrl Pts',(22.7009531840995,-1.78482823578486,2.68337580879852));
#69895=CARTESIAN_POINT('Ctrl Pts',(22.7071060482458,-1.86792601685632,2.62810391378437));
#69896=CARTESIAN_POINT('Ctrl Pts',(22.7132589123921,-1.94851779018614,2.56892591790401));
#69897=CARTESIAN_POINT('Ctrl Pts',(22.7194117765384,-2.02621992593659,2.50610262643762));
#69898=CARTESIAN_POINT('Ctrl Pts',(22.725562309675,-2.10389262426838,2.44330313554652));
#69899=CARTESIAN_POINT('Ctrl Pts',(22.7317128428115,-2.17867752285137,2.37686136594475));
#69900=CARTESIAN_POINT('Ctrl Pts',(22.737863375948,-2.25022235619732,2.3070797364135));
#69901=CARTESIAN_POINT('Ctrl Pts',(22.7440132241632,-2.32175922233442,2.23730587774131));
#69902=CARTESIAN_POINT('Ctrl Pts',(22.7501630723785,-2.39005642962478,2.16419320187664));
#69903=CARTESIAN_POINT('Ctrl Pts',(22.7563129205937,-2.4547977630544,2.0880817764166));
#69904=CARTESIAN_POINT('Ctrl Pts',(22.7624637289728,-2.5195492044234,2.01195846782667));
#69905=CARTESIAN_POINT('Ctrl Pts',(22.7686145373519,-2.58074338775064,1.93283581059582));
#69906=CARTESIAN_POINT('Ctrl Pts',(22.7747653457311,-2.63810432141074,1.85108701898478));
#69907=CARTESIAN_POINT('Ctrl Pts',(22.7809227320972,-2.69552659976824,1.76925080106174));
#69908=CARTESIAN_POINT('Ctrl Pts',(22.7870801184634,-2.74910719225307,1.68478319669865));
#69909=CARTESIAN_POINT('Ctrl Pts',(22.7932375048296,-2.79861349327314,1.59808637994619));
#69910=CARTESIAN_POINT('Ctrl Pts',(22.7993983275666,-2.84814742322464,1.51134117863749));
#69911=CARTESIAN_POINT('Ctrl Pts',(22.8055591503035,-2.89360233581464,1.42236467416699));
#69912=CARTESIAN_POINT('Ctrl Pts',(22.8117199730405,-2.93479260933334,1.33158172963676));
#69913=CARTESIAN_POINT('Ctrl Pts',(22.8178910959571,-2.97605174820308,1.24064700657218));
#69914=CARTESIAN_POINT('Ctrl Pts',(22.8240622188738,-3.01303184513153,1.14790021444844));
#69915=CARTESIAN_POINT('Ctrl Pts',(22.8302333417905,-3.04559619487645,1.05378431391536));
#69916=CARTESIAN_POINT('Ctrl Pts',(22.8349288637362,-3.07037395751986,0.982172828882028));
#69917=CARTESIAN_POINT('Ctrl Pts',(22.8396243856818,-3.09259624749288,0.909769075839418));
#69918=CARTESIAN_POINT('Ctrl Pts',(22.8443199076274,-3.11222268684338,0.836772077687444));
#69919=CARTESIAN_POINT('Ctrl Pts',(22.852243497083,-3.14534186926603,0.71359125742116));
#69920=CARTESIAN_POINT('Ctrl Pts',(22.8601670865385,-3.17116313898967,0.588370950078732));
#69921=CARTESIAN_POINT('Ctrl Pts',(22.868090675994,-3.18948195103085,0.461868429911007));
#69922=CARTESIAN_POINT('Ctrl Pts',(22.8758590689198,-3.20744195901301,0.337843669633462));
#69923=CARTESIAN_POINT('Ctrl Pts',(22.8836274618455,-3.21819054073371,0.212586230235369));
#69924=CARTESIAN_POINT('Ctrl Pts',(22.8913958547713,-3.22158001987508,0.0868316649713684));
#69925=CARTESIAN_POINT('Ctrl Pts',(22.893121719586,-3.22233304342142,0.058893405210885));
#69926=CARTESIAN_POINT('Ctrl Pts',(22.8948475844007,-3.22272302167004,0.0309307026174956));
#69927=CARTESIAN_POINT('Ctrl Pts',(22.8965734492154,-3.22274864819489,0.00295178895407324));
#69928=CARTESIAN_POINT('Ctrl Pts',(22.2208495079139,1.78943601979592,2.68030526126352));
#69929=CARTESIAN_POINT('Ctrl Pts',(22.2274108732164,1.70881056907048,2.73413274417209));
#69930=CARTESIAN_POINT('Ctrl Pts',(22.2339688700644,1.62573948420363,2.78433370019938));
#69931=CARTESIAN_POINT('Ctrl Pts',(22.2449657526838,1.48059623411035,2.86331938725809));
#69932=CARTESIAN_POINT('Ctrl Pts',(22.2494484428537,1.41970581754167,2.89399374300783));
#69933=CARTESIAN_POINT('Ctrl Pts',(22.2561057682776,1.32598625840515,2.93753555360142));
#69934=CARTESIAN_POINT('Ctrl Pts',(22.2583468774917,1.29384594146965,2.95183292413911));
#69935=CARTESIAN_POINT('Ctrl Pts',(22.2610670099127,1.25401890637395,2.96877412793341));
#69936=CARTESIAN_POINT('Ctrl Pts',(22.261574730624,1.24654933655056,2.97191823493393));
#69937=CARTESIAN_POINT('Ctrl Pts',(22.2623697217724,1.23479578628585,2.9768134549211));
#69938=CARTESIAN_POINT('Ctrl Pts',(22.2626581288331,1.23051982166127,2.97858354732088));
#69939=CARTESIAN_POINT('Ctrl Pts',(22.2631962091176,1.22251937160008,2.98187527158602));
#69940=CARTESIAN_POINT('Ctrl Pts',(22.2634460131047,1.21879588973386,2.98339912325581));
#69941=CARTESIAN_POINT('Ctrl Pts',(22.264011549362,1.21034531152132,2.98683909937323));
#69942=CARTESIAN_POINT('Ctrl Pts',(22.264327021526,1.20561652629364,2.9887509717349));
#69943=CARTESIAN_POINT('Ctrl Pts',(22.2652592571518,1.19159962078208,2.99437939932244));
#69944=CARTESIAN_POINT('Ctrl Pts',(22.2658741157098,1.18229860778889,2.99806398389566));
#69945=CARTESIAN_POINT('Ctrl Pts',(22.2701527655441,1.11719659446997,3.0235039861866));
#69946=CARTESIAN_POINT('Ctrl Pts',(22.2737304177496,1.06081165614945,3.0437451102979));
#69947=CARTESIAN_POINT('Ctrl Pts',(22.2781981997703,0.988474739313168,3.06745798001493));
#69948=CARTESIAN_POINT('Ctrl Pts',(22.2791457517092,0.973020097629172,3.07239526681861));
#69949=CARTESIAN_POINT('Ctrl Pts',(22.281697012377,0.93112817349355,3.08543065947846));
#69950=CARTESIAN_POINT('Ctrl Pts',(22.2832927991265,0.904622526772044,3.09330570471412));
#69951=CARTESIAN_POINT('Ctrl Pts',(22.3008608671207,0.609981108372839,3.17673491617553));
#69952=CARTESIAN_POINT('Ctrl Pts',(22.3159093867766,0.333233662088647,3.21755998755489));
#69953=CARTESIAN_POINT('Ctrl Pts',(22.336105817205,-0.0164871055455884,
3.22349355504828));
#69954=CARTESIAN_POINT('Ctrl Pts',(22.340269838053,-0.0876618243376626,
3.22234338610454));
#69955=CARTESIAN_POINT('Ctrl Pts',(22.3470945958057,-0.20221209011489,3.21669434896977));
#69956=CARTESIAN_POINT('Ctrl Pts',(22.3497103120254,-0.245637828466587,
3.21366987160982));
#69957=CARTESIAN_POINT('Ctrl Pts',(22.3531303322343,-0.301723771070749,
3.20862024191851));
#69958=CARTESIAN_POINT('Ctrl Pts',(22.3539093187466,-0.314452991684446,
3.20739776135162));
#69959=CARTESIAN_POINT('Ctrl Pts',(22.3551747183728,-0.335054887804643,
3.20529538928018));
#69960=CARTESIAN_POINT('Ctrl Pts',(22.3556596569679,-0.342932269942511,
3.20446216498833));
#69961=CARTESIAN_POINT('Ctrl Pts',(22.3565897782726,-0.358006565552584,
3.2028114719568));
#69962=CARTESIAN_POINT('Ctrl Pts',(22.3570348078889,-0.365203960426041,
3.20199876511555));
#69963=CARTESIAN_POINT('Ctrl Pts',(22.358048980791,-0.381571263369378,3.20009471915908));
#69964=CARTESIAN_POINT('Ctrl Pts',(22.3586186001243,-0.3907393124357,3.19898821934262));
#69965=CARTESIAN_POINT('Ctrl Pts',(22.360392016489,-0.419204557065618,3.19542853173744));
#69966=CARTESIAN_POINT('Ctrl Pts',(22.3616000806889,-0.43848410980067,3.1928400556282));
#69967=CARTESIAN_POINT('Ctrl Pts',(22.3782104746239,-0.702017099602754,
3.1550261588626));
#69968=CARTESIAN_POINT('Ctrl Pts',(22.3945423426646,-0.941409416115868,
3.09204112996409));
#69969=CARTESIAN_POINT('Ctrl Pts',(22.421592335161,-1.31431522152625,2.94657150086656));
#69970=CARTESIAN_POINT('Ctrl Pts',(22.4320446759238,-1.45323592316047,2.88059308397445));
#69971=CARTESIAN_POINT('Ctrl Pts',(22.4460360715767,-1.63721877248399,2.77650343362528));
#69972=CARTESIAN_POINT('Ctrl Pts',(22.4498165498814,-1.68674116967793,2.74670014527166));
#69973=CARTESIAN_POINT('Ctrl Pts',(22.4555437547966,-1.76185928233883,2.69869461088187));
#69974=CARTESIAN_POINT('Ctrl Pts',(22.4575379283654,-1.78803373429756,2.68142429975549));
#69975=CARTESIAN_POINT('Ctrl Pts',(22.4599983144102,-1.82040522898272,2.65938024726134));
#69976=CARTESIAN_POINT('Ctrl Pts',(22.4604872004205,-1.82684145539995,2.65496305003844));
#69977=CARTESIAN_POINT('Ctrl Pts',(22.4612592901032,-1.8370133857059,2.64792752779077));
#69978=CARTESIAN_POINT('Ctrl Pts',(22.4615435255639,-1.84075963781473,2.64532461677271));
#69979=CARTESIAN_POINT('Ctrl Pts',(22.4620780512621,-1.84780798030369,2.64040517726422));
#69980=CARTESIAN_POINT('Ctrl Pts',(22.4623284539103,-1.85111120961895,2.63809043097738));
#69981=CARTESIAN_POINT('Ctrl Pts',(22.4629009219724,-1.85866602180998,2.6327752011763));
#69982=CARTESIAN_POINT('Ctrl Pts',(22.4632227016896,-1.86291468098162,2.6297706236185));
#69983=CARTESIAN_POINT('Ctrl Pts',(22.4642137769317,-1.87600632211741,2.62046479554595));
#69984=CARTESIAN_POINT('Ctrl Pts',(22.4648807395162,-1.88482486181785,2.61412905447763));
#69985=CARTESIAN_POINT('Ctrl Pts',(22.4703278594223,-1.95689454147366,2.56179580592459));
#69986=CARTESIAN_POINT('Ctrl Pts',(22.4749603422434,-2.01848999116991,2.5135501610744));
#69987=CARTESIAN_POINT('Ctrl Pts',(22.4801507511789,-2.08682664808002,2.45589033218598));
#69988=CARTESIAN_POINT('Ctrl Pts',(22.4807984276688,-2.09534160600894,2.44862948233087));
#69989=CARTESIAN_POINT('Ctrl Pts',(22.4898374609906,-2.2139684370903,2.34640245183753));
#69990=CARTESIAN_POINT('Ctrl Pts',(22.4979306614987,-2.31757441650669,2.24412890790787));
#69991=CARTESIAN_POINT('Ctrl Pts',(22.5196984593772,-2.57563431365835,1.95238284104554));
#69992=CARTESIAN_POINT('Ctrl Pts',(22.533422902302,-2.71602935675514,1.75181437567194));
#69993=CARTESIAN_POINT('Ctrl Pts',(22.5495167272156,-2.84345895973308,1.5170340727136));
#69994=CARTESIAN_POINT('Ctrl Pts',(22.550916017264,-2.85426004808538,1.49661309916348));
#69995=CARTESIAN_POINT('Ctrl Pts',(22.5529328644647,-2.86942569849575,1.46717890685365));
#69996=CARTESIAN_POINT('Ctrl Pts',(22.5535440946468,-2.87396941525613,1.45825840663377));
#69997=CARTESIAN_POINT('Ctrl Pts',(22.5546060694255,-2.88177275009728,1.44276029460733));
#69998=CARTESIAN_POINT('Ctrl Pts',(22.5550561342987,-2.88505161159111,1.43619241327167));
#69999=CARTESIAN_POINT('Ctrl Pts',(22.5559224657763,-2.89130884895211,1.42355065414316));
#70000=CARTESIAN_POINT('Ctrl Pts',(22.5563386112618,-2.89429059964961,1.41747848259027));
#70001=CARTESIAN_POINT('Ctrl Pts',(22.5573202450676,-2.90126772981024,1.40315613915234));
#70002=CARTESIAN_POINT('Ctrl Pts',(22.5578862897191,-2.90524705564717,1.39489825211291));
#70003=CARTESIAN_POINT('Ctrl Pts',(22.5595635752927,-2.91690841232209,1.37043226479771));
#70004=CARTESIAN_POINT('Ctrl Pts',(22.560678276152,-2.9244903270729,1.35417708744585));
#70005=CARTESIAN_POINT('Ctrl Pts',(22.573782995581,-3.01165556281761,1.16315340203976));
#70006=CARTESIAN_POINT('Ctrl Pts',(22.5863179144167,-3.07558605548693,0.981703622427311));
#70007=CARTESIAN_POINT('Ctrl Pts',(22.617176466581,-3.18928353729458,0.535445553183421));
#70008=CARTESIAN_POINT('Ctrl Pts',(22.6357397919378,-3.22279985224095,0.267953609073662));
#70009=CARTESIAN_POINT('Ctrl Pts',(22.6547672674059,-3.22274470320708,-0.0288013055865189));
#70010=CARTESIAN_POINT('Ctrl Pts',(22.6565588762784,-3.22236926176266,-0.0570035763551874));
#70011=CARTESIAN_POINT('Ctrl Pts',(22.6588257315519,-3.22141542651251,-0.0930711313139109));
#70012=CARTESIAN_POINT('Ctrl Pts',(22.6593190022196,-3.22117836607331,-0.100943165610303));
#70013=CARTESIAN_POINT('Ctrl Pts',(22.6600964265175,-3.22075790366327,-0.113388882755708));
#70014=CARTESIAN_POINT('Ctrl Pts',(22.6603816359655,-3.22059361246074,-0.117963116023465));
#70015=CARTESIAN_POINT('Ctrl Pts',(22.6608918675772,-3.22028166114351,-0.126161570237166));
#70016=CARTESIAN_POINT('Ctrl Pts',(22.6611170897166,-3.22013762918286,-0.129785855167971));
#70017=CARTESIAN_POINT('Ctrl Pts',(22.6616501889978,-3.21978167422509,-0.138377197414176));
#70018=CARTESIAN_POINT('Ctrl Pts',(22.6619577604787,-3.21956437663612,-0.143344005546633));
#70019=CARTESIAN_POINT('Ctrl Pts',(22.6628639424556,-3.21888890482661,-0.158006304684478));
#70020=CARTESIAN_POINT('Ctrl Pts',(22.6634607625235,-3.21839841690283,-0.167700356792422));
#70021=CARTESIAN_POINT('Ctrl Pts',(22.6682125972535,-3.21412793969047,-0.245166086537417));
#70022=CARTESIAN_POINT('Ctrl Pts',(22.6722556617736,-3.20825120077412,-0.312810801882906));
#70023=CARTESIAN_POINT('Ctrl Pts',(22.6826228344595,-3.18732150853722,-0.488969930785459));
#70024=CARTESIAN_POINT('Ctrl Pts',(22.6888199653084,-3.16886602173882,-0.59699366117581));
#70025=CARTESIAN_POINT('Ctrl Pts',(22.7112943666572,-3.08139137487716,-0.987834565998656));
#70026=CARTESIAN_POINT('Ctrl Pts',(22.7272950901874,-2.9796848865569,-1.26184488157661));
#70027=CARTESIAN_POINT('Ctrl Pts',(22.745558489706,-2.83601185343854,-1.53080023909181));
#70028=CARTESIAN_POINT('Ctrl Pts',(22.7463976695727,-2.82935160326635,-1.54307553306671));
#70029=CARTESIAN_POINT('Ctrl Pts',(22.7485538739142,-2.81209144323197,-1.57439972315977));
#70030=CARTESIAN_POINT('Ctrl Pts',(22.7498748308684,-2.80137778860837,-1.59338483201151));
#70031=CARTESIAN_POINT('Ctrl Pts',(22.7517477766602,-2.78599616871477,-1.62000709089727));
#70032=CARTESIAN_POINT('Ctrl Pts',(22.7522940013489,-2.78148757318117,-1.62773600572995));
#70033=CARTESIAN_POINT('Ctrl Pts',(22.7532519218091,-2.77354150839616,-1.64122822746724));
#70034=CARTESIAN_POINT('Ctrl Pts',(22.7536631040142,-2.77011810150769,-1.64699978629364));
#70035=CARTESIAN_POINT('Ctrl Pts',(22.7545283605002,-2.76288792068777,-1.65910291435515));
#70036=CARTESIAN_POINT('Ctrl Pts',(22.7549825718224,-2.75907735528893,-1.66543216276936));
#70037=CARTESIAN_POINT('Ctrl Pts',(22.7560700868546,-2.74991790926392,-1.68052804771357));
#70038=CARTESIAN_POINT('Ctrl Pts',(22.7567041300957,-2.74454884692482,-1.68928228836126));
#70039=CARTESIAN_POINT('Ctrl Pts',(22.7588624679506,-2.72617500100832,-1.71892197376686));
#70040=CARTESIAN_POINT('Ctrl Pts',(22.7603940352187,-2.71297317988454,-1.73968369513315));
#70041=CARTESIAN_POINT('Ctrl Pts',(22.7686662402932,-2.64081009093741,-1.85035103100832));
#70042=CARTESIAN_POINT('Ctrl Pts',(22.7755652197611,-2.5776213611351,-1.93740565283392));
#70043=CARTESIAN_POINT('Ctrl Pts',(22.804303227976,-2.30250009082873,-2.27910078241128));
#70044=CARTESIAN_POINT('Ctrl Pts',(22.8274329197411,-2.05631105555062,-2.50346697543796));
#70045=CARTESIAN_POINT('Ctrl Pts',(22.8515441409584,-1.74579779287944,-2.70924718092675));
#70046=CARTESIAN_POINT('Ctrl Pts',(22.854190239538,-1.71086196003921,-2.73144320188437));
#70047=CARTESIAN_POINT('Ctrl Pts',(22.8573063110413,-1.66856258767506,-2.75718743093195));
#70048=CARTESIAN_POINT('Ctrl Pts',(22.8578162233416,-1.661602775722,-2.7613873066547));
#70049=CARTESIAN_POINT('Ctrl Pts',(22.8586445390974,-1.65023368643544,-2.76818939988169));
#70050=CARTESIAN_POINT('Ctrl Pts',(22.8589639573471,-1.64583401955077,-2.7708074914037));
#70051=CARTESIAN_POINT('Ctrl Pts',(22.8595332643613,-1.63796432200819,-2.7754651218513));
#70052=CARTESIAN_POINT('Ctrl Pts',(22.8597834123217,-1.63449670335813,-2.77750864807322));
#70053=CARTESIAN_POINT('Ctrl Pts',(22.8603194511805,-1.62704495357722,-2.78188130209477));
#70054=CARTESIAN_POINT('Ctrl Pts',(22.8606052067855,-1.62305965982871,-2.7842083616673));
#70055=CARTESIAN_POINT('Ctrl Pts',(22.8613876415603,-1.61211261705881,-2.7905689755301));
#70056=CARTESIAN_POINT('Ctrl Pts',(22.8618831956893,-1.60514068245339,-2.79458506581228));
#70057=CARTESIAN_POINT('Ctrl Pts',(22.8644882217917,-1.5682917462653,-2.81562801170943));
#70058=CARTESIAN_POINT('Ctrl Pts',(22.8665697052954,-1.53815733805271,-2.83220273474807));
#70059=CARTESIAN_POINT('Ctrl Pts',(22.8725717656503,-1.44946438257588,-2.87915291865768));
#70060=CARTESIAN_POINT('Ctrl Pts',(22.8764251648675,-1.39022910708218,-2.90821813289801));
#70061=CARTESIAN_POINT('Ctrl Pts',(22.8946346910125,-1.1020242299297,-3.03881249389938));
#70062=CARTESIAN_POINT('Ctrl Pts',(22.9082294073425,-0.862630799188419,
-3.11524017516068));
#70063=CARTESIAN_POINT('Ctrl Pts',(22.9226971690508,-0.613682589113914,
-3.16378274612327));
#70064=CARTESIAN_POINT('Ctrl Pts',(22.9228778414336,-0.610574408103934,
-3.16438405965394));
#70065=CARTESIAN_POINT('Ctrl Pts',(22.9233720341204,-0.602074554745427,
-3.16601546494393));
#70066=CARTESIAN_POINT('Ctrl Pts',(22.9236857387533,-0.596681139529607,
-3.16703636087621));
#70067=CARTESIAN_POINT('Ctrl Pts',(22.9265559817898,-0.547355710390877,
-3.1762424827151));
#70068=CARTESIAN_POINT('Ctrl Pts',(22.9291310329197,-0.503261764607915,
-3.18352665465697));
#70069=CARTESIAN_POINT('Ctrl Pts',(22.9321315502969,-0.452196011776676,
-3.19087511895151));
#70070=CARTESIAN_POINT('Ctrl Pts',(22.9325337640886,-0.445357133807378,
-3.19183681918605));
#70071=CARTESIAN_POINT('Ctrl Pts',(22.9377450543764,-0.356836538386813,
-3.20399477342219));
#70072=CARTESIAN_POINT('Ctrl Pts',(22.9426345742314,-0.274763415539632,
-3.21207380580703));
#70073=CARTESIAN_POINT('Ctrl Pts',(22.9485317719995,-0.177513123613066,
-3.21789237449484));
#70074=CARTESIAN_POINT('Ctrl Pts',(22.9494422995084,-0.162544675375431,
-3.21868318720646));
#70075=CARTESIAN_POINT('Ctrl Pts',(22.9509242792237,-0.138261361757858,
-3.21979630072893));
#70076=CARTESIAN_POINT('Ctrl Pts',(22.951493718465,-0.128949545598851,-3.22018267092986));
#70077=CARTESIAN_POINT('Ctrl Pts',(22.9525074106491,-0.112407276173173,
-3.22079718347781));
#70078=CARTESIAN_POINT('Ctrl Pts',(22.9529511562706,-0.105177455071535,
-3.2210413835318));
#70079=CARTESIAN_POINT('Ctrl Pts',(22.953884576831,-0.0899942067671539,
-3.22150305127324));
#70080=CARTESIAN_POINT('Ctrl Pts',(22.954374409147,-0.0820406834009596,
-3.22171541124716));
#70081=CARTESIAN_POINT('Ctrl Pts',(22.9556636546671,-0.0611447951435151,
-3.22219590545264));
#70082=CARTESIAN_POINT('Ctrl Pts',(22.9564645855179,-0.0482015576009701,
-3.22241551341154));
#70083=CARTESIAN_POINT('Ctrl Pts',(22.9600636699525,0.00978611332053737,
-3.22304994753245));
#70084=CARTESIAN_POINT('Ctrl Pts',(22.9628888477855,0.0548331444038588,
-3.22259828815631));
#70085=CARTESIAN_POINT('Ctrl Pts',(22.9704676618632,0.174370785408352,-3.21889273780565));
#70086=CARTESIAN_POINT('Ctrl Pts',(22.9752703049022,0.248779607193562,-3.2139979642511));
#70087=CARTESIAN_POINT('Ctrl Pts',(23.000026008594,0.625688575460499,-3.17603736397249));
#70088=CARTESIAN_POINT('Ctrl Pts',(23.0211242650034,0.922530263247596,-3.10283665511042));
#70089=CARTESIAN_POINT('Ctrl Pts',(23.0418864685821,1.21496437798842,-2.98497940361677));
#70090=CARTESIAN_POINT('Ctrl Pts',(23.0426147468595,1.22522613262556,-2.98078201303053));
#70091=CARTESIAN_POINT('Ctrl Pts',(23.0473901272484,1.29255214043378,-2.95283707209882));
#70092=CARTESIAN_POINT('Ctrl Pts',(23.0513774555037,1.34894934549943,-2.92750314784193));
#70093=CARTESIAN_POINT('Ctrl Pts',(23.055909009433,1.41366358303851,-2.896165488535));
#70094=CARTESIAN_POINT('Ctrl Pts',(23.0565421223481,1.42271951352171,-2.89172759007916));
#70095=CARTESIAN_POINT('Ctrl Pts',(23.0574926182821,1.43633968614678,-2.88497349401228));
#70096=CARTESIAN_POINT('Ctrl Pts',(23.0578119238001,1.44091938340558,-2.88268886398526));
#70097=CARTESIAN_POINT('Ctrl Pts',(23.0583811075739,1.44909089090398,-2.87858808295975));
#70098=CARTESIAN_POINT('Ctrl Pts',(23.0586312445717,1.45268474745262,-2.87677610991916));
#70099=CARTESIAN_POINT('Ctrl Pts',(23.0591673460186,1.4603932098794,-2.87287148050487));
#70100=CARTESIAN_POINT('Ctrl Pts',(23.0594531748458,1.4645067019542,-2.87077672268807));
#70101=CARTESIAN_POINT('Ctrl Pts',(23.0602360151932,1.47578234496753,-2.86500416311647));
#70102=CARTESIAN_POINT('Ctrl Pts',(23.0607318997247,1.48293529631653,-2.8613083186882));
#70103=CARTESIAN_POINT('Ctrl Pts',(23.0633416538298,1.52062981892973,-2.84165268967512));
#70104=CARTESIAN_POINT('Ctrl Pts',(23.0654274141257,1.5509291765247,-2.82522989707241));
#70105=CARTESIAN_POINT('Ctrl Pts',(23.0714453937451,1.63861449590422,-2.77586697823814));
#70106=CARTESIAN_POINT('Ctrl Pts',(23.0753100095356,1.69525905951608,-2.74164053634942));
#70107=CARTESIAN_POINT('Ctrl Pts',(23.0934545149861,1.95999245884838,-2.57033548781493));
#70108=CARTESIAN_POINT('Ctrl Pts',(23.1069830968265,2.15277646690291,-2.41117454206961));
#70109=CARTESIAN_POINT('Ctrl Pts',(23.1213476503981,2.32719314316601,-2.22941630567756));
#70110=CARTESIAN_POINT('Ctrl Pts',(23.1215031211226,2.32907758890771,-2.22744754696215));
#70111=CARTESIAN_POINT('Ctrl Pts',(23.1217424098329,2.33197287143755,-2.22441503383245));
#70112=CARTESIAN_POINT('Ctrl Pts',(23.1218261796772,2.33298548459705,-2.223352973442));
#70113=CARTESIAN_POINT('Ctrl Pts',(23.1222126583756,2.33765279818632,-2.2184510495001));
#70114=CARTESIAN_POINT('Ctrl Pts',(23.1225156054466,2.34129873660336,-2.21460287400643));
#70115=CARTESIAN_POINT('Ctrl Pts',(23.1253983026039,2.37587058679394,-2.17793255697847));
#70116=CARTESIAN_POINT('Ctrl Pts',(23.1279969107504,2.40611295690471,-2.14447464019431));
#70117=CARTESIAN_POINT('Ctrl Pts',(23.1309360622594,2.43920321932192,-2.10628459226064));
#70118=CARTESIAN_POINT('Ctrl Pts',(23.1312526780715,2.44275349825157,-2.10216613880255));
#70119=CARTESIAN_POINT('Ctrl Pts',(23.1317831101976,2.4486772012971,-2.09525915706361));
#70120=CARTESIAN_POINT('Ctrl Pts',(23.1319967323168,2.45105633188894,-2.09247552654274));
#70121=CARTESIAN_POINT('Ctrl Pts',(23.1368955426035,2.50546439023643,-2.02859689472836));
#70122=CARTESIAN_POINT('Ctrl Pts',(23.1416579449151,2.55519446275298,-1.96558815729063));
#70123=CARTESIAN_POINT('Ctrl Pts',(23.1474149539825,2.61128333717158,-1.88879266322114));
#70124=CARTESIAN_POINT('Ctrl Pts',(23.14831772023,2.61996480060724,-1.87673195308155));
#70125=CARTESIAN_POINT('Ctrl Pts',(23.1497895262613,2.63393204586875,-1.85704218366912));
#70126=CARTESIAN_POINT('Ctrl Pts',(23.1503565985699,2.63926889459873,-1.84944948385854));
#70127=CARTESIAN_POINT('Ctrl Pts',(23.1513676265266,2.64870429754152,-1.83590178541724));
#70128=CARTESIAN_POINT('Ctrl Pts',(23.1518110844487,2.65281576760036,-1.82995582551362));
#70129=CARTESIAN_POINT('Ctrl Pts',(23.1527454845022,2.66142182386746,-1.81741989281754));
#70130=CARTESIAN_POINT('Ctrl Pts',(23.1532365897923,2.66591201295986,-1.81082697370432));
#70131=CARTESIAN_POINT('Ctrl Pts',(23.1545327889721,2.67767603565589,-1.79341533499788));
#70132=CARTESIAN_POINT('Ctrl Pts',(23.1553394304044,2.68490872422207,-1.78256911515401));
#70133=CARTESIAN_POINT('Ctrl Pts',(23.1590007257693,2.71733716558785,-1.73329394443886));
#70134=CARTESIAN_POINT('Ctrl Pts',(23.1618835639994,2.74177400916559,-1.69437425023957));
#70135=CARTESIAN_POINT('Ctrl Pts',(23.1696533712203,2.80470551953948,-1.58921748167914));
#70136=CARTESIAN_POINT('Ctrl Pts',(23.1745924409433,2.8416828260965,-1.52211117706372));
#70137=CARTESIAN_POINT('Ctrl Pts',(23.2002992224889,3.0189254550657,-1.17143944820518));
#70138=CARTESIAN_POINT('Ctrl Pts',(23.2223046391506,3.1192542758292,-0.86970707193378));
#70139=CARTESIAN_POINT('Ctrl Pts',(23.2467766124118,3.18409092564452,-0.50105169839304));
#70140=CARTESIAN_POINT('Ctrl Pts',(23.2505159017358,3.19260072951787,-0.443609539480715));
#70141=CARTESIAN_POINT('Ctrl Pts',(23.2547988401157,3.20074130740883,-0.376126112401251));
#70142=CARTESIAN_POINT('Ctrl Pts',(23.2554208851005,3.20188277840435,-0.366281925311921));
#70143=CARTESIAN_POINT('Ctrl Pts',(23.2563580268791,3.20354072283646,-0.351383280397276));
#70144=CARTESIAN_POINT('Ctrl Pts',(23.2566749680653,3.20409066992438,-0.346332719164976));
#70145=CARTESIAN_POINT('Ctrl Pts',(23.2572415784886,3.2050545451561,-0.337281926182064));
#70146=CARTESIAN_POINT('Ctrl Pts',(23.2574914969327,3.20547292916926,-0.333282216927065));
#70147=CARTESIAN_POINT('Ctrl Pts',(23.2580289636593,3.20635811414663,-0.324664062596542));
#70148=CARTESIAN_POINT('Ctrl Pts',(23.2583163692893,3.20682242232495,-0.320045406178988));
#70149=CARTESIAN_POINT('Ctrl Pts',(23.2591079549104,3.20807618857256,-0.307296999875901));
#70150=CARTESIAN_POINT('Ctrl Pts',(23.2596109655516,3.20884472814982,-0.299165158145801));
#70151=CARTESIAN_POINT('Ctrl Pts',(23.2623251485984,3.21283802509867,-0.255125716406094));
#70152=CARTESIAN_POINT('Ctrl Pts',(23.2645054727785,3.21549114786066,-0.219167157834597));
#70153=CARTESIAN_POINT('Ctrl Pts',(23.2708796541556,3.22155646974443,-0.112624439867952));
#70154=CARTESIAN_POINT('Ctrl Pts',(23.2749959926902,3.22325161967196,-0.0419609880924475));
#70155=CARTESIAN_POINT('Ctrl Pts',(23.2868345377996,3.22141387676489,0.164352304784546));
#70156=CARTESIAN_POINT('Ctrl Pts',(23.2943837828787,3.21164228892319,0.299793938416747));
#70157=CARTESIAN_POINT('Ctrl Pts',(23.3157394214375,3.16016145118908,0.678395216161542));
#70158=CARTESIAN_POINT('Ctrl Pts',(23.3296159701596,3.09907215242517,0.917915604427136));
#70159=CARTESIAN_POINT('Ctrl Pts',(23.3456731400326,3.00436458876187,1.16631470638774));
#70160=CARTESIAN_POINT('Ctrl Pts',(23.346854426868,2.99726432717949,1.18444210657066));
#70161=CARTESIAN_POINT('Ctrl Pts',(23.3486043934329,2.98655353503294,1.21107426658455));
#70162=CARTESIAN_POINT('Ctrl Pts',(23.3491687852462,2.98306988589865,1.21962984132303));
#70163=CARTESIAN_POINT('Ctrl Pts',(23.3501779681718,2.97678904350251,1.23486720845194));
#70164=CARTESIAN_POINT('Ctrl Pts',(23.350622276325,2.97400600503284,1.24155479649283));
#70165=CARTESIAN_POINT('Ctrl Pts',(23.3515539856964,2.96813296359725,1.2555345461036));
#70166=CARTESIAN_POINT('Ctrl Pts',(23.3520415337854,2.96503858245989,1.26282480526295));
#70167=CARTESIAN_POINT('Ctrl Pts',(23.3533182972775,2.95688035032302,1.28185003348522));
#70168=CARTESIAN_POINT('Ctrl Pts',(23.3541089772319,2.95177354527153,1.29356632777188));
#70169=CARTESIAN_POINT('Ctrl Pts',(23.3575990587936,2.92899428944222,1.34499034597902));
#70170=CARTESIAN_POINT('Ctrl Pts',(23.3603235149241,2.91058999464136,1.3843670623726));
#70171=CARTESIAN_POINT('Ctrl Pts',(23.3675722184112,2.8600270086233,1.48708022067686));
#70172=CARTESIAN_POINT('Ctrl Pts',(23.3721403766003,2.82656244679744,1.54974371134979));
#70173=CARTESIAN_POINT('Ctrl Pts',(23.3948230457243,2.65267870303235,1.85095108828039));
#70174=CARTESIAN_POINT('Ctrl Pts',(23.413879664383,2.48400080679834,2.07181749617703));
#70175=CARTESIAN_POINT('Ctrl Pts',(23.4340191851042,2.2714106132874,2.28636228363493));
#70176=CARTESIAN_POINT('Ctrl Pts',(23.4357006804356,2.25337705599289,2.30413770461221));
#70177=CARTESIAN_POINT('Ctrl Pts',(23.4426113934844,2.1780166587465,2.3766883213659));
#70178=CARTESIAN_POINT('Ctrl Pts',(23.4477622470021,2.11888229736856,2.42955636580153));
#70179=CARTESIAN_POINT('Ctrl Pts',(23.4534514783769,2.04946758375718,2.48715075839427));
#70180=CARTESIAN_POINT('Ctrl Pts',(23.454135858154,2.04104724614253,2.49406543997786));
#70181=CARTESIAN_POINT('Ctrl Pts',(23.4551430796862,2.0285480606304,2.50422392804598));
#70182=CARTESIAN_POINT('Ctrl Pts',(23.4554682491299,2.02449626030841,2.50750066978949));
#70183=CARTESIAN_POINT('Ctrl Pts',(23.4560439036238,2.01729343453775,2.51329684625786));
#70184=CARTESIAN_POINT('Ctrl Pts',(23.4562946710023,2.01414561389936,2.51582020127053));
#70185=CARTESIAN_POINT('Ctrl Pts',(23.4568277961067,2.00743175951343,2.5211814815893));
#70186=CARTESIAN_POINT('Ctrl Pts',(23.4571100345536,2.00386445400851,2.52401774613138));
#70187=CARTESIAN_POINT('Ctrl Pts',(23.4578730362004,1.9941859016861,2.53167943930872));
#70188=CARTESIAN_POINT('Ctrl Pts',(23.4583527659639,1.98806311543579,2.53649034019516));
#70189=CARTESIAN_POINT('Ctrl Pts',(23.4607049111446,1.95786195695651,2.5600439781479));
#70190=CARTESIAN_POINT('Ctrl Pts',(23.4625554945712,1.93353471215768,2.57846704250105));
#70191=CARTESIAN_POINT('Ctrl Pts',(23.4673050996564,1.86974974284247,2.6253610231911));
#70192=CARTESIAN_POINT('Ctrl Pts',(23.4701728763249,1.82990213530993,2.65328910871129));
#70193=CARTESIAN_POINT('Ctrl Pts',(23.4730037159736,1.78943621026388,2.68030513410254));
#70194=CARTESIAN_POINT('Origin',(-1.72497344927317,0.,0.));
#70195=CARTESIAN_POINT('',(24.9668672316986,1.78943621037801,2.68030513402634));
#70196=CARTESIAN_POINT('',(24.7182540045911,1.78943620997144,2.68030513429778));
#70197=CARTESIAN_POINT('',(-1.72497344927317,1.78943621037804,2.68030513402633));
#70198=CARTESIAN_POINT('',(24.1465734493135,-3.22274988426607,-0.000863691533537469));
#70199=CARTESIAN_POINT('Ctrl Pts',(24.1465734493135,-3.22274988426607,-0.000863691533536827));
#70200=CARTESIAN_POINT('Ctrl Pts',(24.1531637169248,-3.22272112126392,-0.108189001818177));
#70201=CARTESIAN_POINT('Ctrl Pts',(24.159753984536,-3.21732684989644,-0.215366678563568));
#70202=CARTESIAN_POINT('Ctrl Pts',(24.1663442521473,-3.20663641291505,-0.321870281118511));
#70203=CARTESIAN_POINT('Ctrl Pts',(24.1729596534758,-3.19590520514317,-0.428780063147113));
#70204=CARTESIAN_POINT('Ctrl Pts',(24.1795750548042,-3.17983745155393,-0.535010296933113));
#70205=CARTESIAN_POINT('Ctrl Pts',(24.1861904561327,-3.15855403786441,-0.640042148917126));
#70206=CARTESIAN_POINT('Ctrl Pts',(24.1928189663141,-3.13722844969058,-0.745282128425083));
#70207=CARTESIAN_POINT('Ctrl Pts',(24.1994474764955,-3.11066664840652,-0.849318665726976));
#70208=CARTESIAN_POINT('Ctrl Pts',(24.2060759866769,-3.07903932648084,-0.951648248295786));
#70209=CARTESIAN_POINT('Ctrl Pts',(24.2127248996135,-3.04731465470002,-1.05429280442014));
#70210=CARTESIAN_POINT('Ctrl Pts',(24.2193738125501,-3.01049338766873,-1.15521958537512));
#70211=CARTESIAN_POINT('Ctrl Pts',(24.2260227254866,-2.96879493299132,-1.25394346297792));
#70212=CARTESIAN_POINT('Ctrl Pts',(24.2294319632594,-2.94741400228757,-1.30456424502275));
#70213=CARTESIAN_POINT('Ctrl Pts',(24.2328412010322,-2.92475153766232,-1.35460625311269));
#70214=CARTESIAN_POINT('Ctrl Pts',(24.2362504388049,-2.90084168137317,-1.40400680272856));
#70215=CARTESIAN_POINT('Ctrl Pts',(24.2424226868977,-2.85755412717028,-1.4934439345661));
#70216=CARTESIAN_POINT('Ctrl Pts',(24.2485949349905,-2.8100502931654,-1.58103468319132));
#70217=CARTESIAN_POINT('Ctrl Pts',(24.2547671830832,-2.75851067542112,-1.66635422887444));
#70218=CARTESIAN_POINT('Ctrl Pts',(24.2609310717359,-2.70704086082516,-1.75155822125774));
#70219=CARTESIAN_POINT('Ctrl Pts',(24.2670949603885,-2.65154634918866,-1.83449675610624));
#70220=CARTESIAN_POINT('Ctrl Pts',(24.2732588490411,-2.59225471131267,-1.91476710703345));
#70221=CARTESIAN_POINT('Ctrl Pts',(24.2794162106997,-2.53302585785589,-1.99495245900393));
#70222=CARTESIAN_POINT('Ctrl Pts',(24.2855735723582,-2.47000812856508,-2.07247489667289));
#70223=CARTESIAN_POINT('Ctrl Pts',(24.2917309340168,-2.40347329903488,-2.14695916666489));
#70224=CARTESIAN_POINT('Ctrl Pts',(24.2978837981631,-2.33698706843832,-2.22138903122562));
#70225=CARTESIAN_POINT('Ctrl Pts',(24.3040366623094,-2.26698913369767,-2.29278481721412));
#70226=CARTESIAN_POINT('Ctrl Pts',(24.3101895264557,-2.19379201543417,-2.36080370965425));
#70227=CARTESIAN_POINT('Ctrl Pts',(24.3163400595923,-2.12062262786547,-2.42879683316808));
#70228=CARTESIAN_POINT('Ctrl Pts',(24.3224905927288,-2.04425678287511,-2.49341530980454));
#70229=CARTESIAN_POINT('Ctrl Pts',(24.3286411258654,-1.96504375180514,-2.55435326765731));
#70230=CARTESIAN_POINT('Ctrl Pts',(24.3347909740806,-1.88583954187208,-2.61528443947927));
#70231=CARTESIAN_POINT('Ctrl Pts',(24.3409408222958,-1.80378912051081,-2.67253564252502));
#70232=CARTESIAN_POINT('Ctrl Pts',(24.347090670511,-1.71927392123948,-2.72584202518155));
#70233=CARTESIAN_POINT('Ctrl Pts',(24.3532414788901,-1.63474552677318,-2.77915673046072));
#70234=CARTESIAN_POINT('Ctrl Pts',(24.3593922872693,-1.54775195747746,-2.82852516026726));
#70235=CARTESIAN_POINT('Ctrl Pts',(24.3655430956484,-1.45870176115706,-2.87372697633183));
#70236=CARTESIAN_POINT('Ctrl Pts',(24.3717004820146,-1.36955633003137,-2.91897713351556));
#70237=CARTESIAN_POINT('Ctrl Pts',(24.3778578683808,-1.27835026787136,-2.96005158181559));
#70238=CARTESIAN_POINT('Ctrl Pts',(24.384015254747,-1.18551464409404,-2.99677703393806));
#70239=CARTESIAN_POINT('Ctrl Pts',(24.3901760774839,-1.09262720975868,-3.03352298213834));
#70240=CARTESIAN_POINT('Ctrl Pts',(24.3963369002209,-0.9981088135955,-3.06591495974254));
#70241=CARTESIAN_POINT('Ctrl Pts',(24.4024977229579,-0.902406329458462,
-3.0938294036765));
#70242=CARTESIAN_POINT('Ctrl Pts',(24.4086688458745,-0.806543841888507,
-3.12179051731708));
#70243=CARTESIAN_POINT('Ctrl Pts',(24.4148399687912,-0.709493734442499,
-3.14525904225619));
#70244=CARTESIAN_POINT('Ctrl Pts',(24.4210110917079,-0.61171386643955,-3.16416240229631));
#70245=CARTESIAN_POINT('Ctrl Pts',(24.4257066136534,-0.537314519313144,
-3.17854570710338));
#70246=CARTESIAN_POINT('Ctrl Pts',(24.430402135599,-0.462492905727497,-3.19028707697477));
#70247=CARTESIAN_POINT('Ctrl Pts',(24.4350976575445,-0.387451761467251,
-3.19937473501244));
#70248=CARTESIAN_POINT('Ctrl Pts',(24.4412699056373,-0.288810425123307,
-3.21132043149547));
#70249=CARTESIAN_POINT('Ctrl Pts',(24.44744215373,-0.189442497136187,-3.21872099751619));
#70250=CARTESIAN_POINT('Ctrl Pts',(24.4536144018228,-0.0898029357186574,
-3.22149856359371));
#70251=CARTESIAN_POINT('Ctrl Pts',(24.4597782904754,0.009701677955975,-3.22427236784944));
#70252=CARTESIAN_POINT('Ctrl Pts',(24.4659421791281,0.109476763457256,-3.22243560499243));
#70253=CARTESIAN_POINT('Ctrl Pts',(24.4721060677807,0.209060493896643,-3.21596195132836));
#70254=CARTESIAN_POINT('Ctrl Pts',(24.4782634294392,0.308538774277512,-3.20949515267117));
#70255=CARTESIAN_POINT('Ctrl Pts',(24.4844207910978,0.407825671368895,-3.19840125285889));
#70256=CARTESIAN_POINT('Ctrl Pts',(24.4905781527563,0.506458566839546,-3.18270596860201));
#70257=CARTESIAN_POINT('Ctrl Pts',(24.4967310169026,0.605019418035451,-3.16702214862756));
#70258=CARTESIAN_POINT('Ctrl Pts',(24.5028838810489,0.702926789677983,-3.14674369447273));
#70259=CARTESIAN_POINT('Ctrl Pts',(24.5090367451952,0.799723319653441,-3.12194813770224));
#70260=CARTESIAN_POINT('Ctrl Pts',(24.5151872783318,0.896483178307803,-3.09716197471709));
#70261=CARTESIAN_POINT('Ctrl Pts',(24.5213378114683,0.992132611183931,-3.06786221713491));
#70262=CARTESIAN_POINT('Ctrl Pts',(24.5274883446048,1.08622546151676,-3.03417728705043));
#70263=CARTESIAN_POINT('Ctrl Pts',(24.53363819282,1.18030783370098,-3.0004961081086));
#70264=CARTESIAN_POINT('Ctrl Pts',(24.5397880410353,1.27283355900908,-2.96243087394459));
#70265=CARTESIAN_POINT('Ctrl Pts',(24.5459378892505,1.36337359689445,-2.92015924185499));
#70266=CARTESIAN_POINT('Ctrl Pts',(24.5520886976296,1.45392777062112,-2.87788100997709));
#70267=CARTESIAN_POINT('Ctrl Pts',(24.5582395060087,1.54249524751428,-2.83139525950301));
#70268=CARTESIAN_POINT('Ctrl Pts',(24.5643903143879,1.62866977107641,-2.78092652532963));
#70269=CARTESIAN_POINT('Ctrl Pts',(24.5705477007541,1.71493645405328,-2.73040381732719));
#70270=CARTESIAN_POINT('Ctrl Pts',(24.5767050871202,1.79880469779382,-2.67588983958058));
#70271=CARTESIAN_POINT('Ctrl Pts',(24.5828624734864,1.87989564783416,-2.61765351331191));
#70272=CARTESIAN_POINT('Ctrl Pts',(24.5890232962234,1.96103185385717,-2.55938468597905));
#70273=CARTESIAN_POINT('Ctrl Pts',(24.5951841189604,2.03938733876293,-2.49738964253551));
#70274=CARTESIAN_POINT('Ctrl Pts',(24.6013449416973,2.11461653092351,-2.43197748543135));
#70275=CARTESIAN_POINT('Ctrl Pts',(24.607516064614,2.18997149755173,-2.36645596680145));
#70276=CARTESIAN_POINT('Ctrl Pts',(24.6136871875307,2.26218941674399,-2.29750622303378));
#70277=CARTESIAN_POINT('Ctrl Pts',(24.6198583104474,2.33096166753404,-2.22547416677591));
#70278=CARTESIAN_POINT('Ctrl Pts',(24.624553832393,2.38328952053481,-2.17066597294912));
#70279=CARTESIAN_POINT('Ctrl Pts',(24.6292493543386,2.43362327811525,-2.11407404354159));
#70280=CARTESIAN_POINT('Ctrl Pts',(24.6339448762842,2.4818434121291,-2.05586255381321));
#70281=CARTESIAN_POINT('Ctrl Pts',(24.640117124377,2.54522861906614,-1.97934374278115));
#70282=CARTESIAN_POINT('Ctrl Pts',(24.6462893724698,2.60518329728354,-1.89975611780241));
#70283=CARTESIAN_POINT('Ctrl Pts',(24.6524616205625,2.6613959417158,-1.8174402889555));
#70284=CARTESIAN_POINT('Ctrl Pts',(24.6586255092152,2.71753245404368,-1.73523594529733));
#70285=CARTESIAN_POINT('Ctrl Pts',(24.6647893978678,2.76993676310318,-1.65031109748117));
#70286=CARTESIAN_POINT('Ctrl Pts',(24.6709532865204,2.8183370106406,-1.56304000491138));
#70287=CARTESIAN_POINT('Ctrl Pts',(24.677110648179,2.86668600674453,-1.47586132444329));
#70288=CARTESIAN_POINT('Ctrl Pts',(24.6832680098375,2.91103916120595,-1.38634171633193));
#70289=CARTESIAN_POINT('Ctrl Pts',(24.6894253714961,2.95116796468241,-1.29488424453009));
#70290=CARTESIAN_POINT('Ctrl Pts',(24.6955782356424,2.99126745693846,-1.20349357586919));
#70291=CARTESIAN_POINT('Ctrl Pts',(24.7017310997887,3.02714855887914,-1.11016825428707));
#70292=CARTESIAN_POINT('Ctrl Pts',(24.707883963935,3.05862919036995,-1.01533493898166));
#70293=CARTESIAN_POINT('Ctrl Pts',(24.7140344970716,3.0900978954379,-0.920537551234397));
#70294=CARTESIAN_POINT('Ctrl Pts',(24.7201850302081,3.11716930590786,-0.824233716736039));
#70295=CARTESIAN_POINT('Ctrl Pts',(24.7263355633447,3.13971021005953,-0.72686818567603));
#70296=CARTESIAN_POINT('Ctrl Pts',(24.7324854115599,3.16224860406359,-0.629513497209272));
#70297=CARTESIAN_POINT('Ctrl Pts',(24.7386352597751,3.18025739682994,-0.531097770422997));
#70298=CARTESIAN_POINT('Ctrl Pts',(24.7447851079903,3.19365404864355,-0.432077979168888));
#70299=CARTESIAN_POINT('Ctrl Pts',(24.7509359163694,3.20705279205054,-0.333042728145924));
#70300=CARTESIAN_POINT('Ctrl Pts',(24.7570867247486,3.21583790598795,-0.233403655822401));
#70301=CARTESIAN_POINT('Ctrl Pts',(24.7632375331277,3.21997860416463,-0.133623917103257));
#70302=CARTESIAN_POINT('Ctrl Pts',(24.7693949194939,3.22412373061435,-0.0337374688609638));
#70303=CARTESIAN_POINT('Ctrl Pts',(24.7755523058601,3.22361450472336,0.0662895113338177));
#70304=CARTESIAN_POINT('Ctrl Pts',(24.7817096922263,3.21847229493312,0.165992919270579));
#70305=CARTESIAN_POINT('Ctrl Pts',(24.7878705149633,3.21332721533117,0.265751970601542));
#70306=CARTESIAN_POINT('Ctrl Pts',(24.7940313377002,3.20354404514045,0.365186657745472));
#70307=CARTESIAN_POINT('Ctrl Pts',(24.8001921604372,3.18919594997975,0.463839147908784));
#70308=CARTESIAN_POINT('Ctrl Pts',(24.8063632833539,3.17482386647119,0.562656573572241));
#70309=CARTESIAN_POINT('Ctrl Pts',(24.8125344062706,3.15587169574759,0.660688763402786));
#70310=CARTESIAN_POINT('Ctrl Pts',(24.8187055291873,3.13246354809509,0.757489064182118));
#70311=CARTESIAN_POINT('Ctrl Pts',(24.8234010511328,3.1146526127936,0.831143072177134));
#70312=CARTESIAN_POINT('Ctrl Pts',(24.8280965730784,3.09426295540948,0.904084113421489));
#70313=CARTESIAN_POINT('Ctrl Pts',(24.8327920950239,3.07136805154229,0.97612286852903));
#70314=CARTESIAN_POINT('Ctrl Pts',(24.838963105624,3.04127880990082,1.07079858861741));
#70315=CARTESIAN_POINT('Ctrl Pts',(24.845134116224,3.00675491308035,1.16424834859305));
#70316=CARTESIAN_POINT('Ctrl Pts',(24.8513051268241,2.96791437521401,1.25602620350772));
#70317=CARTESIAN_POINT('Ctrl Pts',(24.8574683454387,2.92912288035311,1.34768817275023));
#70318=CARTESIAN_POINT('Ctrl Pts',(24.8636315640533,2.88602574101968,1.43768203499338));
#70319=CARTESIAN_POINT('Ctrl Pts',(24.869794782668,2.83879072369699,1.52557687107268));
#70320=CARTESIAN_POINT('Ctrl Pts',(24.8759518684649,2.79160270839798,1.61338424587008));
#70321=CARTESIAN_POINT('Ctrl Pts',(24.8821089542619,2.74028520233278,1.69909636506283));
#70322=CARTESIAN_POINT('Ctrl Pts',(24.8882660400589,2.68505366458286,1.78230311137308));
#70323=CARTESIAN_POINT('Ctrl Pts',(24.8944186464997,2.62986230846105,1.86544932374433));
#70324=CARTESIAN_POINT('Ctrl Pts',(24.9005712529404,2.57076282129297,1.94609342622972));
#70325=CARTESIAN_POINT('Ctrl Pts',(24.9067238593812,2.50801561081939,2.02385159001006));
#70326=CARTESIAN_POINT('Ctrl Pts',(24.9128742926136,2.44529056375954,2.10158228824505));
#70327=CARTESIAN_POINT('Ctrl Pts',(24.919024725846,2.37892062463272,2.17642873457796));
#70328=CARTESIAN_POINT('Ctrl Pts',(24.9251751590784,2.30920786141307,2.24803839275224));
#70329=CARTESIAN_POINT('Ctrl Pts',(24.931324399548,2.23950861769477,2.31963416355747));
#70330=CARTESIAN_POINT('Ctrl Pts',(24.9374736400177,2.1664681453471,2.38799408663982));
#70331=CARTESIAN_POINT('Ctrl Pts',(24.9436228804873,2.09042610766343,2.45280171454994));
#70332=CARTESIAN_POINT('Ctrl Pts',(24.949773879861,2.0143623192193,2.51762787977487));
#70333=CARTESIAN_POINT('Ctrl Pts',(24.9559248792348,1.93529558449351,2.57889944242733));
#70334=CARTESIAN_POINT('Ctrl Pts',(24.9620758786086,1.85359888667893,2.63634002545245));
#70335=CARTESIAN_POINT('Ctrl Pts',(24.9636729963052,1.83238619685259,2.65125457284238));
#70336=CARTESIAN_POINT('Ctrl Pts',(24.9652701140019,1.81099635528114,2.6659110624332));
#70337=CARTESIAN_POINT('Ctrl Pts',(24.9668672316986,1.78943621037801,2.68030513402634));
#70338=CARTESIAN_POINT('Ctrl Pts',(23.7170278226866,1.78943621037803,2.68030513402633));
#70339=CARTESIAN_POINT('Ctrl Pts',(23.7231781072839,1.70635511262692,2.73577207427372));
#70340=CARTESIAN_POINT('Ctrl Pts',(23.7293283918812,1.62066068072026,2.78739386047531));
#70341=CARTESIAN_POINT('Ctrl Pts',(23.7354786764785,1.53274737844311,2.83492557863091));
#70342=CARTESIAN_POINT('Ctrl Pts',(23.7416285775026,1.44483955903163,2.88245433238841));
#70343=CARTESIAN_POINT('Ctrl Pts',(23.7477784785267,1.35471352665834,2.92589331889868));
#70344=CARTESIAN_POINT('Ctrl Pts',(23.7539283795508,1.26278875004462,2.96504336144697));
#70345=CARTESIAN_POINT('Ctrl Pts',(23.7600795420464,1.17084511776445,3.00420143447595));
#70346=CARTESIAN_POINT('Ctrl Pts',(23.766230704542,1.0771024079397,3.03906864569759));
#70347=CARTESIAN_POINT('Ctrl Pts',(23.7723818670376,0.98199954061988,3.06949417082397));
#70348=CARTESIAN_POINT('Ctrl Pts',(23.7785397717703,0.886792431852533,3.0999530451108));
#70349=CARTESIAN_POINT('Ctrl Pts',(23.784697676503,0.790222603632329,3.12596038125505));
#70350=CARTESIAN_POINT('Ctrl Pts',(23.7908555812357,0.692743449068784,3.14741545974984));
#70351=CARTESIAN_POINT('Ctrl Pts',(23.7970171931663,0.595205609849946,3.16888345468704));
#70352=CARTESIAN_POINT('Ctrl Pts',(23.8031788050969,0.496757782115097,3.18579366173425));
#70353=CARTESIAN_POINT('Ctrl Pts',(23.8093404170274,0.397860790924237,3.19809698938996));
#70354=CARTESIAN_POINT('Ctrl Pts',(23.8155119924076,0.298803881322749,3.21042021177231));
#70355=CARTESIAN_POINT('Ctrl Pts',(23.8216835677878,0.199296790707494,3.2181216466416));
#70356=CARTESIAN_POINT('Ctrl Pts',(23.827855143168,0.0998026789936531,3.22120427600699));
#70357=CARTESIAN_POINT('Ctrl Pts',(23.8314220958872,0.0422985944674917,
3.22298592696639));
#70358=CARTESIAN_POINT('Ctrl Pts',(23.8349890486064,-0.0152011876087444,
3.22322566903398));
#70359=CARTESIAN_POINT('Ctrl Pts',(23.8385560013256,-0.072608098951784,
3.22193197111091));
#70360=CARTESIAN_POINT('Ctrl Pts',(23.8447282494184,-0.171944907410476,
3.21969335872468));
#70361=CARTESIAN_POINT('Ctrl Pts',(23.8509004975111,-0.271352932954708,
3.21285245620611));
#70362=CARTESIAN_POINT('Ctrl Pts',(23.8570727456039,-0.370370763169425,
3.20139704821025));
#70363=CARTESIAN_POINT('Ctrl Pts',(23.8632366342565,-0.469254487688776,
3.18995715494998));
#70364=CARTESIAN_POINT('Ctrl Pts',(23.8694005229092,-0.567748639562157,
3.17391522765422));
#70365=CARTESIAN_POINT('Ctrl Pts',(23.8755644115618,-0.665392356215619,
3.15331104948272));
#70366=CARTESIAN_POINT('Ctrl Pts',(23.8817217732204,-0.762932677107381,
3.13272868925066));
#70367=CARTESIAN_POINT('Ctrl Pts',(23.8878791348789,-0.859623930451618,
3.10759377182921));
#70368=CARTESIAN_POINT('Ctrl Pts',(23.8940364965375,-0.955011889189508,
3.0779977020795));
#70369=CARTESIAN_POINT('Ctrl Pts',(23.9001893606838,-1.05033017384695,3.04842325014164));
#70370=CARTESIAN_POINT('Ctrl Pts',(23.9063422248301,-1.14434664294999,3.01439425276787));
#70371=CARTESIAN_POINT('Ctrl Pts',(23.9124950889764,-1.23661965869101,2.97605265112009));
#70372=CARTESIAN_POINT('Ctrl Pts',(23.9186456221129,-1.32885771684211,2.93772557517061));
#70373=CARTESIAN_POINT('Ctrl Pts',(23.9247961552494,-1.41935323337495,2.89508930784641));
#70374=CARTESIAN_POINT('Ctrl Pts',(23.930946688386,-1.50768291632923,2.84833456361941));
#70375=CARTESIAN_POINT('Ctrl Pts',(23.9370965366012,-1.59600276291951,2.80158502598512));
#70376=CARTESIAN_POINT('Ctrl Pts',(23.9432463848164,-1.68215687153482,2.75071812648771));
#70377=CARTESIAN_POINT('Ctrl Pts',(23.9493962330316,-1.76574591057609,2.6959708718352));
#70378=CARTESIAN_POINT('Ctrl Pts',(23.9555470414107,-1.84934800021229,2.64121506959975));
#70379=CARTESIAN_POINT('Ctrl Pts',(23.9616978497899,-1.93038386141096,2.58257794688646));
#70380=CARTESIAN_POINT('Ctrl Pts',(23.967848658169,-2.00848339677528,2.52033966111277));
#70381=CARTESIAN_POINT('Ctrl Pts',(23.9740060445352,-2.08666645575175,2.45803481455332));
#70382=CARTESIAN_POINT('Ctrl Pts',(23.9801634309013,-2.161906577763,2.39212138559079));
#70383=CARTESIAN_POINT('Ctrl Pts',(23.9863208172675,-2.2338671152758,2.32291955818306));
#70384=CARTESIAN_POINT('Ctrl Pts',(23.9924816400045,-2.30586781318681,2.25367910998342));
#70385=CARTESIAN_POINT('Ctrl Pts',(23.9986424627415,-2.37458498282635,2.181146923865));
#70386=CARTESIAN_POINT('Ctrl Pts',(24.0048032854784,-2.4397206477835,2.10567820981243));
#70387=CARTESIAN_POINT('Ctrl Pts',(24.0109744083951,-2.50496521200365,2.03008332083947));
#70388=CARTESIAN_POINT('Ctrl Pts',(24.0171455313118,-2.56661604264621,1.95154243913336));
#70389=CARTESIAN_POINT('Ctrl Pts',(24.0233166542285,-2.62441698421198,1.8704419412213));
#70390=CARTESIAN_POINT('Ctrl Pts',(24.0280121761741,-2.6683969199973,1.80873369575489));
#70391=CARTESIAN_POINT('Ctrl Pts',(24.0327076981197,-2.71014883855629,1.7455442114804));
#70392=CARTESIAN_POINT('Ctrl Pts',(24.0374032200653,-2.74957783738817,1.6810530267198));
#70393=CARTESIAN_POINT('Ctrl Pts',(24.0437674626396,-2.80301933248364,1.5936426070746));
#70394=CARTESIAN_POINT('Ctrl Pts',(24.0501317052139,-2.85237038776646,1.50354830229794));
#70395=CARTESIAN_POINT('Ctrl Pts',(24.0564959477882,-2.89736080226112,1.41117608540565));
#70396=CARTESIAN_POINT('Ctrl Pts',(24.0628497727577,-2.94227757211535,1.31895507224808));
#70397=CARTESIAN_POINT('Ctrl Pts',(24.0692035977272,-2.98284773162445,1.22446392104366));
#70398=CARTESIAN_POINT('Ctrl Pts',(24.0755574226967,-3.01884531640117,1.12813585978937));
#70399=CARTESIAN_POINT('Ctrl Pts',(24.0818993142109,-3.05477529220661,1.0319887173708));
#70400=CARTESIAN_POINT('Ctrl Pts',(24.0882412057251,-3.08614966305172,0.934011907863526));
#70401=CARTESIAN_POINT('Ctrl Pts',(24.0945830972393,-3.11278969277883,0.834660344709092));
#70402=CARTESIAN_POINT('Ctrl Pts',(24.1009179698234,-3.13940023847785,0.735418739550518));
#70403=CARTESIAN_POINT('Ctrl Pts',(24.1072528424075,-3.1612867648525,0.634805789739645));
#70404=CARTESIAN_POINT('Ctrl Pts',(24.1135877149915,-3.17831959942743,0.53329362118393));
#70405=CARTESIAN_POINT('Ctrl Pts',(24.1199153215362,-3.19533289750103,0.431897886132405));
#70406=CARTESIAN_POINT('Ctrl Pts',(24.1262429280809,-3.20750352637341,0.329605377401343));
#70407=CARTESIAN_POINT('Ctrl Pts',(24.1325705346256,-3.21475257350628,0.226899655431163));
#70408=CARTESIAN_POINT('Ctrl Pts',(24.1372381728414,-3.22009992391228,0.151137493313834));
#70409=CARTESIAN_POINT('Ctrl Pts',(24.1419058110573,-3.2227702560013,0.0751507821873924));
#70410=CARTESIAN_POINT('Ctrl Pts',(24.1465734492731,-3.22274988426624,-0.000863690875605038));
#70411=CARTESIAN_POINT('',(23.8997658991183,-3.22274856360171,0.00296078655014494));
#70412=CARTESIAN_POINT('Ctrl Pts',(23.4730037159736,1.78943621026388,2.68030513410254));
#70413=CARTESIAN_POINT('Ctrl Pts',(23.4734202769121,1.78348160816408,2.68428056976452));
#70414=CARTESIAN_POINT('Ctrl Pts',(23.4738360373049,1.77751361735375,2.68823625624975));
#70415=CARTESIAN_POINT('Ctrl Pts',(23.4858998166118,1.6036433398868,2.80264826426368));
#70416=CARTESIAN_POINT('Ctrl Pts',(23.4969429837364,1.42577717955715,2.89718490302514));
#70417=CARTESIAN_POINT('Ctrl Pts',(23.519539157923,1.05435708852739,3.05205071370242));
#70418=CARTESIAN_POINT('Ctrl Pts',(23.5310521832852,0.861633880524336,3.1119531568544));
#70419=CARTESIAN_POINT('Ctrl Pts',(23.5442947945494,0.647027675885696,3.15718151956633));
#70420=CARTESIAN_POINT('Ctrl Pts',(23.5453835197282,0.629427807902366,3.16073734678112));
#70421=CARTESIAN_POINT('Ctrl Pts',(23.5470354604113,0.60279463602389,3.16588696999589));
#70422=CARTESIAN_POINT('Ctrl Pts',(23.5475952029045,0.59378253929595,3.16758961567034));
#70423=CARTESIAN_POINT('Ctrl Pts',(23.5485700164668,0.578109659940522,3.1704814401998));
#70424=CARTESIAN_POINT('Ctrl Pts',(23.5489845257417,0.571452140823291,3.17168816109181));
#70425=CARTESIAN_POINT('Ctrl Pts',(23.5498501047665,0.55756457541276,3.17416023245832));
#70426=CARTESIAN_POINT('Ctrl Pts',(23.5503012903154,0.550333914612286,3.17542186458456));
#70427=CARTESIAN_POINT('Ctrl Pts',(23.5511989632057,0.535964674634535,3.17787850887425));
#70428=CARTESIAN_POINT('Ctrl Pts',(23.5516454261434,0.52882625330304,3.17907419574772));
#70429=CARTESIAN_POINT('Ctrl Pts',(23.5531490752581,0.504812778821286,3.18301333882105));
#70430=CARTESIAN_POINT('Ctrl Pts',(23.5542097575234,0.487920159737118,3.18564652093662));
#70431=CARTESIAN_POINT('Ctrl Pts',(23.5620983688909,0.362643093973924,3.20415460434085));
#70432=CARTESIAN_POINT('Ctrl Pts',(23.5690965471975,0.253544721579583,3.21462706749474));
#70433=CARTESIAN_POINT('Ctrl Pts',(23.5898330579131,-0.0637114018025083,
3.22883028399124));
#70434=CARTESIAN_POINT('Ctrl Pts',(23.6039565164935,-0.271951545080688,
3.21798517370643));
#70435=CARTESIAN_POINT('Ctrl Pts',(23.6235097243725,-0.55808966105122,3.17510107928485));
#70436=CARTESIAN_POINT('Ctrl Pts',(23.6289827422467,-0.638032406726126,
3.16000738112245));
#70437=CARTESIAN_POINT('Ctrl Pts',(23.6402207486007,-0.803263558192448,
3.12228382219302));
#70438=CARTESIAN_POINT('Ctrl Pts',(23.6459672121217,-0.888373604689581,
3.09914247916298));
#70439=CARTESIAN_POINT('Ctrl Pts',(23.652226583463,-0.982953433679048,3.06920866357304));
#70440=CARTESIAN_POINT('Ctrl Pts',(23.6529197591336,-0.993454501059695,
3.06582573477126));
#70441=CARTESIAN_POINT('Ctrl Pts',(23.6539387951978,-1.0089355553054,3.06075060493413));
#70442=CARTESIAN_POINT('Ctrl Pts',(23.6542670430012,-1.01392896772216,3.05910007513883));
#70443=CARTESIAN_POINT('Ctrl Pts',(23.6548469012831,-1.02276230808496,3.05615628537534));
#70444=CARTESIAN_POINT('Ctrl Pts',(23.6550988041043,-1.02660386155545,3.05486799905329));
#70445=CARTESIAN_POINT('Ctrl Pts',(23.6556284195854,-1.03468949533506,3.05213946218425));
#70446=CARTESIAN_POINT('Ctrl Pts',(23.6559060348698,-1.03893299233638,3.05069760651524));
#70447=CARTESIAN_POINT('Ctrl Pts',(23.6566435939825,-1.0502201754883,3.04683616441141));
#70448=CARTESIAN_POINT('Ctrl Pts',(23.6571026192863,-1.05725855699463,3.04440098804741));
#70449=CARTESIAN_POINT('Ctrl Pts',(23.6591987978795,-1.08945879916625,3.03313504193927));
#70450=CARTESIAN_POINT('Ctrl Pts',(23.6608194656517,-1.11451977263808,3.02401627680815));
#70451=CARTESIAN_POINT('Ctrl Pts',(23.6652122739396,-1.18278914021981,2.99821155030078));
#70452=CARTESIAN_POINT('Ctrl Pts',(23.6679525952223,-1.22575694448039,2.98090305390752));
#70453=CARTESIAN_POINT('Ctrl Pts',(23.6772013109621,-1.37133905243744,2.91857844963009));
#70454=CARTESIAN_POINT('Ctrl Pts',(23.6835343424194,-1.47197704944423,2.8691388935788));
#70455=CARTESIAN_POINT('Ctrl Pts',(23.6968768182774,-1.67975815318856,2.75324724807418));
#70456=CARTESIAN_POINT('Ctrl Pts',(23.7038636801026,-1.78598835084015,2.68555455362677));
#70457=CARTESIAN_POINT('Ctrl Pts',(23.721035208545,-2.03269792462533,2.50721762445044));
#70458=CARTESIAN_POINT('Ctrl Pts',(23.7313172082078,-2.16844439892737,2.39078160784915));
#70459=CARTESIAN_POINT('Ctrl Pts',(23.7431740645832,-2.30636372838925,2.25102681506842));
#70460=CARTESIAN_POINT('Ctrl Pts',(23.7442550904329,-2.31878012850893,2.23823458683127));
#70461=CARTESIAN_POINT('Ctrl Pts',(23.7458972905683,-2.33739995522785,2.21872993587714));
#70462=CARTESIAN_POINT('Ctrl Pts',(23.74645504988,-2.34368214618957,2.21209291712265));
#70463=CARTESIAN_POINT('Ctrl Pts',(23.7474273765545,-2.35456050885437,2.20050176999303));
#70464=CARTESIAN_POINT('Ctrl Pts',(23.7478413892577,-2.35916950724096,2.19555971556253));
#70465=CARTESIAN_POINT('Ctrl Pts',(23.7487068759005,-2.36875645519572,2.18521495226659));
#70466=CARTESIAN_POINT('Ctrl Pts',(23.7491584686572,-2.37373153838157,2.17980965084313));
#70467=CARTESIAN_POINT('Ctrl Pts',(23.7500572640548,-2.38357915797364,2.16903677065179));
#70468=CARTESIAN_POINT('Ctrl Pts',(23.7505044433147,-2.38845215223162,2.16366966746083));
#70469=CARTESIAN_POINT('Ctrl Pts',(23.7515507192917,-2.39979152802698,2.15109552088826));
#70470=CARTESIAN_POINT('Ctrl Pts',(23.7521504149913,-2.40624359415899,2.14387571474019));
#70471=CARTESIAN_POINT('Ctrl Pts',(23.7556466170595,-2.4435826896545,2.1017126919765));
#70472=CARTESIAN_POINT('Ctrl Pts',(23.7585733458551,-2.47373949083719,2.06613290091525));
#70473=CARTESIAN_POINT('Ctrl Pts',(23.7693838315092,-2.58108875235739,1.93375909647533));
#70474=CARTESIAN_POINT('Ctrl Pts',(23.777452816576,-2.65345106903884,1.83320337967078));
#70475=CARTESIAN_POINT('Ctrl Pts',(23.7919379743233,-2.7703705691159,1.64925325253249));
#70476=CARTESIAN_POINT('Ctrl Pts',(23.7982798247324,-2.81738467775259,1.56758779303045));
#70477=CARTESIAN_POINT('Ctrl Pts',(23.8090474016848,-2.89070842740288,1.42623782647081));
#70478=CARTESIAN_POINT('Ctrl Pts',(23.8134562506303,-2.91890847782342,1.36759748203578));
#70479=CARTESIAN_POINT('Ctrl Pts',(23.8288854891508,-3.01162955033319,1.15883395869922));
#70480=CARTESIAN_POINT('Ctrl Pts',(23.8398164531355,-3.06650388294999,1.00467722062702));
#70481=CARTESIAN_POINT('Ctrl Pts',(23.8508960753897,-3.11261056089464,0.835414503846904));
#70482=CARTESIAN_POINT('Ctrl Pts',(23.8516514028684,-3.11570328980735,0.823805145425565));
#70483=CARTESIAN_POINT('Ctrl Pts',(23.852738723673,-3.12008312673824,0.806986757929483));
#70484=CARTESIAN_POINT('Ctrl Pts',(23.8530736454099,-3.12142221626237,0.801791552741193));
#70485=CARTESIAN_POINT('Ctrl Pts',(23.8536611878988,-3.12375382013524,0.79265136161246));
#70486=CARTESIAN_POINT('Ctrl Pts',(23.8539141272245,-3.1247518464717,0.788707809388391));
#70487=CARTESIAN_POINT('Ctrl Pts',(23.8544416041466,-3.12682115478272,0.780465664475319));
#70488=CARTESIAN_POINT('Ctrl Pts',(23.8547160600656,-3.12789103888566,0.77616675839975));
#70489=CARTESIAN_POINT('Ctrl Pts',(23.8554362523553,-3.13068041336807,0.764859325197769));
#70490=CARTESIAN_POINT('Ctrl Pts',(23.85588114546,-3.13238524575619,0.757847156438468));
#70491=CARTESIAN_POINT('Ctrl Pts',(23.8568506860056,-3.13605999388658,0.742508242486001));
#70492=CARTESIAN_POINT('Ctrl Pts',(23.8573747995252,-3.13802033716632,0.734179230652083));
#70493=CARTESIAN_POINT('Ctrl Pts',(23.8589236345457,-3.14373463389994,0.709459550834804));
#70494=CARTESIAN_POINT('Ctrl Pts',(23.8599432893267,-3.14739357108795,0.693046923359981));
#70495=CARTESIAN_POINT('Ctrl Pts',(23.8746023698498,-3.19846082195336,0.455229022660595));
#70496=CARTESIAN_POINT('Ctrl Pts',(23.8871028727178,-3.22254052557432,0.229433624789051));
#70497=CARTESIAN_POINT('Ctrl Pts',(23.8997657266517,-3.2227486392817,0.00296150433855287));
#70498=CARTESIAN_POINT('Ctrl Pts',(23.8997657671943,-3.22274863994794,0.00296077924363577));
#70499=CARTESIAN_POINT('Ctrl Pts',(23.9124220347313,-3.22295659447685,-0.223393541721828));
#70500=CARTESIAN_POINT('Ctrl Pts',(23.9251913555592,-3.1993184214291,-0.449116445071595));
#70501=CARTESIAN_POINT('Ctrl Pts',(23.9399233137839,-3.14827503912222,-0.689088641369014));
#70502=CARTESIAN_POINT('Ctrl Pts',(23.9410697476223,-3.14415599829387,-0.707645329609252));
#70503=CARTESIAN_POINT('Ctrl Pts',(23.9428931480142,-3.13737487243252,-0.736966349291988));
#70504=CARTESIAN_POINT('Ctrl Pts',(23.9435666652802,-3.13482093605246,-0.747755430789164));
#70505=CARTESIAN_POINT('Ctrl Pts',(23.9448532600821,-3.12984921186356,-0.768285232313295));
#70506=CARTESIAN_POINT('Ctrl Pts',(23.9454660080507,-3.12744149242713,-0.778028273942384));
#70507=CARTESIAN_POINT('Ctrl Pts',(23.9465297708563,-3.12319285852936,-0.794882308526463));
#70508=CARTESIAN_POINT('Ctrl Pts',(23.9469800995703,-3.12137306036934,-0.801998586382847));
#70509=CARTESIAN_POINT('Ctrl Pts',(23.9478463390075,-3.11783201295848,-0.815651142850113));
#70510=CARTESIAN_POINT('Ctrl Pts',(23.9482621265365,-3.11611449615686,-0.822188356516703));
#70511=CARTESIAN_POINT('Ctrl Pts',(23.9492419984857,-3.11202505866147,-0.837556691490353));
#70512=CARTESIAN_POINT('Ctrl Pts',(23.9498066343287,-3.1096361014503,-0.846383182128466));
#70513=CARTESIAN_POINT('Ctrl Pts',(23.9514770064054,-3.102473398428,-0.872407547982178));
#70514=CARTESIAN_POINT('Ctrl Pts',(23.9525861626283,-3.09759437263171,-0.889575853826422));
#70515=CARTESIAN_POINT('Ctrl Pts',(23.9677321791505,-3.02931351866074,-1.12246760876618));
#70516=CARTESIAN_POINT('Ctrl Pts',(23.9825305107754,-2.94366080241747,-1.33097640330434));
#70517=CARTESIAN_POINT('Ctrl Pts',(24.0047132199061,-2.78754706084985,-1.62067303497832));
#70518=CARTESIAN_POINT('Ctrl Pts',(24.0117966993987,-2.73363077361013,-1.71004743944285));
#70519=CARTESIAN_POINT('Ctrl Pts',(24.0279815501492,-2.59986478255717,-1.90924472583986));
#70520=CARTESIAN_POINT('Ctrl Pts',(24.0370367020506,-2.5172130875698,-2.01696762923823));
#70521=CARTESIAN_POINT('Ctrl Pts',(24.0473045077119,-2.41161252548228,-2.13795800786652));
#70522=CARTESIAN_POINT('Ctrl Pts',(24.0488855059699,-2.39499668946518,-2.15655520791147));
#70523=CARTESIAN_POINT('Ctrl Pts',(24.0509120926539,-2.3732105572202,-2.1803768322985));
#70524=CARTESIAN_POINT('Ctrl Pts',(24.0513717239377,-2.36823648829482,-2.18577844662803));
#70525=CARTESIAN_POINT('Ctrl Pts',(24.0521081845331,-2.36021273018471,-2.1944323428019));
#70526=CARTESIAN_POINT('Ctrl Pts',(24.0523858910943,-2.35717471399041,-2.1976953399327));
#70527=CARTESIAN_POINT('Ctrl Pts',(24.0529154030411,-2.35135810384829,-2.20391676395785));
#70528=CARTESIAN_POINT('Ctrl Pts',(24.0531672933293,-2.34858070069279,-2.20687623745996));
#70529=CARTESIAN_POINT('Ctrl Pts',(24.0537474529866,-2.34215980453836,-2.21369220075607));
#70530=CARTESIAN_POINT('Ctrl Pts',(24.0540754165548,-2.33851235117037,-2.21754497002045));
#70531=CARTESIAN_POINT('Ctrl Pts',(24.0551236786137,-2.32679793023771,-2.22985775347512));
#70532=CARTESIAN_POINT('Ctrl Pts',(24.0558411955534,-2.31869432849218,-2.23828300928951));
#70533=CARTESIAN_POINT('Ctrl Pts',(24.0683826639981,-2.17559215281365,-2.38545409714793));
#70534=CARTESIAN_POINT('Ctrl Pts',(24.0792892444952,-2.02838551313346,-2.51182575214239));
#70535=CARTESIAN_POINT('Ctrl Pts',(24.0982675329639,-1.75226450068466,-2.70866067242313));
#70536=CARTESIAN_POINT('Ctrl Pts',(24.1063464504612,-1.62824791669422,-2.78497408957766));
#70537=CARTESIAN_POINT('Ctrl Pts',(24.1202262384422,-1.41248151978341,-2.89839252605533));
#70538=CARTESIAN_POINT('Ctrl Pts',(24.1259073469837,-1.32341629099745,-2.94012758488685));
#70539=CARTESIAN_POINT('Ctrl Pts',(24.1338588851236,-1.1991927212137,-2.99154821290174));
#70540=CARTESIAN_POINT('Ctrl Pts',(24.1360136075413,-1.16556834657176,-3.0048085078227));
#70541=CARTESIAN_POINT('Ctrl Pts',(24.1397328746014,-1.10765792045297,-3.02652811261941));
#70542=CARTESIAN_POINT('Ctrl Pts',(24.1412880863984,-1.08348020644468,-3.03526754483951));
#70543=CARTESIAN_POINT('Ctrl Pts',(24.1433459998904,-1.05155077689729,-3.04637885700123));
#70544=CARTESIAN_POINT('Ctrl Pts',(24.1438400218268,-1.04389055217857,-3.04901224824852));
#70545=CARTESIAN_POINT('Ctrl Pts',(24.1448176028796,-1.0287422708796,-3.05415606597899));
#70546=CARTESIAN_POINT('Ctrl Pts',(24.1453011113823,-1.02125475065553,-3.05666790275898));
#70547=CARTESIAN_POINT('Ctrl Pts',(24.1462302294854,-1.00687623019897,-3.06143273337718));
#70548=CARTESIAN_POINT('Ctrl Pts',(24.1466756929059,-0.9999867041967,-3.06369004861693));
#70549=CARTESIAN_POINT('Ctrl Pts',(24.1476932640905,-0.984258999632539,
-3.06878444118112));
#70550=CARTESIAN_POINT('Ctrl Pts',(24.1482658593667,-0.975416093114644,
-3.07160661009801));
#70551=CARTESIAN_POINT('Ctrl Pts',(24.1497793507929,-0.952062268652112,
-3.07894884599618));
#70552=CARTESIAN_POINT('Ctrl Pts',(24.1507223538793,-0.937531486267142,
-3.0834044916557));
#70553=CARTESIAN_POINT('Ctrl Pts',(24.157043774263,-0.840267451275416,-3.11247795038588));
#70554=CARTESIAN_POINT('Ctrl Pts',(24.1625268956404,-0.75661231091669,-3.13386405203334));
#70555=CARTESIAN_POINT('Ctrl Pts',(24.1720642044643,-0.612431507189188,
-3.16461382936763));
#70556=CARTESIAN_POINT('Ctrl Pts',(24.1760661171515,-0.552309744809216,
-3.17565840092317));
#70557=CARTESIAN_POINT('Ctrl Pts',(24.1921324067065,-0.312215380081605,
-3.21274036577006));
#70558=CARTESIAN_POINT('Ctrl Pts',(24.2045038562107,-0.130500535951932,
-3.22523488105438));
#70559=CARTESIAN_POINT('Ctrl Pts',(24.2265038557349,0.195408718925657,-3.22004830389745));
#70560=CARTESIAN_POINT('Ctrl Pts',(24.2361378471194,0.339237330303576,-3.20808712063632));
#70561=CARTESIAN_POINT('Ctrl Pts',(24.2466684543615,0.502539931309318,-3.18339619838852));
#70562=CARTESIAN_POINT('Ctrl Pts',(24.2479964620516,0.523254053050859,-3.18005707325042));
#70563=CARTESIAN_POINT('Ctrl Pts',(24.249771897695,0.551131169313726,-3.17528349980527));
#70564=CARTESIAN_POINT('Ctrl Pts',(24.2502288999336,0.558323493429724,-3.17402674044763));
#70565=CARTESIAN_POINT('Ctrl Pts',(24.2509621566829,0.569891514551294,-3.17196485124729));
#70566=CARTESIAN_POINT('Ctrl Pts',(24.2512392750444,0.574269872363887,-3.17117509295435));
#70567=CARTESIAN_POINT('Ctrl Pts',(24.2517683757404,0.582642154189509,-3.16964701170753));
#70568=CARTESIAN_POINT('Ctrl Pts',(24.2520204402399,0.586636306743029,-3.16891020737707));
#70569=CARTESIAN_POINT('Ctrl Pts',(24.2526019506715,0.595863437666562,-3.16719002853917));
#70570=CARTESIAN_POINT('Ctrl Pts',(24.2529310861547,0.601095413377917,-3.16620122831886));
#70571=CARTESIAN_POINT('Ctrl Pts',(24.2539868789534,0.617907629362031,-3.16298068367275));
#70572=CARTESIAN_POINT('Ctrl Pts',(24.2547106981569,0.629478242129024,-3.16069830835176));
#70573=CARTESIAN_POINT('Ctrl Pts',(24.2627052050788,0.757730710628542,-3.13466749441315));
#70574=CARTESIAN_POINT('Ctrl Pts',(24.2696314484577,0.873037727802388,-3.10453027186463));
#70575=CARTESIAN_POINT('Ctrl Pts',(24.2906645546229,1.2245995746501,-2.99149875270655));
#70576=CARTESIAN_POINT('Ctrl Pts',(24.3042753896284,1.45304638361967,-2.88745079745108));
#70577=CARTESIAN_POINT('Ctrl Pts',(24.3231511483848,1.73388731700391,-2.71768855264025));
#70578=CARTESIAN_POINT('Ctrl Pts',(24.3276981246716,1.79912095903847,-2.67495023443257));
#70579=CARTESIAN_POINT('Ctrl Pts',(24.3341532234949,1.88778939303036,-2.6121468591654));
#70580=CARTESIAN_POINT('Ctrl Pts',(24.335989619172,1.91258570430405,-2.59404622825271));
#70581=CARTESIAN_POINT('Ctrl Pts',(24.339201215045,1.95517875548305,-2.56201175696724));
#70582=CARTESIAN_POINT('Ctrl Pts',(24.3405701495425,1.97309474593036,-2.54823964576696));
#70583=CARTESIAN_POINT('Ctrl Pts',(24.342556502518,1.99873908623755,-2.52809412699337));
#70584=CARTESIAN_POINT('Ctrl Pts',(24.3431679316176,2.00658514545121,-2.52187111095803));
#70585=CARTESIAN_POINT('Ctrl Pts',(24.3442301406221,2.02013258745581,-2.51102285702446));
#70586=CARTESIAN_POINT('Ctrl Pts',(24.3446802399656,2.02584743657954,-2.50641449518807));
#70587=CARTESIAN_POINT('Ctrl Pts',(24.3455465589255,2.03679730607112,-2.49752278242673));
#70588=CARTESIAN_POINT('Ctrl Pts',(24.3459626571503,2.04203469078258,-2.49324239400952));
#70589=CARTESIAN_POINT('Ctrl Pts',(24.3469440586128,2.05433571617093,-2.48312430247615));
#70590=CARTESIAN_POINT('Ctrl Pts',(24.3475099175341,2.06138798238261,-2.47727291988379));
#70591=CARTESIAN_POINT('Ctrl Pts',(24.3491862910293,2.08216090180188,-2.45988715988291));
#70592=CARTESIAN_POINT('Ctrl Pts',(24.3503002602566,2.09581021539986,-2.44826844534009));
#70593=CARTESIAN_POINT('Ctrl Pts',(24.3632602826306,2.25280591310585,-2.31235392627357));
#70594=CARTESIAN_POINT('Ctrl Pts',(24.3756375758673,2.38497788563792,-2.17576951099838));
#70595=CARTESIAN_POINT('Ctrl Pts',(24.3971781736522,2.58740556101427,-1.92584047345257));
#70596=CARTESIAN_POINT('Ctrl Pts',(24.4061444276756,2.66407811116201,-1.8183000411561));
#70597=CARTESIAN_POINT('Ctrl Pts',(24.4206274598583,2.7776519434225,-1.63633214160681));
#70598=CARTESIAN_POINT('Ctrl Pts',(24.4261723155484,2.81865862069949,-1.56463990762252));
#70599=CARTESIAN_POINT('Ctrl Pts',(24.4352270262218,2.88209127682018,-1.44313474562486));
#70600=CARTESIAN_POINT('Ctrl Pts',(24.4387864063127,2.90608599981429,-1.39418538986573));
#70601=CARTESIAN_POINT('Ctrl Pts',(24.4435636557174,2.9371414275009,-1.32654239064565));
#70602=CARTESIAN_POINT('Ctrl Pts',(24.4448341301516,2.94528609370989,-1.30835941158712));
#70603=CARTESIAN_POINT('Ctrl Pts',(24.4469910027674,2.95892567642942,-1.27713608778465));
#70604=CARTESIAN_POINT('Ctrl Pts',(24.4478819609886,2.9645041931189,-1.26413316215955));
#70605=CARTESIAN_POINT('Ctrl Pts',(24.4491308157636,2.97224735064338,-1.2457515207129));
#70606=CARTESIAN_POINT('Ctrl Pts',(24.4494929116256,2.97448329079731,-1.24040328876596));
#70607=CARTESIAN_POINT('Ctrl Pts',(24.450111242884,2.97828604404049,-1.23123792461093));
#70608=CARTESIAN_POINT('Ctrl Pts',(24.4503679098844,2.97985997330581,-1.22742377658365));
#70609=CARTESIAN_POINT('Ctrl Pts',(24.4508594644979,2.98286555916548,-1.22010039846514));
#70610=CARTESIAN_POINT('Ctrl Pts',(24.4510944225759,2.98429835030322,-1.21659166655155));
#70611=CARTESIAN_POINT('Ctrl Pts',(24.4516510884338,2.98768367818449,-1.20825944224309));
#70612=CARTESIAN_POINT('Ctrl Pts',(24.4519724641509,2.98963073598998,-1.20343371399519));
#70613=CARTESIAN_POINT('Ctrl Pts',(24.4529331064894,2.99542830684835,-1.18896369107299));
#70614=CARTESIAN_POINT('Ctrl Pts',(24.4535703128601,2.99924394767685,-1.17930536728709));
#70615=CARTESIAN_POINT('Ctrl Pts',(24.4668959167809,3.07838646082462,-0.976107545030948));
#70616=CARTESIAN_POINT('Ctrl Pts',(24.4785268946649,3.13489020979572,-0.775719669317487));
#70617=CARTESIAN_POINT('Ctrl Pts',(24.5041585737129,3.21615993811243,-0.324498349993523));
#70618=CARTESIAN_POINT('Ctrl Pts',(24.5181153637159,3.23165206859308,-0.0734265439457822));
#70619=CARTESIAN_POINT('Ctrl Pts',(24.5353381615681,3.21581706078861,0.214631633178711));
#70620=CARTESIAN_POINT('Ctrl Pts',(24.53761405516,3.21307881532083,0.252330041067377));
#70621=CARTESIAN_POINT('Ctrl Pts',(24.5406487632862,3.20858564698239,0.3020648574759));
#70622=CARTESIAN_POINT('Ctrl Pts',(24.5413888612738,3.20742466442282,0.314152905241428));
#70623=CARTESIAN_POINT('Ctrl Pts',(24.5426065644947,3.20540798805554,0.33397260215336));
#70624=CARTESIAN_POINT('Ctrl Pts',(24.5430828968478,3.20459256464288,0.341708299336075));
#70625=CARTESIAN_POINT('Ctrl Pts',(24.5440074619479,3.20295852301971,0.356689542889614));
#70626=CARTESIAN_POINT('Ctrl Pts',(24.5444555846405,3.20214330410689,0.363935418394814));
#70627=CARTESIAN_POINT('Ctrl Pts',(24.5454924893318,3.20020348224519,0.380665805270519));
#70628=CARTESIAN_POINT('Ctrl Pts',(24.5460818237653,3.19906129718454,0.390148172859003));
#70629=CARTESIAN_POINT('Ctrl Pts',(24.5476688146303,3.19587935418773,0.415610684270149));
#70630=CARTESIAN_POINT('Ctrl Pts',(24.5486689194122,3.19376191747903,0.431580683851429));
#70631=CARTESIAN_POINT('Ctrl Pts',(24.5562773525415,3.17680772848648,0.552487088823846));
#70632=CARTESIAN_POINT('Ctrl Pts',(24.5630451041883,3.15692413316605,0.656639280067787));
#70633=CARTESIAN_POINT('Ctrl Pts',(24.5903246141465,3.05835349330857,1.06305383976668));
#70634=CARTESIAN_POINT('Ctrl Pts',(24.6119993037899,2.94107086922114,1.35412853763791));
#70635=CARTESIAN_POINT('Ctrl Pts',(24.6356478877074,2.75988257730599,1.66475738814796));
#70636=CARTESIAN_POINT('Ctrl Pts',(24.6387342229977,2.73507177555099,1.70521314851884));
#70637=CARTESIAN_POINT('Ctrl Pts',(24.643518035678,2.69462388859257,1.76801068495882));
#70638=CARTESIAN_POINT('Ctrl Pts',(24.6452469560196,2.67958210594207,1.79072598077847));
#70639=CARTESIAN_POINT('Ctrl Pts',(24.6474246732853,2.66006756088026,1.81939920994147));
#70640=CARTESIAN_POINT('Ctrl Pts',(24.6478904288879,2.65586027802726,1.82553529130181));
#70641=CARTESIAN_POINT('Ctrl Pts',(24.6486343520619,2.64908552716697,1.83534288417639));
#70642=CARTESIAN_POINT('Ctrl Pts',(24.648913428406,2.64653161775061,1.83902366204834));
#70643=CARTESIAN_POINT('Ctrl Pts',(24.6494439272661,2.6416529957989,1.84602368174154));
#70644=CARTESIAN_POINT('Ctrl Pts',(24.6496954388052,2.6393297260632,1.84934382445071));
#70645=CARTESIAN_POINT('Ctrl Pts',(24.6502725823676,2.63397495253043,1.85696559073099));
#70646=CARTESIAN_POINT('Ctrl Pts',(24.6505979168048,2.63093917340923,1.86126417320882));
#70647=CARTESIAN_POINT('Ctrl Pts',(24.6514648355828,2.62280393316453,1.87272378487449));
#70648=CARTESIAN_POINT('Ctrl Pts',(24.6520051478234,2.61768563390385,1.87987147765501));
#70649=CARTESIAN_POINT('Ctrl Pts',(24.6557905368795,2.58149524406424,1.92997686193812));
#70650=CARTESIAN_POINT('Ctrl Pts',(24.6589679542382,2.54939442962948,1.97218589222974));
#70651=CARTESIAN_POINT('Ctrl Pts',(24.66356306845,2.5006992428584,2.033037501982));
#70652=CARTESIAN_POINT('Ctrl Pts',(24.6650204354975,2.4849085069603,2.05230795959657));
#70653=CARTESIAN_POINT('Ctrl Pts',(24.6839448926844,2.27559942845645,2.30178357203485));
#70654=CARTESIAN_POINT('Ctrl Pts',(24.7000690263606,2.05099992471885,2.50399502260781));
#70655=CARTESIAN_POINT('Ctrl Pts',(24.7176902808396,1.79755176803132,2.67487365050067));
#70656=CARTESIAN_POINT('Ctrl Pts',(24.7179720150962,1.79349702741155,2.67759403485003));
#70657=CARTESIAN_POINT('Ctrl Pts',(24.7182540045911,1.78943620997144,2.68030513429778));
#70658=CARTESIAN_POINT('Origin',(-1.72497344927317,0.,0.));
#70659=CARTESIAN_POINT('',(26.2169191182387,1.78943621037807,2.6803051340263));
#70660=CARTESIAN_POINT('',(25.9683941809562,1.78943611353999,2.68030519867773));
#70661=CARTESIAN_POINT('',(-1.72497344927317,1.78943621037804,2.68030513402633));
#70662=CARTESIAN_POINT('',(25.3965734492343,-3.22274892221719,-0.00263568737792321));
#70663=CARTESIAN_POINT('Ctrl Pts',(25.3965734492731,-3.22274892221668,-0.00263568800522834));
#70664=CARTESIAN_POINT('Ctrl Pts',(25.4064511434359,-3.22261841837125,-0.16220735443242));
#70665=CARTESIAN_POINT('Ctrl Pts',(25.4163288375986,-3.21063356431501,-0.321308852596511));
#70666=CARTESIAN_POINT('Ctrl Pts',(25.4262065317614,-3.18701826592584,-0.47857301966895));
#70667=CARTESIAN_POINT('Ctrl Pts',(25.4272489382552,-3.1845261113816,-0.495169321022294));
#70668=CARTESIAN_POINT('Ctrl Pts',(25.428291344749,-3.18190446401791,-0.511745192054206));
#70669=CARTESIAN_POINT('Ctrl Pts',(25.4293337512428,-3.17915361093883,-0.528299044627735));
#70670=CARTESIAN_POINT('Ctrl Pts',(25.4355059993356,-3.16286538962451,-0.626316934559181));
#70671=CARTESIAN_POINT('Ctrl Pts',(25.4416782474284,-3.14201120273219,-0.723753356799299));
#70672=CARTESIAN_POINT('Ctrl Pts',(25.4478504955211,-3.11664432240526,-0.820149821751527));
#70673=CARTESIAN_POINT('Ctrl Pts',(25.4540143841738,-3.09131179794256,-0.916415731277972));
#70674=CARTESIAN_POINT('Ctrl Pts',(25.4601782728264,-3.06147883750468,-1.01164406664152));
#70675=CARTESIAN_POINT('Ctrl Pts',(25.4663421614791,-3.02725010945302,-1.10538424871928));
#70676=CARTESIAN_POINT('Ctrl Pts',(25.4724995231376,-2.99305762649246,-1.19902516852138));
#70677=CARTESIAN_POINT('Ctrl Pts',(25.4786568847961,-2.95447877809909,-1.29118066213792));
#70678=CARTESIAN_POINT('Ctrl Pts',(25.4848142464547,-2.91166839374426,-1.38141403184228));
#70679=CARTESIAN_POINT('Ctrl Pts',(25.490967110601,-2.86888927931282,-1.47158149252477));
#70680=CARTESIAN_POINT('Ctrl Pts',(25.4971199747473,-2.82188495965848,-1.55982922937228));
#70681=CARTESIAN_POINT('Ctrl Pts',(25.5032728388936,-2.7708585074938,-1.64574016598892));
#70682=CARTESIAN_POINT('Ctrl Pts',(25.5094233720301,-2.71985138667719,-1.73161855528651));
#70683=CARTESIAN_POINT('Ctrl Pts',(25.5155739051667,-2.6648253826722,-1.81516153037809));
#70684=CARTESIAN_POINT('Ctrl Pts',(25.5217244383032,-2.60602925073417,-1.89597708499283));
#70685=CARTESIAN_POINT('Ctrl Pts',(25.5278742865184,-2.54723966631388,-1.97678364001423));
#70686=CARTESIAN_POINT('Ctrl Pts',(25.5340241347336,-2.48468104421193,-2.05486302715625));
#70687=CARTESIAN_POINT('Ctrl Pts',(25.5401739829489,-2.41864457081421,-2.12985351669334));
#70688=CARTESIAN_POINT('Ctrl Pts',(25.546324791328,-2.35259778726936,-2.20485571435081));
#70689=CARTESIAN_POINT('Ctrl Pts',(25.5524755997072,-2.28307236100721,-2.27676773047784));
#70690=CARTESIAN_POINT('Ctrl Pts',(25.5586264080863,-2.21039805259985,-2.34526288751662));
#70691=CARTESIAN_POINT('Ctrl Pts',(25.5647837944525,-2.137646022594,-2.41383129675705));
#70692=CARTESIAN_POINT('Ctrl Pts',(25.5709411808187,-2.06173870246463,-2.47897525141644));
#70693=CARTESIAN_POINT('Ctrl Pts',(25.5770985671849,-1.98304073711152,-2.54040685667793));
#70694=CARTESIAN_POINT('Ctrl Pts',(25.5832593899218,-1.9042988512746,-2.60187274625429));
#70695=CARTESIAN_POINT('Ctrl Pts',(25.5894202126588,-1.8227635730985,-2.65962190935768));
#70696=CARTESIAN_POINT('Ctrl Pts',(25.5955810353958,-1.73882874207579,-2.71340969413598));
#70697=CARTESIAN_POINT('Ctrl Pts',(25.6017521583125,-1.65475358176889,-2.76728740584027));
#70698=CARTESIAN_POINT('Ctrl Pts',(25.6079232812291,-1.56827123162878,-2.81719029285439));
#70699=CARTESIAN_POINT('Ctrl Pts',(25.6140944041458,-1.47980045897549,-2.86291951757571));
#70700=CARTESIAN_POINT('Ctrl Pts',(25.6187899260914,-1.41248427355162,-2.89771425122965));
#70701=CARTESIAN_POINT('Ctrl Pts',(25.6234854480369,-1.34401741123988,-2.93009360253979));
#70702=CARTESIAN_POINT('Ctrl Pts',(25.6281809699825,-1.2745910437658,-2.9599890597183));
#70703=CARTESIAN_POINT('Ctrl Pts',(25.6343532180752,-1.18333031296776,-2.99928653946431));
#70704=CARTESIAN_POINT('Ctrl Pts',(25.640525466168,-1.09008985363507,-3.03442868273002));
#70705=CARTESIAN_POINT('Ctrl Pts',(25.6466977142608,-0.995284156096808,
-3.06521239249789));
#70706=CARTESIAN_POINT('Ctrl Pts',(25.6528616029134,-0.900606859514062,
-3.0959544100695));
#70707=CARTESIAN_POINT('Ctrl Pts',(25.659025491566,-0.804368947753559,-3.12234959380749));
#70708=CARTESIAN_POINT('Ctrl Pts',(25.6651893802186,-0.707006047244728,
-3.14424235892518));
#70709=CARTESIAN_POINT('Ctrl Pts',(25.6713467418772,-0.609746245138786,
-3.16611194160781));
#70710=CARTESIAN_POINT('Ctrl Pts',(25.6775041035357,-0.511364244079028,
-3.18348848943958));
#70711=CARTESIAN_POINT('Ctrl Pts',(25.6836614651943,-0.412311115966327,
-3.19626611941975));
#70712=CARTESIAN_POINT('Ctrl Pts',(25.6898143293406,-0.313330339078197,
-3.20903441625524));
#70713=CARTESIAN_POINT('Ctrl Pts',(25.6959671934869,-0.213679839265979,
-3.21721041845915));
#70714=CARTESIAN_POINT('Ctrl Pts',(25.7021200576332,-0.113820268406736,
-3.22073943512974));
#70715=CARTESIAN_POINT('Ctrl Pts',(25.7082705907697,-0.0139985293002585,
-3.22426711483397));
#70716=CARTESIAN_POINT('Ctrl Pts',(25.7144211239062,0.0860316898480511,
-3.22315129180131));
#70717=CARTESIAN_POINT('Ctrl Pts',(25.7205716570428,0.185806125355152,-3.2173892593655));
#70718=CARTESIAN_POINT('Ctrl Pts',(25.726721505258,0.2855694500142,-3.21162786858772));
#70719=CARTESIAN_POINT('Ctrl Pts',(25.7328713534732,0.385076614009189,-3.20122132211802));
#70720=CARTESIAN_POINT('Ctrl Pts',(25.7390212016884,0.483865879610104,-3.18621897757344));
#70721=CARTESIAN_POINT('Ctrl Pts',(25.7451720100675,0.582670568988227,-3.17121429074179));
#70722=CARTESIAN_POINT('Ctrl Pts',(25.7513228184466,0.680756707852433,-3.15161244585278));
#70723=CARTESIAN_POINT('Ctrl Pts',(25.7574736268258,0.777671187211214,-3.12751420253874));
#70724=CARTESIAN_POINT('Ctrl Pts',(25.7636310131919,0.874689311839299,-3.10339018733865));
#70725=CARTESIAN_POINT('Ctrl Pts',(25.7697883995581,0.970532852425206,-3.07476027630433));
#70726=CARTESIAN_POINT('Ctrl Pts',(25.7759457859243,1.06476246205168,-3.04177554430067));
#70727=CARTESIAN_POINT('Ctrl Pts',(25.7821066086613,1.15904466020469,-3.00877240387463));
#70728=CARTESIAN_POINT('Ctrl Pts',(25.7882674313982,1.25171073075715,-2.97140976485196));
#70729=CARTESIAN_POINT('Ctrl Pts',(25.7944282541352,1.34234191734396,-2.92988664276305));
#70730=CARTESIAN_POINT('Ctrl Pts',(25.8005993770519,1.43312462874343,-2.88829409883899));
#70731=CARTESIAN_POINT('Ctrl Pts',(25.8067704999686,1.52186527437194,-2.84252737696021));
#70732=CARTESIAN_POINT('Ctrl Pts',(25.8129416228852,1.60817015848789,-2.79283123440158));
#70733=CARTESIAN_POINT('Ctrl Pts',(25.8176371448309,1.67383834932636,-2.75501812791398));
#70734=CARTESIAN_POINT('Ctrl Pts',(25.8223326667765,1.73809688178141,-2.71493103980607));
#70735=CARTESIAN_POINT('Ctrl Pts',(25.8270281887221,1.80078475461697,-2.6726937404123));
#70736=CARTESIAN_POINT('Ctrl Pts',(25.8332004368149,1.88318775646201,-2.61717294982807));
#70737=CARTESIAN_POINT('Ctrl Pts',(25.8393726849076,1.96316571170811,-2.55773996097069));
#70738=CARTESIAN_POINT('Ctrl Pts',(25.8455449330004,2.04032365416872,-2.49463363016287));
#70739=CARTESIAN_POINT('Ctrl Pts',(25.851708821653,2.11737709707084,-2.43161276798599));
#70740=CARTESIAN_POINT('Ctrl Pts',(25.8578727103056,2.19161778520991,-2.36492872484808));
#70741=CARTESIAN_POINT('Ctrl Pts',(25.8640365989583,2.26267929160564,-2.29486382729761));
#70742=CARTESIAN_POINT('Ctrl Pts',(25.8701939606168,2.33366555036824,-2.22487312206267));
#70743=CARTESIAN_POINT('Ctrl Pts',(25.8763513222754,2.40147901262755,-2.1515089831154));
#70744=CARTESIAN_POINT('Ctrl Pts',(25.8825086839339,2.46578670946404,-2.07509360413705));
#70745=CARTESIAN_POINT('Ctrl Pts',(25.8886615480802,2.53004743412808,-1.99873404112688));
#70746=CARTESIAN_POINT('Ctrl Pts',(25.8948144122265,2.59080720565419,-1.91932800049423));
#70747=CARTESIAN_POINT('Ctrl Pts',(25.9009672763728,2.64777093838166,-1.83723341477383));
#70748=CARTESIAN_POINT('Ctrl Pts',(25.9071178095093,2.70471309042502,-1.7551699305497));
#70749=CARTESIAN_POINT('Ctrl Pts',(25.9132683426459,2.75786181386659,-1.67042028158036));
#70750=CARTESIAN_POINT('Ctrl Pts',(25.9194188757824,2.80696379970748,-1.58337354709233));
#70751=CARTESIAN_POINT('Ctrl Pts',(25.9255687239976,2.85606031756752,-1.49633650609977));
#70752=CARTESIAN_POINT('Ctrl Pts',(25.9317185722128,2.90111078035803,-1.40700326649594));
#70753=CARTESIAN_POINT('Ctrl Pts',(25.937868420428,2.941907041828,-1.31578893434426));
#70754=CARTESIAN_POINT('Ctrl Pts',(25.9440192288072,2.98270967273951,-1.22456036107502));
#70755=CARTESIAN_POINT('Ctrl Pts',(25.9501700371863,3.01925660569321,-1.13145050847048));
#70756=CARTESIAN_POINT('Ctrl Pts',(25.9563208455654,3.05138759991882,-1.03689501761829));
#70757=CARTESIAN_POINT('Ctrl Pts',(25.9624782319316,3.08355295666249,-0.942238404319069));
#70758=CARTESIAN_POINT('Ctrl Pts',(25.9686356182978,3.11129280404582,-0.846133477572178));
#70759=CARTESIAN_POINT('Ctrl Pts',(25.974793004664,3.13449666821515,-0.749031507647139));
#70760=CARTESIAN_POINT('Ctrl Pts',(25.980953827401,3.15771348221024,-0.651875346162331));
#70761=CARTESIAN_POINT('Ctrl Pts',(25.9871146501379,3.17638919038319,-0.553721460092493));
#70762=CARTESIAN_POINT('Ctrl Pts',(25.9932754728749,3.19046478051791,-0.45502972075985));
#70763=CARTESIAN_POINT('Ctrl Pts',(25.9994465957916,3.20456390340376,-0.356172980307013));
#70764=CARTESIAN_POINT('Ctrl Pts',(26.0056177187082,3.21404750471343,-0.256777023023595));
#70765=CARTESIAN_POINT('Ctrl Pts',(26.0117888416249,3.21890860112972,-0.157305372041514));
#70766=CARTESIAN_POINT('Ctrl Pts',(26.0164843635705,3.22260734205748,-0.0816187706800719));
#70767=CARTESIAN_POINT('Ctrl Pts',(26.0211798855161,3.22363097265403,-0.00588842137078513));
#70768=CARTESIAN_POINT('Ctrl Pts',(26.0258754074616,3.22199655461114,0.0696833163242371));
#70769=CARTESIAN_POINT('Ctrl Pts',(26.0320478199131,3.21984806028064,0.169024761244146));
#70770=CARTESIAN_POINT('Ctrl Pts',(26.0382202323645,3.21309709702631,0.268441605044972));
#70771=CARTESIAN_POINT('Ctrl Pts',(26.0443926448159,3.20173103033753,0.367472409676948));
#70772=CARTESIAN_POINT('Ctrl Pts',(26.050556655457,3.19038043499604,0.466368414820806));
#70773=CARTESIAN_POINT('Ctrl Pts',(26.0567206660981,3.17442727188708,0.564878997462854));
#70774=CARTESIAN_POINT('Ctrl Pts',(26.0628846767392,3.15391091004099,0.662543231815437));
#70775=CARTESIAN_POINT('Ctrl Pts',(26.0693027784683,3.13254882858017,0.764233353372993));
#70776=CARTESIAN_POINT('Ctrl Pts',(26.0757208801975,3.1062392263513,0.865005371543196));
#70777=CARTESIAN_POINT('Ctrl Pts',(26.0821389819266,3.0750863857692,0.964345001831263));
#70778=CARTESIAN_POINT('Ctrl Pts',(26.088291605933,3.04522214819242,1.05957555751343));
#70779=CARTESIAN_POINT('Ctrl Pts',(26.0944442299393,3.01090752128512,1.15348940611871));
#70780=CARTESIAN_POINT('Ctrl Pts',(26.1005968539457,2.97228614769764,1.24564546268379));
#70781=CARTESIAN_POINT('Ctrl Pts',(26.1067471567657,2.93367934470664,1.3377667517461));
#70782=CARTESIAN_POINT('Ctrl Pts',(26.1128974595858,2.89076919182726,1.42813116656454));
#70783=CARTESIAN_POINT('Ctrl Pts',(26.1190477624059,2.84374802133819,1.5163161786498));
#70784=CARTESIAN_POINT('Ctrl Pts',(26.1251973900478,2.79673201281737,1.60449150981415));
#70785=CARTESIAN_POINT('Ctrl Pts',(26.1313470176897,2.74560608890042,1.69048753100129));
#70786=CARTESIAN_POINT('Ctrl Pts',(26.1374966453317,2.69060876380754,1.77390587197349));
#70787=CARTESIAN_POINT('Ctrl Pts',(26.1436472427918,2.63560276544036,1.85733736831557));
#70788=CARTESIAN_POINT('Ctrl Pts',(26.1497978402519,2.57672439283207,1.93819001478082));
#70789=CARTESIAN_POINT('Ctrl Pts',(26.155948437712,2.51425517594452,2.01609485707796));
#70790=CARTESIAN_POINT('Ctrl Pts',(26.1621049069745,2.45172632145301,2.09407407293639));
#70791=CARTESIAN_POINT('Ctrl Pts',(26.168261376237,2.38560005268462,2.16909952858232));
#70792=CARTESIAN_POINT('Ctrl Pts',(26.1744178454995,2.31619765702528,2.24083599937403));
#70793=CARTESIAN_POINT('Ctrl Pts',(26.1805777890285,2.24675609566771,2.31261295304735));
#70794=CARTESIAN_POINT('Ctrl Pts',(26.1867377325574,2.17403504176792,2.38109692834211));
#70795=CARTESIAN_POINT('Ctrl Pts',(26.1928976760864,2.09839062061772,2.44599148931545));
#70796=CARTESIAN_POINT('Ctrl Pts',(26.1990661581254,2.02264134612869,2.51097600287598));
#70797=CARTESIAN_POINT('Ctrl Pts',(26.2052346401643,1.94396095872055,2.57236090548764));
#70798=CARTESIAN_POINT('Ctrl Pts',(26.2114031222033,1.86273620934477,2.62989189452644));
#70799=CARTESIAN_POINT('Ctrl Pts',(26.2132417875484,1.83852520720482,2.64704039802366));
#70800=CARTESIAN_POINT('Ctrl Pts',(26.2150804528936,1.81408831882809,2.66384679315958));
#70801=CARTESIAN_POINT('Ctrl Pts',(26.2169191182387,1.78943621037807,2.6803051340263));
#70802=CARTESIAN_POINT('Ctrl Pts',(24.9668672316986,1.78943621037801,2.68030513402634));
#70803=CARTESIAN_POINT('Ctrl Pts',(24.9730253659514,1.7063050378271,2.73580550541515));
#70804=CARTESIAN_POINT('Ctrl Pts',(24.9791835002043,1.62064010479516,2.7874008839277));
#70805=CARTESIAN_POINT('Ctrl Pts',(24.9853416344572,1.53284979617197,2.8348702024741));
#70806=CARTESIAN_POINT('Ctrl Pts',(24.9915035882499,1.44500503622206,2.8823689635343));
#70807=CARTESIAN_POINT('Ctrl Pts',(24.9976655420425,1.35503266701405,2.92573638099519));
#70808=CARTESIAN_POINT('Ctrl Pts',(25.0038274958352,1.26336234213593,2.96479900751684));
#70809=CARTESIAN_POINT('Ctrl Pts',(25.0099992767797,1.17154582041404,3.0039239315455));
#70810=CARTESIAN_POINT('Ctrl Pts',(25.0161710577242,1.07802634331453,3.03873020710462));
#70811=CARTESIAN_POINT('Ctrl Pts',(25.0223428386687,0.983249997689492,3.06909384094778));
#70812=CARTESIAN_POINT('Ctrl Pts',(25.0254416637003,0.935663196590666,3.08433929269846));
#70813=CARTESIAN_POINT('Ctrl Pts',(25.0285404887319,0.887759724998352,3.09846555476231));
#70814=CARTESIAN_POINT('Ctrl Pts',(25.0316393137636,0.839596895532805,3.11146181328193));
#70815=CARTESIAN_POINT('Ctrl Pts',(25.0378115618563,0.743666041329783,3.1373477962083));
#70816=CARTESIAN_POINT('Ctrl Pts',(25.0439838099491,0.646368063480807,3.15883865464586));
#70817=CARTESIAN_POINT('Ctrl Pts',(25.0501560580419,0.548142172272313,3.17579245566781));
#70818=CARTESIAN_POINT('Ctrl Pts',(25.0563199466945,0.450049314189568,3.19272329515574));
#70819=CARTESIAN_POINT('Ctrl Pts',(25.0624838353471,0.35103146490954,3.20512921747368));
#70820=CARTESIAN_POINT('Ctrl Pts',(25.0686477239998,0.251541981600455,3.21291832980431));
#70821=CARTESIAN_POINT('Ctrl Pts',(25.0748050856583,0.152157848550892,3.22069919417768));
#70822=CARTESIAN_POINT('Ctrl Pts',(25.0809624473169,0.0523035050232203,
3.22387293420183));
#70823=CARTESIAN_POINT('Ctrl Pts',(25.0871198089754,-0.0475594895811064,
3.22239905310481));
#70824=CARTESIAN_POINT('Ctrl Pts',(25.0932726731217,-0.147349541411322,
3.2209262485725));
#70825=CARTESIAN_POINT('Ctrl Pts',(25.099425537268,-0.247147798736351,3.21481257866312));
#70826=CARTESIAN_POINT('Ctrl Pts',(25.1055784014143,-0.346490517966515,
3.20406958155707));
#70827=CARTESIAN_POINT('Ctrl Pts',(25.1117289345509,-0.445795601252857,
3.19333065443057));
#70828=CARTESIAN_POINT('Ctrl Pts',(25.1178794676874,-0.544645057982626,
3.1779659315848));
#70829=CARTESIAN_POINT('Ctrl Pts',(25.1240300008239,-0.642578980517186,
3.15803891937663));
#70830=CARTESIAN_POINT('Ctrl Pts',(25.1301798490392,-0.740501997162669,
3.13811412623391));
#70831=CARTESIAN_POINT('Ctrl Pts',(25.1363296972544,-0.837509256657889,
3.11362814042592));
#70832=CARTESIAN_POINT('Ctrl Pts',(25.1424795454696,-0.933150773795894,
3.08469564071792));
#70833=CARTESIAN_POINT('Ctrl Pts',(25.1486303538487,-1.02880722325928,3.05575862383461));
#70834=CARTESIAN_POINT('Ctrl Pts',(25.1547811622278,-1.12309709102729,3.02237383992554));
#70835=CARTESIAN_POINT('Ctrl Pts',(25.160931970607,-1.21558626036452,2.98470561464829));
#70836=CARTESIAN_POINT('Ctrl Pts',(25.1670893569732,-1.30817434231957,2.94699710505669));
#70837=CARTESIAN_POINT('Ctrl Pts',(25.1732467433394,-1.39895747722821,2.90499617061417));
#70838=CARTESIAN_POINT('Ctrl Pts',(25.1794041297055,-1.48752234279973,2.8589149763803));
#70839=CARTESIAN_POINT('Ctrl Pts',(25.1855649524425,-1.57613663546532,2.81280806473009));
#70840=CARTESIAN_POINT('Ctrl Pts',(25.1917257751795,-1.66252981774675,2.76261657659059));
#70841=CARTESIAN_POINT('Ctrl Pts',(25.1978865979164,-1.74631578201306,2.70859719264274));
#70842=CARTESIAN_POINT('Ctrl Pts',(25.2040577208331,-1.83024182667576,2.65448749456194));
#70843=CARTESIAN_POINT('Ctrl Pts',(25.2102288437498,-1.91155159252995,2.59653736949879));
#70844=CARTESIAN_POINT('Ctrl Pts',(25.2163999666665,-1.98989029754131,2.53504520004101));
#70845=CARTESIAN_POINT('Ctrl Pts',(25.221095488612,-2.0494971330447,2.48825666008384));
#70846=CARTESIAN_POINT('Ctrl Pts',(25.2257910105576,-2.10738452960363,2.43941832528737));
#70847=CARTESIAN_POINT('Ctrl Pts',(25.2304865325031,-2.16341077510467,2.38867565413579));
#70848=CARTESIAN_POINT('Ctrl Pts',(25.2365666600861,-2.23595792206555,2.32297009081808));
#70849=CARTESIAN_POINT('Ctrl Pts',(25.2426467876691,-2.30565498701423,2.25382395116584));
#70850=CARTESIAN_POINT('Ctrl Pts',(25.248726915252,-2.37215020834902,2.18151803832325));
#70851=CARTESIAN_POINT('Ctrl Pts',(25.2548871875013,-2.43952193058788,2.1082590314582));
#70852=CARTESIAN_POINT('Ctrl Pts',(25.2610474597506,-2.50360638839096,2.03175658788883));
#70853=CARTESIAN_POINT('Ctrl Pts',(25.2672077319998,-2.56407194549882,1.95234541534174));
#70854=CARTESIAN_POINT('Ctrl Pts',(25.2732724589536,-2.62359968699002,1.87416590328558));
#70855=CARTESIAN_POINT('Ctrl Pts',(25.2793371859074,-2.67961968610552,1.79316760569218));
#70856=CARTESIAN_POINT('Ctrl Pts',(25.2854019128613,-2.73185329001641,1.70970616315392));
#70857=CARTESIAN_POINT('Ctrl Pts',(25.2914628587965,-2.78405432919192,1.62629675416471));
#70858=CARTESIAN_POINT('Ctrl Pts',(25.2975238047317,-2.83247342331725,1.54042762849967));
#70859=CARTESIAN_POINT('Ctrl Pts',(25.3035847506669,-2.87687433357412,1.45248464064942));
#70860=CARTESIAN_POINT('Ctrl Pts',(25.3096436515148,-2.92126026205435,1.36457132656472));
#70861=CARTESIAN_POINT('Ctrl Pts',(25.3157025523626,-2.96163049860683,1.27458594064752));
#70862=CARTESIAN_POINT('Ctrl Pts',(25.3217614532105,-2.99779459353714,1.18293919432044));
#70863=CARTESIAN_POINT('Ctrl Pts',(25.3279957862125,-3.03500580002009,1.08863886667117));
#70864=CARTESIAN_POINT('Ctrl Pts',(25.3342301192145,-3.0677633322663,0.992579940178667));
#70865=CARTESIAN_POINT('Ctrl Pts',(25.3404644522165,-3.09591328035451,0.8952309886418));
#70866=CARTESIAN_POINT('Ctrl Pts',(25.3465270595895,-3.12328783393962,0.800563528440829));
#70867=CARTESIAN_POINT('Ctrl Pts',(25.3525896669625,-3.14630527403118,0.704676649018005));
#70868=CARTESIAN_POINT('Ctrl Pts',(25.3586522743356,-3.16487541490557,0.608014120416877));
#70869=CARTESIAN_POINT('Ctrl Pts',(25.364972470152,-3.18423456509354,0.507244588220224));
#70870=CARTESIAN_POINT('Ctrl Pts',(25.3712926659685,-3.19876001937384,0.405632565462735));
#70871=CARTESIAN_POINT('Ctrl Pts',(25.3776128617849,-3.20840947697045,0.303687653002588));
#70872=CARTESIAN_POINT('Ctrl Pts',(25.3839330576014,-3.21805893456705,0.201742740542441));
#70873=CARTESIAN_POINT('Ctrl Pts',(25.3902532534178,-3.22283242446457,0.0994654874476783));
#70874=CARTESIAN_POINT('Ctrl Pts',(25.3965734492343,-3.22274892221719,-0.00263568737796789));
#70875=CARTESIAN_POINT('Ctrl Pts',(24.7182540045911,1.78943620997144,2.68030513429778));
#70876=CARTESIAN_POINT('Ctrl Pts',(24.7222453478997,1.73195847831639,2.71867865116884));
#70877=CARTESIAN_POINT('Ctrl Pts',(24.726288389885,1.67326334016704,2.75519200731721));
#70878=CARTESIAN_POINT('Ctrl Pts',(24.7330617147449,1.57466108917989,2.81221744338375));
#70879=CARTESIAN_POINT('Ctrl Pts',(24.7357526037413,1.53541891685696,2.83383361232678));
#70880=CARTESIAN_POINT('Ctrl Pts',(24.7392573642564,1.48429630346652,2.86062038174631));
#70881=CARTESIAN_POINT('Ctrl Pts',(24.7400443197473,1.47281643318138,2.86654778984984));
#70882=CARTESIAN_POINT('Ctrl Pts',(24.7413195042604,1.45421492987351,2.87601107694878));
#70883=CARTESIAN_POINT('Ctrl Pts',(24.7418062160466,1.44711523299443,2.87958994956608));
#70884=CARTESIAN_POINT('Ctrl Pts',(24.7427376194432,1.43352948044272,2.88637543331099));
#70885=CARTESIAN_POINT('Ctrl Pts',(24.7431821494981,1.42704571908599,2.88958654959459));
#70886=CARTESIAN_POINT('Ctrl Pts',(24.7442017171333,1.41217573494316,2.89688873130772));
#70887=CARTESIAN_POINT('Ctrl Pts',(24.7447772584621,1.40378247750127,2.90096524985512));
#70888=CARTESIAN_POINT('Ctrl Pts',(24.7465553994281,1.37785486583098,2.91341915367981));
#70889=CARTESIAN_POINT('Ctrl Pts',(24.7477622288225,1.36026260047563,2.92167431919034));
#70890=CARTESIAN_POINT('Ctrl Pts',(24.7586252128972,1.20197652185344,2.99421053964749));
#70891=CARTESIAN_POINT('Ctrl Pts',(24.7686273519858,1.05692070616148,3.04843407564396));
#70892=CARTESIAN_POINT('Ctrl Pts',(24.788281423995,0.772754196078471,3.13193255696457));
#70893=CARTESIAN_POINT('Ctrl Pts',(24.7978676326064,0.634482763091523,3.16284333564088));
#70894=CARTESIAN_POINT('Ctrl Pts',(24.8154557588334,0.377637103319876,3.2027374071815));
#70895=CARTESIAN_POINT('Ctrl Pts',(24.8234452104858,0.259718266130523,3.21444960419365));
#70896=CARTESIAN_POINT('Ctrl Pts',(24.8343875948278,0.0935378356830638,
3.22174875478681));
#70897=CARTESIAN_POINT('Ctrl Pts',(24.8375057453881,0.0456153291802165,
3.22278359779733));
#70898=CARTESIAN_POINT('Ctrl Pts',(24.8423333836376,-0.0297538041632178,
3.22272945871833));
#70899=CARTESIAN_POINT('Ctrl Pts',(24.844074983371,-0.0571923855762873,
3.22235932262176));
#70900=CARTESIAN_POINT('Ctrl Pts',(24.846266308942,-0.0920799727126928,
3.22144291763584));
#70901=CARTESIAN_POINT('Ctrl Pts',(24.8467332486345,-0.0995353699431762,
3.22122118236531));
#70902=CARTESIAN_POINT('Ctrl Pts',(24.847478614483,-0.111471720943126,3.22082469652651));
#70903=CARTESIAN_POINT('Ctrl Pts',(24.847757955557,-0.115953141308101,3.22066647449443));
#70904=CARTESIAN_POINT('Ctrl Pts',(24.8482886494012,-0.124482584165218,
3.22034750619765));
#70905=CARTESIAN_POINT('Ctrl Pts',(24.8485400924167,-0.128530585015484,
3.22018848257395));
#70906=CARTESIAN_POINT('Ctrl Pts',(24.849116672788,-0.137828274936922,3.21980566768868));
#70907=CARTESIAN_POINT('Ctrl Pts',(24.8494415145162,-0.1430777186857,3.21957667068159));
#70908=CARTESIAN_POINT('Ctrl Pts',(24.8504698776396,-0.159730563815079,
3.21880941272033));
#70909=CARTESIAN_POINT('Ctrl Pts',(24.8511707641062,-0.171131831573002,
3.21822339090448));
#70910=CARTESIAN_POINT('Ctrl Pts',(24.857843494033,-0.28013752918202,3.21203960568476));
#70911=CARTESIAN_POINT('Ctrl Pts',(24.8635837676913,-0.3774534862739,3.20206315653621));
#70912=CARTESIAN_POINT('Ctrl Pts',(24.8779271558124,-0.624308795738743,
3.16534279914013));
#70913=CARTESIAN_POINT('Ctrl Pts',(24.886348299795,-0.772685107795609,3.13243021670104));
#70914=CARTESIAN_POINT('Ctrl Pts',(24.9075991693126,-1.13687318358235,3.02418280067591));
#70915=CARTESIAN_POINT('Ctrl Pts',(24.920496757803,-1.34799813346745,2.93616128672216));
#70916=CARTESIAN_POINT('Ctrl Pts',(24.9356406438767,-1.56849676741873,2.81540031751905));
#70917=CARTESIAN_POINT('Ctrl Pts',(24.9370526181426,-1.58882149121871,2.80398061376712));
#70918=CARTESIAN_POINT('Ctrl Pts',(24.9390845250058,-1.6177263288978,2.78732489188102));
#70919=CARTESIAN_POINT('Ctrl Pts',(24.9396979981633,-1.62640894071049,2.78226750728392));
#70920=CARTESIAN_POINT('Ctrl Pts',(24.9407626159442,-1.64139925088342,2.77344191329835));
#70921=CARTESIAN_POINT('Ctrl Pts',(24.9412130713828,-1.64771801062409,2.76969256476));
#70922=CARTESIAN_POINT('Ctrl Pts',(24.9420792696397,-1.6598225302669,2.76245405021316));
#70923=CARTESIAN_POINT('Ctrl Pts',(24.9424948882769,-1.66561025368352,2.75896822983439));
#70924=CARTESIAN_POINT('Ctrl Pts',(24.9434739272598,-1.67919604927818,2.75072746922713));
#70925=CARTESIAN_POINT('Ctrl Pts',(24.9440378967102,-1.68698492373811,2.74595754632112));
#70926=CARTESIAN_POINT('Ctrl Pts',(24.9457050024538,-1.70989883212784,2.73179073397694));
#70927=CARTESIAN_POINT('Ctrl Pts',(24.9468115399456,-1.72496619371148,2.7223016439022));
#70928=CARTESIAN_POINT('Ctrl Pts',(24.9621143667602,-1.93137195359057,2.58991027985836));
#70929=CARTESIAN_POINT('Ctrl Pts',(24.9770908606751,-2.10921811592356,2.44724207780335));
#70930=CARTESIAN_POINT('Ctrl Pts',(25.0031998477566,-2.38399683153424,2.17445030253602));
#70931=CARTESIAN_POINT('Ctrl Pts',(25.0140993626502,-2.48891221880105,2.05353172791189));
#70932=CARTESIAN_POINT('Ctrl Pts',(25.0291588087393,-2.62420386046175,1.87192568433355));
#70933=CARTESIAN_POINT('Ctrl Pts',(25.0335349463593,-2.66232351270553,1.81730195120155));
#70934=CARTESIAN_POINT('Ctrl Pts',(25.040052546099,-2.7176450009886,1.73254763200282));
#70935=CARTESIAN_POINT('Ctrl Pts',(25.0422574210526,-2.73609718565112,1.70325807623763));
#70936=CARTESIAN_POINT('Ctrl Pts',(25.0449396243877,-2.75826198244533,1.66678535087545));
#70937=CARTESIAN_POINT('Ctrl Pts',(25.0454447242568,-2.76242338031803,1.65987940552182));
#70938=CARTESIAN_POINT('Ctrl Pts',(25.0462365309591,-2.76892779018727,1.64899296153188));
#70939=CARTESIAN_POINT('Ctrl Pts',(25.0465243595754,-2.77128820231631,1.6450229769809));
#70940=CARTESIAN_POINT('Ctrl Pts',(25.0470619332851,-2.77568938356153,1.637584258875));
#70941=CARTESIAN_POINT('Ctrl Pts',(25.0473118066221,-2.77773216749669,1.63411681492495));
#70942=CARTESIAN_POINT('Ctrl Pts',(25.0478782409987,-2.78235611130064,1.62623435775113));
#70943=CARTESIAN_POINT('Ctrl Pts',(25.04819453858,-2.78493325409513,1.62181703268784));
#70944=CARTESIAN_POINT('Ctrl Pts',(25.0491314597365,-2.79255217783527,1.60868618458253));
#70945=CARTESIAN_POINT('Ctrl Pts',(25.0497501498006,-2.7975637150224,1.59995505345611));
#70946=CARTESIAN_POINT('Ctrl Pts',(25.0541255827295,-2.83285774181815,1.53779272684827));
#70947=CARTESIAN_POINT('Ctrl Pts',(25.0577916787118,-2.86165063451717,1.48352494475262));
#70948=CARTESIAN_POINT('Ctrl Pts',(25.0621731504623,-2.89477254502612,1.41654028961094));
#70949=CARTESIAN_POINT('Ctrl Pts',(25.0629499656765,-2.9005943415028,1.40458070422258));
#70950=CARTESIAN_POINT('Ctrl Pts',(25.0813416713987,-3.03716455158955,1.11955705259713));
#70951=CARTESIAN_POINT('Ctrl Pts',(25.0975625961353,-3.12887064671542,0.829444519254396));
#70952=CARTESIAN_POINT('Ctrl Pts',(25.1192993635644,-3.19098294448296,0.457460293207525));
#70953=CARTESIAN_POINT('Ctrl Pts',(25.1236415852499,-3.20068368918857,0.383751007075289));
#70954=CARTESIAN_POINT('Ctrl Pts',(25.1298248044528,-3.21067933504703,0.280242928708544));
#70955=CARTESIAN_POINT('Ctrl Pts',(25.1316008331804,-3.21312324285893,0.250672757106428));
#70956=CARTESIAN_POINT('Ctrl Pts',(25.1347248287541,-3.2166779631481,0.198975130198541));
#70957=CARTESIAN_POINT('Ctrl Pts',(25.1360671343093,-3.21796955658273,0.176861856212914));
#70958=CARTESIAN_POINT('Ctrl Pts',(25.138016176275,-3.21950560520608,0.144907138208664));
#70959=CARTESIAN_POINT('Ctrl Pts',(25.1386171641455,-3.2199331069566,0.135074808901856));
#70960=CARTESIAN_POINT('Ctrl Pts',(25.1396671257129,-3.22059970874648,0.117934477711819));
#70961=CARTESIAN_POINT('Ctrl Pts',(25.1401154625857,-3.22085898864512,0.110627297157542));
#70962=CARTESIAN_POINT('Ctrl Pts',(25.1409826345581,-3.22131159178143,0.0965169001719425));
#70963=CARTESIAN_POINT('Ctrl Pts',(25.141401362908,-3.22150823561545,0.0897138233030848));
#70964=CARTESIAN_POINT('Ctrl Pts',(25.1423955790047,-3.2219232940922,0.0735856904937968));
#70965=CARTESIAN_POINT('Ctrl Pts',(25.1429716583337,-3.22212277615162,0.0642602468846168));
#70966=CARTESIAN_POINT('Ctrl Pts',(25.1446985126069,-3.22259832038217,0.0363661664544118));
#70967=CARTESIAN_POINT('Ctrl Pts',(25.14585304091,-3.2227543666048,0.0177961188830445));
#70968=CARTESIAN_POINT('Ctrl Pts',(25.1588113358357,-3.22270453128891,-0.189724329190089));
#70969=CARTESIAN_POINT('Ctrl Pts',(25.1711411472812,-3.20604255472005,-0.378270519167828));
#70970=CARTESIAN_POINT('Ctrl Pts',(25.1948083481093,-3.14417735314071,-0.726163397843209));
#70971=CARTESIAN_POINT('Ctrl Pts',(25.2060257990343,-3.10303275788517,-0.885635309103736));
#70972=CARTESIAN_POINT('Ctrl Pts',(25.2222300880156,-3.02503908865167,-1.11408070860695));
#70973=CARTESIAN_POINT('Ctrl Pts',(25.2273481028799,-2.99757872940744,-1.18598504394425));
#70974=CARTESIAN_POINT('Ctrl Pts',(25.2358734473504,-2.94660105045497,-1.3063500994954));
#70975=CARTESIAN_POINT('Ctrl Pts',(25.2393302040369,-2.92439567788134,-1.35532987529683));
#70976=CARTESIAN_POINT('Ctrl Pts',(25.2432736179026,-2.897127965109,-1.41168164410416));
#70977=CARTESIAN_POINT('Ctrl Pts',(25.2438278675962,-2.89324969933732,-1.41961321918727));
#70978=CARTESIAN_POINT('Ctrl Pts',(25.2447100024149,-2.88700291640514,-1.43225679716575));
#70979=CARTESIAN_POINT('Ctrl Pts',(25.2450391598449,-2.88465537686563,-1.43697902908275));
#70980=CARTESIAN_POINT('Ctrl Pts',(25.2456200589769,-2.88048274037477,-1.44532113343865));
#70981=CARTESIAN_POINT('Ctrl Pts',(25.2458720965956,-2.87866239267388,-1.44894334813071));
#70982=CARTESIAN_POINT('Ctrl Pts',(25.246401389914,-2.87481853156797,-1.45655620978659));
#70983=CARTESIAN_POINT('Ctrl Pts',(25.2466785504567,-2.87279354638554,-1.46054606984546));
#70984=CARTESIAN_POINT('Ctrl Pts',(25.247413610099,-2.86739090291708,-1.47113627678832));
#70985=CARTESIAN_POINT('Ctrl Pts',(25.2478706016622,-2.86399874080965,-1.47772925470652));
#70986=CARTESIAN_POINT('Ctrl Pts',(25.2499838971357,-2.84815921112237,-1.50825541547001));
#70987=CARTESIAN_POINT('Ctrl Pts',(25.2516232792896,-2.83543396556172,-1.53204426475609));
#70988=CARTESIAN_POINT('Ctrl Pts',(25.2560638194022,-2.79981448791345,-1.59666768377218));
#70989=CARTESIAN_POINT('Ctrl Pts',(25.2588325397859,-2.7763261925034,-1.63716895839225));
#70990=CARTESIAN_POINT('Ctrl Pts',(25.2682361255484,-2.69249802684546,-1.77471926813515));
#70991=CARTESIAN_POINT('Ctrl Pts',(25.2746888741484,-2.62788189543982,-1.86906780491483));
#70992=CARTESIAN_POINT('Ctrl Pts',(25.2969891978706,-2.38595905922603,-2.1848833116506));
#70993=CARTESIAN_POINT('Ctrl Pts',(25.3126208656007,-2.18460500275352,-2.38621041631845));
#70994=CARTESIAN_POINT('Ctrl Pts',(25.3306660999574,-1.94532532248448,-2.56946423624707));
#70995=CARTESIAN_POINT('Ctrl Pts',(25.3317407405264,-1.93104424527404,-2.58021417233837));
#70996=CARTESIAN_POINT('Ctrl Pts',(25.3340123029492,-1.90079862210402,-2.60258950920599));
#70997=CARTESIAN_POINT('Ctrl Pts',(25.335210183852,-1.88481521413602,-2.6141880454436));
#70998=CARTESIAN_POINT('Ctrl Pts',(25.3369885531623,-1.86104268936345,-2.63110748899963));
#70999=CARTESIAN_POINT('Ctrl Pts',(25.3375646470591,-1.85333498710995,-2.63654242007956));
#71000=CARTESIAN_POINT('Ctrl Pts',(25.3385872694928,-1.83964190586644,-2.64610810575319));
#71001=CARTESIAN_POINT('Ctrl Pts',(25.3390332683808,-1.83366616785781,-2.65025259789132));
#71002=CARTESIAN_POINT('Ctrl Pts',(25.3399610100135,-1.82122836919245,-2.65881666920786));
#71003=CARTESIAN_POINT('Ctrl Pts',(25.3404428726232,-1.81476413581595,-2.66323299447073));
#71004=CARTESIAN_POINT('Ctrl Pts',(25.3416885092651,-1.79804367037382,-2.67456717410993));
#71005=CARTESIAN_POINT('Ctrl Pts',(25.3424536185682,-1.78776365298968,-2.68144955641355));
#71006=CARTESIAN_POINT('Ctrl Pts',(25.3456858069415,-1.74429772470826,-2.71018855878836));
#71007=CARTESIAN_POINT('Ctrl Pts',(25.3481735967792,-1.71074983346264,-2.73148885335003));
#71008=CARTESIAN_POINT('Ctrl Pts',(25.368834892233,-1.43150596834491,-2.90162454436661));
#71009=CARTESIAN_POINT('Ctrl Pts',(25.3882605961333,-1.16735440949385,-3.01759018957438));
#71010=CARTESIAN_POINT('Ctrl Pts',(25.4130141012399,-0.815356616330881,
-3.11890616710155));
#71011=CARTESIAN_POINT('Ctrl Pts',(25.4183412625889,-0.738512094248152,
-3.13799027241118));
#71012=CARTESIAN_POINT('Ctrl Pts',(25.429573830687,-0.57284046609421,-3.17271054874872));
#71013=CARTESIAN_POINT('Ctrl Pts',(25.4354525674215,-0.483894699489564,
-3.18748924563328));
#71014=CARTESIAN_POINT('Ctrl Pts',(25.4418484224756,-0.38329620050824,-3.199894937584));
#71015=CARTESIAN_POINT('Ctrl Pts',(25.4425537732969,-0.372147153933057,
-3.20121072306947));
#71016=CARTESIAN_POINT('Ctrl Pts',(25.443582308523,-0.355805555300184,-3.20305279422941));
#71017=CARTESIAN_POINT('Ctrl Pts',(25.443908002188,-0.350618387654371,-3.20362475064689));
#71018=CARTESIAN_POINT('Ctrl Pts',(25.4444849497941,-0.341406985708713,
-3.20461779371705));
#71019=CARTESIAN_POINT('Ctrl Pts',(25.4447364860416,-0.337383325332505,
-3.205043903942));
#71020=CARTESIAN_POINT('Ctrl Pts',(25.445267062303,-0.328879618075118,-3.20592826486408));
#71021=CARTESIAN_POINT('Ctrl Pts',(25.4455459985672,-0.324399423301787,
-3.20638470202705));
#71022=CARTESIAN_POINT('Ctrl Pts',(25.4462908201649,-0.312411147834194,
-3.20758067002698));
#71023=CARTESIAN_POINT('Ctrl Pts',(25.4467557547441,-0.304901346314265,
-3.20830323562666));
#71024=CARTESIAN_POINT('Ctrl Pts',(25.4489614789434,-0.269152135997372,
-3.21161623760856));
#71025=CARTESIAN_POINT('Ctrl Pts',(25.4506834914283,-0.240880835208396,
-3.2138603396312));
#71026=CARTESIAN_POINT('Ctrl Pts',(25.4671451210339,0.0323950907180704,
-3.23192580310718));
#71027=CARTESIAN_POINT('Ctrl Pts',(25.4805872982264,0.278457756224323,-3.22007624882055));
#71028=CARTESIAN_POINT('Ctrl Pts',(25.500139552909,0.622799386095099,-3.16368743775459));
#71029=CARTESIAN_POINT('Ctrl Pts',(25.5059679258127,0.723917063142524,-3.14209160832866));
#71030=CARTESIAN_POINT('Ctrl Pts',(25.5127692398958,0.838192825270334,-3.11187586838479));
#71031=CARTESIAN_POINT('Ctrl Pts',(25.5136270518064,0.852540647959471,-3.1079757186906));
#71032=CARTESIAN_POINT('Ctrl Pts',(25.5159540479529,0.891275380439016,-3.09715810358835));
#71033=CARTESIAN_POINT('Ctrl Pts',(25.5174278753743,0.91560819202678,-3.09005205729914));
#71034=CARTESIAN_POINT('Ctrl Pts',(25.5234412026339,1.01400470287881,-3.06005251711778));
#71035=CARTESIAN_POINT('Ctrl Pts',(25.5280456936087,1.08731022428053,-3.03477873125652));
#71036=CARTESIAN_POINT('Ctrl Pts',(25.5336283849449,1.17333854641769,-3.00160125886792));
#71037=CARTESIAN_POINT('Ctrl Pts',(25.5345211155486,1.18701137817151,-2.99622052571694));
#71038=CARTESIAN_POINT('Ctrl Pts',(25.5359797584074,1.20921225452993,-2.98730789808527));
#71039=CARTESIAN_POINT('Ctrl Pts',(25.5365437613093,1.21776286347696,-2.98383249530038));
#71040=CARTESIAN_POINT('Ctrl Pts',(25.5375513488446,1.23297789515737,-2.97757203817173));
#71041=CARTESIAN_POINT('Ctrl Pts',(25.5379944481783,1.23964813290859,-2.97480120977447));
#71042=CARTESIAN_POINT('Ctrl Pts',(25.538930188915,1.2536903119907,-2.96891263425015));
#71043=CARTESIAN_POINT('Ctrl Pts',(25.5394230011528,1.26106005622917,-2.96578980390144));
#71044=CARTESIAN_POINT('Ctrl Pts',(25.5407285237656,1.28051519819183,-2.95746032190452));
#71045=CARTESIAN_POINT('Ctrl Pts',(25.5415428221267,1.2925803759799,-2.95220708823341));
#71046=CARTESIAN_POINT('Ctrl Pts',(25.5452892666182,1.3477676398697,-2.9277751425098));
#71047=CARTESIAN_POINT('Ctrl Pts',(25.5482512272447,1.3904955335118,-2.90772534571724));
#71048=CARTESIAN_POINT('Ctrl Pts',(25.5562855378268,1.50392941754613,-2.85142519024847));
#71049=CARTESIAN_POINT('Ctrl Pts',(25.5614144515166,1.57375712934127,-2.81348824446929));
#71050=CARTESIAN_POINT('Ctrl Pts',(25.5885625509803,1.93024461063403,-2.60238543815831));
#71051=CARTESIAN_POINT('Ctrl Pts',(25.6119709556168,2.18997949478353,-2.38792771561801));
#71052=CARTESIAN_POINT('Ctrl Pts',(25.6360031766948,2.43687159193019,-2.10930755518569));
#71053=CARTESIAN_POINT('Ctrl Pts',(25.6383945613085,2.46123192761313,-2.08083137479053));
#71054=CARTESIAN_POINT('Ctrl Pts',(25.6412462957966,2.49009690997284,-2.04587310177126));
#71055=CARTESIAN_POINT('Ctrl Pts',(25.6417393133049,2.49508037368628,-2.03979246530145));
#71056=CARTESIAN_POINT('Ctrl Pts',(25.6425456579893,2.50322064080885,-2.02978554654503));
#71057=CARTESIAN_POINT('Ctrl Pts',(25.6428599136691,2.50639054221406,-2.02587003340791));
#71058=CARTESIAN_POINT('Ctrl Pts',(25.6434236290191,2.51207232690855,-2.01881805354956));
#71059=CARTESIAN_POINT('Ctrl Pts',(25.6436733270412,2.51458752485737,-2.0156843228451));
#71060=CARTESIAN_POINT('Ctrl Pts',(25.6442124730355,2.52001498841045,-2.00889617849284));
#71061=CARTESIAN_POINT('Ctrl Pts',(25.6445017700227,2.52292515810312,-2.00524014647778));
#71062=CARTESIAN_POINT('Ctrl Pts',(25.6453038768717,2.53098760521193,-1.9950659978529));
#71063=CARTESIAN_POINT('Ctrl Pts',(25.6458154654982,2.53612268862311,-1.98853421025533));
#71064=CARTESIAN_POINT('Ctrl Pts',(25.6486619244838,2.5646491520489,-1.95195852169992));
#71065=CARTESIAN_POINT('Ctrl Pts',(25.6509622826641,2.58753308149023,-1.92152028296286));
#71066=CARTESIAN_POINT('Ctrl Pts',(25.6683877347154,2.75895266873513,-1.68489487662805));
#71067=CARTESIAN_POINT('Ctrl Pts',(25.6822241054221,2.88318962624129,-1.4621707869376));
#71068=CARTESIAN_POINT('Ctrl Pts',(25.7075109593749,3.05449218316946,-1.04618029976341));
#71069=CARTESIAN_POINT('Ctrl Pts',(25.7187183295096,3.11236148238462,-0.858839695299414));
#71070=CARTESIAN_POINT('Ctrl Pts',(25.7316159962583,3.15659880698721,-0.649864350481781));
#71071=CARTESIAN_POINT('Ctrl Pts',(25.7327042893211,3.16016903462346,-0.632274746273916));
#71072=CARTESIAN_POINT('Ctrl Pts',(25.7343556834629,3.16534098225953,-0.605655110023139));
#71073=CARTESIAN_POINT('Ctrl Pts',(25.7349153148007,3.16705143007519,-0.596646363263539));
#71074=CARTESIAN_POINT('Ctrl Pts',(25.7358899889036,3.16995701321921,-0.58097837276057));
#71075=CARTESIAN_POINT('Ctrl Pts',(25.7363044702751,3.17116967506644,-0.574322406062973));
#71076=CARTESIAN_POINT('Ctrl Pts',(25.7371700437387,3.17365429695081,-0.560437191614757));
#71077=CARTESIAN_POINT('Ctrl Pts',(25.7376212517982,3.17492253391829,-0.553207325056425));
#71078=CARTESIAN_POINT('Ctrl Pts',(25.7386895103552,3.17786148398446,-0.536110162028866));
#71079=CARTESIAN_POINT('Ctrl Pts',(25.7393072331797,3.17951094924722,-0.526239334540342));
#71080=CARTESIAN_POINT('Ctrl Pts',(25.7413545925632,3.18481274392778,-0.493576889058274));
#71081=CARTESIAN_POINT('Ctrl Pts',(25.7427905248514,3.18826612273365,-0.470754123963716));
#71082=CARTESIAN_POINT('Ctrl Pts',(25.7589760372603,3.22422897353678,-0.214501952103334));
#71083=CARTESIAN_POINT('Ctrl Pts',(25.7745627122902,3.23127677550765,0.0217340357278075));
#71084=CARTESIAN_POINT('Ctrl Pts',(25.7988741158303,3.20261910010179,0.3805437024416));
#71085=CARTESIAN_POINT('Ctrl Pts',(25.8073275007937,3.18555130897384,0.50383153661494));
#71086=CARTESIAN_POINT('Ctrl Pts',(25.8185247861165,3.15307712849567,0.667877081081072));
#71087=CARTESIAN_POINT('Ctrl Pts',(25.8213784835601,3.1439142465915,0.70975955228662));
#71088=CARTESIAN_POINT('Ctrl Pts',(25.8257350381447,3.12851590505007,0.773978422217284));
#71089=CARTESIAN_POINT('Ctrl Pts',(25.8272558795155,3.12287065136274,0.796450445278329));
#71090=CARTESIAN_POINT('Ctrl Pts',(25.8323186807997,3.10315441822898,0.871500100214371));
#71091=CARTESIAN_POINT('Ctrl Pts',(25.8358188808968,3.08799313335904,0.92378516090376));
#71092=CARTESIAN_POINT('Ctrl Pts',(25.8398061516744,3.0688308258754,0.984110489091247));
#71093=CARTESIAN_POINT('Ctrl Pts',(25.840362486052,3.06611314154838,0.992545364274838));
#71094=CARTESIAN_POINT('Ctrl Pts',(25.841247301742,3.06171974272827,1.00599090016046));
#71095=CARTESIAN_POINT('Ctrl Pts',(25.8415770673611,3.06006646285892,1.01100876259951));
#71096=CARTESIAN_POINT('Ctrl Pts',(25.8421586636162,3.05712234576144,1.01987105599639));
#71097=CARTESIAN_POINT('Ctrl Pts',(25.8424107925584,3.0558365830291,1.0237171417742));
#71098=CARTESIAN_POINT('Ctrl Pts',(25.8429398761243,3.05311850048225,1.03179695670407));
#71099=CARTESIAN_POINT('Ctrl Pts',(25.8432167370596,3.05168463605442,1.03603012528558));
#71100=CARTESIAN_POINT('Ctrl Pts',(25.8439501500001,3.0478557880578,1.04725703887878));
#71101=CARTESIAN_POINT('Ctrl Pts',(25.8444058016789,3.0454455219901,1.05424560013657));
#71102=CARTESIAN_POINT('Ctrl Pts',(25.8465039069506,3.03420264698613,1.08648397181839));
#71103=CARTESIAN_POINT('Ctrl Pts',(25.8481297338543,3.02507961861375,1.11163237375532));
#71104=CARTESIAN_POINT('Ctrl Pts',(25.8627208722192,2.93957878251326,1.33847145927029));
#71105=CARTESIAN_POINT('Ctrl Pts',(25.8746715512404,2.84343683712916,1.53216282296315));
#71106=CARTESIAN_POINT('Ctrl Pts',(25.9005871819413,2.596705524906,1.92476656642778));
#71107=CARTESIAN_POINT('Ctrl Pts',(25.9145434327586,2.44099546647484,2.1187552258836));
#71108=CARTESIAN_POINT('Ctrl Pts',(25.9306928394981,2.25076808839353,2.30662926390878));
#71109=CARTESIAN_POINT('Ctrl Pts',(25.9318725394989,2.23681221168371,2.32016522102951));
#71110=CARTESIAN_POINT('Ctrl Pts',(25.9336266998634,2.21597722546849,2.34001059767379));
#71111=CARTESIAN_POINT('Ctrl Pts',(25.934196912783,2.20919163218262,2.34641790617689));
#71112=CARTESIAN_POINT('Ctrl Pts',(25.9352114778584,2.19709593793012,2.35774030719268));
#71113=CARTESIAN_POINT('Ctrl Pts',(25.9356553195539,2.19179691339331,2.36266718047914));
#71114=CARTESIAN_POINT('Ctrl Pts',(25.936588429857,2.18064105876955,2.37296972915166));
#71115=CARTESIAN_POINT('Ctrl Pts',(25.9370778539771,2.17478084660683,2.37834165545747));
#71116=CARTESIAN_POINT('Ctrl Pts',(25.9383648694412,2.15934774873143,2.39238409969114));
#71117=CARTESIAN_POINT('Ctrl Pts',(25.9391639688925,2.14974258393941,2.40101878280846));
#71118=CARTESIAN_POINT('Ctrl Pts',(25.9427433305337,2.10662002080281,2.43931815410813));
#71119=CARTESIAN_POINT('Ctrl Pts',(25.9455502546513,2.07254002768217,2.46833921436925));
#71120=CARTESIAN_POINT('Ctrl Pts',(25.9530689124994,1.98061180210791,2.54337509983254));
#71121=CARTESIAN_POINT('Ctrl Pts',(25.957828700725,1.92176880674521,2.5881235048462));
#71122=CARTESIAN_POINT('Ctrl Pts',(25.9645599125487,1.83765515169878,2.64763862344991));
#71123=CARTESIAN_POINT('Ctrl Pts',(25.9664728856645,1.81365036753495,2.66413918124719));
#71124=CARTESIAN_POINT('Ctrl Pts',(25.9683941809562,1.78943611353999,2.68030519867773));
#71125=CARTESIAN_POINT('Origin',(-1.72497344927317,0.,0.));
#71126=CARTESIAN_POINT('',(27.4670789411482,1.78943621037803,2.68030513402633));
#71127=CARTESIAN_POINT('',(27.2231721927303,1.78943620958681,2.68030513455457));
#71128=CARTESIAN_POINT('',(-1.72497344927317,1.78943621037804,2.68030513402633));
#71129=CARTESIAN_POINT('',(26.6465734493259,-3.22274928133509,0.00215224399016846));
#71130=CARTESIAN_POINT('Ctrl Pts',(26.6465734493259,-3.22274928133509,0.00215224399017275));
#71131=CARTESIAN_POINT('Ctrl Pts',(26.6526554760797,-3.222814805559,-0.0959630935353457));
#71132=CARTESIAN_POINT('Ctrl Pts',(26.6587375028335,-3.218395510171,-0.194255137665291));
#71133=CARTESIAN_POINT('Ctrl Pts',(26.6648195295873,-3.20946944460621,-0.292272897544588));
#71134=CARTESIAN_POINT('Ctrl Pts',(26.6708944080508,-3.20055386996977,-0.390175455794581));
#71135=CARTESIAN_POINT('Ctrl Pts',(26.6769692865144,-3.1871420880131,-0.487803927892748));
#71136=CARTESIAN_POINT('Ctrl Pts',(26.683044164978,-3.16926418034635,-0.584706864739565));
#71137=CARTESIAN_POINT('Ctrl Pts',(26.6891138244146,-3.1514016318813,-0.681526550694873));
#71138=CARTESIAN_POINT('Ctrl Pts',(26.6951834838511,-3.12908066328959,-0.777621501811903));
#71139=CARTESIAN_POINT('Ctrl Pts',(26.7012531432877,-3.10238310089514,-0.872546077740451));
#71140=CARTESIAN_POINT('Ctrl Pts',(26.7073200794118,-3.07569751706474,-0.967428063259591));
#71141=CARTESIAN_POINT('Ctrl Pts',(26.7133870155359,-3.04463935925051,-1.06114028614752));
#71142=CARTESIAN_POINT('Ctrl Pts',(26.71945395166,-3.00934118336634,-1.15324897771264));
#71143=CARTESIAN_POINT('Ctrl Pts',(26.7255198934566,-2.97404879260072,-1.24534257332207));
#71144=CARTESIAN_POINT('Ctrl Pts',(26.7315858352533,-2.93451792458771,-1.33583274197713));
#71145=CARTESIAN_POINT('Ctrl Pts',(26.7376517770499,-2.89093007270836,-1.42430364642179));
#71146=CARTESIAN_POINT('Ctrl Pts',(26.7437184522027,-2.84733695117416,-1.51278524676247));
#71147=CARTESIAN_POINT('Ctrl Pts',(26.7497851273556,-2.79968607092538,-1.59924669734376));
#71148=CARTESIAN_POINT('Ctrl Pts',(26.7558518025084,-2.74820532985199,-1.68329588233119));
#71149=CARTESIAN_POINT('Ctrl Pts',(26.7619246713544,-2.69667203018429,-1.76743087624295));
#71150=CARTESIAN_POINT('Ctrl Pts',(26.7679975402005,-2.64130129923939,-1.84914830658508));
#71151=CARTESIAN_POINT('Ctrl Pts',(26.7740704090465,-2.58236471881335,-1.92808454729767));
#71152=CARTESIAN_POINT('Ctrl Pts',(26.7801466663091,-2.52339525414657,-2.0070648312568));
#71153=CARTESIAN_POINT('Ctrl Pts',(26.7862229235716,-2.46085626542934,-2.08326049281699));
#71154=CARTESIAN_POINT('Ctrl Pts',(26.7922991808342,-2.39505859088021,-2.15634225222966));
#71155=CARTESIAN_POINT('Ctrl Pts',(26.7983851600855,-2.32915564029945,-2.22954094218233));
#71156=CARTESIAN_POINT('Ctrl Pts',(26.8044711393368,-2.25998391095859,-2.2996154677175));
#71157=CARTESIAN_POINT('Ctrl Pts',(26.8105571185881,-2.18788977991652,-2.36627468258375));
#71158=CARTESIAN_POINT('Ctrl Pts',(26.8141261731988,-2.1456109813574,-2.40536623520674));
#71159=CARTESIAN_POINT('Ctrl Pts',(26.8176952278095,-2.10232775368222,-2.44328399756727));
#71160=CARTESIAN_POINT('Ctrl Pts',(26.8212642824202,-2.05811463398499,-2.47997615227986));
#71161=CARTESIAN_POINT('Ctrl Pts',(26.827436530513,-1.9816533932666,-2.54343079409588));
#71162=CARTESIAN_POINT('Ctrl Pts',(26.8336087786058,-1.90212022575668,-2.60345769436343));
#71163=CARTESIAN_POINT('Ctrl Pts',(26.8397810266985,-1.81985545862044,-2.65974503895193));
#71164=CARTESIAN_POINT('Ctrl Pts',(26.8459449153511,-1.73770210751716,-2.71595615026513));
#71165=CARTESIAN_POINT('Ctrl Pts',(26.8521088040038,-1.65282486541836,-2.76843752942246));
#71166=CARTESIAN_POINT('Ctrl Pts',(26.8582726926564,-1.56559774479115,-2.81691697854318));
#71167=CARTESIAN_POINT('Ctrl Pts',(26.8644300543149,-1.4784629897034,-2.86534509236316));
#71168=CARTESIAN_POINT('Ctrl Pts',(26.8705874159735,-1.38898368065712,-2.90977949119602));
#71169=CARTESIAN_POINT('Ctrl Pts',(26.876744777632,-1.29756267400655,-2.94999129990666));
#71170=CARTESIAN_POINT('Ctrl Pts',(26.8828976417783,-1.20620844386154,-2.99017373676758));
#71171=CARTESIAN_POINT('Ctrl Pts',(26.8890505059246,-1.11291573229104,-3.02613954125879));
#71172=CARTESIAN_POINT('Ctrl Pts',(26.8952033700709,-1.01811103303148,-3.05770624601507));
#71173=CARTESIAN_POINT('Ctrl Pts',(26.9013539032075,-0.923342250488869,
-3.08926099173969));
#71174=CARTESIAN_POINT('Ctrl Pts',(26.907504436344,-0.827063030111666,-3.11641981217568));
#71175=CARTESIAN_POINT('Ctrl Pts',(26.9136549694805,-0.729718000981313,
-3.13904909192957));
#71176=CARTESIAN_POINT('Ctrl Pts',(26.9198048176957,-0.632383812161213,
-3.16167585169435));
#71177=CARTESIAN_POINT('Ctrl Pts',(26.925954665911,-0.53398447365143,-3.17977397525972));
#71178=CARTESIAN_POINT('Ctrl Pts',(26.9321045141262,-0.434976884188812,
-3.19326050812041));
#71179=CARTESIAN_POINT('Ctrl Pts',(26.9382553225053,-0.335953836862382,
-3.20674914660743));
#71180=CARTESIAN_POINT('Ctrl Pts',(26.9444061308844,-0.236322780399072,
-3.2156247056528));
#71181=CARTESIAN_POINT('Ctrl Pts',(26.9505569392636,-0.136546841566313,
-3.21985597854287));
#71182=CARTESIAN_POINT('Ctrl Pts',(26.9567143256297,-0.0366641972741644,
-3.22409177657119));
#71183=CARTESIAN_POINT('Ctrl Pts',(26.9628717119959,0.0633632039644185,
-3.22367335174628));
#71184=CARTESIAN_POINT('Ctrl Pts',(26.9690290983621,0.163071238732657,-3.21862165120385));
#71185=CARTESIAN_POINT('Ctrl Pts',(26.9751899210991,0.262834919477191,-3.21356713136196));
#71186=CARTESIAN_POINT('Ctrl Pts',(26.981350743836,0.362278446458359,-3.20387422839628));
#71187=CARTESIAN_POINT('Ctrl Pts',(26.987511566573,0.460943920654126,-3.18961569229147));
#71188=CARTESIAN_POINT('Ctrl Pts',(26.9936826894897,0.559774352057922,-3.17533331757113));
#71189=CARTESIAN_POINT('Ctrl Pts',(26.9998538124063,0.65782370558901,-3.15647014471428));
#71190=CARTESIAN_POINT('Ctrl Pts',(27.006024935323,0.754645215550309,-3.13314987850039));
#71191=CARTESIAN_POINT('Ctrl Pts',(27.0107204572687,0.828315361319435,-3.11540581096789));
#71192=CARTESIAN_POINT('Ctrl Pts',(27.0154159792143,0.90127488150179,-3.09508237520985));
#71193=CARTESIAN_POINT('Ctrl Pts',(27.0201115011599,0.973334390090736,-3.07225287493831));
#71194=CARTESIAN_POINT('Ctrl Pts',(27.0262837492527,1.06805637618828,-3.04224357221505));
#71195=CARTESIAN_POINT('Ctrl Pts',(27.0324559973454,1.16155593781016,-3.00779672233859));
#71196=CARTESIAN_POINT('Ctrl Pts',(27.0386282454382,1.25338675574727,-2.96903001046088));
#71197=CARTESIAN_POINT('Ctrl Pts',(27.0447921340908,1.34509320178397,-2.93031580263069));
#71198=CARTESIAN_POINT('Ctrl Pts',(27.0509560227435,1.43513499963557,-2.88729352904775));
#71199=CARTESIAN_POINT('Ctrl Pts',(27.0571199113961,1.52308094164781,-2.84013063215219));
#71200=CARTESIAN_POINT('Ctrl Pts',(27.0632772730547,1.61093375695453,-2.79301767644904));
#71201=CARTESIAN_POINT('Ctrl Pts',(27.0694346347132,1.69669474794529,-2.74177301847029));
#71202=CARTESIAN_POINT('Ctrl Pts',(27.0755919963717,1.77995355426057,-2.6866117894432));
#71203=CARTESIAN_POINT('Ctrl Pts',(27.0817448605181,1.86315154597361,-2.63149085174804));
#71204=CARTESIAN_POINT('Ctrl Pts',(27.0878977246644,1.94385062570489,-2.57245926990061));
#71205=CARTESIAN_POINT('Ctrl Pts',(27.0940505888107,2.02166669074999,-2.50977715226113));
#71206=CARTESIAN_POINT('Ctrl Pts',(27.1002011219472,2.09945327521434,-2.44711878171333));
#71207=CARTESIAN_POINT('Ctrl Pts',(27.1063516550837,2.17435867734285,-2.3808128955805));
#71208=CARTESIAN_POINT('Ctrl Pts',(27.1125021882203,2.24603008317851,-2.31116127259807));
#71209=CARTESIAN_POINT('Ctrl Pts',(27.1186520364355,2.31769350771015,-2.24151740599732));
#71210=CARTESIAN_POINT('Ctrl Pts',(27.1248018846507,2.38612334044547,-2.16852884602008));
#71211=CARTESIAN_POINT('Ctrl Pts',(27.1309517328659,2.45100274948986,-2.09253508560624));
#71212=CARTESIAN_POINT('Ctrl Pts',(27.137102541245,2.51589228803133,-2.01652946043309));
#71213=CARTESIAN_POINT('Ctrl Pts',(27.1432533496242,2.57723001979068,-1.93751803326576));
#71214=CARTESIAN_POINT('Ctrl Pts',(27.1494041580033,2.63473927601702,-1.85587351667976));
#71215=CARTESIAN_POINT('Ctrl Pts',(27.1555615443695,2.69231003556436,-1.77414168529888));
#71216=CARTESIAN_POINT('Ctrl Pts',(27.1617189307357,2.74604389292233,-1.68977149713199));
#71217=CARTESIAN_POINT('Ctrl Pts',(27.1678763171019,2.7957075127245,-1.60316470326532));
#71218=CARTESIAN_POINT('Ctrl Pts',(27.1740371398389,2.84539884925609,-1.51650957508309));
#71219=CARTESIAN_POINT('Ctrl Pts',(27.1801979625758,2.89101522613878,-1.42761574185211));
#71220=CARTESIAN_POINT('Ctrl Pts',(27.1863587853128,2.93237025061843,-1.33690772897309));
#71221=CARTESIAN_POINT('Ctrl Pts',(27.1925299082295,2.97379441589353,-1.24604806283689));
#71222=CARTESIAN_POINT('Ctrl Pts',(27.1987010311462,3.01094283613897,-1.15336856191371));
#71223=CARTESIAN_POINT('Ctrl Pts',(27.2048721540629,3.04367800213099,-1.05931193793137));
#71224=CARTESIAN_POINT('Ctrl Pts',(27.2095676760084,3.06858573649026,-0.987745555605622));
#71225=CARTESIAN_POINT('Ctrl Pts',(27.214263197954,3.09093944077442,-0.915382267047877));
#71226=CARTESIAN_POINT('Ctrl Pts',(27.2189587198996,3.11069837576653,-0.842421021522788));
#71227=CARTESIAN_POINT('Ctrl Pts',(27.2251309679923,3.13667143056936,-0.746513705199134));
#71228=CARTESIAN_POINT('Ctrl Pts',(27.2313032160851,3.1582506037194,-0.649235276058583));
#71229=CARTESIAN_POINT('Ctrl Pts',(27.2374754641779,3.17529356364918,-0.551024815365045));
#71230=CARTESIAN_POINT('Ctrl Pts',(27.2436393528305,3.19231344129171,-0.452947366899128));
#71231=CARTESIAN_POINT('Ctrl Pts',(27.2498032414831,3.20480924330201,-0.353940820061735));
#71232=CARTESIAN_POINT('Ctrl Pts',(27.2559671301357,3.21268866535944,-0.254458448417352));
#71233=CARTESIAN_POINT('Ctrl Pts',(27.2621244917943,3.2205597438299,-0.155081419501796));
#71234=CARTESIAN_POINT('Ctrl Pts',(27.2682818534528,3.22382412668934,-0.0552299981218721));
#71235=CARTESIAN_POINT('Ctrl Pts',(27.2744392151113,3.22244089819566,0.044634293272634));
#71236=CARTESIAN_POINT('Ctrl Pts',(27.2805920792576,3.22105868005145,0.144425640946092));
#71237=CARTESIAN_POINT('Ctrl Pts',(27.286744943404,3.21503560589093,0.244229406919852));
#71238=CARTESIAN_POINT('Ctrl Pts',(27.2928978075503,3.20438279292017,0.343581837321375));
#71239=CARTESIAN_POINT('Ctrl Pts',(27.2990483406868,3.19373401576275,0.442896628099881));
#71240=CARTESIAN_POINT('Ctrl Pts',(27.3051988738233,3.17845903119077,0.541759991638729));
#71241=CARTESIAN_POINT('Ctrl Pts',(27.3113494069599,3.15862092804746,0.639711962840009));
#71242=CARTESIAN_POINT('Ctrl Pts',(27.3174992551751,3.13878503406872,0.737653026142318));
#71243=CARTESIAN_POINT('Ctrl Pts',(27.3236491033903,3.11438711801296,0.834682473156558));
#71244=CARTESIAN_POINT('Ctrl Pts',(27.3297989516055,3.08554145011797,0.930350214759962));
#71245=CARTESIAN_POINT('Ctrl Pts',(27.3359497599847,3.05669127860445,1.02603289278347));
#71246=CARTESIAN_POINT('Ctrl Pts',(27.3421005683638,3.02339210136452,1.12035302719587));
#71247=CARTESIAN_POINT('Ctrl Pts',(27.348251376743,2.98580784991265,1.21287635227174));
#71248=CARTESIAN_POINT('Ctrl Pts',(27.3544087631092,2.94818340395242,1.30549862649307));
#71249=CARTESIAN_POINT('Ctrl Pts',(27.3605661494753,2.90626489644451,1.39631985091888));
#71250=CARTESIAN_POINT('Ctrl Pts',(27.3667235358415,2.86026411716212,1.48492651083304));
#71251=CARTESIAN_POINT('Ctrl Pts',(27.3728843585785,2.81423766534207,1.57358262116629));
#71252=CARTESIAN_POINT('Ctrl Pts',(27.3790451813155,2.76412462247239,1.66002132986056));
#71253=CARTESIAN_POINT('Ctrl Pts',(27.3852060040524,2.71018131863378,1.74385629643858));
#71254=CARTESIAN_POINT('Ctrl Pts',(27.3913771269691,2.65614782785938,1.82783142533906));
#71255=CARTESIAN_POINT('Ctrl Pts',(27.3975482498858,2.59827153672217,1.90919376270899));
#71256=CARTESIAN_POINT('Ctrl Pts',(27.4037193728025,2.53685050562869,1.98758825579934));
#71257=CARTESIAN_POINT('Ctrl Pts',(27.4084148947481,2.49011609386717,2.04723753967971));
#71258=CARTESIAN_POINT('Ctrl Pts',(27.4131104166936,2.44133032726672,2.10516924605325));
#71259=CARTESIAN_POINT('Ctrl Pts',(27.4178059386392,2.39063853561046,2.16124153082303));
#71260=CARTESIAN_POINT('Ctrl Pts',(27.4239782232592,2.32400394852378,2.23494880019669));
#71261=CARTESIAN_POINT('Ctrl Pts',(27.4301505078792,2.25384011050068,2.30570123689203));
#71262=CARTESIAN_POINT('Ctrl Pts',(27.4363227924992,2.1804394257938,2.37314168834143));
#71263=CARTESIAN_POINT('Ctrl Pts',(27.4424858530913,2.10714843304184,2.4404813549686));
#71264=CARTESIAN_POINT('Ctrl Pts',(27.4486489136833,2.0306305303201,2.50451858811781));
#71265=CARTESIAN_POINT('Ctrl Pts',(27.4548119742754,1.95121696965503,2.56493077875997));
#71266=CARTESIAN_POINT('Ctrl Pts',(27.458900963233,1.89852867172407,2.60501228968278));
#71267=CARTESIAN_POINT('Ctrl Pts',(27.4629899521906,1.84456656031302,2.64349878566991));
#71268=CARTESIAN_POINT('Ctrl Pts',(27.4670789411481,1.78943621037803,2.68030513402633));
#71269=CARTESIAN_POINT('Ctrl Pts',(26.2169191182387,1.78943621037807,2.6803051340263));
#71270=CARTESIAN_POINT('Ctrl Pts',(26.2195202875596,1.75456074575711,2.703588833503));
#71271=CARTESIAN_POINT('Ctrl Pts',(26.2221214568805,1.71925451683826,2.72617587672373));
#71272=CARTESIAN_POINT('Ctrl Pts',(26.2247226262013,1.68354830089748,2.74805070569035));
#71273=CARTESIAN_POINT('Ctrl Pts',(26.2308948742941,1.59882193515356,2.79995692736014));
#71274=CARTESIAN_POINT('Ctrl Pts',(26.2370671223868,1.51154367717449,2.84803248428922));
#71275=CARTESIAN_POINT('Ctrl Pts',(26.2432393704796,1.4220948302714,2.89201726416274));
#71276=CARTESIAN_POINT('Ctrl Pts',(26.2494032591323,1.33276712922469,2.93594247285106));
#71277=CARTESIAN_POINT('Ctrl Pts',(26.2555671477849,1.24127506870981,2.97578772661281));
#71278=CARTESIAN_POINT('Ctrl Pts',(26.2617310364375,1.14802764559612,3.0113369269225));
#71279=CARTESIAN_POINT('Ctrl Pts',(26.2678883980961,1.05487896297127,3.04684848388184));
#71280=CARTESIAN_POINT('Ctrl Pts',(26.2740457597546,0.959979016796753,3.07807287760163));
#71281=CARTESIAN_POINT('Ctrl Pts',(26.2802031214132,0.863759177137005,3.10484100179246));
#71282=CARTESIAN_POINT('Ctrl Pts',(26.2863559855595,0.767609619187284,3.13158957378336));
#71283=CARTESIAN_POINT('Ctrl Pts',(26.2925088497058,0.67014250174516,3.15388823164449));
#71284=CARTESIAN_POINT('Ctrl Pts',(26.2986617138521,0.571805974942881,3.17161717259817));
#71285=CARTESIAN_POINT('Ctrl Pts',(26.3048122469887,0.473506702888822,3.18933939695068));
#71286=CARTESIAN_POINT('Ctrl Pts',(26.3109627801252,0.374339102950442,3.20249526736588));
#71287=CARTESIAN_POINT('Ctrl Pts',(26.3171133132617,0.274762311042314,3.21101591944523));
#71288=CARTESIAN_POINT('Ctrl Pts',(26.3232631614769,0.175196607972742,3.21953562266759));
#71289=CARTESIAN_POINT('Ctrl Pts',(26.3294130096922,0.0752222363223799,
3.22342109675458));
#71290=CARTESIAN_POINT('Ctrl Pts',(26.3355628579074,-0.0246967458693113,
3.22265536991523));
#71291=CARTESIAN_POINT('Ctrl Pts',(26.3417136662865,-0.124631328218802,
3.22188952352443));
#71292=CARTESIAN_POINT('Ctrl Pts',(26.3478644746657,-0.224510069529359,
3.21647103714928));
#71293=CARTESIAN_POINT('Ctrl Pts',(26.3540152830448,-0.323870124502197,
3.20643504611507));
#71294=CARTESIAN_POINT('Ctrl Pts',(26.360172669411,-0.423336440167089,3.19638832208203));
#71295=CARTESIAN_POINT('Ctrl Pts',(26.3663300557772,-0.522282528777776,
3.18171427606396));
#71296=CARTESIAN_POINT('Ctrl Pts',(26.3724874421434,-0.620251993612539,
3.16249980662761));
#71297=CARTESIAN_POINT('Ctrl Pts',(26.3786482648803,-0.718276134146572,
3.14327461380358));
#71298=CARTESIAN_POINT('Ctrl Pts',(26.3848090876173,-0.815322143541676,
3.11950405455751));
#71299=CARTESIAN_POINT('Ctrl Pts',(26.3909699103543,-0.910947170904252,
3.09132541385108));
#71300=CARTESIAN_POINT('Ctrl Pts',(26.397141033271,-1.00673207220099,3.06309966173173));
#71301=CARTESIAN_POINT('Ctrl Pts',(26.4033121561876,-1.1010908353553,3.03045124930332));
#71302=CARTESIAN_POINT('Ctrl Pts',(26.4094832791043,-1.19359889319449,2.99356630871355));
#71303=CARTESIAN_POINT('Ctrl Pts',(26.4141788010499,-1.26398699299218,2.96550106834522));
#71304=CARTESIAN_POINT('Ctrl Pts',(26.4188743229954,-1.33330401096612,2.93498411166095));
#71305=CARTESIAN_POINT('Ctrl Pts',(26.423569844941,-1.40137294563341,2.90211499250921));
#71306=CARTESIAN_POINT('Ctrl Pts',(26.4297420930338,-1.49084933548923,2.85890864391843));
#71307=CARTESIAN_POINT('Ctrl Pts',(26.4359143411265,-1.57848317027901,2.81148434118327));
#71308=CARTESIAN_POINT('Ctrl Pts',(26.4420865892193,-1.66384946660023,2.76002219465607));
#71309=CARTESIAN_POINT('Ctrl Pts',(26.4482504778719,-1.74910014630453,2.70862974635332));
#71310=CARTESIAN_POINT('Ctrl Pts',(26.4544143665245,-1.83208902288109,2.65321054616829));
#71311=CARTESIAN_POINT('Ctrl Pts',(26.4605782551772,-1.91241316352887,2.59399179922788));
#71312=CARTESIAN_POINT('Ctrl Pts',(26.4667356168357,-1.99265224826145,2.53483575952191));
#71313=CARTESIAN_POINT('Ctrl Pts',(26.4728929784943,-2.07023185919341,2.47188842824619));
#71314=CARTESIAN_POINT('Ctrl Pts',(26.4790503401528,-2.14477649639595,2.40542124024203));
#71315=CARTESIAN_POINT('Ctrl Pts',(26.4852032042991,-2.21926668407337,2.33900260176415));
#71316=CARTESIAN_POINT('Ctrl Pts',(26.4913560684454,-2.29072598222601,2.26906950636281));
#71317=CARTESIAN_POINT('Ctrl Pts',(26.4975089325918,-2.35881129232412,2.19593416333556));
#71318=CARTESIAN_POINT('Ctrl Pts',(26.5036594657283,-2.42687080833359,2.12282652759961));
#71319=CARTESIAN_POINT('Ctrl Pts',(26.5098099988648,-2.49155858048394,2.04651937237726));
#71320=CARTESIAN_POINT('Ctrl Pts',(26.5159605320014,-2.55256841993906,1.96736169120723));
#71321=CARTESIAN_POINT('Ctrl Pts',(26.5221103802166,-2.61357146535872,1.88821282501031));
#71322=CARTESIAN_POINT('Ctrl Pts',(26.5282602284318,-2.67089712720563,1.80621440801598));
#71323=CARTESIAN_POINT('Ctrl Pts',(26.534410076647,-2.72428020772443,1.72174763316257));
#71324=CARTESIAN_POINT('Ctrl Pts',(26.5405608850261,-2.77767162284053,1.63726767067469));
#71325=CARTESIAN_POINT('Ctrl Pts',(26.5467116934053,-2.82711900190601,1.55031895208767));
#71326=CARTESIAN_POINT('Ctrl Pts',(26.5528625017844,-2.87240163587749,1.46130982502286));
#71327=CARTESIAN_POINT('Ctrl Pts',(26.5590198881506,-2.91773269739892,1.37220550707428));
#71328=CARTESIAN_POINT('Ctrl Pts',(26.5651772745168,-2.95888992232304,1.28103676838367));
#71329=CARTESIAN_POINT('Ctrl Pts',(26.571334660883,-2.99569963211827,1.18823452088654));
#71330=CARTESIAN_POINT('Ctrl Pts',(26.5774954836199,-3.03252988501461,1.0953804814583));
#71331=CARTESIAN_POINT('Ctrl Pts',(26.5836563063569,-3.06500764963663,1.000891528498));
#71332=CARTESIAN_POINT('Ctrl Pts',(26.5898171290939,-3.09300895730525,0.905214423509421));
#71333=CARTESIAN_POINT('Ctrl Pts',(26.5959882520106,-3.12105707990655,0.809377357518942));
#71334=CARTESIAN_POINT('Ctrl Pts',(26.6021593749272,-3.14461369373555,0.712348593933028));
#71335=CARTESIAN_POINT('Ctrl Pts',(26.6083304978439,-3.1636058069966,0.614585926000115));
#71336=CARTESIAN_POINT('Ctrl Pts',(26.6130260197895,-3.17805664290023,0.54019966616785));
#71337=CARTESIAN_POINT('Ctrl Pts',(26.6177215417351,-3.1898659282748,0.465388741797828));
#71338=CARTESIAN_POINT('Ctrl Pts',(26.6224170636807,-3.19902170219092,0.390355877900522));
#71339=CARTESIAN_POINT('Ctrl Pts',(26.6304691922115,-3.21472250589836,0.261685567946234));
#71340=CARTESIAN_POINT('Ctrl Pts',(26.6385213207423,-3.22266253234392,0.132049290773541));
#71341=CARTESIAN_POINT('Ctrl Pts',(26.6465734492731,-3.22274928133452,0.0021522448421233));
#71342=CARTESIAN_POINT('',(26.4010094512492,-3.22274887269075,-0.00269556497428082));
#71343=CARTESIAN_POINT('Ctrl Pts',(25.9683941809562,1.78943611354,2.68030519867773));
#71344=CARTESIAN_POINT('Ctrl Pts',(25.9862750553894,1.56408187620045,2.83075709901863));
#71345=CARTESIAN_POINT('Ctrl Pts',(26.0050028600116,1.32059320147187,2.95223100368197));
#71346=CARTESIAN_POINT('Ctrl Pts',(26.0279673018825,0.992141898416267,3.06719381682171));
#71347=CARTESIAN_POINT('Ctrl Pts',(26.0329550845928,0.918714969711654,3.08998194997807));
#71348=CARTESIAN_POINT('Ctrl Pts',(26.038484691514,0.834103778514802,3.11295764977937));
#71349=CARTESIAN_POINT('Ctrl Pts',(26.0391637296948,0.823656116197414,3.11573828373809));
#71350=CARTESIAN_POINT('Ctrl Pts',(26.0401646110611,0.808168160785729,3.11977703822976));
#71351=CARTESIAN_POINT('Ctrl Pts',(26.040488740381,0.803138632926547,3.12107559690212));
#71352=CARTESIAN_POINT('Ctrl Pts',(26.0410632385907,0.794199046160189,3.12336064179676));
#71353=CARTESIAN_POINT('Ctrl Pts',(26.0413138856295,0.790290261880724,3.12435195301165));
#71354=CARTESIAN_POINT('Ctrl Pts',(26.0417984804571,0.782716445568047,3.12625763434061));
#71355=CARTESIAN_POINT('Ctrl Pts',(26.0420324803753,0.779051689627456,3.12717289187437));
#71356=CARTESIAN_POINT('Ctrl Pts',(26.0426891768176,0.768746072116618,3.12972743653648));
#71357=CARTESIAN_POINT('Ctrl Pts',(26.0431110277056,0.762101539419582,3.13135203962066));
#71358=CARTESIAN_POINT('Ctrl Pts',(26.0448562184165,0.734514802410653,3.13800404937277));
#71359=CARTESIAN_POINT('Ctrl Pts',(26.0461690268333,0.713527051522341,3.14284275995976));
#71360=CARTESIAN_POINT('Ctrl Pts',(26.0560544390594,0.553858272908785,3.17797233277397));
#71361=CARTESIAN_POINT('Ctrl Pts',(26.0641745783986,0.413342969048163,3.19928502823633));
#71362=CARTESIAN_POINT('Ctrl Pts',(26.0814424553223,0.107900091086263,3.22514375483868));
#71363=CARTESIAN_POINT('Ctrl Pts',(26.0905299155026,-0.0568856550565677,
3.22644683427784));
#71364=CARTESIAN_POINT('Ctrl Pts',(26.1090701465529,-0.383501672051364,
3.20399111385713));
#71365=CARTESIAN_POINT('Ctrl Pts',(26.1184930056003,-0.544850785095286,
3.18052817623539));
#71366=CARTESIAN_POINT('Ctrl Pts',(26.1295084298647,-0.722835616403641,
3.14070211854582));
#71367=CARTESIAN_POINT('Ctrl Pts',(26.1306967150248,-0.741908052521871,
3.13625151114838));
#71368=CARTESIAN_POINT('Ctrl Pts',(26.1324550938611,-0.769936639467185,
3.12944098557048));
#71369=CARTESIAN_POINT('Ctrl Pts',(26.1330208393143,-0.778925319812664,
3.12721579912497));
#71370=CARTESIAN_POINT('Ctrl Pts',(26.134031566098,-0.79493103856015,3.12318022560902));
#71371=CARTESIAN_POINT('Ctrl Pts',(26.1344760590866,-0.801951823373376,
3.12138484479681));
#71372=CARTESIAN_POINT('Ctrl Pts',(26.1354072568903,-0.816621854976992,
3.11758060918399));
#71373=CARTESIAN_POINT('Ctrl Pts',(26.135894105322,-0.824269873612342,3.11556724890667));
#71374=CARTESIAN_POINT('Ctrl Pts',(26.1371670437694,-0.844209482136554,
3.11023953752172));
#71375=CARTESIAN_POINT('Ctrl Pts',(26.1379545822111,-0.856488889992263,
3.10688049405498));
#71376=CARTESIAN_POINT('Ctrl Pts',(26.1414119246108,-0.910144754672631,
3.09186061641825));
#71377=CARTESIAN_POINT('Ctrl Pts',(26.1441062070609,-0.951303853931254,
3.07944576748346));
#71378=CARTESIAN_POINT('Ctrl Pts',(26.1512568797071,-1.05878190997055,3.04466675810205));
#71379=CARTESIAN_POINT('Ctrl Pts',(26.1557557282274,-1.12463921888404,3.02096015258786));
#71380=CARTESIAN_POINT('Ctrl Pts',(26.1760522224431,-1.41404286899356,2.90600870926));
#71381=CARTESIAN_POINT('Ctrl Pts',(26.1925389708112,-1.62767324440314,2.79196289073635));
#71382=CARTESIAN_POINT('Ctrl Pts',(26.218195257074,-1.94173101277219,2.57591706722954));
#71383=CARTESIAN_POINT('Ctrl Pts',(26.2274788640208,-2.05166462839362,2.48924690871577));
#71384=CARTESIAN_POINT('Ctrl Pts',(26.2370686372156,-2.16454180999246,2.38768088237464));
#71385=CARTESIAN_POINT('Ctrl Pts',(26.2378222359196,-2.17340773254435,2.37961343121592));
#71386=CARTESIAN_POINT('Ctrl Pts',(26.2389075300396,-2.18617280787062,2.36786713016513));
#71387=CARTESIAN_POINT('Ctrl Pts',(26.2392421388631,-2.19010798949337,2.36422784167202));
#71388=CARTESIAN_POINT('Ctrl Pts',(26.2398293187376,-2.19701311711815,2.35780988772424));
#71389=CARTESIAN_POINT('Ctrl Pts',(26.2400822071318,-2.19998690593365,2.3550353963162));
#71390=CARTESIAN_POINT('Ctrl Pts',(26.2406097732138,-2.20619056196325,2.34922549193433));
#71391=CARTESIAN_POINT('Ctrl Pts',(26.2408843685167,-2.20941941505017,2.34618904963226));
#71392=CARTESIAN_POINT('Ctrl Pts',(26.2414419415908,-2.21597514985097,2.33999844320824));
#71393=CARTESIAN_POINT('Ctrl Pts',(26.2417248831492,-2.21930158732189,2.33684382107471));
#71394=CARTESIAN_POINT('Ctrl Pts',(26.2429084624773,-2.2332146113743,2.3235929229163));
#71395=CARTESIAN_POINT('Ctrl Pts',(26.2438041869038,-2.24373932998335,2.31343152260835));
#71396=CARTESIAN_POINT('Ctrl Pts',(26.2513734583802,-2.33259386740233,2.22646749333747));
#71397=CARTESIAN_POINT('Ctrl Pts',(26.25776322999,-2.40703326878843,2.14577443549519));
#71398=CARTESIAN_POINT('Ctrl Pts',(26.2690676220834,-2.53374420816703,1.99350620570902));
#71399=CARTESIAN_POINT('Ctrl Pts',(26.2740224139885,-2.58745387204066,1.92328110857984));
#71400=CARTESIAN_POINT('Ctrl Pts',(26.2845955633612,-2.69604155936059,1.76850680122655));
#71401=CARTESIAN_POINT('Ctrl Pts',(26.2902049118871,-2.74997689519084,1.68341410550009));
#71402=CARTESIAN_POINT('Ctrl Pts',(26.3059853256336,-2.88853167898846,1.4403399727848));
#71403=CARTESIAN_POINT('Ctrl Pts',(26.316296699378,-2.96408694447702,1.27764225545488));
#71404=CARTESIAN_POINT('Ctrl Pts',(26.3281864926893,-3.03187410057892,1.09278314852782));
#71405=CARTESIAN_POINT('Ctrl Pts',(26.329267857943,-3.03787439526123,1.07599010698718));
#71406=CARTESIAN_POINT('Ctrl Pts',(26.330910487572,-3.04673881745804,1.05051591312671));
#71407=CARTESIAN_POINT('Ctrl Pts',(26.331468334425,-3.04970595377072,1.04187076855414));
#71408=CARTESIAN_POINT('Ctrl Pts',(26.3324407708177,-3.05480289781833,1.02681180846687));
#71409=CARTESIAN_POINT('Ctrl Pts',(26.3328548053832,-3.0569493922244,1.02040366855599));
#71410=CARTESIAN_POINT('Ctrl Pts',(26.3337202957956,-3.06138703336622,1.00701586846609));
#71411=CARTESIAN_POINT('Ctrl Pts',(26.3341718703257,-3.06367450106895,1.00003503812652));
#71412=CARTESIAN_POINT('Ctrl Pts',(26.3352425328886,-3.06903192745464,0.983494485798373));
#71413=CARTESIAN_POINT('Ctrl Pts',(26.3358623016034,-3.07208110432941,0.973928159617502));
#71414=CARTESIAN_POINT('Ctrl Pts',(26.3379233502066,-3.08204846273097,0.942144524659304));
#71415=CARTESIAN_POINT('Ctrl Pts',(26.3393710423203,-3.08877059467976,0.919866946691408));
#71416=CARTESIAN_POINT('Ctrl Pts',(26.3428014094527,-3.10404200772749,0.867200815584315));
#71417=CARTESIAN_POINT('Ctrl Pts',(26.3447905676136,-3.11238707298319,0.836756018406303));
#71418=CARTESIAN_POINT('Ctrl Pts',(26.3641168622528,-3.18856181589396,0.541930374655944));
#71419=CARTESIAN_POINT('Ctrl Pts',(26.3825654833146,-3.22297705881999,0.270117963095652));
#71420=CARTESIAN_POINT('Ctrl Pts',(26.4010094512492,-3.22274887269075,-0.00269556497428082));
#71421=CARTESIAN_POINT('Ctrl Pts',(26.4010096337881,-3.22274887043127,-0.00269826499466809));
#71422=CARTESIAN_POINT('Ctrl Pts',(26.4121186745204,-3.22261129329353,-0.167017398262714));
#71423=CARTESIAN_POINT('Ctrl Pts',(26.4231487577878,-3.20990655326697,-0.331110276176874));
#71424=CARTESIAN_POINT('Ctrl Pts',(26.4343606437183,-3.1828837039125,-0.505484950292156));
#71425=CARTESIAN_POINT('Ctrl Pts',(26.4351254551143,-3.18096512398751,-0.517421103233719));
#71426=CARTESIAN_POINT('Ctrl Pts',(26.436312386118,-3.17786906210822,-0.536014442295224));
#71427=CARTESIAN_POINT('Ctrl Pts',(26.4367369393384,-3.17673774542171,-0.542679055231531));
#71428=CARTESIAN_POINT('Ctrl Pts',(26.4374472336888,-3.17480467837527,-0.553853588593734));
#71429=CARTESIAN_POINT('Ctrl Pts',(26.4377335965835,-3.17401427392945,-0.558365411658908));
#71430=CARTESIAN_POINT('Ctrl Pts',(26.4382958196711,-3.17244058574248,-0.567237087864773));
#71431=CARTESIAN_POINT('Ctrl Pts',(26.4385717144258,-3.17165792730845,-0.571597040425067));
#71432=CARTESIAN_POINT('Ctrl Pts',(26.4390999847287,-3.17013925795697,-0.579957926456444));
#71433=CARTESIAN_POINT('Ctrl Pts',(26.439352436685,-3.16940466263672,-0.583959070395097));
#71434=CARTESIAN_POINT('Ctrl Pts',(26.4399368709176,-3.16768354891457,-0.593234598143494));
#71435=CARTESIAN_POINT('Ctrl Pts',(26.4402685326961,-3.16669142567133,-0.598507953219022));
#71436=CARTESIAN_POINT('Ctrl Pts',(26.4413406748695,-3.16343444176448,-0.615584716931534));
#71437=CARTESIAN_POINT('Ctrl Pts',(26.4420781923233,-3.16111668993797,-0.627378111070465));
#71438=CARTESIAN_POINT('Ctrl Pts',(26.4526362183705,-3.12683037130919,-0.796821729327422));
#71439=CARTESIAN_POINT('Ctrl Pts',(26.4618256011249,-3.08316323520662,-0.951899441759739));
#71440=CARTESIAN_POINT('Ctrl Pts',(26.4741650916175,-3.00808503580704,-1.15799714241869));
#71441=CARTESIAN_POINT('Ctrl Pts',(26.4774315163031,-2.98659147719117,-1.21235492469407));
#71442=CARTESIAN_POINT('Ctrl Pts',(26.483564048068,-2.94347758124824,-1.31327415113217));
#71443=CARTESIAN_POINT('Ctrl Pts',(26.4864293571623,-2.92220021164542,-1.35996144789546));
#71444=CARTESIAN_POINT('Ctrl Pts',(26.4962202709985,-2.84600862856226,-1.51708999299155));
#71445=CARTESIAN_POINT('Ctrl Pts',(26.503194254275,-2.78587726369822,-1.62487287463776));
#71446=CARTESIAN_POINT('Ctrl Pts',(26.5151650145065,-2.67529521899633,-1.79882481666908));
#71447=CARTESIAN_POINT('Ctrl Pts',(26.5200529671178,-2.62819487614635,-1.86696684381829));
#71448=CARTESIAN_POINT('Ctrl Pts',(26.5264392343859,-2.56460305482445,-1.95178569980153));
#71449=CARTESIAN_POINT('Ctrl Pts',(26.5278450121286,-2.55048052957625,-1.97020437306477));
#71450=CARTESIAN_POINT('Ctrl Pts',(26.5298695634986,-2.52997192029836,-1.99636175260268));
#71451=CARTESIAN_POINT('Ctrl Pts',(26.5304819425698,-2.52374651061654,-2.00422596314021));
#71452=CARTESIAN_POINT('Ctrl Pts',(26.5315452706214,-2.51289932347848,-2.01779793095763));
#71453=CARTESIAN_POINT('Ctrl Pts',(26.5319955350353,-2.50829453433871,-2.02351921851635));
#71454=CARTESIAN_POINT('Ctrl Pts',(26.5328617961108,-2.49941348619525,-2.03447671195646));
#71455=CARTESIAN_POINT('Ctrl Pts',(26.5332776700814,-2.49514022402318,-2.03971530558013));
#71456=CARTESIAN_POINT('Ctrl Pts',(26.534257967935,-2.48504483428835,-2.05201204887028));
#71457=CARTESIAN_POINT('Ctrl Pts',(26.5348229444268,-2.47920909225613,-2.05905889940944));
#71458=CARTESIAN_POINT('Ctrl Pts',(26.5364949871602,-2.46188749556562,-2.07979490313753));
#71459=CARTESIAN_POINT('Ctrl Pts',(26.5376054830227,-2.45031784828192,-2.09341331360936));
#71460=CARTESIAN_POINT('Ctrl Pts',(26.5501271182865,-2.31914607461688,-2.24523586001842));
#71461=CARTESIAN_POINT('Ctrl Pts',(26.5620294418599,-2.18812940259257,-2.37309753618723));
#71462=CARTESIAN_POINT('Ctrl Pts',(26.5811807517603,-1.96691318433478,-2.55501924394301));
#71463=CARTESIAN_POINT('Ctrl Pts',(26.5881986166319,-1.88369020936753,-2.61697930134381));
#71464=CARTESIAN_POINT('Ctrl Pts',(26.6048919483904,-1.67898925377064,-2.75454989631325));
#71465=CARTESIAN_POINT('Ctrl Pts',(26.6145534311206,-1.55516851535591,-2.82630616016101));
#71466=CARTESIAN_POINT('Ctrl Pts',(26.6263550834399,-1.3931016571962,-2.90634020776058));
#71467=CARTESIAN_POINT('Ctrl Pts',(26.6287982451854,-1.35892496187755,-2.92247649209751));
#71468=CARTESIAN_POINT('Ctrl Pts',(26.6326755752923,-1.30354428337436,-2.94744241322381));
#71469=CARTESIAN_POINT('Ctrl Pts',(26.6341291656382,-1.28251685610137,-2.95665267883043));
#71470=CARTESIAN_POINT('Ctrl Pts',(26.6360082368995,-1.25496077868726,-2.96837326685409));
#71471=CARTESIAN_POINT('Ctrl Pts',(26.63644557803,-1.24852049012467,-2.97108784712326));
#71472=CARTESIAN_POINT('Ctrl Pts',(26.6371178949995,-1.23857766707844,-2.97524070627342));
#71473=CARTESIAN_POINT('Ctrl Pts',(26.6373537614126,-1.23508139304846,-2.97669377843107));
#71474=CARTESIAN_POINT('Ctrl Pts',(26.6378395552432,-1.22786355836495,-2.97967864721995));
#71475=CARTESIAN_POINT('Ctrl Pts',(26.63808942663,-1.22414173171451,-2.98120961684502));
#71476=CARTESIAN_POINT('Ctrl Pts',(26.6386558362101,-1.21568411128581,-2.98467014160479));
#71477=CARTESIAN_POINT('Ctrl Pts',(26.6389721110374,-1.21094659867696,-2.98659539419578));
#71478=CARTESIAN_POINT('Ctrl Pts',(26.6399089028817,-1.19687082728374,-2.99227657381846));
#71479=CARTESIAN_POINT('Ctrl Pts',(26.6405274871799,-1.18751942777361,-2.99600008117042));
#71480=CARTESIAN_POINT('Ctrl Pts',(26.6449004774938,-1.12102156073245,-3.02211770283802));
#71481=CARTESIAN_POINT('Ctrl Pts',(26.6485643511902,-1.06325873553265,-3.04292076274468));
#71482=CARTESIAN_POINT('Ctrl Pts',(26.6529542810041,-0.992123082267575,
-3.06626664049294));
#71483=CARTESIAN_POINT('Ctrl Pts',(26.6537416294839,-0.97928708375435,-3.07039022569353));
#71484=CARTESIAN_POINT('Ctrl Pts',(26.6639610411744,-0.811740283079375,
-3.1230573279779));
#71485=CARTESIAN_POINT('Ctrl Pts',(26.6729763537689,-0.653594213380525,
-3.15994175292379));
#71486=CARTESIAN_POINT('Ctrl Pts',(26.6956874868583,-0.252017843874257,
-3.22214761244565));
#71487=CARTESIAN_POINT('Ctrl Pts',(26.7094251756833,-0.00727353578249663,
-3.23197667661168));
#71488=CARTESIAN_POINT('Ctrl Pts',(26.7254837568322,0.258400618041433,-3.21245099427739));
#71489=CARTESIAN_POINT('Ctrl Pts',(26.726831532051,0.280564897612453,-3.21059115585256));
#71490=CARTESIAN_POINT('Ctrl Pts',(26.7287870930218,0.312522259269744,-3.20757612260754));
#71491=CARTESIAN_POINT('Ctrl Pts',(26.7293890758968,0.322332400186727,-3.20660514645193));
#71492=CARTESIAN_POINT('Ctrl Pts',(26.7304402002458,0.339413459592343,-3.2048353419119));
#71493=CARTESIAN_POINT('Ctrl Pts',(26.7308887007493,0.346686436824137,-3.20405673770643));
#71494=CARTESIAN_POINT('Ctrl Pts',(26.7317557734559,0.360717235201576,-3.20250634695158));
#71495=CARTESIAN_POINT('Ctrl Pts',(26.7321742374839,0.367475393605659,-3.20173791244673));
#71496=CARTESIAN_POINT('Ctrl Pts',(26.7332785629056,0.385274652062921,-3.19965695562141));
#71497=CARTESIAN_POINT('Ctrl Pts',(26.7339655508869,0.396311407791546,-3.19830868651856));
#71498=CARTESIAN_POINT('Ctrl Pts',(26.7363771269379,0.434926744808454,-3.19338842377495));
#71499=CARTESIAN_POINT('Ctrl Pts',(26.7381111625164,0.46246525763062,-3.18951668842466));
#71500=CARTESIAN_POINT('Ctrl Pts',(26.7402515047593,0.496170128666749,-3.18433232831835));
#71501=CARTESIAN_POINT('Ctrl Pts',(26.7406471000612,0.502387866084007,-3.18335728514112));
#71502=CARTESIAN_POINT('Ctrl Pts',(26.75863090919,0.7845061799744,-3.13826937989728));
#71503=CARTESIAN_POINT('Ctrl Pts',(26.7774279093371,1.05345148678312,-3.0584898526404));
#71504=CARTESIAN_POINT('Ctrl Pts',(26.8042387666291,1.41556997101274,-2.89757853790005));
#71505=CARTESIAN_POINT('Ctrl Pts',(26.8121283714573,1.51980357024219,-2.84429252101251));
#71506=CARTESIAN_POINT('Ctrl Pts',(26.8229480253343,1.66199858984273,-2.76154626606062));
#71507=CARTESIAN_POINT('Ctrl Pts',(26.8260400570294,1.70255148836966,-2.73673090044666));
#71508=CARTESIAN_POINT('Ctrl Pts',(26.8308264346393,1.76541923705433,-2.69632194489141));
#71509=CARTESIAN_POINT('Ctrl Pts',(26.8325524383462,1.78810969535144,-2.681328205838));
#71510=CARTESIAN_POINT('Ctrl Pts',(26.8347257363155,1.81674199547524,-2.66188299049598));
#71511=CARTESIAN_POINT('Ctrl Pts',(26.8351899270656,1.82286115716929,-2.65769632153089));
#71512=CARTESIAN_POINT('Ctrl Pts',(26.8359340837868,1.83267776518594,-2.65093004346586));
#71513=CARTESIAN_POINT('Ctrl Pts',(26.8362149416402,1.83638429760424,-2.64836375871314));
#71514=CARTESIAN_POINT('Ctrl Pts',(26.8367467784661,1.84340628438653,-2.64348012950935));
#71515=CARTESIAN_POINT('Ctrl Pts',(26.8369978546372,1.84672272087482,-2.64116434869057));
#71516=CARTESIAN_POINT('Ctrl Pts',(26.8375713246262,1.85430066103077,-2.63585161993951));
#71517=CARTESIAN_POINT('Ctrl Pts',(26.8378934336712,1.85855925762253,-2.63285058266675));
#71518=CARTESIAN_POINT('Ctrl Pts',(26.8387461822136,1.8698385286706,-2.62486106545853));
#71519=CARTESIAN_POINT('Ctrl Pts',(26.8392756144362,1.87684657349928,-2.61985470584709));
#71520=CARTESIAN_POINT('Ctrl Pts',(26.8428415303304,1.92407575351156,-2.58582867229419));
#71521=CARTESIAN_POINT('Ctrl Pts',(26.8458188982536,1.96364496210872,-2.5559101172501));
#71522=CARTESIAN_POINT('Ctrl Pts',(26.8678764911133,2.25607770989934,-2.3239975929221));
#71523=CARTESIAN_POINT('Ctrl Pts',(26.8850926628562,2.47793538735777,-2.0858435978511));
#71524=CARTESIAN_POINT('Ctrl Pts',(26.9081913231658,2.70453079832163,-1.75433453757879));
#71525=CARTESIAN_POINT('Ctrl Pts',(26.9127311636779,2.74611018197335,-1.68850646065199));
#71526=CARTESIAN_POINT('Ctrl Pts',(26.9201173606876,2.80865392053139,-1.58105741273324));
#71527=CARTESIAN_POINT('Ctrl Pts',(26.9229085389498,2.83117065386919,-1.54037390900502));
#71528=CARTESIAN_POINT('Ctrl Pts',(26.926526107741,2.85888832972751,-1.48763115234238));
#71529=CARTESIAN_POINT('Ctrl Pts',(26.9273233709222,2.86490734440611,-1.47600637780861));
#71530=CARTESIAN_POINT('Ctrl Pts',(26.9286112149478,2.87448523603994,-1.45722888092234));
#71531=CARTESIAN_POINT('Ctrl Pts',(26.9291002225873,2.87808867272459,-1.4500989530794));
#71532=CARTESIAN_POINT('Ctrl Pts',(26.930033344504,2.88490102687603,-1.4364942904525));
#71533=CARTESIAN_POINT('Ctrl Pts',(26.9304772864347,2.88811475465547,-1.43002200820815));
#71534=CARTESIAN_POINT('Ctrl Pts',(26.9314917486236,2.89539612006079,-1.41523304904778));
#71535=CARTESIAN_POINT('Ctrl Pts',(26.9320627548254,2.89944972884628,-1.40690957143963));
#71536=CARTESIAN_POINT('Ctrl Pts',(26.9338133141717,2.91173975813742,-1.3813951320497));
#71537=CARTESIAN_POINT('Ctrl Pts',(26.9349969092012,2.91985945324567,-1.36414870087742));
#71538=CARTESIAN_POINT('Ctrl Pts',(26.9525107317908,3.03720649457058,-1.10905246030922));
#71539=CARTESIAN_POINT('Ctrl Pts',(26.9698977957588,3.11719092759398,-0.858885623109628));
#71540=CARTESIAN_POINT('Ctrl Pts',(27.0013582734629,3.20404110378433,-0.402019905246797));
#71541=CARTESIAN_POINT('Ctrl Pts',(27.0152016872114,3.22302808928914,-0.199007889242898));
#71542=CARTESIAN_POINT('Ctrl Pts',(27.0298840806747,3.22271096853025,0.0304712543785456));
#71543=CARTESIAN_POINT('Ctrl Pts',(27.0315342409979,3.22235994726802,0.0564885580357998));
#71544=CARTESIAN_POINT('Ctrl Pts',(27.0336271922966,3.22150647239905,0.089817575388892));
#71545=CARTESIAN_POINT('Ctrl Pts',(27.0340853976509,3.22129414546707,0.0971348517459847));
#71546=CARTESIAN_POINT('Ctrl Pts',(27.0348201205761,3.2209125534913,0.108902326003328));
#71547=CARTESIAN_POINT('Ctrl Pts',(27.0350975081195,3.22075899471722,0.113352954834058));
#71548=CARTESIAN_POINT('Ctrl Pts',(27.035626796076,3.2204477951274,0.121860767114268));
#71549=CARTESIAN_POINT('Ctrl Pts',(27.0358787799092,3.2202917127762,0.125917959286913));
#71550=CARTESIAN_POINT('Ctrl Pts',(27.0364596679059,3.21991357723222,0.135286268947646));
#71551=CARTESIAN_POINT('Ctrl Pts',(27.0367882637617,3.21968604915869,0.140597173600685));
#71552=CARTESIAN_POINT('Ctrl Pts',(27.0378405847351,3.21891361318267,0.157640950095602));
#71553=CARTESIAN_POINT('Ctrl Pts',(27.0385614978897,3.21831769657642,0.169371579920336));
#71554=CARTESIAN_POINT('Ctrl Pts',(27.0508935673475,3.20697436914158,0.370913082575582));
#71555=CARTESIAN_POINT('Ctrl Pts',(27.0616203192773,3.17951396796986,0.559441617585424));
#71556=CARTESIAN_POINT('Ctrl Pts',(27.0815126609903,3.09743822290574,0.905129658231472));
#71557=CARTESIAN_POINT('Ctrl Pts',(27.090671127175,3.04700341536141,1.06261516721349));
#71558=CARTESIAN_POINT('Ctrl Pts',(27.1051168285971,2.9518144187653,1.2963499831127));
#71559=CARTESIAN_POINT('Ctrl Pts',(27.1101839477628,2.91563640314851,1.37578858887188));
#71560=CARTESIAN_POINT('Ctrl Pts',(27.1183507704404,2.85349719420353,1.49874045733883));
#71561=CARTESIAN_POINT('Ctrl Pts',(27.1213790762972,2.82965666111281,1.54327960747503));
#71562=CARTESIAN_POINT('Ctrl Pts',(27.1252623657313,2.79814518715527,1.59896296564468));
#71563=CARTESIAN_POINT('Ctrl Pts',(27.1260826333789,2.79143677480003,1.61064576415304));
#71564=CARTESIAN_POINT('Ctrl Pts',(27.1273987367103,2.7805911672252,1.62926225913326));
#71565=CARTESIAN_POINT('Ctrl Pts',(27.1278928713464,2.77650077489499,1.63622314902888));
#71566=CARTESIAN_POINT('Ctrl Pts',(27.1288300439717,2.76870851826612,1.64937038823725));
#71567=CARTESIAN_POINT('Ctrl Pts',(27.1292728861002,2.76501196274502,1.65555983922217));
#71568=CARTESIAN_POINT('Ctrl Pts',(27.1302769789456,2.75659795575244,1.6695413271059));
#71569=CARTESIAN_POINT('Ctrl Pts',(27.1308386791731,2.75186818963315,1.67732584691534));
#71570=CARTESIAN_POINT('Ctrl Pts',(27.1322851961244,2.73962967443922,1.69727759415437));
#71571=CARTESIAN_POINT('Ctrl Pts',(27.1331717792957,2.73207290316657,1.70941499521389));
#71572=CARTESIAN_POINT('Ctrl Pts',(27.1384913559115,2.68640354481649,1.78169098624212));
#71573=CARTESIAN_POINT('Ctrl Pts',(27.1429948707185,2.64638991860623,1.84059932545311));
#71574=CARTESIAN_POINT('Ctrl Pts',(27.1484414938695,2.59645874091737,1.90911083082271));
#71575=CARTESIAN_POINT('Ctrl Pts',(27.1493168732594,2.58838727599272,1.92003996274891));
#71576=CARTESIAN_POINT('Ctrl Pts',(27.15056074101,2.57685231411846,1.93545390435554));
#71577=CARTESIAN_POINT('Ctrl Pts',(27.1509272280218,2.57344565101361,1.93998122292042));
#71578=CARTESIAN_POINT('Ctrl Pts',(27.1542208252032,2.54275782642465,1.9805410378715));
#71579=CARTESIAN_POINT('Ctrl Pts',(27.1571735936018,2.51473445496887,2.01600359557661));
#71580=CARTESIAN_POINT('Ctrl Pts',(27.1604927693031,2.48265541429687,2.05488853164906));
#71581=CARTESIAN_POINT('Ctrl Pts',(27.1608366038338,2.47932546493765,2.05890505418431));
#71582=CARTESIAN_POINT('Ctrl Pts',(27.161405992525,2.47379967420169,2.06553731463336));
#71583=CARTESIAN_POINT('Ctrl Pts',(27.1616313791936,2.47160939505537,2.068157688462));
#71584=CARTESIAN_POINT('Ctrl Pts',(27.1783784459326,2.30864378689708,2.26249545822776));
#71585=CARTESIAN_POINT('Ctrl Pts',(27.1955990383909,2.12611257465518,2.43482023122181));
#71586=CARTESIAN_POINT('Ctrl Pts',(27.2159207726962,1.8809818804662,2.617461929932));
#71587=CARTESIAN_POINT('Ctrl Pts',(27.2195749660459,1.83561176651236,2.64947722153259));
#71588=CARTESIAN_POINT('Ctrl Pts',(27.2231721927303,1.78943620958681,2.68030513455457));
#71589=CARTESIAN_POINT('Origin',(-1.72497344927317,0.,0.));
#71590=CARTESIAN_POINT('',(28.7169416469173,1.789436210378,2.68030513402635));
#71591=CARTESIAN_POINT('',(28.4706129526677,1.78943608566475,2.68030521728792));
#71592=CARTESIAN_POINT('',(-1.72497344927317,1.78943621037804,2.68030513402633));
#71593=CARTESIAN_POINT('',(27.8965734492388,-3.22274961841222,0.00156828692453643));
#71594=CARTESIAN_POINT('Ctrl Pts',(27.8965734492731,-3.22274961841249,0.00156828636609923));
#71595=CARTESIAN_POINT('Ctrl Pts',(27.9028189460097,-3.22279908535359,-0.10008379004733));
#71596=CARTESIAN_POINT('Ctrl Pts',(27.9090644427464,-3.21803473533519,-0.20172558506841));
#71597=CARTESIAN_POINT('Ctrl Pts',(27.915309939483,-3.2084859097739,-0.30287906709174));
#71598=CARTESIAN_POINT('Ctrl Pts',(27.9215577451443,-3.19893355406604,-0.404069944982713));
#71599=CARTESIAN_POINT('Ctrl Pts',(27.9278055508057,-3.18459324202756,-0.504771737031726));
#71600=CARTESIAN_POINT('Ctrl Pts',(27.934053356467,-3.16554606939534,-0.604512733559599));
#71601=CARTESIAN_POINT('Ctrl Pts',(27.9403049328509,-3.14648740127037,-0.704313926523192));
#71602=CARTESIAN_POINT('Ctrl Pts',(27.9465565092348,-3.122716297478,-0.803152762404056));
#71603=CARTESIAN_POINT('Ctrl Pts',(27.9528080856187,-3.09436453475874,-0.900569646683341));
#71604=CARTESIAN_POINT('Ctrl Pts',(27.9590691794596,-3.06596960905706,-0.998134839316647));
#71605=CARTESIAN_POINT('Ctrl Pts',(27.9653302733005,-3.03298021842741,-1.09427335940052));
#71606=CARTESIAN_POINT('Ctrl Pts',(27.9715913671414,-2.99557747238081,-1.18854245589487));
#71607=CARTESIAN_POINT('Ctrl Pts',(27.9778580248593,-2.95814148864664,-1.2828953239597));
#71608=CARTESIAN_POINT('Ctrl Pts',(27.9841246825773,-2.91628450781737,-1.37537508170243));
#71609=CARTESIAN_POINT('Ctrl Pts',(27.9903913402952,-2.87023420671054,-1.46556240437885));
#71610=CARTESIAN_POINT('Ctrl Pts',(27.9966690963733,-2.82410234971761,-1.55590945037606));
#71611=CARTESIAN_POINT('Ctrl Pts',(28.0029468524513,-2.77376255116826,-1.64395559618616));
#71612=CARTESIAN_POINT('Ctrl Pts',(28.0092246085293,-2.71948654939906,-1.72930924653099));
#71613=CARTESIAN_POINT('Ctrl Pts',(28.0109322706389,-2.70472250464632,-1.75252696840483));
#71614=CARTESIAN_POINT('Ctrl Pts',(28.0126399327485,-2.68966743765888,-1.77554564917328));
#71615=CARTESIAN_POINT('Ctrl Pts',(28.0143475948581,-2.67432732614984,-1.79835783844825));
#71616=CARTESIAN_POINT('Ctrl Pts',(28.0205198429509,-2.6188813608904,-1.88081120609726));
#71617=CARTESIAN_POINT('Ctrl Pts',(28.0266920910437,-2.55952099760056,-1.96084307949786));
#71618=CARTESIAN_POINT('Ctrl Pts',(28.0328643391364,-2.49648473396866,-2.03805827580112));
#71619=CARTESIAN_POINT('Ctrl Pts',(28.0390282277891,-2.43353384407167,-2.11516889500351));
#71620=CARTESIAN_POINT('Ctrl Pts',(28.0451921164417,-2.36691722140644,-2.18947008590427));
#71621=CARTESIAN_POINT('Ctrl Pts',(28.0513560050944,-2.29691685977599,-2.26059516538827));
#71622=CARTESIAN_POINT('Ctrl Pts',(28.0575133667529,-2.2269906221233,-2.33164492992122));
#71623=CARTESIAN_POINT('Ctrl Pts',(28.0636707284115,-2.15368807199885,-2.39952496153859));
#71624=CARTESIAN_POINT('Ctrl Pts',(28.06982809007,-2.07733110069408,-2.46390199898233));
#71625=CARTESIAN_POINT('Ctrl Pts',(28.0759809542163,-2.00102990269496,-2.52823201360518));
#71626=CARTESIAN_POINT('Ctrl Pts',(28.0821338183627,-1.92167905029059,-2.58906384201416));
#71627=CARTESIAN_POINT('Ctrl Pts',(28.088286682509,-1.83963620800017,-2.64610207375202));
#71628=CARTESIAN_POINT('Ctrl Pts',(28.0944372156455,-1.75762444760312,-2.70311869658181));
#71629=CARTESIAN_POINT('Ctrl Pts',(28.100587748782,-1.67292308003103,-2.75634433077547));
#71630=CARTESIAN_POINT('Ctrl Pts',(28.1067382819186,-1.58592095440542,-2.80552531424648));
#71631=CARTESIAN_POINT('Ctrl Pts',(28.1128881301338,-1.49892851730764,-2.8547008209395));
#71632=CARTESIAN_POINT('Ctrl Pts',(28.119037978349,-1.40963620968297,-2.89983235863566));
#71633=CARTESIAN_POINT('Ctrl Pts',(28.1251878265642,-1.3184589484762,-2.94071140435151));
#71634=CARTESIAN_POINT('Ctrl Pts',(28.1313386349433,-1.22726745193973,-2.98159683243382));
#71635=CARTESIAN_POINT('Ctrl Pts',(28.1374894433224,-1.1341908136752,-3.01822827206873));
#71636=CARTESIAN_POINT('Ctrl Pts',(28.1436402517016,-1.03966452913,-3.05044508709285));
#71637=CARTESIAN_POINT('Ctrl Pts',(28.1497976380678,-0.945037153372402,
-3.08269635641617));
#71638=CARTESIAN_POINT('Ctrl Pts',(28.155955024434,-0.848957447447346,-3.11052343292884));
#71639=CARTESIAN_POINT('Ctrl Pts',(28.1621124108001,-0.751876581154286,
-3.13381543317595));
#71640=CARTESIAN_POINT('Ctrl Pts',(28.1682732335371,-0.654741535079018,
-3.15712043243665));
#71641=CARTESIAN_POINT('Ctrl Pts',(28.1744340562741,-0.556604642579021,
-3.17588523344432));
#71642=CARTESIAN_POINT('Ctrl Pts',(28.180594879011,-0.457925721217903,-3.1900504065527));
#71643=CARTESIAN_POINT('Ctrl Pts',(28.1867660019277,-0.359081820166839,
-3.20423926218452));
#71644=CARTESIAN_POINT('Ctrl Pts',(28.1929371248444,-0.259694512704669,
-3.21381308762326));
#71645=CARTESIAN_POINT('Ctrl Pts',(28.1991082477611,-0.160227315433129,
-3.21876447878516));
#71646=CARTESIAN_POINT('Ctrl Pts',(28.2038037697067,-0.0845441028384395,
-3.22253192373409));
#71647=CARTESIAN_POINT('Ctrl Pts',(28.2084992916522,-0.00881471394602323,
-3.2236242991668));
#71648=CARTESIAN_POINT('Ctrl Pts',(28.2131948135978,0.0667584762774016,
-3.22205848307338));
#71649=CARTESIAN_POINT('Ctrl Pts',(28.2193670616906,0.166099185282368,-3.22000022298892));
#71650=CARTESIAN_POINT('Ctrl Pts',(28.2255393097833,0.265519466835396,-3.21333980965354));
#71651=CARTESIAN_POINT('Ctrl Pts',(28.2317115578761,0.364557931459154,-3.20206419003589));
#71652=CARTESIAN_POINT('Ctrl Pts',(28.2378754465287,0.463462262440905,-3.19080384165585));
#71653=CARTESIAN_POINT('Ctrl Pts',(28.2440393351813,0.561985376533668,-3.17494075954533));
#71654=CARTESIAN_POINT('Ctrl Pts',(28.250203223834,0.659666339695656,-3.15451389009028));
#71655=CARTESIAN_POINT('Ctrl Pts',(28.2563605854925,0.75724386765521,-3.13410865082098));
#71656=CARTESIAN_POINT('Ctrl Pts',(28.262517947151,0.853980594754985,-3.10914932036058));
#71657=CARTESIAN_POINT('Ctrl Pts',(28.2686753088095,0.949422128736799,-3.07972647875828));
#71658=CARTESIAN_POINT('Ctrl Pts',(28.2748281729558,1.04479394950559,-3.05032512843697));
#71659=CARTESIAN_POINT('Ctrl Pts',(28.2809810371022,1.13887204421094,-3.01646687654044));
#71660=CARTESIAN_POINT('Ctrl Pts',(28.2871339012485,1.23121451807512,-2.97829286219154));
#71661=CARTESIAN_POINT('Ctrl Pts',(28.293284434385,1.32352200803526,-2.94013331005053));
#71662=CARTESIAN_POINT('Ctrl Pts',(28.2994349675215,1.41409478270028,-2.89766141000608));
#71663=CARTESIAN_POINT('Ctrl Pts',(28.3055855006581,1.50250920456033,-2.851067107718));
#71664=CARTESIAN_POINT('Ctrl Pts',(28.3117353488733,1.59091378061973,-2.80447799415595));
#71665=CARTESIAN_POINT('Ctrl Pts',(28.3178851970885,1.67716009745321,-2.75376759356169));
#71666=CARTESIAN_POINT('Ctrl Pts',(28.3240350453037,1.76084839382784,-2.69917218725555));
#71667=CARTESIAN_POINT('Ctrl Pts',(28.3301858536828,1.8445497562946,-2.64456825707403));
#71668=CARTESIAN_POINT('Ctrl Pts',(28.336336662062,1.92569194119349,-2.58607835375549));
#71669=CARTESIAN_POINT('Ctrl Pts',(28.3424874704411,2.00390434310439,-2.523981962334));
#71670=CARTESIAN_POINT('Ctrl Pts',(28.3486448568073,2.08220038933238,-2.46181916187599));
#71671=CARTESIAN_POINT('Ctrl Pts',(28.3548022431735,2.15756005492245,-2.39604244198193));
#71672=CARTESIAN_POINT('Ctrl Pts',(28.3609596295397,2.22964611159373,-2.32697137488947));
#71673=CARTESIAN_POINT('Ctrl Pts',(28.3671204522766,2.30177239871393,-2.25786175998117));
#71674=CARTESIAN_POINT('Ctrl Pts',(28.3732812750136,2.37062113921173,-2.18545445124638));
#71675=CARTESIAN_POINT('Ctrl Pts',(28.3794420977505,2.43589371227412,-2.11010411710025));
#71676=CARTESIAN_POINT('Ctrl Pts',(28.3856132206672,2.5012754134941,-2.03462780595101));
#71677=CARTESIAN_POINT('Ctrl Pts',(28.3917843435839,2.56306873558721,-1.95619898240512));
#71678=CARTESIAN_POINT('Ctrl Pts',(28.3979554665006,2.62101682199957,-1.87520355729592));
#71679=CARTESIAN_POINT('Ctrl Pts',(28.4026509884462,2.66510871826058,-1.81357526026954));
#71680=CARTESIAN_POINT('Ctrl Pts',(28.4073465103919,2.70697529019553,-1.75046168185185));
#71681=CARTESIAN_POINT('Ctrl Pts',(28.4120420323375,2.74652130950348,-1.68604218777091));
#71682=CARTESIAN_POINT('Ctrl Pts',(28.4182142804302,2.79850442130151,-1.60136297551682));
#71683=CARTESIAN_POINT('Ctrl Pts',(28.424386528523,2.84665918645213,-1.51412839474084));
#71684=CARTESIAN_POINT('Ctrl Pts',(28.4305587766158,2.8907251466144,-1.42471951247646));
#71685=CARTESIAN_POINT('Ctrl Pts',(28.4367226652684,2.9347314256441,-1.33543172194218));
#71686=CARTESIAN_POINT('Ctrl Pts',(28.442886553921,2.97465971615513,-1.24397586919675));
#71687=CARTESIAN_POINT('Ctrl Pts',(28.4490504425736,3.01029354843852,-1.15076075477461));
#71688=CARTESIAN_POINT('Ctrl Pts',(28.4552078042322,3.04588964775434,-1.05764434662862));
#71689=CARTESIAN_POINT('Ctrl Pts',(28.4613651658908,3.07720017533033,-0.962772783923574));
#71690=CARTESIAN_POINT('Ctrl Pts',(28.4675225275494,3.1040556333647,-0.866577283037629));
#71691=CARTESIAN_POINT('Ctrl Pts',(28.4736753916957,3.13089147540787,-0.770452046084509));
#71692=CARTESIAN_POINT('Ctrl Pts',(28.479828255842,3.15327860118733,-0.673005210711577));
#71693=CARTESIAN_POINT('Ctrl Pts',(28.4859811199883,3.17109680116036,-0.574684818113822));
#71694=CARTESIAN_POINT('Ctrl Pts',(28.4921316531248,3.18890825071646,-0.476401674151972));
#71695=CARTESIAN_POINT('Ctrl Pts',(28.4982821862613,3.20215413645317,-0.377246057493469));
#71696=CARTESIAN_POINT('Ctrl Pts',(28.5044327193979,3.21076517721345,-0.277677041351127));
#71697=CARTESIAN_POINT('Ctrl Pts',(28.5105825676131,3.21937525905109,-0.178119113181222));
#71698=CARTESIAN_POINT('Ctrl Pts',(28.5167324158283,3.22335148463723,-0.0781483098141737));
#71699=CARTESIAN_POINT('Ctrl Pts',(28.5228822640435,3.22267646093287,0.0217713263081345));
#71700=CARTESIAN_POINT('Ctrl Pts',(28.5290330724226,3.22200133183836,0.1217065626904));
#71701=CARTESIAN_POINT('Ctrl Pts',(28.5351838808018,3.216673513986,0.22159018155417));
#71702=CARTESIAN_POINT('Ctrl Pts',(28.5413346891809,3.20672772253247,0.320959305896789));
#71703=CARTESIAN_POINT('Ctrl Pts',(28.5474920755471,3.19677129454414,0.420434700630556));
#71704=CARTESIAN_POINT('Ctrl Pts',(28.5536494619133,3.18218707423412,0.519394069039138));
#71705=CARTESIAN_POINT('Ctrl Pts',(28.5598068482795,3.163061545833,0.617380935705489));
#71706=CARTESIAN_POINT('Ctrl Pts',(28.5659676710165,3.1439253436812,0.715422487783006));
#71707=CARTESIAN_POINT('Ctrl Pts',(28.5721284937534,3.12024288906826,0.812490035242985));
#71708=CARTESIAN_POINT('Ctrl Pts',(28.5782893164904,3.09215106489531,0.908140602752004));
#71709=CARTESIAN_POINT('Ctrl Pts',(28.5844604394071,3.06401227445665,1.00395108689522));
#71710=CARTESIAN_POINT('Ctrl Pts',(28.5906315623237,3.03144953093479,1.09833944821386));
#71711=CARTESIAN_POINT('Ctrl Pts',(28.5968026852404,2.9946485809941,1.19088095074614));
#71712=CARTESIAN_POINT('Ctrl Pts',(28.601498207186,2.96664724794732,1.26129449814728));
#71713=CARTESIAN_POINT('Ctrl Pts',(28.6061937291315,2.93619322730563,1.33063918974492));
#71714=CARTESIAN_POINT('Ctrl Pts',(28.610889251077,2.90338591220099,1.39873793375773));
#71715=CARTESIAN_POINT('Ctrl Pts',(28.6170612315427,2.86026267471918,1.48824962652837));
#71716=CARTESIAN_POINT('Ctrl Pts',(28.6232332120084,2.81292017849583,1.57592275347687));
#71717=CARTESIAN_POINT('Ctrl Pts',(28.6294051924741,2.76153812358604,1.66133222279016));
#71718=CARTESIAN_POINT('Ctrl Pts',(28.6355691632302,2.71022274992083,1.74663085166076));
#71719=CARTESIAN_POINT('Ctrl Pts',(28.6417331339863,2.65487845658288,1.82967129146932));
#71720=CARTESIAN_POINT('Ctrl Pts',(28.6478971047424,2.59573209018716,1.91005038637011));
#71721=CARTESIAN_POINT('Ctrl Pts',(28.6540538745981,2.53665482001392,1.99033558045903));
#71722=CARTESIAN_POINT('Ctrl Pts',(28.6602106444537,2.47378456805033,2.06796526619833));
#71723=CARTESIAN_POINT('Ctrl Pts',(28.6663674143094,2.40739234662908,2.14256380345877));
#71724=CARTESIAN_POINT('Ctrl Pts',(28.6725199514532,2.34104576913317,2.21711105504159));
#71725=CARTESIAN_POINT('Ctrl Pts',(28.678672488597,2.2711823221187,2.28863097628703));
#71726=CARTESIAN_POINT('Ctrl Pts',(28.6848250257408,2.19811384756102,2.35678023490959));
#71727=CARTESIAN_POINT('Ctrl Pts',(28.6909756411917,2.12506819532269,2.42490820768825));
#71728=CARTESIAN_POINT('Ctrl Pts',(28.6971262566426,2.04881981890187,2.48966731064813));
#71729=CARTESIAN_POINT('Ctrl Pts',(28.7032768720936,1.96971744171717,2.55075101926769));
#71730=CARTESIAN_POINT('Ctrl Pts',(28.7078317970348,1.91113706165191,2.59598742042381));
#71731=CARTESIAN_POINT('Ctrl Pts',(28.712386721976,1.85099224515406,2.63920884383267));
#71732=CARTESIAN_POINT('Ctrl Pts',(28.7169416469173,1.789436210378,2.68030513402635));
#71733=CARTESIAN_POINT('Ctrl Pts',(27.4670789411481,1.78943621037803,2.68030513402633));
#71734=CARTESIAN_POINT('Ctrl Pts',(27.4733112001578,1.70540893037057,2.73640376831841));
#71735=CARTESIAN_POINT('Ctrl Pts',(27.4795434591674,1.61866637486224,2.78859711560752));
#71736=CARTESIAN_POINT('Ctrl Pts',(27.485775718177,1.52961023515413,2.83661948294299));
#71737=CARTESIAN_POINT('Ctrl Pts',(27.4919268250731,1.44171372214755,2.88401653663231));
#71738=CARTESIAN_POINT('Ctrl Pts',(27.4980779319692,1.35156391773072,2.92735038660131));
#71739=CARTESIAN_POINT('Ctrl Pts',(27.5042290388653,1.25957439429802,2.96641027299475));
#71740=CARTESIAN_POINT('Ctrl Pts',(27.5103789285969,1.16760307350456,3.00546243032303));
#71741=CARTESIAN_POINT('Ctrl Pts',(27.5165288183286,1.07379315695264,3.04024213522712));
#71742=CARTESIAN_POINT('Ctrl Pts',(27.5226787080602,0.978579412407021,3.07058624632384));
#71743=CARTESIAN_POINT('Ctrl Pts',(27.5288290258927,0.883359039924092,3.10093246970873));
#71744=CARTESIAN_POINT('Ctrl Pts',(27.5349793437251,0.786735059401567,3.12684235444456));
#71745=CARTESIAN_POINT('Ctrl Pts',(27.5411296615576,0.689157689316571,3.14820254141246));
#71746=CARTESIAN_POINT('Ctrl Pts',(27.5474232862094,0.589306696481606,3.17006043606597));
#71747=CARTESIAN_POINT('Ctrl Pts',(27.5537169108612,0.488457794806372,3.18715385470366));
#71748=CARTESIAN_POINT('Ctrl Pts',(27.5600105355129,0.387103143988446,3.19941693413257));
#71749=CARTESIAN_POINT('Ctrl Pts',(27.5661701684073,0.287906341554656,3.21141893164845));
#71750=CARTESIAN_POINT('Ctrl Pts',(27.5723298013017,0.188225555102932,3.21879425826122));
#71751=CARTESIAN_POINT('Ctrl Pts',(27.578489434196,0.0885246612456093,3.22153394314748));
#71752=CARTESIAN_POINT('Ctrl Pts',(27.5848500547265,-0.0144294535940865,
3.22436302342441));
#71753=CARTESIAN_POINT('Ctrl Pts',(27.591210675257,-0.117404501863241,3.22224875637744));
#71754=CARTESIAN_POINT('Ctrl Pts',(27.5975712957875,-0.219894358238718,
3.21523934314613));
#71755=CARTESIAN_POINT('Ctrl Pts',(27.603931916318,-0.322384214614165,3.20822992991483));
#71756=CARTESIAN_POINT('Ctrl Pts',(27.6102925368484,-0.424388388104331,
3.19632549798911));
#71757=CARTESIAN_POINT('Ctrl Pts',(27.6166531573789,-0.525412906889123,
3.17963187173835));
#71758=CARTESIAN_POINT('Ctrl Pts',(27.6228254054717,-0.623445542290536,
3.16343263421212));
#71759=CARTESIAN_POINT('Ctrl Pts',(27.6289976535645,-0.72090085505774,3.14266690515393));
#71760=CARTESIAN_POINT('Ctrl Pts',(27.6351699016572,-0.817320307424585,
3.11738754048504));
#71761=CARTESIAN_POINT('Ctrl Pts',(27.6413337903099,-0.913609173232671,
3.09214241315269));
#71762=CARTESIAN_POINT('Ctrl Pts',(27.6474976789625,-1.00886455063752,3.0623959098273));
#71763=CARTESIAN_POINT('Ctrl Pts',(27.6536615676151,-1.10263576568776,3.0282522898078));
#71764=CARTESIAN_POINT('Ctrl Pts',(27.6598189292737,-1.19630768560157,2.99414482475766));
#71765=CARTESIAN_POINT('Ctrl Pts',(27.6659762909323,-1.28849816172489,2.95564964766606));
#71766=CARTESIAN_POINT('Ctrl Pts',(27.6721336525908,-1.37877035596248,2.9129211915222));
#71767=CARTESIAN_POINT('Ctrl Pts',(27.6782865167371,-1.46897661281919,2.87022394545926));
#71768=CARTESIAN_POINT('Ctrl Pts',(27.6844393808835,-1.55726698211956,2.82329975325878));
#71769=CARTESIAN_POINT('Ctrl Pts',(27.6905922450298,-1.64322420329754,2.77235130894285));
#71770=CARTESIAN_POINT('Ctrl Pts',(27.6967427781663,-1.72914885962163,2.72142216642173));
#71771=CARTESIAN_POINT('Ctrl Pts',(27.7028933113028,-1.812741750898,2.66647202236397));
#71772=CARTESIAN_POINT('Ctrl Pts',(27.7090438444394,-1.89361064520634,2.60774927607338));
#71773=CARTESIAN_POINT('Ctrl Pts',(27.7151936926546,-1.97447053398155,2.54903306912825));
#71774=CARTESIAN_POINT('Ctrl Pts',(27.7213435408698,-2.05260667739641,2.4865453504305));
#71775=CARTESIAN_POINT('Ctrl Pts',(27.727493389085,-2.12765708154595,2.42057697788097));
#71776=CARTESIAN_POINT('Ctrl Pts',(27.7336441974642,-2.20271920317026,2.35459830581674));
#71777=CARTESIAN_POINT('Ctrl Pts',(27.7397950058433,-2.27469430232273,2.28513818731402));
#71778=CARTESIAN_POINT('Ctrl Pts',(27.7459458142225,-2.34325540223546,2.21252608626302));
#71779=CARTESIAN_POINT('Ctrl Pts',(27.7521032005887,-2.41188982487238,2.13983633014136));
#71780=CARTESIAN_POINT('Ctrl Pts',(27.7582605869548,-2.47710265859685,2.06398817660085));
#71781=CARTESIAN_POINT('Ctrl Pts',(27.764417973321,-2.53860567769926,1.98534600905058));
#71782=CARTESIAN_POINT('Ctrl Pts',(27.770578796058,-2.60014302097202,1.90665995215642));
#71783=CARTESIAN_POINT('Ctrl Pts',(27.776739618795,-2.65796617504315,1.82517713016482));
#71784=CARTESIAN_POINT('Ctrl Pts',(27.782900441532,-2.71183013064817,1.74129116032004));
#71785=CARTESIAN_POINT('Ctrl Pts',(27.7890715644487,-2.76578414052778,1.65726494288153));
#71786=CARTESIAN_POINT('Ctrl Pts',(27.7952426873654,-2.81576551251435,1.57082792840027));
#71787=CARTESIAN_POINT('Ctrl Pts',(27.801413810282,-2.86157502894539,1.48239870352621));
#71788=CARTESIAN_POINT('Ctrl Pts',(27.8061093322275,-2.89643085544834,1.41511413123345));
#71789=CARTESIAN_POINT('Ctrl Pts',(27.8108048541729,-2.92887234514541,1.34667668993071));
#71790=CARTESIAN_POINT('Ctrl Pts',(27.8155003761184,-2.95883081273827,1.2772774890722));
#71791=CARTESIAN_POINT('Ctrl Pts',(27.8223228167748,-3.00235949169766,1.1764427075586));
#71792=CARTESIAN_POINT('Ctrl Pts',(27.8291452574313,-3.04077590270347,1.07327399786143));
#71793=CARTESIAN_POINT('Ctrl Pts',(27.8359676980877,-3.07384959702334,0.968280030455798));
#71794=CARTESIAN_POINT('Ctrl Pts',(27.8427712225131,-3.10683158960843,0.863577174434908));
#71795=CARTESIAN_POINT('Ctrl Pts',(27.8495747469385,-3.13450030393611,0.75705940657642));
#71796=CARTESIAN_POINT('Ctrl Pts',(27.8563782713639,-3.15667327320979,0.649254502258558));
#71797=CARTESIAN_POINT('Ctrl Pts',(27.8631479113503,-3.17873581168638,0.541986512116085));
#71798=CARTESIAN_POINT('Ctrl Pts',(27.8699175513366,-3.19535709541191,0.433444429808308));
#71799=CARTESIAN_POINT('Ctrl Pts',(27.876687191323,-3.2064049839161,0.324167613462539));
#71800=CARTESIAN_POINT('Ctrl Pts',(27.8833159439616,-3.21722294768089,0.217165027483141));
#71801=CARTESIAN_POINT('Ctrl Pts',(27.8899446966002,-3.22269711590572,0.109458259196475));
#71802=CARTESIAN_POINT('Ctrl Pts',(27.8965734492388,-3.22274961841222,0.00156828692453539));
#71803=CARTESIAN_POINT('Ctrl Pts',(27.2231721927303,1.78943620958681,2.68030513455457));
#71804=CARTESIAN_POINT('Ctrl Pts',(27.2238480330952,1.78076083047407,2.68609702642393));
#71805=CARTESIAN_POINT('Ctrl Pts',(27.2245218578103,1.77205702048223,2.69184700624272));
#71806=CARTESIAN_POINT('Ctrl Pts',(27.22740730015,1.73454512105204,2.71636760973045));
#71807=CARTESIAN_POINT('Ctrl Pts',(27.2295972711144,1.70546450763826,2.73471951247519));
#71808=CARTESIAN_POINT('Ctrl Pts',(27.2322638556065,1.66922264459362,2.75678763313491));
#71809=CARTESIAN_POINT('Ctrl Pts',(27.2327678639155,1.66233518012192,2.76094622251951));
#71810=CARTESIAN_POINT('Ctrl Pts',(27.233558344089,1.65147266073824,2.76744953160831));
#71811=CARTESIAN_POINT('Ctrl Pts',(27.2338459315801,1.64750807689072,2.76981154528296));
#71812=CARTESIAN_POINT('Ctrl Pts',(27.234383295355,1.64007615292079,2.77421772320716));
#71813=CARTESIAN_POINT('Ctrl Pts',(27.2346331988297,1.63661009499939,2.77626388520872));
#71814=CARTESIAN_POINT('Ctrl Pts',(27.2352000132547,1.62872643314744,2.78089805290653));
#71815=CARTESIAN_POINT('Ctrl Pts',(27.2355166593318,1.6243065008625,2.78348202200232));
#71816=CARTESIAN_POINT('Ctrl Pts',(27.2364555620696,1.61115451809709,2.79112890457759));
#71817=CARTESIAN_POINT('Ctrl Pts',(27.2370758730568,1.60240472039727,2.79616139762017));
#71818=CARTESIAN_POINT('Ctrl Pts',(27.2414890166815,1.53973536954442,2.83181523239541));
#71819=CARTESIAN_POINT('Ctrl Pts',(27.245189423963,1.48496149192908,2.86091822272689));
#71820=CARTESIAN_POINT('Ctrl Pts',(27.2671600285214,1.14899766528563,3.02717467850755));
#71821=CARTESIAN_POINT('Ctrl Pts',(27.2838631665485,0.849890696075904,3.12437374701242));
#71822=CARTESIAN_POINT('Ctrl Pts',(27.3062590786234,0.466471820723136,3.18971854825837));
#71823=CARTESIAN_POINT('Ctrl Pts',(27.3106980235768,0.391083682982989,3.19983635496571));
#71824=CARTESIAN_POINT('Ctrl Pts',(27.3179339237413,0.269923907952096,3.21175151972092));
#71825=CARTESIAN_POINT('Ctrl Pts',(27.3206785407704,0.224347663239141,3.2152565288252));
#71826=CARTESIAN_POINT('Ctrl Pts',(27.3242437698862,0.165721903624434,3.21851256445583));
#71827=CARTESIAN_POINT('Ctrl Pts',(27.3250362924795,0.15272574021701,3.21915543542226));
#71828=CARTESIAN_POINT('Ctrl Pts',(27.3263183139507,0.131762377175069,3.22006518259725));
#71829=CARTESIAN_POINT('Ctrl Pts',(27.3268062654648,0.123797369539631,3.22038123732308));
#71830=CARTESIAN_POINT('Ctrl Pts',(27.3277385889466,0.108605666226845,3.22092760699104));
#71831=CARTESIAN_POINT('Ctrl Pts',(27.3281827935099,0.101379198276591,3.22116315901778));
#71832=CARTESIAN_POINT('Ctrl Pts',(27.3291995659685,0.0848649106216545,
3.22164582690221));
#71833=CARTESIAN_POINT('Ctrl Pts',(27.3297726278733,0.0755767243877204,
3.22187709928331));
#71834=CARTESIAN_POINT('Ctrl Pts',(27.3315356593533,0.0470621070573929,
3.22246373170955));
#71835=CARTESIAN_POINT('Ctrl Pts',(27.3327297552293,0.0278336591630101,
3.22268717155366));
#71836=CARTESIAN_POINT('Ctrl Pts',(27.349879662908,-0.247089536006223,3.22342121487121));
#71837=CARTESIAN_POINT('Ctrl Pts',(27.3668397170065,-0.501901568342063,
3.19367174408501));
#71838=CARTESIAN_POINT('Ctrl Pts',(27.398244351387,-0.953525121665733,3.08553146246579));
#71839=CARTESIAN_POINT('Ctrl Pts',(27.4124741627459,-1.15139496122458,3.01728671391873));
#71840=CARTESIAN_POINT('Ctrl Pts',(27.4275251235296,-1.36523747769293,2.91940716620469));
#71841=CARTESIAN_POINT('Ctrl Pts',(27.4291962726676,-1.38905712083657,2.90814923866551));
#71842=CARTESIAN_POINT('Ctrl Pts',(27.4313118537463,-1.41934547446522,2.89337692810322));
#71843=CARTESIAN_POINT('Ctrl Pts',(27.4317721047328,-1.42594304663215,2.89013114827778));
#71844=CARTESIAN_POINT('Ctrl Pts',(27.4325093204974,-1.43652512686493,2.88488007000728));
#71845=CARTESIAN_POINT('Ctrl Pts',(27.432787165695,-1.44051663297238,2.88288905252125));
#71846=CARTESIAN_POINT('Ctrl Pts',(27.4333167756684,-1.4481315260626,2.8790708766506));
#71847=CARTESIAN_POINT('Ctrl Pts',(27.4335686259894,-1.45175558478329,2.87724516712595));
#71848=CARTESIAN_POINT('Ctrl Pts',(27.434148472238,-1.46010583246841,2.87301872957268));
#71849=CARTESIAN_POINT('Ctrl Pts',(27.4344761634438,-1.46482958273714,2.8706131674218));
#71850=CARTESIAN_POINT('Ctrl Pts',(27.4353534844092,-1.47748828929879,2.86412735895395));
#71851=CARTESIAN_POINT('Ctrl Pts',(27.435901793436,-1.48541234092871,2.86002576126802));
#71852=CARTESIAN_POINT('Ctrl Pts',(27.4398563809841,-1.54264407668412,2.83009981109492));
#71853=CARTESIAN_POINT('Ctrl Pts',(27.4431880062344,-1.59129588585395,2.80303299529659));
#71854=CARTESIAN_POINT('Ctrl Pts',(27.447029180231,-1.64748836798729,2.76983605017949));
#71855=CARTESIAN_POINT('Ctrl Pts',(27.4475923480799,-1.65572952867481,2.76491761161707));
#71856=CARTESIAN_POINT('Ctrl Pts',(27.4589487261483,-1.82192944646596,2.66471764704984));
#71857=CARTESIAN_POINT('Ctrl Pts',(27.469161911215,-1.97145487287852,2.55607605126568));
#71858=CARTESIAN_POINT('Ctrl Pts',(27.4926815127812,-2.28924954169539,2.28060942763938));
#71859=CARTESIAN_POINT('Ctrl Pts',(27.5060231318166,-2.45007108750799,2.10688688602693));
#71860=CARTESIAN_POINT('Ctrl Pts',(27.5214564907231,-2.60207726935541,1.90149728140294));
#71861=CARTESIAN_POINT('Ctrl Pts',(27.5226400132841,-2.61353807531062,1.88571385154051));
#71862=CARTESIAN_POINT('Ctrl Pts',(27.5243987795243,-2.63027668331909,1.86221627693074));
#71863=CARTESIAN_POINT('Ctrl Pts',(27.5249697429993,-2.63566548231103,1.85458145017496));
#71864=CARTESIAN_POINT('Ctrl Pts',(27.5259851558146,-2.64516853006042,1.84099250066742));
#71865=CARTESIAN_POINT('Ctrl Pts',(27.5264290916484,-2.64929608922764,1.83504772967395));
#71866=CARTESIAN_POINT('Ctrl Pts',(27.5273014392519,-2.65735348543378,1.82335911194502));
#71867=CARTESIAN_POINT('Ctrl Pts',(27.5277297909691,-2.66128481199732,1.81761633627087));
#71868=CARTESIAN_POINT('Ctrl Pts',(27.5288946584354,-2.67190738908606,1.80199081800324));
#71869=CARTESIAN_POINT('Ctrl Pts',(27.529632543403,-2.67856234294779,1.79208364001474));
#71870=CARTESIAN_POINT('Ctrl Pts',(27.5324191975941,-2.7034159547631,1.75463653631705));
#71871=CARTESIAN_POINT('Ctrl Pts',(27.5344817311047,-2.72124565583472,1.72685527734292));
#71872=CARTESIAN_POINT('Ctrl Pts',(27.5535912642751,-2.88122298447622,1.46895582221554));
#71873=CARTESIAN_POINT('Ctrl Pts',(27.5717481779801,-2.99427029064344,1.22211448809788));
#71874=CARTESIAN_POINT('Ctrl Pts',(27.5983540607978,-3.11187394531926,0.847008138719422));
#71875=CARTESIAN_POINT('Ctrl Pts',(27.6066463246093,-3.14187405204064,0.727882507468044));
#71876=CARTESIAN_POINT('Ctrl Pts',(27.6179660007046,-3.17427470461006,0.559031598303127));
#71877=CARTESIAN_POINT('Ctrl Pts',(27.6211681570472,-3.18243645823766,0.510524205878982));
#71878=CARTESIAN_POINT('Ctrl Pts',(27.6261112276352,-3.19349129038588,0.434180159233793));
#71879=CARTESIAN_POINT('Ctrl Pts',(27.6278860510557,-3.19713746042052,0.406461828944376));
#71880=CARTESIAN_POINT('Ctrl Pts',(27.6301129859493,-3.20130477556738,0.37124338753867));
#71881=CARTESIAN_POINT('Ctrl Pts',(27.6305829885249,-3.20216087635693,0.363785161144907));
#71882=CARTESIAN_POINT('Ctrl Pts',(27.6313320858415,-3.203487910875,0.351856465842583));
#71883=CARTESIAN_POINT('Ctrl Pts',(27.631612111472,-3.2039755596557,0.34738794077672));
#71884=CARTESIAN_POINT('Ctrl Pts',(27.6321433158255,-3.2048846216203,0.338893070528992));
#71885=CARTESIAN_POINT('Ctrl Pts',(27.6323945879422,-3.205307792317,0.334867000195016));
#71886=CARTESIAN_POINT('Ctrl Pts',(27.6329697404343,-3.20626068533308,0.325633803812677));
#71887=CARTESIAN_POINT('Ctrl Pts',(27.6332933301567,-3.2067853090427,0.320426183581449));
#71888=CARTESIAN_POINT('Ctrl Pts',(27.634313777896,-3.2084032253391,0.303964082469341));
#71889=CARTESIAN_POINT('Ctrl Pts',(27.6350080581697,-3.2094499892626,0.292704962507583));
#71890=CARTESIAN_POINT('Ctrl Pts',(27.6413990189643,-3.21858085674732,0.188547626912244));
#71891=CARTESIAN_POINT('Ctrl Pts',(27.6468851710463,-3.22268952531855,0.0953351988905227));
#71892=CARTESIAN_POINT('Ctrl Pts',(27.6614374253509,-3.22285155288648,-0.157324226192558));
#71893=CARTESIAN_POINT('Ctrl Pts',(27.6702712317488,-3.21112892640575,-0.316512004701471));
#71894=CARTESIAN_POINT('Ctrl Pts',(27.6920848388944,-3.15375973317529,-0.702171279841489));
#71895=CARTESIAN_POINT('Ctrl Pts',(27.7051346273545,-3.0954924411043,-0.925824020369713));
#71896=CARTESIAN_POINT('Ctrl Pts',(27.7201256606333,-3.00757630179329,-1.15798062649805));
#71897=CARTESIAN_POINT('Ctrl Pts',(27.7212049559113,-3.0011353571452,-1.17457264181912));
#71898=CARTESIAN_POINT('Ctrl Pts',(27.7228449659654,-2.99118250973019,-1.19959498895647));
#71899=CARTESIAN_POINT('Ctrl Pts',(27.7234022787466,-2.98777159617318,-1.20806532540585));
#71900=CARTESIAN_POINT('Ctrl Pts',(27.7243740458556,-2.98177455170537,-1.22277705543178));
#71901=CARTESIAN_POINT('Ctrl Pts',(27.7247879471271,-2.97920469554067,-1.22902505485243));
#71902=CARTESIAN_POINT('Ctrl Pts',(27.7256534149903,-2.97379883315036,-1.24205155017328));
#71903=CARTESIAN_POINT('Ctrl Pts',(27.7261051010829,-2.97095925530326,-1.24882851314205));
#71904=CARTESIAN_POINT('Ctrl Pts',(27.7271764921108,-2.96418083222222,-1.26485199485873));
#71905=CARTESIAN_POINT('Ctrl Pts',(27.7277968802615,-2.96022187711769,-1.27408987499967));
#71906=CARTESIAN_POINT('Ctrl Pts',(27.7298620859044,-2.94693118832376,-1.30470619378309));
#71907=CARTESIAN_POINT('Ctrl Pts',(27.7313133512209,-2.93741073377235,-1.32600143883758));
#71908=CARTESIAN_POINT('Ctrl Pts',(27.7472500448558,-2.83092148646036,-1.55741949420045));
#71909=CARTESIAN_POINT('Ctrl Pts',(27.7625399367467,-2.71184042812416,-1.75657449958189));
#71910=CARTESIAN_POINT('Ctrl Pts',(27.7881359425568,-2.48346646917698,-2.05921291587329));
#71911=CARTESIAN_POINT('Ctrl Pts',(27.7981991066249,-2.3864243556292,-2.17093160042393));
#71912=CARTESIAN_POINT('Ctrl Pts',(27.8145905366298,-2.21254224802675,-2.34530723003864));
#71913=CARTESIAN_POINT('Ctrl Pts',(27.821032681864,-2.13986338382035,-2.41180391202702));
#71914=CARTESIAN_POINT('Ctrl Pts',(27.8279689574275,-2.0554677621893,-2.4821967121598));
#71915=CARTESIAN_POINT('Ctrl Pts',(27.828687324874,-2.04665009979174,-2.48947215640897));
#71916=CARTESIAN_POINT('Ctrl Pts',(27.8297312106478,-2.03372089361142,-2.50002490552392));
#71917=CARTESIAN_POINT('Ctrl Pts',(27.8300593444938,-2.0296398674067,-2.50333921211656));
#71918=CARTESIAN_POINT('Ctrl Pts',(27.8306390725323,-2.02239945024623,-2.50918999699666));
#71919=CARTESIAN_POINT('Ctrl Pts',(27.8308909586197,-2.01924336668597,-2.51173051982105));
#71920=CARTESIAN_POINT('Ctrl Pts',(27.8314206151855,-2.01258524567719,-2.51706938436435));
#71921=CARTESIAN_POINT('Ctrl Pts',(27.8316982880087,-2.0090821678938,-2.51986636551565));
#71922=CARTESIAN_POINT('Ctrl Pts',(27.8324361633962,-1.99974019449305,-2.52729346278987));
#71923=CARTESIAN_POINT('Ctrl Pts',(27.8328954460419,-1.9938910136549,-2.53191068578585));
#71924=CARTESIAN_POINT('Ctrl Pts',(27.8350349794586,-1.96648548843877,-2.55339017614526));
#71925=CARTESIAN_POINT('Ctrl Pts',(27.8366977922625,-1.94473015369002,-2.56999831011822));
#71926=CARTESIAN_POINT('Ctrl Pts',(27.8412170756525,-1.88444173658231,-2.61481879096467));
#71927=CARTESIAN_POINT('Ctrl Pts',(27.8440396845546,-1.84548780824245,-2.64245590499762));
#71928=CARTESIAN_POINT('Ctrl Pts',(27.8536955548271,-1.70838546890498,-2.73521620288345));
#71929=CARTESIAN_POINT('Ctrl Pts',(27.8603364431917,-1.60728737931182,-2.79582183036316));
#71930=CARTESIAN_POINT('Ctrl Pts',(27.8825148958391,-1.25706519991061,-2.98048002034257));
#71931=CARTESIAN_POINT('Ctrl Pts',(27.8978766973831,-0.995314585336189,
-3.07779234881496));
#71932=CARTESIAN_POINT('Ctrl Pts',(27.9149917990916,-0.716709782021276,
-3.14205439352657));
#71933=CARTESIAN_POINT('Ctrl Pts',(27.9154607824233,-0.709082995238445,
-3.14378434816814));
#71934=CARTESIAN_POINT('Ctrl Pts',(27.9175394978057,-0.675312720949102,
-3.15131518959347));
#71935=CARTESIAN_POINT('Ctrl Pts',(27.9191583856158,-0.649104398494685,
-3.15681771866805));
#71936=CARTESIAN_POINT('Ctrl Pts',(27.9214536904776,-0.612092166582058,
-3.1641081748379));
#71937=CARTESIAN_POINT('Ctrl Pts',(27.9221213924775,-0.601342596038615,
-3.16616873208228));
#71938=CARTESIAN_POINT('Ctrl Pts',(27.9232048813275,-0.583928199338438,
-3.16941496866566));
#71939=CARTESIAN_POINT('Ctrl Pts',(27.9236195856776,-0.577269707025343,
-3.17063449010249));
#71940=CARTESIAN_POINT('Ctrl Pts',(27.9244852047861,-0.563385926521309,
-3.17313215902541));
#71941=CARTESIAN_POINT('Ctrl Pts',(27.9249362341709,-0.556160023551465,
-3.17440662606845));
#71942=CARTESIAN_POINT('Ctrl Pts',(27.9260033142691,-0.5390842589185,-3.17735826700009));
#71943=CARTESIAN_POINT('Ctrl Pts',(27.9266200332169,-0.529230868168161,
-3.17901432517391));
#71944=CARTESIAN_POINT('Ctrl Pts',(27.9286606983437,-0.496679598192446,
-3.18432968187484));
#71945=CARTESIAN_POINT('Ctrl Pts',(27.9300908836919,-0.473950663811787,
-3.18779184863668));
#71946=CARTESIAN_POINT('Ctrl Pts',(27.9334734704151,-0.420401360956075,
-3.19536335451879));
#71947=CARTESIAN_POINT('Ctrl Pts',(27.9354321160453,-0.389555150379547,
-3.199270377393));
#71948=CARTESIAN_POINT('Ctrl Pts',(27.9424401598065,-0.279778423930402,
-3.21156373514226));
#71949=CARTESIAN_POINT('Ctrl Pts',(27.9475641468296,-0.200605221789714,
-3.21747936065744));
#71950=CARTESIAN_POINT('Ctrl Pts',(27.9746704427703,0.212784087038432,-3.23304974306907));
#71951=CARTESIAN_POINT('Ctrl Pts',(27.9980372784334,0.546731491541803,-3.19357592075675));
#71952=CARTESIAN_POINT('Ctrl Pts',(28.0220809468677,0.905253442884408,-3.09323153453452));
#71953=CARTESIAN_POINT('Ctrl Pts',(28.0245098501895,0.941709773456022,-3.08232836208689));
#71954=CARTESIAN_POINT('Ctrl Pts',(28.027400672289,0.985496463149671,-3.06838340786059));
#71955=CARTESIAN_POINT('Ctrl Pts',(28.0278962864641,0.993017840449468,-3.06595753202135));
#71956=CARTESIAN_POINT('Ctrl Pts',(28.0287060114665,1.00533115511809,-3.0619360440072));
#71957=CARTESIAN_POINT('Ctrl Pts',(28.0290210638473,1.01012834630088,-3.06035680826154));
#71958=CARTESIAN_POINT('Ctrl Pts',(28.0295856348363,1.0187365150749,-3.05750055260106));
#71959=CARTESIAN_POINT('Ctrl Pts',(28.0298353950201,1.02254881632375,-3.05622768051081));
#71960=CARTESIAN_POINT('Ctrl Pts',(28.0303740279289,1.03077943452877,-3.05346247196442));
#71961=CARTESIAN_POINT('Ctrl Pts',(28.0306627521813,1.0351968799202,-3.05196768180817));
#71962=CARTESIAN_POINT('Ctrl Pts',(28.0314616691937,1.04743507700694,-3.04779685125671));
#71963=CARTESIAN_POINT('Ctrl Pts',(28.0319706565559,1.05524886906468,-3.04510027994782));
#71964=CARTESIAN_POINT('Ctrl Pts',(28.0347762105434,1.09840549316296,-3.03002068949016));
#71965=CARTESIAN_POINT('Ctrl Pts',(28.0370394213258,1.13354250914406,-3.01705181828206));
#71966=CARTESIAN_POINT('Ctrl Pts',(28.0542719861256,1.40270933883836,-2.91233728714002));
#71967=CARTESIAN_POINT('Ctrl Pts',(28.0679738256536,1.62553600585687,-2.79409542300904));
#71968=CARTESIAN_POINT('Ctrl Pts',(28.0932840146536,1.99619110573798,-2.53791149606969));
#71969=CARTESIAN_POINT('Ctrl Pts',(28.1046757140041,2.14913753103029,-2.40976449089171));
#71970=CARTESIAN_POINT('Ctrl Pts',(28.1177812751899,2.30190864736685,-2.25558340020309));
#71971=CARTESIAN_POINT('Ctrl Pts',(28.1188698921541,2.31443835301224,-2.24272490199992));
#71972=CARTESIAN_POINT('Ctrl Pts',(28.1205216959687,2.3332050901733,-2.22314094891634));
#71973=CARTESIAN_POINT('Ctrl Pts',(28.1210814106269,2.33952206190571,-2.21649231685619));
#71974=CARTESIAN_POINT('Ctrl Pts',(28.1220561892657,2.35044985172532,-2.20489202332356));
#71975=CARTESIAN_POINT('Ctrl Pts',(28.1224706915524,2.35507363717263,-2.19995261366683));
#71976=CARTESIAN_POINT('Ctrl Pts',(28.1233362691803,2.36468105612943,-2.18962438357931));
#71977=CARTESIAN_POINT('Ctrl Pts',(28.1237874603628,2.36966189760876,-2.18423302968863));
#71978=CARTESIAN_POINT('Ctrl Pts',(28.1248556077881,2.38138920895217,-2.17145184664944));
#71979=CARTESIAN_POINT('Ctrl Pts',(28.125473235972,2.38811973648419,-2.16404755202499));
#71980=CARTESIAN_POINT('Ctrl Pts',(28.1275199636159,2.41025619884647,-2.13946605881892));
#71981=CARTESIAN_POINT('Ctrl Pts',(28.1289553534561,2.42551186621469,-2.12215506104539));
#71982=CARTESIAN_POINT('Ctrl Pts',(28.1436954109205,2.57941165068406,-1.94369355382461));
#71983=CARTESIAN_POINT('Ctrl Pts',(28.1576709689823,2.70194736839792,-1.76939494225287));
#71984=CARTESIAN_POINT('Ctrl Pts',(28.1814809518632,2.87579308642091,-1.46145307721002));
#71985=CARTESIAN_POINT('Ctrl Pts',(28.1910899214638,2.93702002618647,-1.33414549362111));
#71986=CARTESIAN_POINT('Ctrl Pts',(28.2048647682225,3.01370436490644,-1.14360619307692));
#71987=CARTESIAN_POINT('Ctrl Pts',(28.2091411314489,3.03591463867732,-1.08326924731916));
#71988=CARTESIAN_POINT('Ctrl Pts',(28.2174068066051,3.07593729136249,-0.963616677390161));
#71989=CARTESIAN_POINT('Ctrl Pts',(28.2213992222562,3.09387523539417,-0.904369703475032));
#71990=CARTESIAN_POINT('Ctrl Pts',(28.2259358603936,3.11274097505395,-0.834902961275591));
#71991=CARTESIAN_POINT('Ctrl Pts',(28.2265691916793,3.11533924569788,-0.825154969164982));
#71992=CARTESIAN_POINT('Ctrl Pts',(28.2275199508806,3.11918681177818,-0.810442716005799));
#71993=CARTESIAN_POINT('Ctrl Pts',(28.2278393028512,3.1204700938411,-0.805487527529994));
#71994=CARTESIAN_POINT('Ctrl Pts',(28.2284085374021,3.12274134848174,-0.796630549556623));
#71995=CARTESIAN_POINT('Ctrl Pts',(28.2286586789113,3.12373381920064,-0.792729959955686));
#71996=CARTESIAN_POINT('Ctrl Pts',(28.229194754541,3.12584875387049,-0.784352238683463));
#71997=CARTESIAN_POINT('Ctrl Pts',(28.2294805531749,3.12696890372939,-0.779874568213961));
#71998=CARTESIAN_POINT('Ctrl Pts',(28.2302632262783,3.13001602330244,-0.767581945025658));
#71999=CARTESIAN_POINT('Ctrl Pts',(28.2307589745625,3.13192335747994,-0.759762090783327));
#72000=CARTESIAN_POINT('Ctrl Pts',(28.233366777799,3.14183471465703,-0.718455033790611));
#72001=CARTESIAN_POINT('Ctrl Pts',(28.2354507733549,3.14933137284442,-0.684846800540951));
#72002=CARTESIAN_POINT('Ctrl Pts',(28.241462182205,3.16963895771056,-0.586406776887985));
#72003=CARTESIAN_POINT('Ctrl Pts',(28.2453221679367,3.18099691236946,-0.521290545033046));
#72004=CARTESIAN_POINT('Ctrl Pts',(28.2634922060828,3.22566073134494,-0.208714749865713));
#72005=CARTESIAN_POINT('Ctrl Pts',(28.2770469271652,3.23213914685798,0.0417116433594993));
#72006=CARTESIAN_POINT('Ctrl Pts',(28.2992390819529,3.1970764524655,0.429258378900335));
#72007=CARTESIAN_POINT('Ctrl Pts',(28.3073664286035,3.17551456022348,0.567151264390502));
#72008=CARTESIAN_POINT('Ctrl Pts',(28.3169418900405,3.14093327577061,0.72181678609747));
#72009=CARTESIAN_POINT('Ctrl Pts',(28.3180993837322,3.13660662499194,0.740391903908868));
#72010=CARTESIAN_POINT('Ctrl Pts',(28.3198267634744,3.1299347564821,0.767926905585768));
#72011=CARTESIAN_POINT('Ctrl Pts',(28.3203925899964,3.12771532704182,0.776917075577408));
#72012=CARTESIAN_POINT('Ctrl Pts',(28.3214022195633,3.12369494969013,0.792905824274794));
#72013=CARTESIAN_POINT('Ctrl Pts',(28.3218455299276,3.12190914304143,0.799908173562081));
#72014=CARTESIAN_POINT('Ctrl Pts',(28.3227804643318,3.1180998602555,0.814637728043578));
#72015=CARTESIAN_POINT('Ctrl Pts',(28.3232722546208,3.1160711796675,0.822363525387183));
#72016=CARTESIAN_POINT('Ctrl Pts',(28.3245721953189,3.11064330407087,0.842725955597413));
#72017=CARTESIAN_POINT('Ctrl Pts',(28.3253819094511,3.1071958552759,0.85534946673081));
#72018=CARTESIAN_POINT('Ctrl Pts',(28.3290771327382,3.09116256843338,0.912682231214344));
#72019=CARTESIAN_POINT('Ctrl Pts',(28.3319914698645,3.07768850032045,0.957135314934866));
#72020=CARTESIAN_POINT('Ctrl Pts',(28.3398662395477,3.03910939137692,1.075162056889));
#72021=CARTESIAN_POINT('Ctrl Pts',(28.3448805190001,3.01229648263755,1.14814094974775));
#72022=CARTESIAN_POINT('Ctrl Pts',(28.3711270365197,2.86051555190064,1.51921930548057));
#72023=CARTESIAN_POINT('Ctrl Pts',(28.393651532448,2.69388118092647,1.79820365230385));
#72024=CARTESIAN_POINT('Ctrl Pts',(28.417950484081,2.45666141037764,2.0864930467848));
#72025=CARTESIAN_POINT('Ctrl Pts',(28.4211735880942,2.4238548398555,2.12451568840209));
#72026=CARTESIAN_POINT('Ctrl Pts',(28.4248803846094,2.38437191999677,2.16817039242104));
#72027=CARTESIAN_POINT('Ctrl Pts',(28.4254230074428,2.37854697457605,2.17455894314404));
#72028=CARTESIAN_POINT('Ctrl Pts',(28.4262901744422,2.36916416439731,2.18476679930449));
#72029=CARTESIAN_POINT('Ctrl Pts',(28.4266159248978,2.36562265513643,2.18860098227811));
#72030=CARTESIAN_POINT('Ctrl Pts',(28.4271929370244,2.35931916174096,2.19539222639864));
#72031=CARTESIAN_POINT('Ctrl Pts',(28.4274444812251,2.35656090816645,2.19835270634656));
#72032=CARTESIAN_POINT('Ctrl Pts',(28.4279750351948,2.35072135488711,2.20459677716374));
#72033=CARTESIAN_POINT('Ctrl Pts',(28.4282539413585,2.34763875605334,2.20787909765711));
#72034=CARTESIAN_POINT('Ctrl Pts',(28.428998597427,2.33937452469762,2.21664189258255));
#72035=CARTESIAN_POINT('Ctrl Pts',(28.4294633973172,2.33418047708267,2.22211069702994));
#72036=CARTESIAN_POINT('Ctrl Pts',(28.4316675193693,2.3093828903969,2.24803715164135));
#72037=CARTESIAN_POINT('Ctrl Pts',(28.4333880974362,2.28952859473432,2.26825468425339));
#72038=CARTESIAN_POINT('Ctrl Pts',(28.4475416242872,2.12234246979009,2.43406726891935));
#72039=CARTESIAN_POINT('Ctrl Pts',(28.4590453248097,1.9616000965906,2.56536439196085));
#72040=CARTESIAN_POINT('Ctrl Pts',(28.4706129526677,1.78943608566483,2.68030521728786));
#72041=CARTESIAN_POINT('Origin',(-1.72497344927317,0.,0.));
#72042=CARTESIAN_POINT('',(29.9668448649094,1.78943621037805,2.68030513402632));
#72043=CARTESIAN_POINT('',(29.720404475637,1.78943621037806,2.68030513402631));
#72044=CARTESIAN_POINT('',(-1.72497344927317,1.78943621037804,2.68030513402633));
#72045=CARTESIAN_POINT('',(29.1465734493345,-3.22274883168487,-0.00274415265993233));
#72046=CARTESIAN_POINT('Ctrl Pts',(29.1465734493345,-3.22274883168487,-0.00274415265989018));
#72047=CARTESIAN_POINT('Ctrl Pts',(29.1539365945277,-3.22264704388241,-0.12228433941176));
#72048=CARTESIAN_POINT('Ctrl Pts',(29.1612997397209,-3.21589035883655,-0.241535363539396));
#72049=CARTESIAN_POINT('Ctrl Pts',(29.168662884914,-3.20259786199393,-0.35983954320209));
#72050=CARTESIAN_POINT('Ctrl Pts',(29.1761213949534,-3.18913320544464,-0.479675956658851));
#72051=CARTESIAN_POINT('Ctrl Pts',(29.1835799049927,-3.16896241550941,-0.598540812488225));
#72052=CARTESIAN_POINT('Ctrl Pts',(29.1910384150321,-3.14225835233315,-0.715772316936422));
#72053=CARTESIAN_POINT('Ctrl Pts',(29.1965025791201,-3.12269474214264,-0.801657054398812));
#72054=CARTESIAN_POINT('Ctrl Pts',(29.2019667432081,-3.09962565234784,-0.886665604916692));
#72055=CARTESIAN_POINT('Ctrl Pts',(29.2074309072961,-3.0731351666899,-0.97054510959247));
#72056=CARTESIAN_POINT('Ctrl Pts',(29.2136031553889,-3.04321186150635,-1.06529429801687));
#72057=CARTESIAN_POINT('Ctrl Pts',(29.2197754034816,-3.00884990132546,-1.15882509071326));
#72058=CARTESIAN_POINT('Ctrl Pts',(29.2259476515744,-2.97016656609833,-1.2506910618261));
#72059=CARTESIAN_POINT('Ctrl Pts',(29.232111540227,-2.9315356219968,-1.34243261342848));
#72060=CARTESIAN_POINT('Ctrl Pts',(29.2382754288797,-2.88859510281043,-1.4325134282371));
#72061=CARTESIAN_POINT('Ctrl Pts',(29.2444393175323,-2.84151205947572,-1.5205021467772));
#72062=CARTESIAN_POINT('Ctrl Pts',(29.2505966791908,-2.79447887277581,-1.60839769331532));
#72063=CARTESIAN_POINT('Ctrl Pts',(29.2567540408494,-2.74331208662058,-1.69420516700848));
#72064=CARTESIAN_POINT('Ctrl Pts',(29.2629114025079,-2.68822645963843,-1.77751401237791));
#72065=CARTESIAN_POINT('Ctrl Pts',(29.2690642666542,-2.63318106876631,-1.86076200659519));
#72066=CARTESIAN_POINT('Ctrl Pts',(29.2752171308005,-2.57422276693174,-1.94151463980089));
#72067=CARTESIAN_POINT('Ctrl Pts',(29.2813699949468,-2.51161131371327,-2.01938757333195));
#72068=CARTESIAN_POINT('Ctrl Pts',(29.2875205280834,-2.44902358081521,-2.09723100473777));
#72069=CARTESIAN_POINT('Ctrl Pts',(29.2936710612199,-2.38278571840238,-2.17219656607689));
#72070=CARTESIAN_POINT('Ctrl Pts',(29.2998215943565,-2.31319918481417,-2.2439311695939));
#72071=CARTESIAN_POINT('Ctrl Pts',(29.3059714425717,-2.24362040035934,-2.31565778476918));
#72072=CARTESIAN_POINT('Ctrl Pts',(29.3121212907869,-2.17069398856901,-2.38415384567149));
#72073=CARTESIAN_POINT('Ctrl Pts',(29.3182711390021,-2.09475915463473,-2.44910221235742));
#72074=CARTESIAN_POINT('Ctrl Pts',(29.3244219473812,-2.01881246514147,-2.51406071930641));
#72075=CARTESIAN_POINT('Ctrl Pts',(29.3305727557603,-1.9398567506914,-2.5754701494945));
#72076=CARTESIAN_POINT('Ctrl Pts',(29.3367235641395,-1.85826447255666,-2.63305349594985));
#72077=CARTESIAN_POINT('Ctrl Pts',(29.3428809505056,-1.77658493549327,-2.69069842496221));
#72078=CARTESIAN_POINT('Ctrl Pts',(29.3490383368718,-1.69226355973061,-2.74450884837043));
#72079=CARTESIAN_POINT('Ctrl Pts',(29.355195723238,-1.60570188437601,-2.79425106620922));
#72080=CARTESIAN_POINT('Ctrl Pts',(29.361356545975,-1.51909189988605,-2.8440210446421));
#72081=CARTESIAN_POINT('Ctrl Pts',(29.3675173687119,-1.4302395121695,-2.8897180973201));
#72082=CARTESIAN_POINT('Ctrl Pts',(29.3736781914489,-1.3395690772516,-2.93115544619716));
#72083=CARTESIAN_POINT('Ctrl Pts',(29.3798493143656,-1.24874705190247,-2.97266207350651));
#72084=CARTESIAN_POINT('Ctrl Pts',(29.3860204372823,-1.15610131115029,-3.00989460952773));
#72085=CARTESIAN_POINT('Ctrl Pts',(29.392191560199,-1.06207444171456,-3.04271514321612));
#72086=CARTESIAN_POINT('Ctrl Pts',(29.3968870821445,-0.990530699211425,
-3.06768783267297));
#72087=CARTESIAN_POINT('Ctrl Pts',(29.4015826040901,-0.918187732348987,
-3.09010721650955));
#72088=CARTESIAN_POINT('Ctrl Pts',(29.4062781260356,-0.845244453328345,
-3.10993237492677));
#72089=CARTESIAN_POINT('Ctrl Pts',(29.4124503741284,-0.749360753915163,
-3.13599248020334));
#72090=CARTESIAN_POINT('Ctrl Pts',(29.4186226222212,-0.652101953643976,
-3.15765995028383));
#72091=CARTESIAN_POINT('Ctrl Pts',(29.4247948703139,-0.55390700439437,-3.17479205507744));
#72092=CARTESIAN_POINT('Ctrl Pts',(29.4309587589665,-0.455845046364051,
-3.19190095684969));
#72093=CARTESIAN_POINT('Ctrl Pts',(29.4371226476192,-0.356849883553671,
-3.20448662825541));
#72094=CARTESIAN_POINT('Ctrl Pts',(29.4432865362718,-0.257374705550446,
-3.21245635354674));
#72095=CARTESIAN_POINT('Ctrl Pts',(29.4494438979303,-0.158004862658673,
-3.22041763962822));
#72096=CARTESIAN_POINT('Ctrl Pts',(29.4556012595889,-0.0581564457071889,
-3.22377266263295));
#72097=CARTESIAN_POINT('Ctrl Pts',(29.4617586212474,0.0417090601862012,
-3.22248008788237));
#72098=CARTESIAN_POINT('Ctrl Pts',(29.4679114853937,0.141501621471133,-3.22118845726519));
#72099=CARTESIAN_POINT('Ctrl Pts',(29.4740643495401,0.24131081385163,-3.2152559838167));
#72100=CARTESIAN_POINT('Ctrl Pts',(29.4802172136864,0.340672873554422,-3.2046933637595));
#72101=CARTESIAN_POINT('Ctrl Pts',(29.4863677468229,0.439997289986294,-3.19413474534608));
#72102=CARTESIAN_POINT('Ctrl Pts',(29.4925182799594,0.538874478867406,-3.17894951163492));
#72103=CARTESIAN_POINT('Ctrl Pts',(29.498668813096,0.63684441801961,-3.1592003339037));
#72104=CARTESIAN_POINT('Ctrl Pts',(29.5048186613112,0.734803447271938,-3.13945335543435));
#72105=CARTESIAN_POINT('Ctrl Pts',(29.5109685095264,0.831855001849586,-3.11514352923547));
#72106=CARTESIAN_POINT('Ctrl Pts',(29.5171183577416,0.927548889084868,-3.08638471692325));
#72107=CARTESIAN_POINT('Ctrl Pts',(29.5232691661207,1.023257716822,-3.05762141455319));
#72108=CARTESIAN_POINT('Ctrl Pts',(29.5294199744998,1.11760804015507,-3.02440787142227));
#72109=CARTESIAN_POINT('Ctrl Pts',(29.535570782879,1.21016544472654,-2.98690762476676));
#72110=CARTESIAN_POINT('Ctrl Pts',(29.5417281692452,1.30282183489,-2.94936727344181));
#72111=CARTESIAN_POINT('Ctrl Pts',(29.5478855556114,1.39368107399298,-2.90753122741089));
#72112=CARTESIAN_POINT('Ctrl Pts',(29.5540429419775,1.48232945523467,-2.86161090098631));
#72113=CARTESIAN_POINT('Ctrl Pts',(29.5602037647145,1.57102731017963,-2.81566494692396));
#72114=CARTESIAN_POINT('Ctrl Pts',(29.5663645874514,1.65751147405801,-2.76563039061914));
#72115=CARTESIAN_POINT('Ctrl Pts',(29.5725254101884,1.74139537386461,-2.71176321134109));
#72116=CARTESIAN_POINT('Ctrl Pts',(29.5786965331051,1.8254195178044,-2.65780597239864));
#72117=CARTESIAN_POINT('Ctrl Pts',(29.5848676560218,1.90683435964463,-2.60000356287951));
#72118=CARTESIAN_POINT('Ctrl Pts',(29.5910387789385,1.98528457621415,-2.53865372076347));
#72119=CARTESIAN_POINT('Ctrl Pts',(29.5957343008841,2.04497625931844,-2.4919734757084));
#72120=CARTESIAN_POINT('Ctrl Pts',(29.6004298228297,2.10295222776889,-2.44324031750513));
#72121=CARTESIAN_POINT('Ctrl Pts',(29.6051253447753,2.15907050560192,-2.39259944711602));
#72122=CARTESIAN_POINT('Ctrl Pts',(29.6112975928681,2.23283779650938,-2.32603219020704));
#72123=CARTESIAN_POINT('Ctrl Pts',(29.6174698409608,2.30365349464721,-2.25593304337086));
#72124=CARTESIAN_POINT('Ctrl Pts',(29.6236420890536,2.3711601884149,-2.18259408121992));
#72125=CARTESIAN_POINT('Ctrl Pts',(29.6298059777062,2.43857545388016,-2.10935444635694));
#72126=CARTESIAN_POINT('Ctrl Pts',(29.6359698663589,2.50269033102026,-2.0328840343408));
#72127=CARTESIAN_POINT('Ctrl Pts',(29.6421337550115,2.5631817822715,-1.95351393993785));
#72128=CARTESIAN_POINT('Ctrl Pts',(29.6482911166701,2.62360917861084,-1.8742278912025));
#72129=CARTESIAN_POINT('Ctrl Pts',(29.6544484783286,2.68042051528346,-1.79204860809198));
#72130=CARTESIAN_POINT('Ctrl Pts',(29.6606058399872,2.73333149146086,-1.7073419459172));
#72131=CARTESIAN_POINT('Ctrl Pts',(29.6667587041335,2.78620381995504,-1.62269715589984));
#72132=CARTESIAN_POINT('Ctrl Pts',(29.6729115682798,2.83518122269407,-1.53552902441922));
#72133=CARTESIAN_POINT('Ctrl Pts',(29.6790644324261,2.88002193561497,-1.44623345725253));
#72134=CARTESIAN_POINT('Ctrl Pts',(29.6852149655626,2.92484566065228,-1.35697171967064));
#72135=CARTESIAN_POINT('Ctrl Pts',(29.6913654986992,2.9655356151429,-1.26558453562675));
#72136=CARTESIAN_POINT('Ctrl Pts',(29.6975160318357,3.00189578002228,-1.17249276687937));
#72137=CARTESIAN_POINT('Ctrl Pts',(29.7036658800509,3.03825189584574,-1.07941136480051));
#72138=CARTESIAN_POINT('Ctrl Pts',(29.7098157282661,3.07027902263686,-0.984626160020059));
#72139=CARTESIAN_POINT('Ctrl Pts',(29.7159655764813,3.09782951801712,-0.888577424764883));
#72140=CARTESIAN_POINT('Ctrl Pts',(29.7221163848605,3.12538431480304,-0.792513693606092));
#72141=CARTESIAN_POINT('Ctrl Pts',(29.7282671932396,3.14846097214959,-0.695186457715568));
#72142=CARTESIAN_POINT('Ctrl Pts',(29.7344180016188,3.16696216674654,-0.597049576581456));
#72143=CARTESIAN_POINT('Ctrl Pts',(29.740575387985,3.18548314746118,-0.498807742879522));
#72144=CARTESIAN_POINT('Ctrl Pts',(29.7467327743511,3.19941881351695,-0.399754962557698));
#72145=CARTESIAN_POINT('Ctrl Pts',(29.7528901607173,3.20872331301471,-0.300353563348061));
#72146=CARTESIAN_POINT('Ctrl Pts',(29.7590509834543,3.21803300525307,-0.200896689292029));
#72147=CARTESIAN_POINT('Ctrl Pts',(29.7652118061913,3.22270636341255,-0.101091242797806));
#72148=CARTESIAN_POINT('Ctrl Pts',(29.7713726289282,3.22274969555418,-0.00140082313525882));
#72149=CARTESIAN_POINT('Ctrl Pts',(29.7775437518449,3.22279310014211,0.0984562673249473));
#72150=CARTESIAN_POINT('Ctrl Pts',(29.7837148747616,3.21819103660215,0.198197512701616));
#72151=CARTESIAN_POINT('Ctrl Pts',(29.7898859976783,3.20900183790008,0.297363022001526));
#72152=CARTESIAN_POINT('Ctrl Pts',(29.7945815196239,3.20200990389554,0.372816684397168));
#72153=CARTESIAN_POINT('Ctrl Pts',(29.7992770415694,3.19236333657,0.447937103491324));
#72154=CARTESIAN_POINT('Ctrl Pts',(29.8039725635149,3.18010751241009,0.522526336190751));
#72155=CARTESIAN_POINT('Ctrl Pts',(29.810145611432,3.16399518439208,0.620586341636635));
#72156=CARTESIAN_POINT('Ctrl Pts',(29.8163186593491,3.1433146578272,0.718073021349551));
#72157=CARTESIAN_POINT('Ctrl Pts',(29.8224917072661,3.11811839613133,0.81452761169121));
#72158=CARTESIAN_POINT('Ctrl Pts',(29.8286544219621,3.09296431109531,0.910820744254038));
#72159=CARTESIAN_POINT('Ctrl Pts',(29.8348171366581,3.06330964035645,1.00608480836208));
#72160=CARTESIAN_POINT('Ctrl Pts',(29.8409798513541,3.02925817651817,1.09986929336982));
#72161=CARTESIAN_POINT('Ctrl Pts',(29.8471366564326,2.9952393656805,1.19356384553765));
#72162=CARTESIAN_POINT('Ctrl Pts',(29.8532934615111,2.95683228615114,1.28578123187714));
#72163=CARTESIAN_POINT('Ctrl Pts',(29.8594502665896,2.91419092727959,1.37608459109945));
#72164=CARTESIAN_POINT('Ctrl Pts',(29.8656028148151,2.87157905090681,1.46632551402171));
#72165=CARTESIAN_POINT('Ctrl Pts',(29.8717553630405,2.82473889859891,1.55465464853763));
#72166=CARTESIAN_POINT('Ctrl Pts',(29.877907911266,2.77387274597147,1.64065461071388));
#72167=CARTESIAN_POINT('Ctrl Pts',(29.8840578514049,2.72302815568237,1.72661811720819));
#72168=CARTESIAN_POINT('Ctrl Pts',(29.8902077915439,2.6681611795069,1.81025404137264));
#72169=CARTESIAN_POINT('Ctrl Pts',(29.8963577316828,2.60951977773627,1.89117003257329));
#72170=CARTESIAN_POINT('Ctrl Pts',(29.9025088196169,2.5508674314176,1.97210112554378));
#72171=CARTESIAN_POINT('Ctrl Pts',(29.9086599075509,2.48843949847947,2.05031091321287));
#72172=CARTESIAN_POINT('Ctrl Pts',(29.914810995485,2.42252667572612,2.12543691223601));
#72173=CARTESIAN_POINT('Ctrl Pts',(29.9209624546204,2.35660987531491,2.2005674449069));
#72174=CARTESIAN_POINT('Ctrl Pts',(29.9271139137557,2.28720805933935,2.27261349720804));
#72175=CARTESIAN_POINT('Ctrl Pts',(29.933265372891,2.21465049758197,2.34124768789207));
#72176=CARTESIAN_POINT('Ctrl Pts',(29.939422434067,2.14202685875271,2.40994438269339));
#72177=CARTESIAN_POINT('Ctrl Pts',(29.9455794952429,2.06624205488755,2.47522271598359));
#72178=CARTESIAN_POINT('Ctrl Pts',(29.9517365564189,1.9876601493618,2.53679417634522));
#72179=CARTESIAN_POINT('Ctrl Pts',(29.9567726592491,1.923384913903,2.58715589875203));
#72180=CARTESIAN_POINT('Ctrl Pts',(29.9618087620792,1.85723906645935,2.63503831559634));
#72181=CARTESIAN_POINT('Ctrl Pts',(29.9668448649094,1.78943621037805,2.68030513402632));
#72182=CARTESIAN_POINT('Ctrl Pts',(28.7169416469173,1.789436210378,2.68030513402635));
#72183=CARTESIAN_POINT('Ctrl Pts',(28.7230920480723,1.70631863714223,2.7357964261851));
#72184=CARTESIAN_POINT('Ctrl Pts',(28.7292424492274,1.62062725861836,2.78741127799514));
#72185=CARTESIAN_POINT('Ctrl Pts',(28.7353928503824,1.53276367189768,2.83491676925633));
#72186=CARTESIAN_POINT('Ctrl Pts',(28.741588152002,1.44425864476448,2.88276907019202));
#72187=CARTESIAN_POINT('Ctrl Pts',(28.7477834536215,1.35354995273938,2.92645154487067));
#72188=CARTESIAN_POINT('Ctrl Pts',(28.753978755241,1.26107138082195,2.96577418812893));
#72189=CARTESIAN_POINT('Ctrl Pts',(28.7601385685403,1.1691225505343,3.00487158092436));
#72190=CARTESIAN_POINT('Ctrl Pts',(28.7662983818395,1.07542449523086,3.03965886479008));
#72191=CARTESIAN_POINT('Ctrl Pts',(28.7724581951388,0.980420403090224,3.06999892438164));
#72192=CARTESIAN_POINT('Ctrl Pts',(28.7786712409184,0.884595295242538,3.10060117968409));
#72193=CARTESIAN_POINT('Ctrl Pts',(28.7848842866981,0.78744190608317,3.12667886497971));
#72194=CARTESIAN_POINT('Ctrl Pts',(28.7910973324778,0.689425724449649,3.14814385518945));
#72195=CARTESIAN_POINT('Ctrl Pts',(28.7973103782574,0.591409542816158,3.16960884539918));
#72196=CARTESIAN_POINT('Ctrl Pts',(28.8035234240371,0.492531019570413,3.18646112753636));
#72197=CARTESIAN_POINT('Ctrl Pts',(28.8097364698167,0.393259672669308,3.19866603326325));
#72198=CARTESIAN_POINT('Ctrl Pts',(28.8159087179095,0.294640186622187,3.21079079602322));
#72199=CARTESIAN_POINT('Ctrl Pts',(28.8220809660022,0.195285858324367,3.21837175495798));
#72200=CARTESIAN_POINT('Ctrl Pts',(28.828253214095,0.0956515038647144,3.22133021472627));
#72201=CARTESIAN_POINT('Ctrl Pts',(28.8344171027476,-0.00384790990404077,
3.22428466767777));
#72202=CARTESIAN_POINT('Ctrl Pts',(28.8405809914002,-0.103626165660649,
3.22262905216384));
#72203=CARTESIAN_POINT('Ctrl Pts',(28.8467448800529,-0.203221485069067,
3.2163362060746));
#72204=CARTESIAN_POINT('Ctrl Pts',(28.8529022417114,-0.302711342146973,
3.21005002353357));
#72205=CARTESIAN_POINT('Ctrl Pts',(28.8590596033699,-0.402018216875769,
3.19913640000185));
#72206=CARTESIAN_POINT('Ctrl Pts',(28.8652169650284,-0.500679444997268,
3.18362021225165));
#72207=CARTESIAN_POINT('Ctrl Pts',(28.8713698291747,-0.599268608149499,
3.16811535796663));
#72208=CARTESIAN_POINT('Ctrl Pts',(28.877522693321,-0.697212634505651,3.14801469066403));
#72209=CARTESIAN_POINT('Ctrl Pts',(28.8836755574673,-0.794054021945161,
3.12339491142774));
#72210=CARTESIAN_POINT('Ctrl Pts',(28.8898260906039,-0.890858721069464,
3.09878445938353));
#72211=CARTESIAN_POINT('Ctrl Pts',(28.8959766237404,-0.986561190796377,
3.0696584041735));
#72212=CARTESIAN_POINT('Ctrl Pts',(28.902127156877,-1.08071504194242,3.03614435767132));
#72213=CARTESIAN_POINT('Ctrl Pts',(28.9082770050922,-1.17485840814676,3.00263404328226));
#72214=CARTESIAN_POINT('Ctrl Pts',(28.9144268533074,-1.26745308940907,2.96473685476253));
#72215=CARTESIAN_POINT('Ctrl Pts',(28.9205767015226,-1.35806972334827,2.92262967018142));
#72216=CARTESIAN_POINT('Ctrl Pts',(28.9267275099017,-1.44870050508751,2.88051591148691));
#72217=CARTESIAN_POINT('Ctrl Pts',(28.9328783182809,-1.53735223212915,2.83419103422965));
#72218=CARTESIAN_POINT('Ctrl Pts',(28.93902912666,-1.62361824099614,2.78387883536705));
#72219=CARTESIAN_POINT('Ctrl Pts',(28.9451865130262,-1.70997650711697,2.73351283008216));
#72220=CARTESIAN_POINT('Ctrl Pts',(28.9513438993924,-1.79394358421042,2.67915120720089));
#72221=CARTESIAN_POINT('Ctrl Pts',(28.9575012857586,-1.87514013020339,2.62106219968181));
#72222=CARTESIAN_POINT('Ctrl Pts',(28.9636621084956,-1.9563819911109,2.56294077331559));
#72223=CARTESIAN_POINT('Ctrl Pts',(28.9698229312325,-2.03484990052825,2.50108808850675));
#72224=CARTESIAN_POINT('Ctrl Pts',(28.9759837539695,-2.11019772621331,2.43581261980148));
#72225=CARTESIAN_POINT('Ctrl Pts',(28.9821548768862,-2.18567152470756,2.37042801809751));
#72226=CARTESIAN_POINT('Ctrl Pts',(28.9883259998029,-2.25801450496965,2.30160950151284));
#72227=CARTESIAN_POINT('Ctrl Pts',(28.9944971227196,-2.32691741852836,2.22970242181536));
#72228=CARTESIAN_POINT('Ctrl Pts',(28.9991926446652,-2.37934469101972,2.1749893209224));
#72229=CARTESIAN_POINT('Ctrl Pts',(29.0038881666108,-2.42978110979645,2.11848886705525));
#72230=CARTESIAN_POINT('Ctrl Pts',(29.0085836885564,-2.47810684884475,2.06036501819672));
#72231=CARTESIAN_POINT('Ctrl Pts',(29.0147236408184,-2.54129848850042,1.98436118701271));
#72232=CARTESIAN_POINT('Ctrl Pts',(29.0208635930804,-2.60110917768486,1.90530443147936));
#72233=CARTESIAN_POINT('Ctrl Pts',(29.0270035453424,-2.65722736051133,1.82352963152509));
#72234=CARTESIAN_POINT('Ctrl Pts',(29.0331355937507,-2.71327330337753,1.74186009884785));
#72235=CARTESIAN_POINT('Ctrl Pts',(29.039267642159,-2.76563593488611,1.65747982917819));
#72236=CARTESIAN_POINT('Ctrl Pts',(29.0453996905672,-2.81404291051849,1.57075779809003));
#72237=CARTESIAN_POINT('Ctrl Pts',(29.0515255272026,-2.86240084982258,1.48412361653038));
#72238=CARTESIAN_POINT('Ctrl Pts',(29.057651363838,-2.90681088164606,1.39515276731076));
#72239=CARTESIAN_POINT('Ctrl Pts',(29.0637772004734,-2.94704370153479,1.30424345263609));
#72240=CARTESIAN_POINT('Ctrl Pts',(29.0698985113498,-2.98724679747584,1.21340130162832));
#72241=CARTESIAN_POINT('Ctrl Pts',(29.0760198222262,-3.02327863810538,1.12062393158621));
#72242=CARTESIAN_POINT('Ctrl Pts',(29.0821411331026,-3.05495616561474,1.02633346855322));
#72243=CARTESIAN_POINT('Ctrl Pts',(29.0882604710991,-3.08662348355351,0.932073395049127));
#72244=CARTESIAN_POINT('Ctrl Pts',(29.0943798090956,-3.11393913225344,0.83630161145799));
#72245=CARTESIAN_POINT('Ctrl Pts',(29.1004991470922,-3.13676878203506,0.739458701044398));
#72246=CARTESIAN_POINT('Ctrl Pts',(29.1066172902293,-3.15959397410869,0.642634700137558));
#72247=CARTESIAN_POINT('Ctrl Pts',(29.1127354333664,-3.17793481269061,0.54474041657791));
#72248=CARTESIAN_POINT('Ctrl Pts',(29.1188535765035,-3.19170760561652,0.446228778486655));
#72249=CARTESIAN_POINT('Ctrl Pts',(29.1249740935066,-3.20548574244542,0.347678917455325));
#72250=CARTESIAN_POINT('Ctrl Pts',(29.1310946105096,-3.21469223594896,0.248511658979369));
#72251=CARTESIAN_POINT('Ctrl Pts',(29.1372151275126,-3.21929509697444,0.149186598246397));
#72252=CARTESIAN_POINT('Ctrl Pts',(29.1403345680994,-3.22164103466096,0.0985636483246456));
#72253=CARTESIAN_POINT('Ctrl Pts',(29.1434540086863,-3.22279195468255,0.0478997648342351));
#72254=CARTESIAN_POINT('Ctrl Pts',(29.1465734492731,-3.22274883168572,-0.00274415166250658));
#72255=CARTESIAN_POINT('',(28.9000265507269,-3.22274949573006,0.00180285098271473));
#72256=CARTESIAN_POINT('Ctrl Pts',(28.4706129526677,1.78943608566483,2.68030521728786));
#72257=CARTESIAN_POINT('Ctrl Pts',(28.4727295044825,1.75793489507861,2.7013361680963));
#72258=CARTESIAN_POINT('Ctrl Pts',(28.4748473913004,1.72605128848407,2.72181956088802));
#72259=CARTESIAN_POINT('Ctrl Pts',(28.4890742403561,1.51003995035203,2.85526737105806));
#72260=CARTESIAN_POINT('Ctrl Pts',(28.5013624938769,1.31536319151967,2.95001232999312));
#72261=CARTESIAN_POINT('Ctrl Pts',(28.5154841624719,1.09587243875544,3.03075935681712));
#72262=CARTESIAN_POINT('Ctrl Pts',(28.5165707468582,1.07900356595487,3.03680588210346));
#72263=CARTESIAN_POINT('Ctrl Pts',(28.5182199797039,1.05343481829922,3.04573088050518));
#72264=CARTESIAN_POINT('Ctrl Pts',(28.5187791713373,1.04477146750845,3.04871351406174));
#72265=CARTESIAN_POINT('Ctrl Pts',(28.5197532938551,1.02969094157001,3.05383363581636));
#72266=CARTESIAN_POINT('Ctrl Pts',(28.5201676649291,1.02327950743741,3.05598795137482));
#72267=CARTESIAN_POINT('Ctrl Pts',(28.5210242119371,1.01003396508126,3.06039224924279));
#72268=CARTESIAN_POINT('Ctrl Pts',(28.521466473438,1.0031990139534,3.06263955876425));
#72269=CARTESIAN_POINT('Ctrl Pts',(28.5225032579769,0.987186039440626,3.06784521674254));
#72270=CARTESIAN_POINT('Ctrl Pts',(28.5230983797989,0.978002186986164,3.07078528545501));
#72271=CARTESIAN_POINT('Ctrl Pts',(28.5243615879796,0.958525617742078,3.07692417423077));
#72272=CARTESIAN_POINT('Ctrl Pts',(28.5250300065371,0.948229790891023,3.08011265913365));
#72273=CARTESIAN_POINT('Ctrl Pts',(28.5268349413851,0.92045626586622,3.08856130954047));
#72274=CARTESIAN_POINT('Ctrl Pts',(28.5279746068773,0.902949755768552,3.09372468338722));
#72275=CARTESIAN_POINT('Ctrl Pts',(28.537049582533,0.763801217389873,3.13348350209853));
#72276=CARTESIAN_POINT('Ctrl Pts',(28.5452117401538,0.640277226405743,3.16103611379191));
#72277=CARTESIAN_POINT('Ctrl Pts',(28.5689797169024,0.284827672248869,3.21863040137646));
#72278=CARTESIAN_POINT('Ctrl Pts',(28.5850097161605,0.0508145721802403,
3.23080647441244));
#72279=CARTESIAN_POINT('Ctrl Pts',(28.6028215701293,-0.215184034125109,
3.21572543488327));
#72280=CARTESIAN_POINT('Ctrl Pts',(28.6050048580802,-0.247914768802032,
3.21336779972816));
#72281=CARTESIAN_POINT('Ctrl Pts',(28.6124861683806,-0.360676076150754,
3.20351225285942));
#72282=CARTESIAN_POINT('Ctrl Pts',(28.6177100565749,-0.440465734777603,
3.19352006309415));
#72283=CARTESIAN_POINT('Ctrl Pts',(28.6234706604028,-0.530594618158025,
3.17879008952027));
#72284=CARTESIAN_POINT('Ctrl Pts',(28.6241573930998,-0.541375115963997,
3.17697184028573));
#72285=CARTESIAN_POINT('Ctrl Pts',(28.6251639226805,-0.557232459611563,
3.17421426488825));
#72286=CARTESIAN_POINT('Ctrl Pts',(28.6254860804061,-0.562316495106303,
3.17331756584224));
#72287=CARTESIAN_POINT('Ctrl Pts',(28.6260590295858,-0.571374123468075,
3.17169757158011));
#72288=CARTESIAN_POINT('Ctrl Pts',(28.6263100894441,-0.575348529106249,
3.17097901999995));
#72289=CARTESIAN_POINT('Ctrl Pts',(28.6268421416797,-0.583782908579059,
3.16943774914286));
#72290=CARTESIAN_POINT('Ctrl Pts',(28.6271230211045,-0.588242485315028,
3.1686130892104));
#72291=CARTESIAN_POINT('Ctrl Pts',(28.627878534898,-0.600256045964039,3.1663653183137));
#72292=CARTESIAN_POINT('Ctrl Pts',(28.6283521702342,-0.607806761761256,
3.16492457934481));
#72293=CARTESIAN_POINT('Ctrl Pts',(28.6306640656055,-0.644753076792489,
3.15773782044793));
#72294=CARTESIAN_POINT('Ctrl Pts',(28.6324812895651,-0.674073902545802,
3.15160898561473));
#72295=CARTESIAN_POINT('Ctrl Pts',(28.637530472391,-0.756162766545356,3.13325213706511));
#72296=CARTESIAN_POINT('Ctrl Pts',(28.6407180921002,-0.808716082753272,
3.1201009711335));
#72297=CARTESIAN_POINT('Ctrl Pts',(28.6535268632144,-1.02140915835613,3.06114004849999));
#72298=CARTESIAN_POINT('Ctrl Pts',(28.6627656154892,-1.17822366782285,3.00427228577279));
#72299=CARTESIAN_POINT('Ctrl Pts',(28.6854293264578,-1.54743747174325,2.83699934920233));
#72300=CARTESIAN_POINT('Ctrl Pts',(28.6989100470409,-1.75326871871093,2.7146186528809));
#72301=CARTESIAN_POINT('Ctrl Pts',(28.7145128574428,-1.95934218713017,2.55880460220443));
#72302=CARTESIAN_POINT('Ctrl Pts',(28.7157037052972,-1.9748893587462,2.54682445269971));
#72303=CARTESIAN_POINT('Ctrl Pts',(28.7174651636032,-1.99761535818559,2.52897930859047));
#72304=CARTESIAN_POINT('Ctrl Pts',(28.7180314036468,-2.00488006208335,2.52322400836126));
#72305=CARTESIAN_POINT('Ctrl Pts',(28.7190426952652,-2.01778144644494,2.51291228039299));
#72306=CARTESIAN_POINT('Ctrl Pts',(28.7194872565306,-2.02342779457625,2.50836800596334));
#72307=CARTESIAN_POINT('Ctrl Pts',(28.7199376348755,-2.02912255966154,2.50375302438614));
#72308=CARTESIAN_POINT('Ctrl Pts',(28.7199426831262,-2.02918638854648,2.50370129404203));
#72309=CARTESIAN_POINT('Ctrl Pts',(28.7199525544446,-2.02931119283795,2.5036001380579));
#72310=CARTESIAN_POINT('Ctrl Pts',(28.7199573775245,-2.02937216868127,2.50355071241681));
#72311=CARTESIAN_POINT('Ctrl Pts',(28.7199668101851,-2.02949141543693,2.50345404647158));
#72312=CARTESIAN_POINT('Ctrl Pts',(28.7199714197684,-2.02954968663765,2.50340680625344));
#72313=CARTESIAN_POINT('Ctrl Pts',(28.719980436379,-2.02966366319617,2.50331439934023));
#72314=CARTESIAN_POINT('Ctrl Pts',(28.7199848434139,-2.02971936888273,2.50326923266861));
#72315=CARTESIAN_POINT('Ctrl Pts',(28.7199934652108,-2.0298283450773,2.50318086776095));
#72316=CARTESIAN_POINT('Ctrl Pts',(28.7199976799805,-2.02988161589276,2.50313766953882));
#72317=CARTESIAN_POINT('Ctrl Pts',(28.7200059269046,-2.02998584503108,2.5030531428194));
#72318=CARTESIAN_POINT('Ctrl Pts',(28.7200099590702,-2.03003680368479,2.5030118142929));
#72319=CARTESIAN_POINT('Ctrl Pts',(28.7200178498728,-2.03013652390136,2.50293093407779));
#72320=CARTESIAN_POINT('Ctrl Pts',(28.7200217085217,-2.03018528578732,2.50289138234451));
#72321=CARTESIAN_POINT('Ctrl Pts',(28.7200292608351,-2.03028072095256,2.50281396836442));
#72322=CARTESIAN_POINT('Ctrl Pts',(28.7200329545167,-2.03032739460655,2.50277610601144));
#72323=CARTESIAN_POINT('Ctrl Pts',(28.7200401849441,-2.03041875547619,2.50270198849596));
#72324=CARTESIAN_POINT('Ctrl Pts',(28.7200437217096,-2.03046344308596,2.50266573319381));
#72325=CARTESIAN_POINT('Ctrl Pts',(28.7200506458915,-2.03055092815146,2.50259475219629));
#72326=CARTESIAN_POINT('Ctrl Pts',(28.7200540333285,-2.0305937259991,2.50256002634706));
#72327=CARTESIAN_POINT('Ctrl Pts',(28.7200606660094,-2.03067752233993,2.50249203106638));
#72328=CARTESIAN_POINT('Ctrl Pts',(28.7200639112747,-2.03071852122213,2.50245876146894));
#72329=CARTESIAN_POINT('Ctrl Pts',(28.7200702663552,-2.03079880517355,2.50239360971951));
#72330=CARTESIAN_POINT('Ctrl Pts',(28.7200733761979,-2.03083809069897,2.50236172733389));
#72331=CARTESIAN_POINT('Ctrl Pts',(28.7200794668121,-2.03091502883903,2.50229928475532));
#72332=CARTESIAN_POINT('Ctrl Pts',(28.7200824476102,-2.0309526818909,2.50226872433223));
#72333=CARTESIAN_POINT('Ctrl Pts',(28.7200882861469,-2.03102643131658,2.50220886417468));
#72334=CARTESIAN_POINT('Ctrl Pts',(28.7200911439205,-2.0310625282243,2.50217956412083));
#72335=CARTESIAN_POINT('Ctrl Pts',(28.720096742103,-2.03113323756459,2.5021221664314));
#72336=CARTESIAN_POINT('Ctrl Pts',(28.7200994825457,-2.03116785050777,2.50209406848553));
#72337=CARTESIAN_POINT('Ctrl Pts',(28.7201048514603,-2.03123566029126,2.50203901981741));
#72338=CARTESIAN_POINT('Ctrl Pts',(28.7201074799629,-2.0312688575962,2.50201206881331));
#72339=CARTESIAN_POINT('Ctrl Pts',(28.7201126300838,-2.03133390056996,2.50195926197395));
#72340=CARTESIAN_POINT('Ctrl Pts',(28.7201151517418,-2.03136574680939,2.50193340576271));
#72341=CARTESIAN_POINT('Ctrl Pts',(28.720120093006,-2.03142814889091,2.50188273904716));
#72342=CARTESIAN_POINT('Ctrl Pts',(28.7201225126508,-2.03145870528253,2.50185792817662));
#72343=CARTESIAN_POINT('Ctrl Pts',(28.7201276943124,-2.03152414011088,2.50180479507587));
#72344=CARTESIAN_POINT('Ctrl Pts',(28.7201304563826,-2.03155901899685,2.50177647219966));
#72345=CARTESIAN_POINT('Ctrl Pts',(28.7201359554465,-2.03162845818275,2.50172008273973));
#72346=CARTESIAN_POINT('Ctrl Pts',(28.7201386919801,-2.03166301269002,2.50169202088279));
#72347=CARTESIAN_POINT('Ctrl Pts',(28.7201441397585,-2.03173180049443,2.50163615565982));
#72348=CARTESIAN_POINT('Ctrl Pts',(28.7201468510127,-2.03176603392591,2.50160835220658));
#72349=CARTESIAN_POINT('Ctrl Pts',(28.7201522486444,-2.03183418483247,2.50155299958952));
#72350=CARTESIAN_POINT('Ctrl Pts',(28.7201549350277,-2.03186810239707,2.50152545037433));
#72351=CARTESIAN_POINT('Ctrl Pts',(28.7201602833151,-2.03193562663903,2.50147060217975));
#72352=CARTESIAN_POINT('Ctrl Pts',(28.7201629452272,-2.03196923343427,2.50144330312541));
#72353=CARTESIAN_POINT('Ctrl Pts',(28.7201682449533,-2.03203614099672,2.50138895136757));
#72354=CARTESIAN_POINT('Ctrl Pts',(28.720170882781,-2.03206944195467,2.5013618985294));
#72355=CARTESIAN_POINT('Ctrl Pts',(28.7206759851055,-2.03844588039425,2.49618163325451));
#72356=CARTESIAN_POINT('Ctrl Pts',(28.721179424105,-2.04476934623587,2.49100435010067));
#72357=CARTESIAN_POINT('Ctrl Pts',(28.7225532920708,-2.06193840546178,2.47683790474673));
#72358=CARTESIAN_POINT('Ctrl Pts',(28.7234256375139,-2.07274476785869,2.46780167588261));
#72359=CARTESIAN_POINT('Ctrl Pts',(28.7253669157401,-2.09658027330571,2.44760353392396));
#72360=CARTESIAN_POINT('Ctrl Pts',(28.7264372253725,-2.10958015509097,2.43640789946328));
#72361=CARTESIAN_POINT('Ctrl Pts',(28.7296998049574,-2.14877495982948,2.40210405235703));
#72362=CARTESIAN_POINT('Ctrl Pts',(28.7319053879873,-2.17468346662151,2.37867386844445));
#72363=CARTESIAN_POINT('Ctrl Pts',(28.7400861426802,-2.26861112306329,2.29091368874828));
#72364=CARTESIAN_POINT('Ctrl Pts',(28.7461659480859,-2.33419368736704,2.22405464748236));
#72365=CARTESIAN_POINT('Ctrl Pts',(28.7671310659061,-2.5465483442188,1.98781472318676));
#72366=CARTESIAN_POINT('Ctrl Pts',(28.7824746059258,-2.67853733533576,1.80602848377298));
#72367=CARTESIAN_POINT('Ctrl Pts',(28.8003815918656,-2.8121610109073,1.57471495854765));
#72368=CARTESIAN_POINT('Ctrl Pts',(28.8032560882735,-2.83297843608909,1.53694832855815));
#72369=CARTESIAN_POINT('Ctrl Pts',(28.8113903376117,-2.89022355897624,1.42797782149335));
#72370=CARTESIAN_POINT('Ctrl Pts',(28.8165870148902,-2.9247704374252,1.35581459108444));
#72371=CARTESIAN_POINT('Ctrl Pts',(28.82232103569,-2.96094428794717,1.27241726824758));
#72372=CARTESIAN_POINT('Ctrl Pts',(28.8230068946184,-2.96523833001631,1.26237808723768));
#72373=CARTESIAN_POINT('Ctrl Pts',(28.8240123900179,-2.97148636917695,1.24756280157262));
#72374=CARTESIAN_POINT('Ctrl Pts',(28.8243343804688,-2.97347999505174,1.24280364739755));
#72375=CARTESIAN_POINT('Ctrl Pts',(28.8249071414465,-2.97701360861734,1.23431108152394));
#72376=CARTESIAN_POINT('Ctrl Pts',(28.8251581797195,-2.9785580154974,1.23057954674583));
#72377=CARTESIAN_POINT('Ctrl Pts',(28.8256903062262,-2.98182247472593,1.22264993903493));
#72378=CARTESIAN_POINT('Ctrl Pts',(28.8259712810604,-2.98354067259231,1.21845114789025));
#72379=CARTESIAN_POINT('Ctrl Pts',(28.8267273202313,-2.98814884432928,1.20712188346871));
#72380=CARTESIAN_POINT('Ctrl Pts',(28.8272013831376,-2.99102218193026,1.19998461134786));
#72381=CARTESIAN_POINT('Ctrl Pts',(28.8295186355071,-3.00498587026777,1.16493752107379));
#72382=CARTESIAN_POINT('Ctrl Pts',(28.8313406712834,-3.01571171473066,1.13688280614774));
#72383=CARTESIAN_POINT('Ctrl Pts',(28.8364066778901,-3.04474754066777,1.05763215788102));
#72384=CARTESIAN_POINT('Ctrl Pts',(28.8396059511832,-3.06215717023721,1.00611506704069));
#72385=CARTESIAN_POINT('Ctrl Pts',(28.8614999018027,-3.17387395674761,0.645708082223044));
#72386=CARTESIAN_POINT('Ctrl Pts',(28.8787363876768,-3.2225834237722,0.324626768808879));
#72387=CARTESIAN_POINT('Ctrl Pts',(28.8975369561408,-3.22274957354346,0.00165792806279125));
#72388=CARTESIAN_POINT('Ctrl Pts',(28.9000265507269,-3.22274949573006,0.00180285098271473));
#72389=CARTESIAN_POINT('Ctrl Pts',(28.9062469553981,-3.22280611626949,-0.0994111798219162));
#72390=CARTESIAN_POINT('Ctrl Pts',(28.9124673600693,-3.2180902853374,-0.200629471102156));
#72391=CARTESIAN_POINT('Ctrl Pts',(28.9186877647406,-3.20862730534657,-0.301377467446362));
#72392=CARTESIAN_POINT('Ctrl Pts',(28.9249096482869,-3.199162075572,-0.402149416203597));
#72393=CARTESIAN_POINT('Ctrl Pts',(28.9311315318332,-3.18494749082946,-0.502450428911549));
#72394=CARTESIAN_POINT('Ctrl Pts',(28.9373534153795,-3.16606066637834,-0.601811780635709));
#72395=CARTESIAN_POINT('Ctrl Pts',(28.9435782946896,-3.14716474814318,-0.701220973683151));
#72396=CARTESIAN_POINT('Ctrl Pts',(28.9498031739997,-3.12359219348165,-0.799689192911505));
#72397=CARTESIAN_POINT('Ctrl Pts',(28.9560280533098,-3.09547090486905,-0.896759410103493));
#72398=CARTESIAN_POINT('Ctrl Pts',(28.9622617721606,-3.06730968306884,-0.993967470310051));
#72399=CARTESIAN_POINT('Ctrl Pts',(28.9684954910114,-3.03458694818972,-1.08977316063798));
#72400=CARTESIAN_POINT('Ctrl Pts',(28.9747292098621,-2.99748007068733,-1.18373594535788));
#72401=CARTESIAN_POINT('Ctrl Pts',(28.9809679115004,-2.96034353261007,-1.27777383718453));
#72402=CARTESIAN_POINT('Ctrl Pts',(28.9872066131386,-2.9188160442815,-1.3699655066406));
#72403=CARTESIAN_POINT('Ctrl Pts',(28.9934453147768,-2.87312170876266,-1.45989356089297));
#72404=CARTESIAN_POINT('Ctrl Pts',(28.9996951751885,-2.82734564265821,-1.54998246380312));
#72405=CARTESIAN_POINT('Ctrl Pts',(29.0059450356002,-2.77738805389628,-1.63779930163882));
#72406=CARTESIAN_POINT('Ctrl Pts',(29.0121948960119,-2.72351734831205,-1.72295409571565));
#72407=CARTESIAN_POINT('Ctrl Pts',(29.0151140239309,-2.69835590944289,-1.76272742191107));
#72408=CARTESIAN_POINT('Ctrl Pts',(29.01803315185,-2.67234139295002,-1.80192046270654));
#72409=CARTESIAN_POINT('Ctrl Pts',(29.020952279769,-2.64550411478208,-1.84049600411711));
#72410=CARTESIAN_POINT('Ctrl Pts',(29.0271245278618,-2.58875896911496,-1.92206071059866));
#72411=CARTESIAN_POINT('Ctrl Pts',(29.0332967759546,-2.52813827528339,-2.00114221898893));
#72412=CARTESIAN_POINT('Ctrl Pts',(29.0394690240473,-2.46388676111151,-2.07734917404837));
#72413=CARTESIAN_POINT('Ctrl Pts',(29.0456329127,-2.39972226656004,-2.1534529175277));
#72414=CARTESIAN_POINT('Ctrl Pts',(29.0517968013526,-2.33193700313867,-2.22668951662612));
#72415=CARTESIAN_POINT('Ctrl Pts',(29.0579606900052,-2.26081873786643,-2.2966968012805));
#72416=CARTESIAN_POINT('Ctrl Pts',(29.0641180516638,-2.18977578032973,-2.36662995462615));
#72417=CARTESIAN_POINT('Ctrl Pts',(29.0702754133223,-2.11540714546243,-2.43334028887111));
#72418=CARTESIAN_POINT('Ctrl Pts',(29.0764327749809,-2.03803996333273,-2.49649968362881));
#72419=CARTESIAN_POINT('Ctrl Pts',(29.0825856391272,-1.96072929239533,-2.55961294496656));
#72420=CARTESIAN_POINT('Ctrl Pts',(29.0887385032735,-1.88042476420995,-2.61918014968364));
#72421=CARTESIAN_POINT('Ctrl Pts',(29.0948913674198,-1.79748867799225,-2.67491159012586));
#72422=CARTESIAN_POINT('Ctrl Pts',(29.1010419005564,-1.71458401207297,-2.7306219167373));
#72423=CARTESIAN_POINT('Ctrl Pts',(29.1071924336929,-1.62905012921972,-2.78249912452597));
#72424=CARTESIAN_POINT('Ctrl Pts',(29.1133429668295,-1.54127984800482,-2.83029574296296));
#72425=CARTESIAN_POINT('Ctrl Pts',(29.1194928150447,-1.45351934085925,-2.87808703878441));
#72426=CARTESIAN_POINT('Ctrl Pts',(29.1256426632599,-1.36352331196813,-2.92179844095367));
#72427=CARTESIAN_POINT('Ctrl Pts',(29.1317925114751,-1.27170992941109,-2.96122802531943));
#72428=CARTESIAN_POINT('Ctrl Pts',(29.1379433198542,-1.17988221220785,-3.0006637657501));
#72429=CARTESIAN_POINT('Ctrl Pts',(29.1440941282334,-1.08623697692175,-3.03581618911754));
#72430=CARTESIAN_POINT('Ctrl Pts',(29.1502449366125,-0.991212208981483,
-3.06653157806439));
#72431=CARTESIAN_POINT('Ctrl Pts',(29.1564023229787,-0.896085816725511,
-3.09727981560903));
#72432=CARTESIAN_POINT('Ctrl Pts',(29.1625597093449,-0.79957735983448,-3.12358140921857));
#72433=CARTESIAN_POINT('Ctrl Pts',(29.1687170957111,-0.70213970799351,-3.1453326362976));
#72434=CARTESIAN_POINT('Ctrl Pts',(29.1748779184481,-0.604647677252323,
-3.16709600250133));
#72435=CARTESIAN_POINT('Ctrl Pts',(29.181038741185,-0.506225846727573,-3.18430386996202));
#72436=CARTESIAN_POINT('Ctrl Pts',(29.187199563922,-0.407334917707618,-3.19690410042531));
#72437=CARTESIAN_POINT('Ctrl Pts',(29.1933706868387,-0.308278654545428,
-3.20952539700978));
#72438=CARTESIAN_POINT('Ctrl Pts',(29.1995418097554,-0.208752159497449,
-3.217523634414));
#72439=CARTESIAN_POINT('Ctrl Pts',(29.2057129326721,-0.109219008293064,
-3.22089875201433));
#72440=CARTESIAN_POINT('Ctrl Pts',(29.2104084546176,-0.0334856122647015,
-3.22346683224464));
#72441=CARTESIAN_POINT('Ctrl Pts',(29.2151039765632,0.0422515786952583,
-3.2233594471387));
#72442=CARTESIAN_POINT('Ctrl Pts',(29.2197994985087,0.117790482376118,-3.22059667837524));
#72443=CARTESIAN_POINT('Ctrl Pts',(29.2259717466015,0.217086121834415,-3.21696502795835));
#72444=CARTESIAN_POINT('Ctrl Pts',(29.2321439946942,0.316388421497807,-3.20873054124445));
#72445=CARTESIAN_POINT('Ctrl Pts',(29.238316242787,0.415235843009876,-3.19588747567556));
#72446=CARTESIAN_POINT('Ctrl Pts',(29.2444801314396,0.513949389620937,-3.18306180422889));
#72447=CARTESIAN_POINT('Ctrl Pts',(29.2506440200922,0.612208855622406,-3.16564001540881));
#72448=CARTESIAN_POINT('Ctrl Pts',(29.2568079087449,0.709553981755064,-3.14366835233546));
#72449=CARTESIAN_POINT('Ctrl Pts',(29.2629652704034,0.806796028306152,-3.12171995524291));
#72450=CARTESIAN_POINT('Ctrl Pts',(29.2691226320619,0.903125238486049,-3.0952313574475));
#72451=CARTESIAN_POINT('Ctrl Pts',(29.2752799937205,0.998088711923224,-3.06430032562597));
#72452=CARTESIAN_POINT('Ctrl Pts',(29.2814328578668,1.09298282133614,-3.03339188671058));
#72453=CARTESIAN_POINT('Ctrl Pts',(29.2875857220131,1.18651276557843,-2.99804759926694));
#72454=CARTESIAN_POINT('Ctrl Pts',(29.2937385861594,1.27823894109332,-2.95841558472988));
#72455=CARTESIAN_POINT('Ctrl Pts',(29.2998891192959,1.36993036618858,-2.91879858476339));
#72456=CARTESIAN_POINT('Ctrl Pts',(29.3060396524325,1.45981898207847,-2.87489725747929));
#72457=CARTESIAN_POINT('Ctrl Pts',(29.312190185569,1.54748421332389,-2.82690823551338));
#72458=CARTESIAN_POINT('Ctrl Pts',(29.3183400337842,1.63513968219823,-2.77892455758903));
#72459=CARTESIAN_POINT('Ctrl Pts',(29.3244898819994,1.72057187766139,-2.72685429857199));
#72460=CARTESIAN_POINT('Ctrl Pts',(29.3306397302146,1.80338483155499,-2.6709400427223));
#72461=CARTESIAN_POINT('Ctrl Pts',(29.3367905385938,1.88621071487524,-2.61501705708776));
#72462=CARTESIAN_POINT('Ctrl Pts',(29.3429413469729,1.96641618433717,-2.55524912564648));
#72463=CARTESIAN_POINT('Ctrl Pts',(29.3490921553521,2.0436351083236,-2.49192156909626));
#72464=CARTESIAN_POINT('Ctrl Pts',(29.3552495417182,2.1209366141514,-2.42852628683894));
#72465=CARTESIAN_POINT('Ctrl Pts',(29.3614069280844,2.19524485996242,-2.36156405358489));
#72466=CARTESIAN_POINT('Ctrl Pts',(29.3675643144506,2.26622772210905,-2.29135974348081));
#72467=CARTESIAN_POINT('Ctrl Pts',(29.3737251371876,2.33725019902376,-2.22111625311013));
#72468=CARTESIAN_POINT('Ctrl Pts',(29.3798859599245,2.40494330205086,-2.14762740205811));
#72469=CARTESIAN_POINT('Ctrl Pts',(29.3860467826615,2.46901406612221,-2.07125254466728));
#72470=CARTESIAN_POINT('Ctrl Pts',(29.3922179055782,2.53319194906604,-1.99474999738968));
#72471=CARTESIAN_POINT('Ctrl Pts',(29.3983890284949,2.59373513261231,-1.91535215142283));
#72472=CARTESIAN_POINT('Ctrl Pts',(29.4045601514116,2.65039290562038,-1.83344893802286));
#72473=CARTESIAN_POINT('Ctrl Pts',(29.4092556733572,2.69350302028513,-1.77112991746091));
#72474=CARTESIAN_POINT('Ctrl Pts',(29.4139511953028,2.73436456161787,-1.70736105306669));
#72475=CARTESIAN_POINT('Ctrl Pts',(29.4186467172484,2.77288515458528,-1.64232319656655));
#72476=CARTESIAN_POINT('Ctrl Pts',(29.4248189653411,2.82352034684489,-1.55683114895389));
#72477=CARTESIAN_POINT('Ctrl Pts',(29.4309912134339,2.87028719342223,-1.46884469800217));
#72478=CARTESIAN_POINT('Ctrl Pts',(29.4371634615267,2.91293130511126,-1.37874898883112));
#72479=CARTESIAN_POINT('Ctrl Pts',(29.4433273501793,2.95551766136126,-1.28877530160005));
#72480=CARTESIAN_POINT('Ctrl Pts',(29.4494912388319,2.9939921966713,-1.19669842330112));
#72481=CARTESIAN_POINT('Ctrl Pts',(29.4556551274846,3.0281449442721,-1.10293053225455));
#72482=CARTESIAN_POINT('Ctrl Pts',(29.4618124891431,3.06226152723814,-1.00926193282493));
#72483=CARTESIAN_POINT('Ctrl Pts',(29.4679698508016,3.09206527292834,-0.91390628647984));
#72484=CARTESIAN_POINT('Ctrl Pts',(29.4741272124602,3.11739353567447,-0.817297440492172));
#72485=CARTESIAN_POINT('Ctrl Pts',(29.4802800766065,3.14270329793646,-0.720759160355769));
#72486=CARTESIAN_POINT('Ctrl Pts',(29.4864329407528,3.16354396679903,-0.622969919402475));
#72487=CARTESIAN_POINT('Ctrl Pts',(29.4925858048991,3.17980244518916,-0.524379606839389));
#72488=CARTESIAN_POINT('Ctrl Pts',(29.4987363380356,3.1960547640622,-0.425826645171083));
#72489=CARTESIAN_POINT('Ctrl Pts',(29.5048868711722,3.20772827120792,-0.326473643028091));
#72490=CARTESIAN_POINT('Ctrl Pts',(29.5110374043087,3.21476096630608,-0.22678071349838));
#72491=CARTESIAN_POINT('Ctrl Pts',(29.5171872525239,3.22179287824564,-0.127098885740212));
#72492=CARTESIAN_POINT('Ctrl Pts',(29.5233371007391,3.22418497504372,-0.0270776391539264));
#72493=CARTESIAN_POINT('Ctrl Pts',(29.5294869489544,3.22192721670464,0.0728187665226462));
#72494=CARTESIAN_POINT('Ctrl Pts',(29.5356377573335,3.21966910586612,0.172730768832007));
#72495=CARTESIAN_POINT('Ctrl Pts',(29.5417885657126,3.21275970773648,0.272517457211904));
#72496=CARTESIAN_POINT('Ctrl Pts',(29.5479393740917,3.20124106551578,0.371716562659478));
#72497=CARTESIAN_POINT('Ctrl Pts',(29.5540967604579,3.18971010467375,0.471021756671506));
#72498=CARTESIAN_POINT('Ctrl Pts',(29.5602541468241,3.17356010651732,0.56973768060177));
#72499=CARTESIAN_POINT('Ctrl Pts',(29.5664115331903,3.15288477541773,0.667409286299719));
#72500=CARTESIAN_POINT('Ctrl Pts',(29.5725723559272,3.13219790563933,0.765135401465064));
#72501=CARTESIAN_POINT('Ctrl Pts',(29.5787331786642,3.10698078297506,0.861815617387977));
#72502=CARTESIAN_POINT('Ctrl Pts',(29.5848940014011,3.07737729028909,0.957009182669087));
#72503=CARTESIAN_POINT('Ctrl Pts',(29.5910651243178,3.04772430400328,1.05236190052986));
#72504=CARTESIAN_POINT('Ctrl Pts',(29.5972362472345,3.01367044747031,1.14622259450404));
#72505=CARTESIAN_POINT('Ctrl Pts',(29.6034073701512,2.9754081722579,1.23816952432246));
#72506=CARTESIAN_POINT('Ctrl Pts',(29.6081028920968,2.94629493705372,1.30813066958225));
#72507=CARTESIAN_POINT('Ctrl Pts',(29.6127984140423,2.91474625366956,1.37698424031645));
#72508=CARTESIAN_POINT('Ctrl Pts',(29.6174939359879,2.88086430806338,1.44455474144336));
#72509=CARTESIAN_POINT('Ctrl Pts',(29.6236660414796,2.8363276314235,1.53337388996756));
#72510=CARTESIAN_POINT('Ctrl Pts',(29.6298381469713,2.78760118013189,1.62028778915822));
#72511=CARTESIAN_POINT('Ctrl Pts',(29.636010252463,2.73487137736418,1.70487422168737));
#72512=CARTESIAN_POINT('Ctrl Pts',(29.6421743238165,2.68221021219859,1.789350549312));
#72513=CARTESIAN_POINT('Ctrl Pts',(29.64833839517,2.62555627850347,1.87150506521703));
#72514=CARTESIAN_POINT('Ctrl Pts',(29.6545024665236,2.56514279352223,1.95093823873053));
#72515=CARTESIAN_POINT('Ctrl Pts',(29.6606592480018,2.50480075592461,2.03027747142233));
#72516=CARTESIAN_POINT('Ctrl Pts',(29.6668160294801,2.4407082733548,2.10690142022294));
#72517=CARTESIAN_POINT('Ctrl Pts',(29.6729728109583,2.3731422778064,2.18043878423308));
#72518=CARTESIAN_POINT('Ctrl Pts',(29.6791253500184,2.30562283957199,2.25392547627254));
#72519=CARTESIAN_POINT('Ctrl Pts',(29.6852778890784,2.23463493812672,2.32432949173243));
#72520=CARTESIAN_POINT('Ctrl Pts',(29.6914304281385,2.16049581681903,2.39131248230077));
#72521=CARTESIAN_POINT('Ctrl Pts',(29.6975807723252,2.08638314410144,2.45827157717639));
#72522=CARTESIAN_POINT('Ctrl Pts',(29.7037311165119,2.00912180615334,2.52181178025222));
#72523=CARTESIAN_POINT('Ctrl Pts',(29.7098814606986,1.92906529208145,2.58163217004024));
#72524=CARTESIAN_POINT('Ctrl Pts',(29.7133891323447,1.88340736530937,2.61574900622882));
#72525=CARTESIAN_POINT('Ctrl Pts',(29.7168968039908,1.83684090763758,2.64865661731778));
#72526=CARTESIAN_POINT('Ctrl Pts',(29.720404475637,1.78943621037806,2.68030513402631));
#72527=CARTESIAN_POINT('Origin',(-1.72497344927317,0.,0.));
#72528=CARTESIAN_POINT('',(31.2170551299057,1.78943621037803,2.68030513402633));
#72529=CARTESIAN_POINT('',(30.9709191047552,1.78943620529092,2.68030513742261));
#72530=CARTESIAN_POINT('',(-1.72497344927317,1.78943621037804,2.68030513402633));
#72531=CARTESIAN_POINT('',(30.3965734492365,-3.22274997554544,-0.000397016205367042));
#72532=CARTESIAN_POINT('Ctrl Pts',(30.3965734492731,-3.22274997554537,-0.000397016795153058));
#72533=CARTESIAN_POINT('Ctrl Pts',(30.3978870394267,-3.22274737029783,-0.0215448914758832));
#72534=CARTESIAN_POINT('Ctrl Pts',(30.3992006295803,-3.22253660744666,-0.0426913043998582));
#72535=CARTESIAN_POINT('Ctrl Pts',(30.4005142197338,-3.22211775644669,-0.0638335812169476));
#72536=CARTESIAN_POINT('Ctrl Pts',(30.4066864678266,-3.22014967509443,-0.163176117705557));
#72537=CARTESIAN_POINT('Ctrl Pts',(30.4128587159193,-3.21357951462047,-0.262602404376855));
#72538=CARTESIAN_POINT('Ctrl Pts',(30.4190309640121,-3.20239380316626,-0.361651063792674));
#72539=CARTESIAN_POINT('Ctrl Pts',(30.4251948526647,-3.1912232411817,-0.460565575759197));
#72540=CARTESIAN_POINT('Ctrl Pts',(30.4313587413174,-3.17544960130822,-0.559103049188145));
#72541=CARTESIAN_POINT('Ctrl Pts',(30.43752262997,-3.15511141149656,-0.656802514873532));
#72542=CARTESIAN_POINT('Ctrl Pts',(30.4436799916286,-3.134794757967,-0.754398525764095));
#72543=CARTESIAN_POINT('Ctrl Pts',(30.4498373532871,-3.10992325187422,-0.851157870179716));
#72544=CARTESIAN_POINT('Ctrl Pts',(30.4559947149457,-3.08058706074934,-0.946626073824156));
#72545=CARTESIAN_POINT('Ctrl Pts',(30.462147579092,-3.05127229761354,-1.04202454477506));
#72546=CARTESIAN_POINT('Ctrl Pts',(30.4683004432383,-3.01749946034137,-1.13613333600877));
#72547=CARTESIAN_POINT('Ctrl Pts',(30.4744533073846,-2.97940928686148,-1.22851042480867));
#72548=CARTESIAN_POINT('Ctrl Pts',(30.4806038405211,-2.9413335438264,-1.32085251659069));
#72549=CARTESIAN_POINT('Ctrl Pts',(30.4867543736577,-2.89894387995318,-1.41146380838497));
#72550=CARTESIAN_POINT('Ctrl Pts',(30.4929049067942,-2.85242985626061,-1.49992049043043));
#72551=CARTESIAN_POINT('Ctrl Pts',(30.4990547550094,-2.8059210123543,-1.58836732196911));
#72552=CARTESIAN_POINT('Ctrl Pts',(30.5052046032246,-2.75528892392457,-1.67465963632566));
#72553=CARTESIAN_POINT('Ctrl Pts',(30.5113544514398,-2.70076950930567,-1.75839745794425));
#72554=CARTESIAN_POINT('Ctrl Pts',(30.517505259819,-2.6462415826758,-1.8421483533873));
#72555=CARTESIAN_POINT('Ctrl Pts',(30.5236560681981,-2.58782536138163,-1.92334359986204));
#72556=CARTESIAN_POINT('Ctrl Pts',(30.5298068765773,-2.52579999391996,-2.0016123383947));
#72557=CARTESIAN_POINT('Ctrl Pts',(30.5359642629434,-2.46370829337835,-2.07996478149378));
#72558=CARTESIAN_POINT('Ctrl Pts',(30.5421216493096,-2.39800000935009,-2.15538412574944));
#72559=CARTESIAN_POINT('Ctrl Pts',(30.5482790356758,-2.32899440781758,-2.22753285292371));
#72560=CARTESIAN_POINT('Ctrl Pts',(30.5544398584128,-2.25995029500473,-2.29972184552276));
#72561=CARTESIAN_POINT('Ctrl Pts',(30.5606006811498,-2.18760551448642,-2.36863628637636));
#72562=CARTESIAN_POINT('Ctrl Pts',(30.5667615038867,-2.11231446345453,-2.43397723283945));
#72563=CARTESIAN_POINT('Ctrl Pts',(30.5729326268034,-2.03689753453418,-2.49942742177238));
#72564=CARTESIAN_POINT('Ctrl Pts',(30.5791037497201,-1.95852483703355,-2.56129191324031));
#72565=CARTESIAN_POINT('Ctrl Pts',(30.5852748726368,-1.87758204846191,-2.61931350047939));
#72566=CARTESIAN_POINT('Ctrl Pts',(30.5899703945824,-1.81599380184881,-2.66346132250063));
#72567=CARTESIAN_POINT('Ctrl Pts',(30.5946659165279,-1.75291825438787,-2.70538516939721));
#72568=CARTESIAN_POINT('Ctrl Pts',(30.5993614384735,-1.68853468528847,-2.74498965008573));
#72569=CARTESIAN_POINT('Ctrl Pts',(30.6055336865663,-1.60390269630269,-2.79704960917627));
#72570=CARTESIAN_POINT('Ctrl Pts',(30.611705934659,-1.51671186461396,-2.8452835428674));
#72571=CARTESIAN_POINT('Ctrl Pts',(30.6178781827518,-1.42734302066416,-2.88943064700666));
#72572=CARTESIAN_POINT('Ctrl Pts',(30.6240420714044,-1.33809521421804,-2.93351796011536));
#72573=CARTESIAN_POINT('Ctrl Pts',(30.6302059600571,-1.24667564460432,-2.97352925447361));
#72574=CARTESIAN_POINT('Ctrl Pts',(30.6363698487097,-1.15349291568567,-3.00924768936739));
#72575=CARTESIAN_POINT('Ctrl Pts',(30.6425272103682,-1.06040885875063,-3.04492830170689));
#72576=CARTESIAN_POINT('Ctrl Pts',(30.6486845720268,-0.965565757693471,
-3.07632493733784));
#72577=CARTESIAN_POINT('Ctrl Pts',(30.6548419336853,-0.869394674850752,
-3.10326770708574));
#72578=CARTESIAN_POINT('Ctrl Pts',(30.6609947978316,-0.773293838104692,
-3.13019079706761));
#72579=CARTESIAN_POINT('Ctrl Pts',(30.6671476619779,-0.675867365100445,
-3.15266637231773));
#72580=CARTESIAN_POINT('Ctrl Pts',(30.6733005261242,-0.577563187726553,
-3.17057381662739));
#72581=CARTESIAN_POINT('Ctrl Pts',(30.6794510592608,-0.479296252845346,
-3.18847447670994));
#72582=CARTESIAN_POINT('Ctrl Pts',(30.6856015923973,-0.380152701174109,
-3.20181036685319));
#72583=CARTESIAN_POINT('Ctrl Pts',(30.6917521255338,-0.280591542845579,
-3.21051178919865));
#72584=CARTESIAN_POINT('Ctrl Pts',(30.6979019737491,-0.181041471614624,
-3.21921224255661));
#72585=CARTESIAN_POINT('Ctrl Pts',(30.7040518219643,-0.0810743189103917,
-3.22327921636538));
#72586=CARTESIAN_POINT('Ctrl Pts',(30.7102016701795,0.018845888805191,-3.2226948963523));
#72587=CARTESIAN_POINT('Ctrl Pts',(30.7163524785586,0.118781696869881,-3.22211048511046));
#72588=CARTESIAN_POINT('Ctrl Pts',(30.7225032869377,0.218670110979054,-3.21687334017127));
#72589=CARTESIAN_POINT('Ctrl Pts',(30.7286540953169,0.318048222807609,-3.20701775649417));
#72590=CARTESIAN_POINT('Ctrl Pts',(30.734811481683,0.417532614639169,-3.19715163275505));
#72591=CARTESIAN_POINT('Ctrl Pts',(30.7409688680492,0.51650518129978,-3.18265725017103));
#72592=CARTESIAN_POINT('Ctrl Pts',(30.7471262544154,0.614509369053244,-3.16362067856527));
#72593=CARTESIAN_POINT('Ctrl Pts',(30.7532870771524,0.712568251884493,-3.14457348285468));
#72594=CARTESIAN_POINT('Ctrl Pts',(30.7594478998893,0.809657257422227,-3.12097915239011));
#72595=CARTESIAN_POINT('Ctrl Pts',(30.7656087226263,0.905333286258208,-3.09297416789939));
#72596=CARTESIAN_POINT('Ctrl Pts',(30.771779845543,1.00116927429686,-3.06492236232878));
#72597=CARTESIAN_POINT('Ctrl Pts',(30.7779509684597,1.09558715600064,-3.03244531454632));
#72598=CARTESIAN_POINT('Ctrl Pts',(30.7841220913764,1.18816202696872,-2.99572838557997));
#72599=CARTESIAN_POINT('Ctrl Pts',(30.788817613322,1.25860096395163,-2.96779098292825));
#72600=CARTESIAN_POINT('Ctrl Pts',(30.7935131352676,1.32797327203204,-2.93739992342364));
#72601=CARTESIAN_POINT('Ctrl Pts',(30.7982086572132,1.39610176927607,-2.90465443939967));
#72602=CARTESIAN_POINT('Ctrl Pts',(30.8043809053059,1.48565645394122,-2.86161060877664));
#72603=CARTESIAN_POINT('Ctrl Pts',(30.8105531533987,1.57337624438467,-2.81434548575309));
#72604=CARTESIAN_POINT('Ctrl Pts',(30.8167254014915,1.65883583090921,-2.76303840881587));
#72605=CARTESIAN_POINT('Ctrl Pts',(30.8228892901441,1.7441796744684,-2.7118008200832));
#72606=CARTESIAN_POINT('Ctrl Pts',(30.8290531787967,1.82726902930238,-2.65653237974099));
#72607=CARTESIAN_POINT('Ctrl Pts',(30.8352170674494,1.90770055077724,-2.59745956100653));
#72608=CARTESIAN_POINT('Ctrl Pts',(30.8413744291079,1.98804690263037,-2.53844929498192));
#72609=CARTESIAN_POINT('Ctrl Pts',(30.8475317907664,2.06574066825636,-2.47564291529061));
#72610=CARTESIAN_POINT('Ctrl Pts',(30.853689152425,2.14040585554809,-2.40931117459648));
#72611=CARTESIAN_POINT('Ctrl Pts',(30.8598420165713,2.21501650526149,-2.34302788449404));
#72612=CARTESIAN_POINT('Ctrl Pts',(30.8659948807176,2.28660265103505,-2.27322464059985));
#72613=CARTESIAN_POINT('Ctrl Pts',(30.8721477448639,2.35482062808022,-2.20021302879241));
#72614=CARTESIAN_POINT('Ctrl Pts',(30.8782982780005,2.42301276077596,-2.12722907740074));
#72615=CARTESIAN_POINT('Ctrl Pts',(30.884448811137,2.48783896398199,-2.05103949030523));
#72616=CARTESIAN_POINT('Ctrl Pts',(30.8905993442735,2.54899241575982,-1.97199270457548));
#72617=CARTESIAN_POINT('Ctrl Pts',(30.8967491924887,2.61013905750953,-1.89295472146958));
#72618=CARTESIAN_POINT('Ctrl Pts',(30.9028990407039,2.6676134951822,-1.81106051587506));
#72619=CARTESIAN_POINT('Ctrl Pts',(30.9090488889191,2.72114983939361,-1.72669079862844));
#72620=CARTESIAN_POINT('Ctrl Pts',(30.9151996972983,2.77469454213108,-1.64230790890077));
#72621=CARTESIAN_POINT('Ctrl Pts',(30.9213505056774,2.82429969741022,-1.55544910664051));
#72622=CARTESIAN_POINT('Ctrl Pts',(30.9275013140565,2.86974385518543,-1.46652233809289));
#72623=CARTESIAN_POINT('Ctrl Pts',(30.9336587004227,2.91523661325236,-1.3775004667399));
#72624=CARTESIAN_POINT('Ctrl Pts',(30.9398160867889,2.95655928961141,-1.28640660033605));
#72625=CARTESIAN_POINT('Ctrl Pts',(30.9459734731551,2.99353742368518,-1.19367133478872));
#72626=CARTESIAN_POINT('Ctrl Pts',(30.9521342958921,3.03053619485585,-1.10088431469213));
#72627=CARTESIAN_POINT('Ctrl Pts',(30.958295118629,3.06318545315432,-1.00645448169995));
#72628=CARTESIAN_POINT('Ctrl Pts',(30.964455941366,3.09136041899844,-0.910828371511226));
#72629=CARTESIAN_POINT('Ctrl Pts',(30.9706270642827,3.11958249011152,-0.815042385578012));
#72630=CARTESIAN_POINT('Ctrl Pts',(30.9767981871994,3.14331522341325,-0.718056549559979));
#72631=CARTESIAN_POINT('Ctrl Pts',(30.982969310116,3.16248479609247,-0.620328523432538));
#72632=CARTESIAN_POINT('Ctrl Pts',(30.9876648320616,3.17707065840917,-0.545968622070545));
#72633=CARTESIAN_POINT('Ctrl Pts',(30.9923603540072,3.18901574554004,-0.471179261065576));
#72634=CARTESIAN_POINT('Ctrl Pts',(30.9970558759527,3.19830772852275,-0.396163143378616));
#72635=CARTESIAN_POINT('Ctrl Pts',(31.0032281240455,3.21052200947129,-0.297554704383292));
#72636=CARTESIAN_POINT('Ctrl Pts',(31.0094003721383,3.21819315552981,-0.198207298740116));
#72637=CARTESIAN_POINT('Ctrl Pts',(31.015572620231,3.22124205852399,-0.0985756709137832));
#72638=CARTESIAN_POINT('Ctrl Pts',(31.0217365088837,3.22428683220878,0.000921019914584459));
#72639=CARTESIAN_POINT('Ctrl Pts',(31.0279003975363,3.22272179245018,0.100700737468478));
#72640=CARTESIAN_POINT('Ctrl Pts',(31.0340642861889,3.2165193579639,0.200301728258884));
#72641=CARTESIAN_POINT('Ctrl Pts',(31.0402216478475,3.21032349128822,0.299797250713579));
#72642=CARTESIAN_POINT('Ctrl Pts',(31.046379009506,3.19950001942366,0.399113991517258));
#72643=CARTESIAN_POINT('Ctrl Pts',(31.0525363711645,3.18407339914241,0.497789264020125));
#72644=CARTESIAN_POINT('Ctrl Pts',(31.0586892353109,3.16865804690377,0.596392461294946));
#72645=CARTESIAN_POINT('Ctrl Pts',(31.0648420994572,3.14864629790938,0.694354693951464));
#72646=CARTESIAN_POINT('Ctrl Pts',(31.0709949636035,3.12411443790773,0.791218390431176));
#72647=CARTESIAN_POINT('Ctrl Pts',(31.07714549674,3.09959187179002,0.888045390143763));
#72648=CARTESIAN_POINT('Ctrl Pts',(31.0832960298766,3.07055270380325,0.983774260013495));
#72649=CARTESIAN_POINT('Ctrl Pts',(31.0894465630131,3.03712414055262,1.07795849519938));
#72650=CARTESIAN_POINT('Ctrl Pts',(31.0955964112283,3.0036992998957,1.17213224206007));
#72651=CARTESIAN_POINT('Ctrl Pts',(31.1017462594435,2.9658861810757,1.26476128686167));
#72652=CARTESIAN_POINT('Ctrl Pts',(31.1078961076587,2.92386127232947,1.35541610683653));
#72653=CARTESIAN_POINT('Ctrl Pts',(31.1140469160379,2.88182980231534,1.44608508057347));
#72654=CARTESIAN_POINT('Ctrl Pts',(31.120197724417,2.83558541895962,1.53477882312855));
#72655=CARTESIAN_POINT('Ctrl Pts',(31.1263485327961,2.78535154997316,1.62109046803753));
#72656=CARTESIAN_POINT('Ctrl Pts',(31.1325059191623,2.73506395833447,1.70749441900567));
#72657=CARTESIAN_POINT('Ctrl Pts',(31.1386633055285,2.68077858011121,1.79151080900805));
#72658=CARTESIAN_POINT('Ctrl Pts',(31.1448206918947,2.62276330379848,1.87276005263571));
#72659=CARTESIAN_POINT('Ctrl Pts',(31.1509815146316,2.56471564978715,1.95405464058799));
#72660=CARTESIAN_POINT('Ctrl Pts',(31.1571423373686,2.50293422077824,2.03257866529377));
#72661=CARTESIAN_POINT('Ctrl Pts',(31.1633031601056,2.43772717698457,2.10798571463159));
#72662=CARTESIAN_POINT('Ctrl Pts',(31.1694742830222,2.37241111459072,2.18351883579362));
#72663=CARTESIAN_POINT('Ctrl Pts',(31.1756454059389,2.30365829668805,2.25592425719654));
#72664=CARTESIAN_POINT('Ctrl Pts',(31.1818165288556,2.23181379417764,2.32489241699877));
#72665=CARTESIAN_POINT('Ctrl Pts',(31.1865120508012,2.17714830739939,2.37736933445314));
#72666=CARTESIAN_POINT('Ctrl Pts',(31.1912075727468,2.12069366115876,2.42785702150719));
#72667=CARTESIAN_POINT('Ctrl Pts',(31.1959030946924,2.06261370459727,2.47623550336141));
#72668=CARTESIAN_POINT('Ctrl Pts',(31.2020759937542,1.98625974149879,2.53983556501688));
#72669=CARTESIAN_POINT('Ctrl Pts',(31.2082488928159,1.90682698354292,2.60001274540606));
#72670=CARTESIAN_POINT('Ctrl Pts',(31.2144217918776,1.82465530069742,2.6564545161054));
#72671=CARTESIAN_POINT('Ctrl Pts',(31.2152995712203,1.81297057929927,2.66448047277323));
#72672=CARTESIAN_POINT('Ctrl Pts',(31.216177350563,1.80123053679588,2.67243095787333));
#72673=CARTESIAN_POINT('Ctrl Pts',(31.2170551299057,1.78943621037803,2.68030513402633));
#72674=CARTESIAN_POINT('Ctrl Pts',(29.9668448649094,1.78943621037805,2.68030513402632));
#72675=CARTESIAN_POINT('Ctrl Pts',(29.9730155973569,1.70635742939051,2.73577052754659));
#72676=CARTESIAN_POINT('Ctrl Pts',(29.9791863298045,1.62079052020137,2.78730753432573));
#72677=CARTESIAN_POINT('Ctrl Pts',(29.9853570622521,1.53315005596254,2.83470782769619));
#72678=CARTESIAN_POINT('Ctrl Pts',(29.9911779689196,1.45047802845725,2.87942094499099));
#72679=CARTESIAN_POINT('Ctrl Pts',(29.9969988755871,1.36596137328465,2.92045337514309));
#72680=CARTESIAN_POINT('Ctrl Pts',(30.0028197822546,1.27996288185344,2.95767012757972));
#72681=CARTESIAN_POINT('Ctrl Pts',(30.0089920303474,1.18877364707692,2.99713322883979));
#72682=CARTESIAN_POINT('Ctrl Pts',(30.0151642784402,1.09559714290483,3.03244459471753));
#72683=CARTESIAN_POINT('Ctrl Pts',(30.0213365265329,1.00084749025507,3.06340037601195));
#72684=CARTESIAN_POINT('Ctrl Pts',(30.0275004151856,0.906226162655928,3.09431423206347));
#72685=CARTESIAN_POINT('Ctrl Pts',(30.0336643038382,0.810036330658838,3.12088409478352));
#72686=CARTESIAN_POINT('Ctrl Pts',(30.0398281924908,0.712713337506968,3.14295358875051));
#72687=CARTESIAN_POINT('Ctrl Pts',(30.0459855541494,0.615493400499778,3.16499971314274));
#72688=CARTESIAN_POINT('Ctrl Pts',(30.0521429158079,0.517143109164207,3.18255484747094));
#72689=CARTESIAN_POINT('Ctrl Pts',(30.0583002774665,0.418113342424336,3.19551228997586));
#72690=CARTESIAN_POINT('Ctrl Pts',(30.0644531416128,0.319155909845194,3.20846026799591));
#72691=CARTESIAN_POINT('Ctrl Pts',(30.0706060057591,0.219520418012922,3.21681717485254));
#72692=CARTESIAN_POINT('Ctrl Pts',(30.0767588699054,0.119667418752613,3.22052748340844));
#72693=CARTESIAN_POINT('Ctrl Pts',(30.0829094030419,0.0198522487554531,
3.22423638631563));
#72694=CARTESIAN_POINT('Ctrl Pts',(30.0890599361785,-0.0801798313424153,
3.2233021726398));
#72695=CARTESIAN_POINT('Ctrl Pts',(30.095210469315,-0.179964563537114,3.21772129283611));
#72696=CARTESIAN_POINT('Ctrl Pts',(30.1013603175302,-0.279738183737156,
3.21214103451735));
#72697=CARTESIAN_POINT('Ctrl Pts',(30.1075101657454,-0.379264077098757,
3.20191516309571));
#72698=CARTESIAN_POINT('Ctrl Pts',(30.1136600139606,-0.478080417042818,
3.18709219780981));
#72699=CARTESIAN_POINT('Ctrl Pts',(30.1198108223397,-0.576912184991273,
3.17226691824295));
#72700=CARTESIAN_POINT('Ctrl Pts',(30.1259616307189,-0.675033749872496,
3.15284318364763));
#72701=CARTESIAN_POINT('Ctrl Pts',(30.132112439098,-0.771991820509954,3.12892093085871));
#72702=CARTESIAN_POINT('Ctrl Pts',(30.1382698254642,-0.869053583035296,
3.10497309439699));
#72703=CARTESIAN_POINT('Ctrl Pts',(30.1444272118304,-0.964948944027739,
3.07651723703857));
#72704=CARTESIAN_POINT('Ctrl Pts',(30.1505845981966,-1.05923828301367,3.04370363575336));
#72705=CARTESIAN_POINT('Ctrl Pts',(30.1567454209335,-1.15358024386045,3.01087172155198));
#72706=CARTESIAN_POINT('Ctrl Pts',(30.1629062436705,-1.24631399455558,2.97367738181617));
#72707=CARTESIAN_POINT('Ctrl Pts',(30.1690670664074,-1.33702041810612,2.93231887148504));
#72708=CARTESIAN_POINT('Ctrl Pts',(30.1752381893241,-1.42787849225677,2.8908912145305));
#72709=CARTESIAN_POINT('Ctrl Pts',(30.1814093122408,-1.51670208233278,2.84528567907598));
#72710=CARTESIAN_POINT('Ctrl Pts',(30.1875804351575,-1.60309704887808,2.79574630722789));
#72711=CARTESIAN_POINT('Ctrl Pts',(30.192275957103,-1.66883378218812,2.75805248540301));
#72712=CARTESIAN_POINT('Ctrl Pts',(30.1969714790486,-1.73316498791198,2.71808212643338));
#72713=CARTESIAN_POINT('Ctrl Pts',(30.2016670009941,-1.79592944037064,2.67595870814742));
#72714=CARTESIAN_POINT('Ctrl Pts',(30.207818424657,-1.87815474833823,2.62077442937924));
#72715=CARTESIAN_POINT('Ctrl Pts',(30.2139698483198,-1.95798373458385,2.56169632975944));
#72716=CARTESIAN_POINT('Ctrl Pts',(30.2201212719827,-2.03502252916728,2.49895995731857));
#72717=CARTESIAN_POINT('Ctrl Pts',(30.2262643515467,-2.11195682447542,2.43630868363202));
#72718=CARTESIAN_POINT('Ctrl Pts',(30.2324074311108,-2.18610811322559,2.37000927244701));
#72719=CARTESIAN_POINT('Ctrl Pts',(30.2385505106748,-2.25711084438849,2.30034088748687));
#72720=CARTESIAN_POINT('Ctrl Pts',(30.2446871053043,-2.32803862160367,2.23074604787349));
#72721=CARTESIAN_POINT('Ctrl Pts',(30.2508236999338,-2.39582413755272,2.1577896088));
#72722=CARTESIAN_POINT('Ctrl Pts',(30.2569602945633,-2.46013513106599,2.08179074342137));
#72723=CARTESIAN_POINT('Ctrl Pts',(30.2630924739142,-2.5243998528322,2.00584655921129));
#72724=CARTESIAN_POINT('Ctrl Pts',(30.269224653265,-2.58519473974204,1.92686463325162));
#72725=CARTESIAN_POINT('Ctrl Pts',(30.2753568326159,-2.64222529150039,1.84520000852365));
#72726=CARTESIAN_POINT('Ctrl Pts',(30.281486766945,-2.69923496408644,1.7635652816262));
#72727=CARTESIAN_POINT('Ctrl Pts',(30.2876167012741,-2.75248278917626,1.67925016568173));
#72728=CARTESIAN_POINT('Ctrl Pts',(30.2937466356033,-2.80171596576564,1.59264095441312));
#72729=CARTESIAN_POINT('Ctrl Pts',(30.2998759946897,-2.85094452223643,1.50603987068885));
#72730=CARTESIAN_POINT('Ctrl Pts',(30.3060053537762,-2.89615896302052,1.41714550021788));
#72731=CARTESIAN_POINT('Ctrl Pts',(30.3121347128627,-2.93715160641279,1.32637023618852));
#72732=CARTESIAN_POINT('Ctrl Pts',(30.3182651655735,-2.97815156387378,1.23557877567937));
#72733=CARTESIAN_POINT('Ctrl Pts',(30.3243956182843,-3.01492804798627,1.14290615409432));
#72734=CARTESIAN_POINT('Ctrl Pts',(30.3305260709951,-3.04732126375728,1.04878533454314));
#72735=CARTESIAN_POINT('Ctrl Pts',(30.3366630861763,-3.07974915551832,0.954563761407506));
#72736=CARTESIAN_POINT('Ctrl Pts',(30.3428001013574,-3.10778426918983,0.858891310021853));
#72737=CARTESIAN_POINT('Ctrl Pts',(30.3489371165386,-3.13131658115752,0.762216525055679));
#72738=CARTESIAN_POINT('Ctrl Pts',(30.3550777343895,-3.15486270751969,0.665484988181035));
#72739=CARTESIAN_POINT('Ctrl Pts',(30.3612183522404,-3.17390068635141,0.567750375655364));
#72740=CARTESIAN_POINT('Ctrl Pts',(30.3673589700913,-3.18837194979263,0.469469777808461));
#72741=CARTESIAN_POINT('Ctrl Pts',(30.3735094707065,-3.20286650341247,0.371031006303314));
#72742=CARTESIAN_POINT('Ctrl Pts',(30.3796599713218,-3.21277962373837,0.272044930090738));
#72743=CARTESIAN_POINT('Ctrl Pts',(30.3858104719371,-3.21810475772262,0.17297205214433));
#72744=CARTESIAN_POINT('Ctrl Pts',(30.3893981310369,-3.22121097079231,0.115181681190473));
#72745=CARTESIAN_POINT('Ctrl Pts',(30.3929857901367,-3.22275709095059,0.0573617640601762));
#72746=CARTESIAN_POINT('Ctrl Pts',(30.3965734492365,-3.22274997554544,-0.000397016205362354));
#72747=CARTESIAN_POINT('',(30.1500265507269,-3.22274893555634,-0.00261932634679408));
#72748=CARTESIAN_POINT('Ctrl Pts',(29.720404475637,1.78943621037806,2.68030513402631));
#72749=CARTESIAN_POINT('Ctrl Pts',(29.7265546697647,1.70631894054126,2.7357962236286));
#72750=CARTESIAN_POINT('Ctrl Pts',(29.7327048638924,1.6206233134869,2.78741395090235));
#72751=CARTESIAN_POINT('Ctrl Pts',(29.7388550580201,1.53275019332222,2.83492405672016));
#72752=CARTESIAN_POINT('Ctrl Pts',(29.7453122327457,1.44049097697766,2.88480558047833));
#72753=CARTESIAN_POINT('Ctrl Pts',(29.7517694074713,1.34583171789474,2.93015853342363));
#72754=CARTESIAN_POINT('Ctrl Pts',(29.7582265821969,1.24926354461491,2.97076726765935));
#72755=CARTESIAN_POINT('Ctrl Pts',(29.764385922519,1.15714953674241,3.0095029415158));
#72756=CARTESIAN_POINT('Ctrl Pts',(29.7705452628411,1.06329923530287,3.04392222124192));
#72757=CARTESIAN_POINT('Ctrl Pts',(29.7767046031631,0.968156156258745,3.07388861535325));
#72758=CARTESIAN_POINT('Ctrl Pts',(29.7828682965992,0.872945834840306,3.10387618821461));
#72759=CARTESIAN_POINT('Ctrl Pts',(29.7890319900352,0.776441336148424,3.12940450066375));
#72760=CARTESIAN_POINT('Ctrl Pts',(29.7951956834712,0.679097560101669,3.15038792315549));
#72761=CARTESIAN_POINT('Ctrl Pts',(29.8013685837513,0.58160837952145,3.17140268904566));
#72762=CARTESIAN_POINT('Ctrl Pts',(29.8075414840315,0.483277847267676,3.18785895065528));
#72763=CARTESIAN_POINT('Ctrl Pts',(29.8137143843116,0.384566885514254,3.19972278065864));
#72764=CARTESIAN_POINT('Ctrl Pts',(29.8145899744502,0.370565307525707,3.201405596205));
#72765=CARTESIAN_POINT('Ctrl Pts',(29.8154655645889,0.356556075577454,3.20299609869579));
#72766=CARTESIAN_POINT('Ctrl Pts',(29.8163411547275,0.342540503666624,3.20449427614527));
#72767=CARTESIAN_POINT('Ctrl Pts',(29.8225134028203,0.243741324487471,3.21505529379159));
#72768=CARTESIAN_POINT('Ctrl Pts',(29.8286856509131,0.144279373311957,3.2210614371678));
#72769=CARTESIAN_POINT('Ctrl Pts',(29.8348578990058,0.044610655767646,3.22244122551397));
#72770=CARTESIAN_POINT('Ctrl Pts',(29.8410217876585,-0.0549230745456297,
3.22381914513128));
#72771=CARTESIAN_POINT('Ctrl Pts',(29.8471856763111,-0.154662584116093,
3.22058315761827));
#72772=CARTESIAN_POINT('Ctrl Pts',(29.8533495649637,-0.254145722276558,
3.2127134192686));
#72773=CARTESIAN_POINT('Ctrl Pts',(29.8595069266223,-0.353523516896889,
3.20485201425172));
#72774=CARTESIAN_POINT('Ctrl Pts',(29.8656642882808,-0.452645049188138,
3.19236664748308));
#72775=CARTESIAN_POINT('Ctrl Pts',(29.8718216499394,-0.5510481070161,3.17528952164271));
#72776=CARTESIAN_POINT('Ctrl Pts',(29.8779745140857,-0.649379288449273,
3.15822486942121));
#72777=CARTESIAN_POINT('Ctrl Pts',(29.884127378232,-0.746992612111663,3.13657520040593));
#72778=CARTESIAN_POINT('Ctrl Pts',(29.8902802423783,-0.843431848303963,
3.11042445331285));
#72779=CARTESIAN_POINT('Ctrl Pts',(29.8964307755149,-0.939834548535634,
3.08428361341839));
#72780=CARTESIAN_POINT('Ctrl Pts',(29.9025813086514,-1.03506362634721,3.0536451972866));
#72781=CARTESIAN_POINT('Ctrl Pts',(29.9087318417879,-1.12867477005597,3.01864387199602));
#72782=CARTESIAN_POINT('Ctrl Pts',(29.9148816900032,-1.2222754892591,2.9836464444413));
#72783=CARTESIAN_POINT('Ctrl Pts',(29.9210315382184,-1.31425822570343,2.94428722580029));
#72784=CARTESIAN_POINT('Ctrl Pts',(29.9271813864336,-1.40419647279428,2.90074987344516));
#72785=CARTESIAN_POINT('Ctrl Pts',(29.9333321948127,-1.49414876176942,2.85720572368755));
#72786=CARTESIAN_POINT('Ctrl Pts',(29.9394830031919,-1.58205553636154,2.80948233381311));
#72787=CARTESIAN_POINT('Ctrl Pts',(29.945633811571,-1.66751372927036,2.75780991462335));
#72788=CARTESIAN_POINT('Ctrl Pts',(29.9517911979372,-1.7530633155138,2.70608223432244));
#72789=CARTESIAN_POINT('Ctrl Pts',(29.9579485843034,-1.83615871849149,2.65039731641945));
#72790=CARTESIAN_POINT('Ctrl Pts',(29.9641059706696,-1.91642489278621,2.59102936934519));
#72791=CARTESIAN_POINT('Ctrl Pts',(29.9702667934065,-1.99673586276528,2.53162828966134));
#72792=CARTESIAN_POINT('Ctrl Pts',(29.9764276161435,-2.07421412273621,2.46854036166959));
#72793=CARTESIAN_POINT('Ctrl Pts',(29.9825884388805,-2.14851847040971,2.40207950426465));
#72794=CARTESIAN_POINT('Ctrl Pts',(29.9887595617972,-2.22294704631827,2.33550753202896));
#72795=CARTESIAN_POINT('Ctrl Pts',(29.9949306847139,-2.29419080045137,2.26555167083688));
#72796=CARTESIAN_POINT('Ctrl Pts',(30.0011018076305,-2.36194599383186,2.19256212790462));
#72797=CARTESIAN_POINT('Ctrl Pts',(30.0057973295761,-2.41349998193723,2.13702539573097));
#72798=CARTESIAN_POINT('Ctrl Pts',(30.0104928515217,-2.46303505280887,2.07973307181364));
#72799=CARTESIAN_POINT('Ctrl Pts',(30.0151883734672,-2.51043399271408,2.02085099171751));
#72800=CARTESIAN_POINT('Ctrl Pts',(30.021344038126,-2.57257234125583,1.94365864895218));
#72801=CARTESIAN_POINT('Ctrl Pts',(30.0274997027848,-2.63126207956789,1.86345465956792));
#72802=CARTESIAN_POINT('Ctrl Pts',(30.0336553674436,-2.68619615029831,1.78058074925642));
#72803=CARTESIAN_POINT('Ctrl Pts',(30.0398029872817,-2.74105842784748,1.69781514662327));
#72804=CARTESIAN_POINT('Ctrl Pts',(30.0459506071198,-2.79217454934574,1.61238691446173));
#72805=CARTESIAN_POINT('Ctrl Pts',(30.0520982269579,-2.83927725477578,1.52467118849046));
#72806=CARTESIAN_POINT('Ctrl Pts',(30.0582394767409,-2.88633115321394,1.43704635200603));
#72807=CARTESIAN_POINT('Ctrl Pts',(30.0643807265238,-2.9293796938176,1.34713911356048));
#72808=CARTESIAN_POINT('Ctrl Pts',(30.0705219763068,-2.96819913856499,1.25535311220471));
#72809=CARTESIAN_POINT('Ctrl Pts',(30.0766585247557,-3.00698886571653,1.16363737613252));
#72810=CARTESIAN_POINT('Ctrl Pts',(30.0827950732045,-3.04155576315581,1.07004613669127));
#72811=CARTESIAN_POINT('Ctrl Pts',(30.0889316216534,-3.07172271706089,0.975006211258182));
#72812=CARTESIAN_POINT('Ctrl Pts',(30.0950657497165,-3.10187777247517,0.880003771601183));
#72813=CARTESIAN_POINT('Ctrl Pts',(30.1011998777796,-3.12763619914388,0.783554196195001));
#72814=CARTESIAN_POINT('Ctrl Pts',(30.1073340058427,-3.14886990419533,0.686101952302203));
#72815=CARTESIAN_POINT('Ctrl Pts',(30.1134667720909,-3.17009889523106,0.588671343418859));
#72816=CARTESIAN_POINT('Ctrl Pts',(30.1195995383391,-3.18680507343115,0.490238935921755));
#72817=CARTESIAN_POINT('Ctrl Pts',(30.1257323045873,-3.19891115011677,0.391260803248455));
#72818=CARTESIAN_POINT('Ctrl Pts',(30.1318667393409,-3.21102052043089,0.292255742181479));
#72819=CARTESIAN_POINT('Ctrl Pts',(30.1380011740944,-3.21852724015429,0.192705093162679));
#72820=CARTESIAN_POINT('Ctrl Pts',(30.144135608848,-3.22140581046504,0.0930707623373361));
#72821=CARTESIAN_POINT('Ctrl Pts',(30.146099256141,-3.22232724773277,0.0611775738249374));
#72822=CARTESIAN_POINT('Ctrl Pts',(30.1480629034339,-3.22277485870878,0.0292758256471393));
#72823=CARTESIAN_POINT('Ctrl Pts',(30.1500265507269,-3.22274893555634,-0.00261932634679408));
#72824=CARTESIAN_POINT('Ctrl Pts',(30.1484629751925,-3.22274884946717,-0.0027231889481761));
#72825=CARTESIAN_POINT('Ctrl Pts',(30.1525076918999,-3.2226973975967,-0.0636137329032254));
#72826=CARTESIAN_POINT('Ctrl Pts',(30.1565871213781,-3.22092026463483,-0.124489196182319));
#72827=CARTESIAN_POINT('Ctrl Pts',(30.1770332226003,-3.20346580768911,-0.427594650789332));
#72828=CARTESIAN_POINT('Ctrl Pts',(30.1937165015244,-3.16218169450938,-0.667570143758494));
#72829=CARTESIAN_POINT('Ctrl Pts',(30.211082995921,-3.08645744844924,-0.927736036973237));
#72830=CARTESIAN_POINT('Ctrl Pts',(30.2128746803827,-3.07821613849804,-0.954724709180287));
#72831=CARTESIAN_POINT('Ctrl Pts',(30.2151196606511,-3.06732714690351,-0.988776242510945));
#72832=CARTESIAN_POINT('Ctrl Pts',(30.2155911960253,-3.06500803781895,-0.995941772743104));
#72833=CARTESIAN_POINT('Ctrl Pts',(30.2163421605527,-3.0612630157065,-1.00737607929524));
#72834=CARTESIAN_POINT('Ctrl Pts',(30.2166225286293,-3.05985326048818,-1.01165005873636));
#72835=CARTESIAN_POINT('Ctrl Pts',(30.217153991692,-3.05715882342239,-1.0197616723132));
#72836=CARTESIAN_POINT('Ctrl Pts',(30.2174051816405,-3.05587588149516,-1.02359979337814));
#72837=CARTESIAN_POINT('Ctrl Pts',(30.2179796348581,-3.05292028144768,-1.0323868492942));
#72838=CARTESIAN_POINT('Ctrl Pts',(30.2183026099155,-3.05124281989081,-1.03733413442749));
#72839=CARTESIAN_POINT('Ctrl Pts',(30.219319185047,-3.0459135471012,-1.05292681844884));
#72840=CARTESIAN_POINT('Ctrl Pts',(30.2200102351208,-3.04221794987839,-1.06355732125542));
#72841=CARTESIAN_POINT('Ctrl Pts',(30.2262720008826,-3.00807503409262,-1.16013632046875));
#72842=CARTESIAN_POINT('Ctrl Pts',(30.2316414863821,-2.97404538874837,-1.24478477794849));
#72843=CARTESIAN_POINT('Ctrl Pts',(30.2392602759745,-2.91959731055285,-1.36519064838015));
#72844=CARTESIAN_POINT('Ctrl Pts',(30.2415976711563,-2.90201714353768,-1.40217354191918));
#72845=CARTESIAN_POINT('Ctrl Pts',(30.2529718163308,-2.81247825112063,-1.58163167710049));
#72846=CARTESIAN_POINT('Ctrl Pts',(30.2617869019478,-2.73070742261281,-1.71896251313565));
#72847=CARTESIAN_POINT('Ctrl Pts',(30.2776065823303,-2.56931083319896,-1.94924178698007));
#72848=CARTESIAN_POINT('Ctrl Pts',(30.2845269823892,-2.49395081926028,-2.04477565064196));
#72849=CARTESIAN_POINT('Ctrl Pts',(30.2945956494331,-2.37990992420549,-2.17363675140672));
#72850=CARTESIAN_POINT('Ctrl Pts',(30.297581798312,-2.34555801549107,-2.21066170438581));
#72851=CARTESIAN_POINT('Ctrl Pts',(30.3026031541494,-2.28706107148186,-2.27081157500828));
#72852=CARTESIAN_POINT('Ctrl Pts',(30.3046177872112,-2.26340022303195,-2.29439596776597));
#72853=CARTESIAN_POINT('Ctrl Pts',(30.3073464316548,-2.23112437449246,-2.32558235745632));
#72854=CARTESIAN_POINT('Ctrl Pts',(30.3080460740022,-2.22282861187287,-2.33351285247458));
#72855=CARTESIAN_POINT('Ctrl Pts',(30.309159456605,-2.20959641322487,-2.34602784208437));
#72856=CARTESIAN_POINT('Ctrl Pts',(30.3095719345827,-2.20468760425548,-2.35064151067801));
#72857=CARTESIAN_POINT('Ctrl Pts',(30.3104280696165,-2.19448544726556,-2.36017019747952));
#72858=CARTESIAN_POINT('Ctrl Pts',(30.310871823504,-2.18918997272894,-2.36508287408306));
#72859=CARTESIAN_POINT('Ctrl Pts',(30.3118845979425,-2.17708750405103,-2.37623501113201));
#72860=CARTESIAN_POINT('Ctrl Pts',(30.3124540985345,-2.17027014274783,-2.38246308115771));
#72861=CARTESIAN_POINT('Ctrl Pts',(30.3139338854978,-2.15252577873012,-2.39853426493817));
#72862=CARTESIAN_POINT('Ctrl Pts',(30.314846077536,-2.14155808975292,-2.40833195071775));
#72863=CARTESIAN_POINT('Ctrl Pts',(30.3206000894993,-2.07219656138116,-2.46944571655035));
#72864=CARTESIAN_POINT('Ctrl Pts',(30.3255263838029,-2.01203340162778,-2.51870614452558));
#72865=CARTESIAN_POINT('Ctrl Pts',(30.3318330975683,-1.93412038244038,-2.57792579716918));
#72866=CARTESIAN_POINT('Ctrl Pts',(30.3331361598672,-1.91797489253195,-2.58996049270319));
#72867=CARTESIAN_POINT('Ctrl Pts',(30.3453968930367,-1.7656106867121,-2.70132530484808));
#72868=CARTESIAN_POINT('Ctrl Pts',(30.3567112240603,-1.6219215758414,-2.78996385928485));
#72869=CARTESIAN_POINT('Ctrl Pts',(30.3818406144486,-1.29148044801831,-2.95962206631521));
#72870=CARTESIAN_POINT('Ctrl Pts',(30.3956460398804,-1.10262010665849,-3.03504995236058));
#72871=CARTESIAN_POINT('Ctrl Pts',(30.4102921367267,-0.88297389207063,-3.09954027179283));
#72872=CARTESIAN_POINT('Ctrl Pts',(30.4119402030115,-0.857952626019397,
-3.10655921955369));
#72873=CARTESIAN_POINT('Ctrl Pts',(30.4140308949078,-0.825779829014118,
-3.11516593055914));
#72874=CARTESIAN_POINT('Ctrl Pts',(30.4144888947993,-0.818704886209376,
-3.11703278980236));
#72875=CARTESIAN_POINT('Ctrl Pts',(30.4152233673394,-0.807314564566318,
-3.1199968880119));
#72876=CARTESIAN_POINT('Ctrl Pts',(30.4155007089138,-0.803003213570458,
-3.12110929429502));
#72877=CARTESIAN_POINT('Ctrl Pts',(30.4160299647778,-0.794755783334021,
-3.12321905962687));
#72878=CARTESIAN_POINT('Ctrl Pts',(30.4162819622733,-0.790820135862571,
-3.12421791212089));
#72879=CARTESIAN_POINT('Ctrl Pts',(30.4168629560509,-0.781726297196373,
-3.12650760939784));
#72880=CARTESIAN_POINT('Ctrl Pts',(30.4171916436612,-0.776566758632681,
-3.12779313665401));
#72881=CARTESIAN_POINT('Ctrl Pts',(30.4182445544558,-0.759992111116426,
-3.13187926015103));
#72882=CARTESIAN_POINT('Ctrl Pts',(30.4189659612436,-0.748564693650268,
-3.13463022037141));
#72883=CARTESIAN_POINT('Ctrl Pts',(30.4313017251401,-0.551994536310598,
-3.18081495905926));
#72884=CARTESIAN_POINT('Ctrl Pts',(30.4420312303724,-0.36334890615327,-3.20784697814671));
#72885=CARTESIAN_POINT('Ctrl Pts',(30.4628511491851,0.00798076035520758,
-3.22785481080897));
#72886=CARTESIAN_POINT('Ctrl Pts',(30.4729184139981,0.18984902859802,-3.22227622167041));
#72887=CARTESIAN_POINT('Ctrl Pts',(30.487766785037,0.446044141777314,-3.19264465485629));
#72888=CARTESIAN_POINT('Ctrl Pts',(30.4922186182654,0.521473374627156,-3.18119467296213));
#72889=CARTESIAN_POINT('Ctrl Pts',(30.498547455831,0.626122649257305,-3.16148721652626));
#72890=CARTESIAN_POINT('Ctrl Pts',(30.500355917757,0.655742651155446,-3.15547658464048));
#72891=CARTESIAN_POINT('Ctrl Pts',(30.5035214687553,0.707062485085161,-3.14430874263182));
#72892=CARTESIAN_POINT('Ctrl Pts',(30.5048725174265,0.728801716718271,-3.13934114839539));
#72893=CARTESIAN_POINT('Ctrl Pts',(30.5068307236203,0.760065040630739,-3.13185499198639));
#72894=CARTESIAN_POINT('Ctrl Pts',(30.5074320393701,0.769632199713784,-3.12951766740417));
#72895=CARTESIAN_POINT('Ctrl Pts',(30.508484452908,0.786318040804871,-3.12536005745325));
#72896=CARTESIAN_POINT('Ctrl Pts',(30.5089349196094,0.793441525938676,-3.12355920281921));
#72897=CARTESIAN_POINT('Ctrl Pts',(30.5098011142994,0.807103142441979,-3.12005572478635));
#72898=CARTESIAN_POINT('Ctrl Pts',(30.5102167180195,0.81364220721099,-3.1183568695464));
#72899=CARTESIAN_POINT('Ctrl Pts',(30.5111956833793,0.82900762134596,-3.11431329964828));
#72900=CARTESIAN_POINT('Ctrl Pts',(30.5117595939188,0.837829407609145,-3.11195161363531));
#72901=CARTESIAN_POINT('Ctrl Pts',(30.5134264110297,0.863818365991999,-3.10487557394435));
#72902=CARTESIAN_POINT('Ctrl Pts',(30.5145327171416,0.880956434355125,-3.10005648970598));
#72903=CARTESIAN_POINT('Ctrl Pts',(30.5299117550583,1.11763274437505,-3.03138398697964));
#72904=CARTESIAN_POINT('Ctrl Pts',(30.5449737274413,1.32976388134954,-2.94450016619016));
#72905=CARTESIAN_POINT('Ctrl Pts',(30.5710795249889,1.67038503282617,-2.7606273243974));
#72906=CARTESIAN_POINT('Ctrl Pts',(30.5818861196854,1.80414191769187,-2.67513045347115));
#72907=CARTESIAN_POINT('Ctrl Pts',(30.5968629480797,1.98444461280531,-2.54018553525053));
#72908=CARTESIAN_POINT('Ctrl Pts',(30.6012448433717,2.03657492920037,-2.49858494664192));
#72909=CARTESIAN_POINT('Ctrl Pts',(30.6077700056286,2.11377516631272,-2.43295546614008));
#72910=CARTESIAN_POINT('Ctrl Pts',(30.6099768492875,2.13980784328686,-2.41009136411543));
#72911=CARTESIAN_POINT('Ctrl Pts',(30.6126611149765,2.17144102525117,-2.38139171078626));
#72912=CARTESIAN_POINT('Ctrl Pts',(30.613166358437,2.1773937654689,-2.37595012568702));
#72913=CARTESIAN_POINT('Ctrl Pts',(30.6139583396298,2.18672369970377,-2.36735682993711));
#72914=CARTESIAN_POINT('Ctrl Pts',(30.6142461999564,2.19011460220398,-2.36422015238613));
#72915=CARTESIAN_POINT('Ctrl Pts',(30.614783801329,2.19644716989505,-2.35833703872997));
#72916=CARTESIAN_POINT('Ctrl Pts',(30.6150336707569,2.19939040245093,-2.35559241300943));
#72917=CARTESIAN_POINT('Ctrl Pts',(30.6156000554038,2.20606165135364,-2.34934793064447));
#72918=CARTESIAN_POINT('Ctrl Pts',(30.6159163073498,2.20978647465463,-2.34584471909132));
#72919=CARTESIAN_POINT('Ctrl Pts',(30.6168738781703,2.22106347408047,-2.33518796117636));
#72920=CARTESIAN_POINT('Ctrl Pts',(30.6175130868203,2.22858945800586,-2.32800661608087));
#72921=CARTESIAN_POINT('Ctrl Pts',(30.6222007495476,2.28375442661872,-2.27485515433697));
#72922=CARTESIAN_POINT('Ctrl Pts',(30.6261437506206,2.33000546512973,-2.22745958775654));
#72923=CARTESIAN_POINT('Ctrl Pts',(30.6338755019509,2.41941687517277,-2.13000041903725));
#72924=CARTESIAN_POINT('Ctrl Pts',(30.637662775036,2.4625622784975,-2.07996819594275));
#72925=CARTESIAN_POINT('Ctrl Pts',(30.6493123962766,2.59181367775369,-1.92042124981092));
#72926=CARTESIAN_POINT('Ctrl Pts',(30.6570305699771,2.67238009693623,-1.80662740954408));
#72927=CARTESIAN_POINT('Ctrl Pts',(30.6765116443411,2.85440597340829,-1.51057947252612));
#72928=CARTESIAN_POINT('Ctrl Pts',(30.6883664289255,2.94601220550981,-1.32305642531547));
#72929=CARTESIAN_POINT('Ctrl Pts',(30.7022919054544,3.02690551112755,-1.10656466533573));
#72930=CARTESIAN_POINT('Ctrl Pts',(30.7036795992858,3.03469449869471,-1.08502146971086));
#72931=CARTESIAN_POINT('Ctrl Pts',(30.7056826681184,3.04554505923698,-1.05397931396381));
#72932=CARTESIAN_POINT('Ctrl Pts',(30.7062918360714,3.04879333108799,-1.04454598888579));
#72933=CARTESIAN_POINT('Ctrl Pts',(30.7073513845387,3.05435357603803,-1.02815154320923));
#72934=CARTESIAN_POINT('Ctrl Pts',(30.707801094007,3.05668569652833,-1.02119729459456));
#72935=CARTESIAN_POINT('Ctrl Pts',(30.7086675634826,3.06112548359041,-1.00780663107401));
#72936=CARTESIAN_POINT('Ctrl Pts',(30.7090842052122,3.06323664337082,-1.00137140837751));
#72937=CARTESIAN_POINT('Ctrl Pts',(30.7101770816675,3.06871222449474,-0.984501421754472));
#72938=CARTESIAN_POINT('Ctrl Pts',(30.7108543987847,3.07204368843388,-0.97405612661003));
#72939=CARTESIAN_POINT('Ctrl Pts',(30.7131989522372,3.08336133153536,-0.937935738695031));
#72940=CARTESIAN_POINT('Ctrl Pts',(30.7148749547858,3.09107927440623,-0.912178381339127));
#72941=CARTESIAN_POINT('Ctrl Pts',(30.7171253692701,3.10094601046948,-0.877685709630992));
#72942=CARTESIAN_POINT('Ctrl Pts',(30.7176903941089,3.10338199794549,-0.869033104621488));
#72943=CARTESIAN_POINT('Ctrl Pts',(30.7343681768453,3.17406903101491,-0.613865710666124));
#72944=CARTESIAN_POINT('Ctrl Pts',(30.7514762168481,3.21275329840638,-0.360154796611872));
#72945=CARTESIAN_POINT('Ctrl Pts',(30.7815929127867,3.22719472706063,0.0845590682518872));
#72946=CARTESIAN_POINT('Ctrl Pts',(30.7944210539115,3.21666344999222,0.273909449555979));
#72947=CARTESIAN_POINT('Ctrl Pts',(30.8081294869286,3.18597574615162,0.486114166049166));
#72948=CARTESIAN_POINT('Ctrl Pts',(30.8097217645548,3.18209022427304,0.51093085147319));
#72949=CARTESIAN_POINT('Ctrl Pts',(30.8117521499249,3.17671321006679,0.542828701401955));
#72950=CARTESIAN_POINT('Ctrl Pts',(30.812204582021,3.17548761109585,0.549952954580014));
#72951=CARTESIAN_POINT('Ctrl Pts',(30.8129322692036,3.17347180115034,0.561439168057784));
#72952=CARTESIAN_POINT('Ctrl Pts',(30.8132083650399,3.17269655206728,0.56580367725317));
#72953=CARTESIAN_POINT('Ctrl Pts',(30.8137367693971,3.17119277849933,0.574169368670177));
#72954=CARTESIAN_POINT('Ctrl Pts',(30.8139891552782,3.17046568708685,0.578170761515104));
#72955=CARTESIAN_POINT('Ctrl Pts',(30.8145730980991,3.16876296624351,0.587441523919209));
#72956=CARTESIAN_POINT('Ctrl Pts',(30.8149043362293,3.16778176004689,0.59270988009287));
#72957=CARTESIAN_POINT('Ctrl Pts',(30.8159737255753,3.16456441155667,0.60974846013079));
#72958=CARTESIAN_POINT('Ctrl Pts',(30.8167089350636,3.16227574283745,0.621508838456927));
#72959=CARTESIAN_POINT('Ctrl Pts',(30.8259113450526,3.13266895832791,0.769245388484313));
#72960=CARTESIAN_POINT('Ctrl Pts',(30.8339103308113,3.09666237275746,0.903352498968228));
#72961=CARTESIAN_POINT('Ctrl Pts',(30.8519922706406,2.99405000668099,1.20602372996415));
#72962=CARTESIAN_POINT('Ctrl Pts',(30.8619505095565,2.92166437418214,1.37211806222729));
#72963=CARTESIAN_POINT('Ctrl Pts',(30.8813753106195,2.75869013229493,1.67392755718296));
#72964=CARTESIAN_POINT('Ctrl Pts',(30.8907569172403,2.67100855350224,1.81055445371313));
#72965=CARTESIAN_POINT('Ctrl Pts',(30.9017515178581,2.56139251919219,1.95596159008688));
#72966=CARTESIAN_POINT('Ctrl Pts',(30.9029644691363,2.54920778101746,1.97181567105065));
#72967=CARTESIAN_POINT('Ctrl Pts',(30.9047586544124,2.5310546669354,1.99498595166849));
#72968=CARTESIAN_POINT('Ctrl Pts',(30.9053353519348,2.52520025440604,2.00239115722437));
#72969=CARTESIAN_POINT('Ctrl Pts',(30.9063572704619,2.51479220037355,2.01543799553888));
#72970=CARTESIAN_POINT('Ctrl Pts',(30.9068019546391,2.51025187852354,2.02109020826043));
#72971=CARTESIAN_POINT('Ctrl Pts',(30.9076729436232,2.50133709237883,2.03211177804844));
#72972=CARTESIAN_POINT('Ctrl Pts',(30.9080991788263,2.49696431351498,2.03748245244718));
#72973=CARTESIAN_POINT('Ctrl Pts',(30.9092512481354,2.48511806238501,2.05193668087805));
#72974=CARTESIAN_POINT('Ctrl Pts',(30.9099783988559,2.47761216855141,2.06099341645721));
#72975=CARTESIAN_POINT('Ctrl Pts',(30.9126820459508,2.44959903315156,2.09442034719071));
#72976=CARTESIAN_POINT('Ctrl Pts',(30.9146712751398,2.42878098127011,2.11852657323258));
#72977=CARTESIAN_POINT('Ctrl Pts',(30.9339402741997,2.22521185499937,2.34730429157861));
#72978=CARTESIAN_POINT('Ctrl Pts',(30.9523649325636,2.01745175930793,2.52807646687659));
#72979=CARTESIAN_POINT('Ctrl Pts',(30.9709191047552,1.78943620529091,2.68030513742261));
#72980=CARTESIAN_POINT('Origin',(-1.72497344927317,0.,0.));
#72981=CARTESIAN_POINT('',(32.4670258968214,1.789436210378,2.68030513402635));
#72982=CARTESIAN_POINT('',(32.2229614699496,1.78943610001022,2.68030520771053));
#72983=CARTESIAN_POINT('',(-1.72497344927317,1.78943621037804,2.68030513402633));
#72984=CARTESIAN_POINT('',(31.646573449241,-3.22274865695249,0.00294221191095898));
#72985=CARTESIAN_POINT('Ctrl Pts',(31.6465734492731,-3.22274865695296,0.00294221139083024));
#72986=CARTESIAN_POINT('Ctrl Pts',(31.6526668782384,-3.22283885314083,-0.0958541035867903));
#72987=CARTESIAN_POINT('Ctrl Pts',(31.6587603072037,-3.21838176727151,-0.194756389147862));
#72988=CARTESIAN_POINT('Ctrl Pts',(31.664853736169,-3.20937494631332,-0.2933087391749));
#72989=CARTESIAN_POINT('Ctrl Pts',(31.6709440299356,-3.20037275955595,-0.391810381923121));
#72990=CARTESIAN_POINT('Ctrl Pts',(31.6770343237022,-3.18682552646746,-0.489962005563697));
#72991=CARTESIAN_POINT('Ctrl Pts',(31.6831246174688,-3.1687828431129,-0.587309846412713));
#72992=CARTESIAN_POINT('Ctrl Pts',(31.689213485821,-3.15074438259228,-0.684634903302244));
#72993=CARTESIAN_POINT('Ctrl Pts',(31.6953023541733,-3.12821264279287,-0.781156114813821));
#72994=CARTESIAN_POINT('Ctrl Pts',(31.7013912225256,-3.10128865968275,-0.876428098490201));
#72995=CARTESIAN_POINT('Ctrl Pts',(31.7074803735783,-3.07436342651702,-0.971704505556635));
#72996=CARTESIAN_POINT('Ctrl Pts',(31.7135695246311,-3.04304566681001,-1.06573114265188));
#72997=CARTESIAN_POINT('Ctrl Pts',(31.7196586756839,-3.0074864811343,-1.15807712536532));
#72998=CARTESIAN_POINT('Ctrl Pts',(31.7257538952436,-2.9718918568299,-1.25051514097915));
#72999=CARTESIAN_POINT('Ctrl Pts',(31.7318491148033,-2.93204752346106,-1.34126874151655));
#73000=CARTESIAN_POINT('Ctrl Pts',(31.737944334363,-2.8881529416912,-1.42992662325746));
#73001=CARTESIAN_POINT('Ctrl Pts',(31.7440424976996,-2.8442371603799,-1.51862732364161));
#73002=CARTESIAN_POINT('Ctrl Pts',(31.7501406610363,-2.79626745147484,-1.60522990161825));
#73003=CARTESIAN_POINT('Ctrl Pts',(31.7562388243729,-2.74448841329757,-1.6893492568961));
#73004=CARTESIAN_POINT('Ctrl Pts',(31.7623476079941,-2.69261919909692,-1.77361511062611));
#73005=CARTESIAN_POINT('Ctrl Pts',(31.7684563916154,-2.63692765202575,-1.85538873433251));
#73006=CARTESIAN_POINT('Ctrl Pts',(31.7745651752366,-2.57770082090494,-1.93431539320918));
#73007=CARTESIAN_POINT('Ctrl Pts',(31.7805250337949,-2.51991787126655,-2.0113179116403));
#73008=CARTESIAN_POINT('Ctrl Pts',(31.7864848923532,-2.45877035239737,-2.08561045375693));
#73009=CARTESIAN_POINT('Ctrl Pts',(31.7924447509115,-2.39455838703441,-2.15689770123277));
#73010=CARTESIAN_POINT('Ctrl Pts',(31.7986169990043,-2.32805812081721,-2.23072538908249));
#73011=CARTESIAN_POINT('Ctrl Pts',(31.804789247097,-2.25802328677941,-2.30160469149998));
#73012=CARTESIAN_POINT('Ctrl Pts',(31.8109614951898,-2.18474563496786,-2.36917793189725));
#73013=CARTESIAN_POINT('Ctrl Pts',(31.8171253838424,-2.11156722740795,-2.43665965386414));
#73014=CARTESIAN_POINT('Ctrl Pts',(31.8232892724951,-2.03515504805348,-2.50084392164774));
#73015=CARTESIAN_POINT('Ctrl Pts',(31.8294531611477,-1.95583989829263,-2.56140739726164));
#73016=CARTESIAN_POINT('Ctrl Pts',(31.8356105228063,-1.87660873601796,-2.62190674169649));
#73017=CARTESIAN_POINT('Ctrl Pts',(31.8417678844648,-1.79448105803267,-2.67879265432747));
#73018=CARTESIAN_POINT('Ctrl Pts',(31.8479252461234,-1.70982246141898,-2.73178050233307));
#73019=CARTESIAN_POINT('Ctrl Pts',(31.8540781102697,-1.62522570185443,-2.78472964650596));
#73020=CARTESIAN_POINT('Ctrl Pts',(31.860230974416,-1.53810206619429,-2.83378615712614));
#73021=CARTESIAN_POINT('Ctrl Pts',(31.8663838385623,-1.448847240588,-2.87870791084134));
#73022=CARTESIAN_POINT('Ctrl Pts',(31.8725343716988,-1.35962622913159,-2.9236126459707));
#73023=CARTESIAN_POINT('Ctrl Pts',(31.8786849048354,-1.26827601960228,-2.96438554165958));
#73024=CARTESIAN_POINT('Ctrl Pts',(31.8848354379719,-1.1752172956462,-3.0008301968812));
#73025=CARTESIAN_POINT('Ctrl Pts',(31.8909852861871,-1.08216893467882,-3.03727079363807));
#73026=CARTESIAN_POINT('Ctrl Pts',(31.8971351344023,-0.987412842012983,
-3.06938394979638));
#73027=CARTESIAN_POINT('Ctrl Pts',(31.9032849826175,-0.891389155669776,
-3.09702162337532));
#73028=CARTESIAN_POINT('Ctrl Pts',(31.9094357909966,-0.795350477333879,
-3.12466361197086));
#73029=CARTESIAN_POINT('Ctrl Pts',(31.9155865993758,-0.698044229694665,
-3.14782860993577));
#73030=CARTESIAN_POINT('Ctrl Pts',(31.9217374077549,-0.59992418370671,-3.1664188820028));
#73031=CARTESIAN_POINT('Ctrl Pts',(31.9278947941211,-0.501699203155232,
-3.1850290354515));
#73032=CARTESIAN_POINT('Ctrl Pts',(31.9340521804873,-0.402659113936038,
-3.19905461227844));
#73033=CARTESIAN_POINT('Ctrl Pts',(31.9402095668535,-0.30326620196804,-3.20844934091905));
#73034=CARTESIAN_POINT('Ctrl Pts',(31.9463703895904,-0.203817819890132,
-3.21784931265617));
#73035=CARTESIAN_POINT('Ctrl Pts',(31.9525312123274,-0.104016656822131,
-3.22261326864607));
#73036=CARTESIAN_POINT('Ctrl Pts',(31.9586920350644,-0.00432631756911811,
-3.22274709610858));
#73037=CARTESIAN_POINT('Ctrl Pts',(31.964863157981,0.0955306923469966,-3.22288114731506));
#73038=CARTESIAN_POINT('Ctrl Pts',(31.9710342808977,0.19527607421438,-3.21836962714771));
#73039=CARTESIAN_POINT('Ctrl Pts',(31.9772054038144,0.294449884276756,-3.20927045107598));
#73040=CARTESIAN_POINT('Ctrl Pts',(31.9819009257599,0.369909862607305,-3.20234701404389));
#73041=CARTESIAN_POINT('Ctrl Pts',(31.9865964477054,0.445039007553297,-3.19276864227843));
#73042=CARTESIAN_POINT('Ctrl Pts',(31.991291969651,0.519639334911914,-3.18058053256199));
#73043=CARTESIAN_POINT('Ctrl Pts',(31.9974642177437,0.617701218894503,-3.16455930258487));
#73044=CARTESIAN_POINT('Ctrl Pts',(32.0036364658365,0.715194071780944,-3.14397054045711));
#73045=CARTESIAN_POINT('Ctrl Pts',(32.0098087139293,0.811659260599448,-3.11886626952538));
#73046=CARTESIAN_POINT('Ctrl Pts',(32.0159726025819,0.907993800915114,-3.09379599879053));
#73047=CARTESIAN_POINT('Ctrl Pts',(32.0221364912345,1.00330302689841,-3.06422248315563));
#73048=CARTESIAN_POINT('Ctrl Pts',(32.0283003798871,1.09713607605518,-3.03024916353726));
#73049=CARTESIAN_POINT('Ctrl Pts',(32.0344577415457,1.19086976459878,-2.99631181855574));
#73050=CARTESIAN_POINT('Ctrl Pts',(32.0406151032042,1.2831299778011,-2.95798407916353));
#73051=CARTESIAN_POINT('Ctrl Pts',(32.0467724648627,1.37347959790967,-2.91541958500417));
#73052=CARTESIAN_POINT('Ctrl Pts',(32.052925329009,1.4637632240837,-2.87288618116304));
#73053=CARTESIAN_POINT('Ctrl Pts',(32.0590781931553,1.55213863999183,-2.82612235980595));
#73054=CARTESIAN_POINT('Ctrl Pts',(32.0652310573016,1.63818821775929,-2.77533005707333));
#73055=CARTESIAN_POINT('Ctrl Pts',(32.0713815904382,1.72420519568361,-2.72455699698134));
#73056=CARTESIAN_POINT('Ctrl Pts',(32.0775321235747,1.80789771263815,-2.66975870859827));
#73057=CARTESIAN_POINT('Ctrl Pts',(32.0836826567112,1.88887308637349,-2.61118287871108));
#73058=CARTESIAN_POINT('Ctrl Pts',(32.0898325049264,1.96983944271802,-2.55261357180891));
#73059=CARTESIAN_POINT('Ctrl Pts',(32.0959823531417,2.04808890547082,-2.49026781433787));
#73060=CARTESIAN_POINT('Ctrl Pts',(32.1021322013569,2.12325895326331,-2.42443580650988));
#73061=CARTESIAN_POINT('Ctrl Pts',(32.108283009736,2.19844073721022,-2.35859352045761));
#73062=CARTESIAN_POINT('Ctrl Pts',(32.1144338181151,2.27054182443136,-2.2892641891333));
#73063=CARTESIAN_POINT('Ctrl Pts',(32.1205846264943,2.33923464054728,-2.21677668224917));
#73064=CARTESIAN_POINT('Ctrl Pts',(32.1267420128604,2.40800092025162,-2.14421165354147));
#73065=CARTESIAN_POINT('Ctrl Pts',(32.1328993992266,2.47335135083689,-2.0684820206347));
#73066=CARTESIAN_POINT('Ctrl Pts',(32.1390567855928,2.53499704552073,-1.98995164305598));
#73067=CARTESIAN_POINT('Ctrl Pts',(32.1452176083298,2.59667714400032,-1.91137743852251));
#73068=CARTESIAN_POINT('Ctrl Pts',(32.1513784310667,2.65464813700084,-1.82999973029181));
#73069=CARTESIAN_POINT('Ctrl Pts',(32.1575392538037,2.70866430103904,-1.7462116901386));
#73070=CARTESIAN_POINT('Ctrl Pts',(32.1637103767203,2.76277077382688,-1.66228356611834));
#73071=CARTESIAN_POINT('Ctrl Pts',(32.169881499637,2.8129089921349,-1.57593743659895));
#73072=CARTESIAN_POINT('Ctrl Pts',(32.1760526225537,2.85887897867376,-1.48759152585556));
#73073=CARTESIAN_POINT('Ctrl Pts',(32.1807481444994,2.89385690466046,-1.42037034612784));
#73074=CARTESIAN_POINT('Ctrl Pts',(32.185443666445,2.92642259088435,-1.35199191599748));
#73075=CARTESIAN_POINT('Ctrl Pts',(32.1901391883907,2.95650700519601,-1.28264721990378));
#73076=CARTESIAN_POINT('Ctrl Pts',(32.1963114364834,2.99605286846886,-1.19149384586733));
#73077=CARTESIAN_POINT('Ctrl Pts',(32.2024836845762,3.03144880204087,-1.09834943445963));
#73078=CARTESIAN_POINT('Ctrl Pts',(32.208655932669,3.06249058087111,-1.00362792138109));
#73079=CARTESIAN_POINT('Ctrl Pts',(32.2148198213216,3.09349031798691,-0.909034695242089));
#73080=CARTESIAN_POINT('Ctrl Pts',(32.2209837099743,3.1201474873923,-0.812869022032163));
#73081=CARTESIAN_POINT('Ctrl Pts',(32.2271475986269,3.14230531854134,-0.715566102863193));
#73082=CARTESIAN_POINT('Ctrl Pts',(32.2333049602855,3.16443968657456,-0.618366218582687));
#73083=CARTESIAN_POINT('Ctrl Pts',(32.239462321944,3.1820840924887,-0.520031903682021));
#73084=CARTESIAN_POINT('Ctrl Pts',(32.2456196836025,3.19513142527696,-0.421013940039524));
#73085=CARTESIAN_POINT('Ctrl Pts',(32.2517725477488,3.20816922792196,-0.322068301936224));
#73086=CARTESIAN_POINT('Ctrl Pts',(32.2579254118952,3.21661657681269,-0.222440437251676));
#73087=CARTESIAN_POINT('Ctrl Pts',(32.2640782760415,3.22041752676248,-0.122590847215692));
#73088=CARTESIAN_POINT('Ctrl Pts',(32.270228809178,3.22421703672411,-0.0227790851513653));
#73089=CARTESIAN_POINT('Ctrl Pts',(32.2763793423145,3.22337362891887,0.0772538017767354));
#73090=CARTESIAN_POINT('Ctrl Pts',(32.2825298754511,3.21788333236684,0.177043558978158));
#73091=CARTESIAN_POINT('Ctrl Pts',(32.2886797236663,3.21239364721242,0.276822203625462));
#73092=CARTESIAN_POINT('Ctrl Pts',(32.2948295718815,3.20225812599177,0.37635733865508));
#73093=CARTESIAN_POINT('Ctrl Pts',(32.3009794200967,3.18752486869412,0.475187093634188));
#73094=CARTESIAN_POINT('Ctrl Pts',(32.3071302284758,3.17278931112146,0.574032278712152));
#73095=CARTESIAN_POINT('Ctrl Pts',(32.313281036855,3.15345465571844,0.672171435325801));
#73096=CARTESIAN_POINT('Ctrl Pts',(32.3194318452341,3.12962042779751,0.769151181766334));
#73097=CARTESIAN_POINT('Ctrl Pts',(32.3255892316003,3.10576071034205,0.866234643275956));
#73098=CARTESIAN_POINT('Ctrl Pts',(32.3317466179665,3.07739191503035,0.962155795950736));
#73099=CARTESIAN_POINT('Ctrl Pts',(32.3379040043327,3.04466391969892,1.05647488308223));
#73100=CARTESIAN_POINT('Ctrl Pts',(32.3440648270697,3.01191765922705,1.15084660867677));
#73101=CARTESIAN_POINT('Ctrl Pts',(32.3502256498066,2.97480751514342,1.24361408483356));
#73102=CARTESIAN_POINT('Ctrl Pts',(32.3563864725436,2.93353136184629,1.33435801476374));
#73103=CARTESIAN_POINT('Ctrl Pts',(32.3625575954603,2.89218619961718,1.42525365800025));
#73104=CARTESIAN_POINT('Ctrl Pts',(32.368728718377,2.84666131377875,1.51411861052658));
#73105=CARTESIAN_POINT('Ctrl Pts',(32.3748998412937,2.7972003885514,1.60055851151649));
#73106=CARTESIAN_POINT('Ctrl Pts',(32.3795953632392,2.75956625567364,1.66632943482297));
#73107=CARTESIAN_POINT('Ctrl Pts',(32.3842908851848,2.71965431070223,1.73069689768004));
#73108=CARTESIAN_POINT('Ctrl Pts',(32.3889864071303,2.67758788505995,1.7934995623864));
#73109=CARTESIAN_POINT('Ctrl Pts',(32.3951596181536,2.62228308071711,1.87606633697594));
#73110=CARTESIAN_POINT('Ctrl Pts',(32.4013328291769,2.5630582644798,1.95621797396748));
#73111=CARTESIAN_POINT('Ctrl Pts',(32.4075060402002,2.50015133106894,2.03355867489833));
#73112=CARTESIAN_POINT('Ctrl Pts',(32.4136691809538,2.43734701682694,2.11077321106451));
#73113=CARTESIAN_POINT('Ctrl Pts',(32.4198323217074,2.37087280745839,2.1851855998657));
#73114=CARTESIAN_POINT('Ctrl Pts',(32.425995462461,2.30100993230182,2.25642878326535));
#73115=CARTESIAN_POINT('Ctrl Pts',(32.4321528014495,2.23121282361269,2.32760490082366));
#73116=CARTESIAN_POINT('Ctrl Pts',(32.4383101404379,2.15803368874889,2.39561743152967));
#73117=CARTESIAN_POINT('Ctrl Pts',(32.4444674794264,2.08179381116393,2.46013253510854));
#73118=CARTESIAN_POINT('Ctrl Pts',(32.4506200279823,2.00561324848577,2.52459744569816));
#73119=CARTESIAN_POINT('Ctrl Pts',(32.4567725765383,1.92637700977985,2.5855700613177));
#73120=CARTESIAN_POINT('Ctrl Pts',(32.4629251250942,1.84444216790488,2.6427543684108));
#73121=CARTESIAN_POINT('Ctrl Pts',(32.4642920490033,1.82623854166322,2.65545911927611));
#73122=CARTESIAN_POINT('Ctrl Pts',(32.4656589729124,1.80790184371059,2.66797703282869));
#73123=CARTESIAN_POINT('Ctrl Pts',(32.4670258968214,1.789436210378,2.68030513402635));
#73124=CARTESIAN_POINT('Ctrl Pts',(31.2170551299057,1.78943621037803,2.68030513402633));
#73125=CARTESIAN_POINT('Ctrl Pts',(31.2232179771471,1.70662880253117,2.73558935230715));
#73126=CARTESIAN_POINT('Ctrl Pts',(31.2293808243885,1.62114288271662,2.78710868993221));
#73127=CARTESIAN_POINT('Ctrl Pts',(31.23554367163,1.53335639378915,2.83459622029769));
#73128=CARTESIAN_POINT('Ctrl Pts',(31.2417002522632,1.44565916937131,2.88203546360711));
#73129=CARTESIAN_POINT('Ctrl Pts',(31.2478568328964,1.35566640687756,2.92545084492418));
#73130=CARTESIAN_POINT('Ctrl Pts',(31.2540134135295,1.26378424804521,2.9646191891865));
#73131=CARTESIAN_POINT('Ctrl Pts',(31.2601658450428,1.17196401158862,3.00376113662746));
#73132=CARTESIAN_POINT('Ctrl Pts',(31.266318276556,1.07825730864577,3.03866156717211));
#73133=CARTESIAN_POINT('Ctrl Pts',(31.2724707080692,0.983093245736578,3.06914405538207));
#73134=CARTESIAN_POINT('Ctrl Pts',(31.2786210431498,0.887961609851441,3.09961615672595));
#73135=CARTESIAN_POINT('Ctrl Pts',(31.2847713782304,0.791374014071506,3.12567317470469));
#73136=CARTESIAN_POINT('Ctrl Pts',(31.290921713311,0.693776968053361,3.14718780518397));
#73137=CARTESIAN_POINT('Ctrl Pts',(31.2970715978239,0.596187071901783,3.16870085952193));
#73138=CARTESIAN_POINT('Ctrl Pts',(31.3032214823369,0.497588296812218,3.18567209466996));
#73139=CARTESIAN_POINT('Ctrl Pts',(31.3093713668498,0.398438662534779,3.1980250459772));
#73140=CARTESIAN_POINT('Ctrl Pts',(31.3155224458448,0.299269770584,3.21038039657823));
#73141=CARTESIAN_POINT('Ctrl Pts',(31.3216735248399,0.19955023796126,3.21811562776666));
#73142=CARTESIAN_POINT('Ctrl Pts',(31.327824603835,0.0997435368877103,3.22120610786536));
#73143=CARTESIAN_POINT('Ctrl Pts',(31.3339823890386,-0.000171978355588673,
3.22429995735733));
#73144=CARTESIAN_POINT('Ctrl Pts',(31.3401401742422,-0.100174416881713,
3.22273893209103));
#73145=CARTESIAN_POINT('Ctrl Pts',(31.3462979594459,-0.199800114916488,
3.21655055557648));
#73146=CARTESIAN_POINT('Ctrl Pts',(31.3524593916297,-0.299484816787854,
3.21035851396383));
#73147=CARTESIAN_POINT('Ctrl Pts',(31.3586208238136,-0.398791902276235,
3.19953371115868));
#73148=CARTESIAN_POINT('Ctrl Pts',(31.3647822559975,-0.497264710914674,
3.18415536206683));
#73149=CARTESIAN_POINT('Ctrl Pts',(31.3709537255055,-0.595897937370692,
3.16875196076784));
#73150=CARTESIAN_POINT('Ctrl Pts',(31.3771251950136,-0.693693747658595,
3.14878028696303));
#73151=CARTESIAN_POINT('Ctrl Pts',(31.3832966645216,-0.790207480306894,
3.1243702886449));
#73152=CARTESIAN_POINT('Ctrl Pts',(31.3871145474918,-0.84991418967032,3.10926942542937));
#73153=CARTESIAN_POINT('Ctrl Pts',(31.3909324304619,-0.909130543615332,
3.0924709655686));
#73154=CARTESIAN_POINT('Ctrl Pts',(31.3947503134321,-0.967755029328688,
3.07401492607128));
#73155=CARTESIAN_POINT('Ctrl Pts',(31.4009225615248,-1.06253134200341,3.04417764308534));
#73156=CARTESIAN_POINT('Ctrl Pts',(31.4070948096176,-1.15609328870176,3.00990060091551));
#73157=CARTESIAN_POINT('Ctrl Pts',(31.4132670577104,-1.24799433728965,2.97130067421541));
#73158=CARTESIAN_POINT('Ctrl Pts',(31.419430946363,-1.33977091885955,2.93275302567585));
#73159=CARTESIAN_POINT('Ctrl Pts',(31.4255948350156,-1.42989067639552,2.88989429627056));
#73160=CARTESIAN_POINT('Ctrl Pts',(31.4317587236682,-1.51792209895778,2.8428911452948));
#73161=CARTESIAN_POINT('Ctrl Pts',(31.4379160853268,-1.60586030429849,2.7959377663551));
#73162=CARTESIAN_POINT('Ctrl Pts',(31.4440734469853,-1.69171418998586,2.74484889418658));
#73163=CARTESIAN_POINT('Ctrl Pts',(31.4502308086439,-1.77507300576022,2.6898389146418));
#73164=CARTESIAN_POINT('Ctrl Pts',(31.4563836727902,-1.85837093388257,2.63486911595204));
#73165=CARTESIAN_POINT('Ctrl Pts',(31.4625365369365,-1.93917705401979,2.575984142714));
#73166=CARTESIAN_POINT('Ctrl Pts',(31.4686894010828,-2.01710679186687,2.51344340551056));
#73167=CARTESIAN_POINT('Ctrl Pts',(31.4748399342194,-2.09500700606836,2.45092636183685));
#73168=CARTESIAN_POINT('Ctrl Pts',(31.4809904673559,-2.17003266484376,2.38475657772647));
#73169=CARTESIAN_POINT('Ctrl Pts',(31.4871410004924,-2.24183040693022,2.31523519087437));
#73170=CARTESIAN_POINT('Ctrl Pts',(31.4932908487076,-2.3136201536439,2.24572154590089));
#73171=CARTESIAN_POINT('Ctrl Pts',(31.4994406969228,-2.38218238627006,2.17285734239147));
#73172=CARTESIAN_POINT('Ctrl Pts',(31.505590545138,-2.44719965707779,2.09698149750978));
#73173=CARTESIAN_POINT('Ctrl Pts',(31.5117413535172,-2.51222707890648,2.02109380627893));
#73174=CARTESIAN_POINT('Ctrl Pts',(31.5178921618963,-2.57370815692001,1.94219386960818));
#73175=CARTESIAN_POINT('Ctrl Pts',(31.5240429702755,-2.63136554615387,1.86065389715936));
#73176=CARTESIAN_POINT('Ctrl Pts',(31.5302003566416,-2.68908459712986,1.77902672172025));
#73177=CARTESIAN_POINT('Ctrl Pts',(31.5363577430078,-2.74297154224672,1.69475422784555));
#73178=CARTESIAN_POINT('Ctrl Pts',(31.542515129374,-2.79279231713283,1.60823774233284));
#73179=CARTESIAN_POINT('Ctrl Pts',(31.548675952111,-2.84264089645487,1.52167297290476));
#73180=CARTESIAN_POINT('Ctrl Pts',(31.554836774848,-2.88841858727227,1.43286210392005));
#73181=CARTESIAN_POINT('Ctrl Pts',(31.5609975975849,-2.92993822640096,1.34222932167883));
#73182=CARTESIAN_POINT('Ctrl Pts',(31.5671687205016,-2.97152728154169,1.25144501195721));
#73183=CARTESIAN_POINT('Ctrl Pts',(31.5733398434183,-3.00884390265784,1.15883310771925));
#73184=CARTESIAN_POINT('Ctrl Pts',(31.579510966335,-3.04174977699738,1.06483607031147));
#73185=CARTESIAN_POINT('Ctrl Pts',(31.5842064882806,-3.06678740097381,0.993315026584462));
#73186=CARTESIAN_POINT('Ctrl Pts',(31.5889020102262,-3.08927244588873,0.92099244102941));
#73187=CARTESIAN_POINT('Ctrl Pts',(31.5935975321718,-3.10916381139467,0.84806718861996));
#73188=CARTESIAN_POINT('Ctrl Pts',(31.6014764629116,-3.1425408657365,0.725701023670892));
#73189=CARTESIAN_POINT('Ctrl Pts',(31.6093553936514,-3.16870984081663,0.601290341548845));
#73190=CARTESIAN_POINT('Ctrl Pts',(31.6172343243912,-3.18746608133155,0.475581268408342));
#73191=CARTESIAN_POINT('Ctrl Pts',(31.6249655353474,-3.20587066654171,0.352229078161851));
#73192=CARTESIAN_POINT('Ctrl Pts',(31.6326967463036,-3.21713787939234,0.227626547890882));
#73193=CARTESIAN_POINT('Ctrl Pts',(31.6404279572598,-3.22111956307449,0.102500355505779));
#73194=CARTESIAN_POINT('Ctrl Pts',(31.6424764545869,-3.22217456835456,0.069346342234137));
#73195=CARTESIAN_POINT('Ctrl Pts',(31.6445249519139,-3.22271833466869,0.0361556929095487));
#73196=CARTESIAN_POINT('Ctrl Pts',(31.646573449241,-3.22274865695249,0.00294221191100407));
#73197=CARTESIAN_POINT('Ctrl Pts',(30.9709191047552,1.78943620529092,2.68030513742261));
#73198=CARTESIAN_POINT('Ctrl Pts',(30.9718568373112,1.77791224151339,2.6879988129389));
#73199=CARTESIAN_POINT('Ctrl Pts',(30.9727945355257,1.76633652017013,2.69561959581997));
#73200=CARTESIAN_POINT('Ctrl Pts',(30.9853875055158,1.61014525231306,2.79700820363487));
#73201=CARTESIAN_POINT('Ctrl Pts',(30.996967889745,1.45826721413129,2.87911338138045));
#73202=CARTESIAN_POINT('Ctrl Pts',(31.0088238281147,1.28701476112885,2.95464530819892));
#73203=CARTESIAN_POINT('Ctrl Pts',(31.009754705807,1.27345418040215,2.96051521913541));
#73204=CARTESIAN_POINT('Ctrl Pts',(31.0110495128099,1.25442372661726,2.96859789735097));
#73205=CARTESIAN_POINT('Ctrl Pts',(31.0114180622943,1.2489876751289,2.97088911788172));
#73206=CARTESIAN_POINT('Ctrl Pts',(31.0120440708352,1.23972065409924,2.97476510825769));
#73207=CARTESIAN_POINT('Ctrl Pts',(31.0123019881025,1.2358928779266,2.97635742888257));
#73208=CARTESIAN_POINT('Ctrl Pts',(31.0127934745622,1.22857984276965,2.97938304576577));
#73209=CARTESIAN_POINT('Ctrl Pts',(31.0130271228413,1.22509513918222,2.98081761665446));
#73210=CARTESIAN_POINT('Ctrl Pts',(31.0135773246771,1.21687026935222,2.98418674372764));
#73211=CARTESIAN_POINT('Ctrl Pts',(31.0138935643402,1.21212797641181,2.98611613028156));
#73212=CARTESIAN_POINT('Ctrl Pts',(31.0148287773001,1.19806029002336,2.99180048893859));
#73213=CARTESIAN_POINT('Ctrl Pts',(31.0154458391643,1.18872179803311,2.99552317921845));
#73214=CARTESIAN_POINT('Ctrl Pts',(31.0214196829157,1.09778478844465,3.03128202501158));
#73215=CARTESIAN_POINT('Ctrl Pts',(31.0265900173565,1.01492034094531,3.06002319245713));
#73216=CARTESIAN_POINT('Ctrl Pts',(31.0326872739042,0.913854592082875,3.09051893608328));
#73217=CARTESIAN_POINT('Ctrl Pts',(31.03371584146,0.896687161425791,3.09554351635211));
#73218=CARTESIAN_POINT('Ctrl Pts',(31.0425888804298,0.747675345730186,3.13781278533194));
#73219=CARTESIAN_POINT('Ctrl Pts',(31.0502061815097,0.613616203277497,3.16675955363183));
#73220=CARTESIAN_POINT('Ctrl Pts',(31.065972900184,0.334713752149143,3.20859960573247));
#73221=CARTESIAN_POINT('Ctrl Pts',(31.0741119362097,0.190029630775623,3.22040826776404));
#73222=CARTESIAN_POINT('Ctrl Pts',(31.0863632704994,-0.0215458968595493,
3.22336613798423));
#73223=CARTESIAN_POINT('Ctrl Pts',(31.0902688662274,-0.0881513830149897,
3.22223244938175));
#73224=CARTESIAN_POINT('Ctrl Pts',(31.0967049007624,-0.196057898045551,
3.21704766848016));
#73225=CARTESIAN_POINT('Ctrl Pts',(31.0991966434073,-0.237401156262834,
3.21426116727348));
#73226=CARTESIAN_POINT('Ctrl Pts',(31.102476540778,-0.291192910561514,3.20959219513189));
#73227=CARTESIAN_POINT('Ctrl Pts',(31.1032419044757,-0.303701410540815,
3.20843276639131));
#73228=CARTESIAN_POINT('Ctrl Pts',(31.1044905837684,-0.324035877437877,
3.20642796084972));
#73229=CARTESIAN_POINT('Ctrl Pts',(31.1049724967607,-0.331866168494229,
3.2056269842973));
#73230=CARTESIAN_POINT('Ctrl Pts',(31.1059005302566,-0.346910992517077,
3.20403230395705));
#73231=CARTESIAN_POINT('Ctrl Pts',(31.106346512395,-0.354125940409939,3.20324289720358));
#73232=CARTESIAN_POINT('Ctrl Pts',(31.1073680387804,-0.370616952115945,
3.201382174978));
#73233=CARTESIAN_POINT('Ctrl Pts',(31.1079440838551,-0.379891117504225,
3.20029490693649));
#73234=CARTESIAN_POINT('Ctrl Pts',(31.1094726305353,-0.404432688541827,
3.19730956566316));
#73235=CARTESIAN_POINT('Ctrl Pts',(31.1104273069893,-0.419691310744896,
3.19534246188166));
#73236=CARTESIAN_POINT('Ctrl Pts',(31.1169820348231,-0.523974464562714,
3.18113869804931));
#73237=CARTESIAN_POINT('Ctrl Pts',(31.1226957867421,-0.612459695148485,
3.16529353968943));
#73238=CARTESIAN_POINT('Ctrl Pts',(31.1312864919747,-0.74187806838251,3.13648864763356));
#73239=CARTESIAN_POINT('Ctrl Pts',(31.134078884545,-0.783405023158639,3.12637496625337));
#73240=CARTESIAN_POINT('Ctrl Pts',(31.1373152764683,-0.830936761069419,
3.1137923911115));
#73241=CARTESIAN_POINT('Ctrl Pts',(31.1377392146266,-0.837151321918574,
3.11212734625159));
#73242=CARTESIAN_POINT('Ctrl Pts',(31.1437071565212,-0.924473376089669,
3.08845098151552));
#73243=CARTESIAN_POINT('Ctrl Pts',(31.1493256040755,-1.00469048338039,3.0632949869048));
#73244=CARTESIAN_POINT('Ctrl Pts',(31.1713120903255,-1.31214008878246,2.95350287724719));
#73245=CARTESIAN_POINT('Ctrl Pts',(31.1879744780598,-1.53053146364814,2.84646744972768));
#73246=CARTESIAN_POINT('Ctrl Pts',(31.2053214238543,-1.75862822741037,2.70076649731007));
#73247=CARTESIAN_POINT('Ctrl Pts',(31.2071121718094,-1.7821959302303,2.68527293055207));
#73248=CARTESIAN_POINT('Ctrl Pts',(31.2093561502504,-1.81179541823263,2.66525263833305));
#73249=CARTESIAN_POINT('Ctrl Pts',(31.2098276008651,-1.81801795961574,2.66101201892952));
#73250=CARTESIAN_POINT('Ctrl Pts',(31.2105784621442,-1.82793545137813,2.65420229058835));
#73251=CARTESIAN_POINT('Ctrl Pts',(31.2108588112871,-1.83163993593818,2.6516472162485));
#73252=CARTESIAN_POINT('Ctrl Pts',(31.211390259989,-1.83866568211478,2.64677963759236));
#73253=CARTESIAN_POINT('Ctrl Pts',(31.2116414544237,-1.84198789962386,2.64446866465808));
#73254=CARTESIAN_POINT('Ctrl Pts',(31.2122159460476,-1.84958902990053,2.63915995682519));
#73255=CARTESIAN_POINT('Ctrl Pts',(31.2125389548908,-1.85386500684233,2.63615807465281));
#73256=CARTESIAN_POINT('Ctrl Pts',(31.213555742657,-1.86733138912021,2.62665524389273));
#73257=CARTESIAN_POINT('Ctrl Pts',(31.2142469700604,-1.87649516533766,2.62011644593684));
#73258=CARTESIAN_POINT('Ctrl Pts',(31.2205157131932,-1.95966021579396,2.56011403928519));
#73259=CARTESIAN_POINT('Ctrl Pts',(31.2258915021273,-2.03140047486081,2.50357097013144));
#73260=CARTESIAN_POINT('Ctrl Pts',(31.2477496771461,-2.31893160637899,2.25643951993253));
#73261=CARTESIAN_POINT('Ctrl Pts',(31.263250028093,-2.51110256810998,2.04042841684177));
#73262=CARTESIAN_POINT('Ctrl Pts',(31.2840254493609,-2.71236963561823,1.74194490322321));
#73263=CARTESIAN_POINT('Ctrl Pts',(31.2882440717604,-2.75067690512347,1.6808023622322));
#73264=CARTESIAN_POINT('Ctrl Pts',(31.2942628825759,-2.80148334426456,1.59331480534135));
#73265=CARTESIAN_POINT('Ctrl Pts',(31.296002010293,-2.81572737447259,1.568005187606));
#73266=CARTESIAN_POINT('Ctrl Pts',(31.299066340802,-2.84004982270219,1.52338726835963));
#73267=CARTESIAN_POINT('Ctrl Pts',(31.3003861769416,-2.85027831351838,1.50416264559979));
#73268=CARTESIAN_POINT('Ctrl Pts',(31.3023084145479,-2.86481405096525,1.47616175916599));
#73269=CARTESIAN_POINT('Ctrl Pts',(31.3029052880589,-2.86927757660002,1.46746695735861));
#73270=CARTESIAN_POINT('Ctrl Pts',(31.3039504519946,-2.87700599173559,1.45224219207693));
#73271=CARTESIAN_POINT('Ctrl Pts',(31.3043981226943,-2.88028838802071,1.44572115616103));
#73272=CARTESIAN_POINT('Ctrl Pts',(31.3052657481803,-2.88659593280366,1.4330834060438));
#73273=CARTESIAN_POINT('Ctrl Pts',(31.3056856021823,-2.88962386975111,1.42696812093962));
#73274=CARTESIAN_POINT('Ctrl Pts',(31.3067985817369,-2.89758600680907,1.41075835654535));
#73275=CARTESIAN_POINT('Ctrl Pts',(31.3074928676233,-2.90248684486014,1.4006476779333));
#73276=CARTESIAN_POINT('Ctrl Pts',(31.3099549579941,-2.91963250054836,1.36479888945936));
#73277=CARTESIAN_POINT('Ctrl Pts',(31.3117327388648,-2.93158835718976,1.33892478008489));
#73278=CARTESIAN_POINT('Ctrl Pts',(31.3139614120278,-2.94604759478254,1.30651062769269));
#73279=CARTESIAN_POINT('Ctrl Pts',(31.3144011621319,-2.94887522827616,1.30011589399433));
#73280=CARTESIAN_POINT('Ctrl Pts',(31.330557449065,-3.05183069479925,1.06521679209629));
#73281=CARTESIAN_POINT('Ctrl Pts',(31.3472172188721,-3.12508959796379,0.825909031198407));
#73282=CARTESIAN_POINT('Ctrl Pts',(31.3772841357442,-3.20512887646001,0.388905514104594));
#73283=CARTESIAN_POINT('Ctrl Pts',(31.3905150821367,-3.22278173040772,0.194399018396028));
#73284=CARTESIAN_POINT('Ctrl Pts',(31.4045794950268,-3.22274588361549,-0.0255161102361829));
#73285=CARTESIAN_POINT('Ctrl Pts',(31.4061643337136,-3.22245112344944,-0.0505069351096372));
#73286=CARTESIAN_POINT('Ctrl Pts',(31.4082060354822,-3.22168949455668,-0.0830116157642455));
#73287=CARTESIAN_POINT('Ctrl Pts',(31.4086769155593,-3.2214869939441,-0.090529985258089));
#73288=CARTESIAN_POINT('Ctrl Pts',(31.4094270818381,-3.22112132400558,-0.102543706001211));
#73289=CARTESIAN_POINT('Ctrl Pts',(31.4097073035252,-3.2209750611107,-0.107039487567294));
#73290=CARTESIAN_POINT('Ctrl Pts',(31.4102134432731,-3.22069334016856,-0.115174803177854));
#73291=CARTESIAN_POINT('Ctrl Pts',(31.4104395395049,-3.22056112682172,-0.118814372992826));
#73292=CARTESIAN_POINT('Ctrl Pts',(31.4109810724537,-3.2202291661926,-0.127544635872793));
#73293=CARTESIAN_POINT('Ctrl Pts',(31.4112961740388,-3.22002351742405,-0.13263508217206));
#73294=CARTESIAN_POINT('Ctrl Pts',(31.4122468511133,-3.21936525328147,-0.148024312619176));
#73295=CARTESIAN_POINT('Ctrl Pts',(31.4128803608031,-3.21887528854726,-0.158321554729984));
#73296=CARTESIAN_POINT('Ctrl Pts',(31.4190815910356,-3.21357380493439,-0.25950952887032));
#73297=CARTESIAN_POINT('Ctrl Pts',(31.42444690139,-3.20496276882851,-0.35016979713089));
#73298=CARTESIAN_POINT('Ctrl Pts',(31.4305789503432,-3.19044163039852,-0.455446966742716));
#73299=CARTESIAN_POINT('Ctrl Pts',(31.4314549030594,-3.18825258259106,-0.470526531380754));
#73300=CARTESIAN_POINT('Ctrl Pts',(31.4443682547491,-3.15429625737877,-0.693313947476272));
#73301=CARTESIAN_POINT('Ctrl Pts',(31.4558717632582,-3.10239592895722,-0.897450214191542));
#73302=CARTESIAN_POINT('Ctrl Pts',(31.4772782250561,-2.97376254982325,-1.25348205321784));
#73303=CARTESIAN_POINT('Ctrl Pts',(31.4870070420694,-2.90421593163919,-1.40712443249551));
#73304=CARTESIAN_POINT('Ctrl Pts',(31.4983639603198,-2.81350154599667,-1.57185038242648));
#73305=CARTESIAN_POINT('Ctrl Pts',(31.4995575221663,-2.80385428208745,-1.58899518952283));
#73306=CARTESIAN_POINT('Ctrl Pts',(31.5013222411697,-2.78942770440681,-1.61409315248506));
#73307=CARTESIAN_POINT('Ctrl Pts',(31.501889004364,-2.78476992405964,-1.62211592995961));
#73308=CARTESIAN_POINT('Ctrl Pts',(31.5029008938608,-2.77641087703687,-1.63637182644417));
#73309=CARTESIAN_POINT('Ctrl Pts',(31.5033455277716,-2.7727230822145,-1.6426128029758));
#73310=CARTESIAN_POINT('Ctrl Pts',(31.504276350482,-2.76497227876,-1.65562926867469));
#73311=CARTESIAN_POINT('Ctrl Pts',(31.5047626804751,-2.76090535392729,-1.66240235878185));
#73312=CARTESIAN_POINT('Ctrl Pts',(31.5060327838787,-2.75023935423209,-1.68001850480032));
#73313=CARTESIAN_POINT('Ctrl Pts',(31.5068179938066,-2.74360109905355,-1.690837568752));
#73314=CARTESIAN_POINT('Ctrl Pts',(31.5102512664145,-2.71438544528438,-1.7378283417913));
#73315=CARTESIAN_POINT('Ctrl Pts',(31.5129233886671,-2.69115620144992,-1.77358780696242));
#73316=CARTESIAN_POINT('Ctrl Pts',(31.520002316422,-2.62837500581031,-1.86616005695016));
#73317=CARTESIAN_POINT('Ctrl Pts',(31.5244505347263,-2.58769190148283,-1.92217533139614));
#73318=CARTESIAN_POINT('Ctrl Pts',(31.5436413408014,-2.40700544326516,-2.15481510779151));
#73319=CARTESIAN_POINT('Ctrl Pts',(31.5589735989678,-2.25049647183128,-2.31778903304238));
#73320=CARTESIAN_POINT('Ctrl Pts',(31.5847756108577,-1.95831544950045,-2.56432522365094));
#73321=CARTESIAN_POINT('Ctrl Pts',(31.5952579310794,-1.83107788513926,-2.65667643276602));
#73322=CARTESIAN_POINT('Ctrl Pts',(31.6059350802332,-1.68737804616615,-2.74572713596673));
#73323=CARTESIAN_POINT('Ctrl Pts',(31.6066911438714,-1.67712057384789,-2.7520044998854));
#73324=CARTESIAN_POINT('Ctrl Pts',(31.6077793275476,-1.66223455606751,-2.76100029853469));
#73325=CARTESIAN_POINT('Ctrl Pts',(31.6081143823965,-1.65763412973647,-2.76376472602513));
#73326=CARTESIAN_POINT('Ctrl Pts',(31.6087020792051,-1.64953451243075,-2.76860434243004));
#73327=CARTESIAN_POINT('Ctrl Pts',(31.6089550402622,-1.64603827043442,-2.77068441465842));
#73328=CARTESIAN_POINT('Ctrl Pts',(31.6094824795683,-1.63872743769506,-2.77501523667903));
#73329=CARTESIAN_POINT('Ctrl Pts',(31.6097568764401,-1.63491215102918,-2.77726474032212));
#73330=CARTESIAN_POINT('Ctrl Pts',(31.6104767439983,-1.6248721118458,-2.7831565165705));
#73331=CARTESIAN_POINT('Ctrl Pts',(31.6109213728019,-1.61863970631877,-2.78678579712752));
#73332=CARTESIAN_POINT('Ctrl Pts',(31.6128986631237,-1.59078789804133,-2.80287962348328));
#73333=CARTESIAN_POINT('Ctrl Pts',(31.6144169462331,-1.56903562772546,-2.81511413776269));
#73334=CARTESIAN_POINT('Ctrl Pts',(31.6271823437826,-1.38328140962469,-2.91676910785503));
#73335=CARTESIAN_POINT('Ctrl Pts',(31.637659149537,-1.21191015892472,-2.992039842147));
#73336=CARTESIAN_POINT('Ctrl Pts',(31.6625615569337,-0.790150275129712,
-3.13506056100569));
#73337=CARTESIAN_POINT('Ctrl Pts',(31.6769360845876,-0.536273405546267,
-3.18831218615426));
#73338=CARTESIAN_POINT('Ctrl Pts',(31.6932177673185,-0.265140164853087,
-3.21185390674351));
#73339=CARTESIAN_POINT('Ctrl Pts',(31.6940390270914,-0.251499817466008,
-3.21295077125242));
#73340=CARTESIAN_POINT('Ctrl Pts',(31.6962788801574,-0.214400406016497,
-3.21569635809882));
#73341=CARTESIAN_POINT('Ctrl Pts',(31.6977025952015,-0.190929958730246,
-3.21717520620153));
#73342=CARTESIAN_POINT('Ctrl Pts',(31.6997023643734,-0.158129455741269,
-3.21888174196235));
#73343=CARTESIAN_POINT('Ctrl Pts',(31.7002716222817,-0.148811032453913,
-3.21932599580344));
#73344=CARTESIAN_POINT('Ctrl Pts',(31.7012584037785,-0.132690953681515,
-3.22002437866627));
#73345=CARTESIAN_POINT('Ctrl Pts',(31.701675331044,-0.125890144987925,-3.2202974332603));
#73346=CARTESIAN_POINT('Ctrl Pts',(31.7025415457956,-0.111781990224092,
-3.22081912068506));
#73347=CARTESIAN_POINT('Ctrl Pts',(31.7029909350175,-0.104474567262003,
-3.22106443352196));
#73348=CARTESIAN_POINT('Ctrl Pts',(31.7040469771363,-0.0873306738823321,
-3.22158155970496));
#73349=CARTESIAN_POINT('Ctrl Pts',(31.7046542600163,-0.0774937087897892,
-3.22183319153665));
#73350=CARTESIAN_POINT('Ctrl Pts',(31.706632720485,-0.0455178241931978,
-3.22250461561555));
#73351=CARTESIAN_POINT('Ctrl Pts',(31.7080096244559,-0.023376073238716,
-3.22274128495128));
#73352=CARTESIAN_POINT('Ctrl Pts',(31.7112475528611,0.0284229655212935,
-3.2227611202018));
#73353=CARTESIAN_POINT('Ctrl Pts',(31.7131141291294,0.0580779214703715,
-3.22236310234424));
#73354=CARTESIAN_POINT('Ctrl Pts',(31.719700220006,0.16197589124951,-3.21953397939226));
#73355=CARTESIAN_POINT('Ctrl Pts',(31.7244848019074,0.236132105075009,-3.21494563817498));
#73356=CARTESIAN_POINT('Ctrl Pts',(31.7491120463682,0.61129144228927,-3.1786835341629));
#73357=CARTESIAN_POINT('Ctrl Pts',(31.7700875496439,0.906865114661656,-3.107291427219));
#73358=CARTESIAN_POINT('Ctrl Pts',(31.7909228106255,1.20071295762352,-2.99075065622397));
#73359=CARTESIAN_POINT('Ctrl Pts',(31.7918130847609,1.21327464854142,-2.98567676271985));
#73360=CARTESIAN_POINT('Ctrl Pts',(31.7967232695209,1.28260822550317,-2.95716184624025));
#73361=CARTESIAN_POINT('Ctrl Pts',(31.8006849569311,1.33873745854938,-2.93217892504118));
#73362=CARTESIAN_POINT('Ctrl Pts',(31.8051908758082,1.40319891665997,-2.9012500256173));
#73363=CARTESIAN_POINT('Ctrl Pts',(31.8058228817619,1.41225510188272,-2.89685250650147));
#73364=CARTESIAN_POINT('Ctrl Pts',(31.8067720430191,1.42588060306782,-2.89015712768423));
#73365=CARTESIAN_POINT('Ctrl Pts',(31.8070911129435,1.43046519599901,-2.88789075984663));
#73366=CARTESIAN_POINT('Ctrl Pts',(31.8076600393183,1.43864785995965,-2.88382143929574));
#73367=CARTESIAN_POINT('Ctrl Pts',(31.8079101535613,1.44224795455179,-2.88202265725333));
#73368=CARTESIAN_POINT('Ctrl Pts',(31.8084463865298,1.44997245888146,-2.87814502112768));
#73369=CARTESIAN_POINT('Ctrl Pts',(31.8087323689451,1.45409575697795,-2.876064050805));
#73370=CARTESIAN_POINT('Ctrl Pts',(31.8095160601535,1.4654046027778,-2.87032609950894));
#73371=CARTESIAN_POINT('Ctrl Pts',(31.8100126378669,1.47258098276264,-2.86665097628697));
#73372=CARTESIAN_POINT('Ctrl Pts',(31.8126323433805,1.51049089476066,-2.8470568616918));
#73373=CARTESIAN_POINT('Ctrl Pts',(31.814727106725,1.54098167602527,-2.83066974775283));
#73374=CARTESIAN_POINT('Ctrl Pts',(31.8207786512525,1.62933845920627,-2.78133190081705));
#73375=CARTESIAN_POINT('Ctrl Pts',(31.8246669260992,1.68645693630787,-2.74707392341374));
#73376=CARTESIAN_POINT('Ctrl Pts',(31.8427016850797,1.95018427174449,-2.57756929056213));
#73377=CARTESIAN_POINT('Ctrl Pts',(31.8561150851861,2.14186907493889,-2.4206389240634));
#73378=CARTESIAN_POINT('Ctrl Pts',(31.8736881265182,2.35649858237966,-2.19927288952568));
#73379=CARTESIAN_POINT('Ctrl Pts',(31.8772201950863,2.39796499777074,-2.15398470951607));
#73380=CARTESIAN_POINT('Ctrl Pts',(31.8810498038622,2.44093154423135,-2.10427882129607));
#73381=CARTESIAN_POINT('Ctrl Pts',(31.8813013979548,2.44374526815775,-2.10101052484569));
#73382=CARTESIAN_POINT('Ctrl Pts',(31.8862195519977,2.49857006570099,-2.03706935090795));
#73383=CARTESIAN_POINT('Ctrl Pts',(31.8909627159985,2.54830949233569,-1.97449260278181));
#73384=CARTESIAN_POINT('Ctrl Pts',(31.896698437439,2.60446459142978,-1.89818385869962));
#73385=CARTESIAN_POINT('Ctrl Pts',(31.8975999434085,2.61317716950491,-1.8861714765036));
#73386=CARTESIAN_POINT('Ctrl Pts',(31.8990700969091,2.62719960047433,-1.86655453585588));
#73387=CARTESIAN_POINT('Ctrl Pts',(31.8996367843073,2.63256019793536,-1.85898638442272));
#73388=CARTESIAN_POINT('Ctrl Pts',(31.9006473799141,2.64204047266189,-1.84547878637101));
#73389=CARTESIAN_POINT('Ctrl Pts',(31.9010907919559,2.64617299230767,-1.8395483966338));
#73390=CARTESIAN_POINT('Ctrl Pts',(31.9020253557007,2.65482585172728,-1.82704158194553));
#73391=CARTESIAN_POINT('Ctrl Pts',(31.9025166715137,2.65934178008565,-1.82046217758512));
#73392=CARTESIAN_POINT('Ctrl Pts',(31.9038140205991,2.671179125355,-1.80307792139402));
#73393=CARTESIAN_POINT('Ctrl Pts',(31.90462160638,2.67845936542319,-1.79224533199922));
#73394=CARTESIAN_POINT('Ctrl Pts',(31.9082932948113,2.71115726008248,-1.74294848642564));
#73395=CARTESIAN_POINT('Ctrl Pts',(31.9111857781073,2.73581248610222,-1.70398732405315));
#73396=CARTESIAN_POINT('Ctrl Pts',(31.9189876779968,2.79936400734458,-1.59862420252664));
#73397=CARTESIAN_POINT('Ctrl Pts',(31.9239497257552,2.83673020597455,-1.53133875064609));
#73398=CARTESIAN_POINT('Ctrl Pts',(31.9498188143069,3.0161655111583,-1.17908223516967));
#73399=CARTESIAN_POINT('Ctrl Pts',(31.9719797483963,3.11781930780934,-0.875584491674431));
#73400=CARTESIAN_POINT('Ctrl Pts',(31.996399167963,3.18305669505688,-0.507314728790725));
#73401=CARTESIAN_POINT('Ctrl Pts',(31.9999821251394,3.19134754878536,-0.452238746554153));
#73402=CARTESIAN_POINT('Ctrl Pts',(32.0040528369765,3.19930665256675,-0.388116136712351));
#73403=CARTESIAN_POINT('Ctrl Pts',(32.0046130908301,3.20036907026165,-0.379255865179498));
#73404=CARTESIAN_POINT('Ctrl Pts',(32.0055029445585,3.20200396159674,-0.365125041287943));
#73405=CARTESIAN_POINT('Ctrl Pts',(32.005833851441,3.20260024675012,-0.359857369428019));
#73406=CARTESIAN_POINT('Ctrl Pts',(32.0064167583648,3.20363002126332,-0.350554869469031));
#73407=CARTESIAN_POINT('Ctrl Pts',(32.0066690611967,3.20406889103615,-0.346520665869661));
#73408=CARTESIAN_POINT('Ctrl Pts',(32.0071977630978,3.20497415104665,-0.338050511253339));
#73409=CARTESIAN_POINT('Ctrl Pts',(32.0074740712038,3.20543895129553,-0.333614428838062));
#73410=CARTESIAN_POINT('Ctrl Pts',(32.008204445718,3.20664548457706,-0.321863868530349));
#73411=CARTESIAN_POINT('Ctrl Pts',(32.0086576250436,3.20737140583532,-0.314547740655233));
#73412=CARTESIAN_POINT('Ctrl Pts',(32.0107279953892,3.21058303116174,-0.281012095937483));
#73413=CARTESIAN_POINT('Ctrl Pts',(32.0123290913117,3.21277239367324,-0.254764300912664));
#73414=CARTESIAN_POINT('Ctrl Pts',(32.0264792356516,3.22943426055764,-0.0203491551274071));
#73415=CARTESIAN_POINT('Ctrl Pts',(32.0380755920255,3.22398056375685,0.188769188707624));
#73416=CARTESIAN_POINT('Ctrl Pts',(32.0640333990523,3.16691323639598,0.649778777265243));
#73417=CARTESIAN_POINT('Ctrl Pts',(32.0783918428295,3.10538295617856,0.898957528271592));
#73418=CARTESIAN_POINT('Ctrl Pts',(32.0950041113787,3.00826288004313,1.15621872492417));
#73419=CARTESIAN_POINT('Ctrl Pts',(32.0961709871799,3.00131092428477,1.17414650119475));
#73420=CARTESIAN_POINT('Ctrl Pts',(32.0979096866292,2.99076262547037,1.20064266146669));
#73421=CARTESIAN_POINT('Ctrl Pts',(32.0984773718535,2.98728889997552,1.20925965271242));
#73422=CARTESIAN_POINT('Ctrl Pts',(32.0994890887956,2.98104569454348,1.22455559563851));
#73423=CARTESIAN_POINT('Ctrl Pts',(32.0999326203038,2.97829089676763,1.23124050154442));
#73424=CARTESIAN_POINT('Ctrl Pts',(32.1008667622713,2.97245167289945,1.24527593671515));
#73425=CARTESIAN_POINT('Ctrl Pts',(32.1013575343809,2.96936242747509,1.25262439652089));
#73426=CARTESIAN_POINT('Ctrl Pts',(32.1026519136461,2.96115855889027,1.27193823797456));
#73427=CARTESIAN_POINT('Ctrl Pts',(32.1034570604981,2.95599871316007,1.28388414271871));
#73428=CARTESIAN_POINT('Ctrl Pts',(32.1071019687216,2.93238633113737,1.33765379915358));
#73429=CARTESIAN_POINT('Ctrl Pts',(32.1099696062844,2.91311828231345,1.37911160100351));
#73430=CARTESIAN_POINT('Ctrl Pts',(32.1176889196197,2.85945953894696,1.48841984917936));
#73431=CARTESIAN_POINT('Ctrl Pts',(32.1225918677153,2.82353920206244,1.55548300270557));
#73432=CARTESIAN_POINT('Ctrl Pts',(32.1470608962971,2.63534101101962,1.87881284115265));
#73433=CARTESIAN_POINT('Ctrl Pts',(32.1677063064154,2.45041758858012,2.11432602159685));
#73434=CARTESIAN_POINT('Ctrl Pts',(32.1887693412923,2.2204414365796,2.33585356160358));
#73435=CARTESIAN_POINT('Ctrl Pts',(32.1901691111009,2.20494099196384,2.35049086273359));
#73436=CARTESIAN_POINT('Ctrl Pts',(32.1952125600549,2.14826348814997,2.4029581883151));
#73437=CARTESIAN_POINT('Ctrl Pts',(32.1988108140421,2.10624615585131,2.43987133141046));
#73438=CARTESIAN_POINT('Ctrl Pts',(32.2028969345638,2.05642289285425,2.48139522862742));
#73439=CARTESIAN_POINT('Ctrl Pts',(32.2034579057847,2.04953536418456,2.48708708940991));
#73440=CARTESIAN_POINT('Ctrl Pts',(32.2043486812749,2.03852115084044,2.49611242105123));
#73441=CARTESIAN_POINT('Ctrl Pts',(32.2046797967259,2.03440981416464,2.49946442462005));
#73442=CARTESIAN_POINT('Ctrl Pts',(32.2052629435263,2.02713835303626,2.50536307375515));
#73443=CARTESIAN_POINT('Ctrl Pts',(32.205515278486,2.02398167220108,2.50791391897998));
#73444=CARTESIAN_POINT('Ctrl Pts',(32.2060439122908,2.01734689608931,2.51325465150519));
#73445=CARTESIAN_POINT('Ctrl Pts',(32.2063201206667,2.01386783590622,2.51604327914905));
#73446=CARTESIAN_POINT('Ctrl Pts',(32.2070499470418,2.0046425734538,2.52340636026616));
#73447=CARTESIAN_POINT('Ctrl Pts',(32.2075026803392,1.99888646051604,2.52796843864617));
#73448=CARTESIAN_POINT('Ctrl Pts',(32.2095337917484,1.97291511151948,2.5484081845814));
#73449=CARTESIAN_POINT('Ctrl Pts',(32.2110968997592,1.95252526584211,2.5640638635015));
#73450=CARTESIAN_POINT('Ctrl Pts',(32.2161530595648,1.88534548008219,2.61437952181738));
#73451=CARTESIAN_POINT('Ctrl Pts',(32.2195835957846,1.83782282852045,2.64800106618646));
#73452=CARTESIAN_POINT('Ctrl Pts',(32.2229614699496,1.78943610001022,2.68030520771053));
#73453=CARTESIAN_POINT('Origin',(-1.72497344927317,0.,0.));
#73454=CARTESIAN_POINT('',(33.7168658186985,1.789436210378,2.68030513402635));
#73455=CARTESIAN_POINT('',(33.4682079605267,1.78943620863048,2.68030513519304));
#73456=CARTESIAN_POINT('',(-1.72497344927317,1.78943621037804,2.68030513402633));
#73457=CARTESIAN_POINT('',(32.8965734493162,-3.22274986705245,-0.000925696185107025));
#73458=CARTESIAN_POINT('Ctrl Pts',(32.8965734493162,-3.22274986705245,-0.000925696185104952));
#73459=CARTESIAN_POINT('Ctrl Pts',(32.903176172867,-3.22271898196672,-0.108450073561471));
#73460=CARTESIAN_POINT('Ctrl Pts',(32.9097788964179,-3.21730268941124,-0.215823221241665));
#73461=CARTESIAN_POINT('Ctrl Pts',(32.9163816199687,-3.20657144425315,-0.322516876147978));
#73462=CARTESIAN_POINT('Ctrl Pts',(32.9230102303649,-3.19579812583817,-0.42962883754956));
#73463=CARTESIAN_POINT('Ctrl Pts',(32.9296388407611,-3.17966819140822,-0.536055648712403));
#73464=CARTESIAN_POINT('Ctrl Pts',(32.9362674511573,-3.15830363032908,-0.641276649465874));
#73465=CARTESIAN_POINT('Ctrl Pts',(32.9429096034773,-3.13689542250632,-0.746712611529645));
#73466=CARTESIAN_POINT('Ctrl Pts',(32.9495517557973,-3.11023131595963,-0.850937528863337));
#73467=CARTESIAN_POINT('Ctrl Pts',(32.9561939081173,-3.0784830880185,-0.953446086196845));
#73468=CARTESIAN_POINT('Ctrl Pts',(32.9628566866951,-3.04663627047854,-1.05627296925117));
#73469=CARTESIAN_POINT('Ctrl Pts',(32.9695194652728,-3.00967386291915,-1.1573725235921));
#73470=CARTESIAN_POINT('Ctrl Pts',(32.9761822438506,-2.96781633813462,-1.25625783404571));
#73471=CARTESIAN_POINT('Ctrl Pts',(32.9792975170168,-2.94824528046805,-1.30249301214636));
#73472=CARTESIAN_POINT('Ctrl Pts',(32.982412790183,-2.92760472747754,-1.34824447746458));
#73473=CARTESIAN_POINT('Ctrl Pts',(32.9855280633492,-2.90592057306307,-1.39346445435425));
#73474=CARTESIAN_POINT('Ctrl Pts',(32.991700311442,-2.86295805466186,-1.48305817574598));
#73475=CARTESIAN_POINT('Ctrl Pts',(32.9978725595347,-2.8157725799491,-1.57082083560781));
#73476=CARTESIAN_POINT('Ctrl Pts',(33.0040448076275,-2.76454310125707,-1.65632696162078));
#73477=CARTESIAN_POINT('Ctrl Pts',(33.0102086962801,-2.71338300567364,-1.74171728163733));
#73478=CARTESIAN_POINT('Ctrl Pts',(33.0163725849328,-2.65819001359854,-1.8248567729181));
#73479=CARTESIAN_POINT('Ctrl Pts',(33.0225364735854,-2.59919023201414,-1.9053418854112));
#73480=CARTESIAN_POINT('Ctrl Pts',(33.028693835244,-2.5402529258,-1.98574177153449));
#73481=CARTESIAN_POINT('Ctrl Pts',(33.0348511969025,-2.47751709956189,-2.06349251849753));
#73482=CARTESIAN_POINT('Ctrl Pts',(33.0410085585611,-2.41125316454014,-2.1382178885687));
#73483=CARTESIAN_POINT('Ctrl Pts',(33.0471614227074,-2.34503763058292,-2.21288867710229));
#73484=CARTESIAN_POINT('Ctrl Pts',(33.0533142868537,-2.2752993987495,-2.28453815822827));
#73485=CARTESIAN_POINT('Ctrl Pts',(33.059467151,-2.20234974282361,-2.35282238445336));
#73486=CARTESIAN_POINT('Ctrl Pts',(33.0656176841365,-2.12942772384154,-2.42108074123053));
#73487=CARTESIAN_POINT('Ctrl Pts',(33.0717682172731,-2.05329701500797,-2.48597607986439));
#73488=CARTESIAN_POINT('Ctrl Pts',(33.0779187504096,-1.97430577472716,-2.54720126224431));
#73489=CARTESIAN_POINT('Ctrl Pts',(33.0840685986248,-1.89532333088464,-2.60841962660824));
#73490=CARTESIAN_POINT('Ctrl Pts',(33.0902184468401,-1.81348133223696,-2.66596838118307));
#73491=CARTESIAN_POINT('Ctrl Pts',(33.0963682950553,-1.72916024809905,-2.71958129109869));
#73492=CARTESIAN_POINT('Ctrl Pts',(33.1025191034344,-1.64482599907298,-2.77320257149449));
#73493=CARTESIAN_POINT('Ctrl Pts',(33.1086699118135,-1.55801226235647,-2.82288655359849));
#73494=CARTESIAN_POINT('Ctrl Pts',(33.1148207201927,-1.46912678300237,-2.86841141713756));
#73495=CARTESIAN_POINT('Ctrl Pts',(33.1209781065589,-1.38014624499979,-2.91398496727912));
#73496=CARTESIAN_POINT('Ctrl Pts',(33.1271354929251,-1.28908992735148,-2.95539031831274));
#73497=CARTESIAN_POINT('Ctrl Pts',(33.1332928792913,-1.19638826741843,-2.99245261885356));
#73498=CARTESIAN_POINT('Ctrl Pts',(33.1394537020282,-1.10363487169103,-3.02953560346369));
#73499=CARTESIAN_POINT('Ctrl Pts',(33.1456145247652,-1.00923471541523,-3.06227056827951));
#73500=CARTESIAN_POINT('Ctrl Pts',(33.1517753475021,-0.913634220835751,
-3.09053232842141));
#73501=CARTESIAN_POINT('Ctrl Pts',(33.1579464704188,-0.817873893338074,
-3.11884133894226));
#73502=CARTESIAN_POINT('Ctrl Pts',(33.1641175933355,-0.720909640992276,
-3.14266210268172));
#73503=CARTESIAN_POINT('Ctrl Pts',(33.1702887162522,-0.623199056571544,
-3.16192038141196));
#73504=CARTESIAN_POINT('Ctrl Pts',(33.1749842381978,-0.548852426362706,
-3.17657373893411));
#73505=CARTESIAN_POINT('Ctrl Pts',(33.1796797601433,-0.474073939488129,
-3.18858671220633));
#73506=CARTESIAN_POINT('Ctrl Pts',(33.1843752820889,-0.399066287633495,
-3.197946788265));
#73507=CARTESIAN_POINT('Ctrl Pts',(33.1905475301817,-0.300468976946768,
-3.21025057733703));
#73508=CARTESIAN_POINT('Ctrl Pts',(33.1967197782744,-0.201128575823972,
-3.21801190419797));
#73509=CARTESIAN_POINT('Ctrl Pts',(33.2028920263672,-0.10149975673091,-3.22115124790556));
#73510=CARTESIAN_POINT('Ctrl Pts',(33.2090559150198,-0.00200587083171862,
-3.22428633981457));
#73511=CARTESIAN_POINT('Ctrl Pts',(33.2152198036724,0.0977752262974409,
-3.22281187710088));
#73512=CARTESIAN_POINT('Ctrl Pts',(33.2213836923251,0.197381806395091,-3.21669985932853));
#73513=CARTESIAN_POINT('Ctrl Pts',(33.2275410539836,0.296882912238404,-3.21059431362376));
#73514=CARTESIAN_POINT('Ctrl Pts',(33.2336984156422,0.396209437276115,-3.19986100234528));
#73515=CARTESIAN_POINT('Ctrl Pts',(33.2398557773007,0.494898672848096,-3.18452396224509));
#73516=CARTESIAN_POINT('Ctrl Pts',(33.246008641447,0.593515822993007,-3.1691981247556));
#73517=CARTESIAN_POINT('Ctrl Pts',(33.2521615055933,0.691496181225578,-3.14927531055976));
#73518=CARTESIAN_POINT('Ctrl Pts',(33.2583143697396,0.788382106926401,-3.12483139000783));
#73519=CARTESIAN_POINT('Ctrl Pts',(33.2644649028761,0.885231327438567,-3.10039673002403));
#73520=CARTESIAN_POINT('Ctrl Pts',(33.2706154360127,0.980986518567305,-3.07144447318973));
#73521=CARTESIAN_POINT('Ctrl Pts',(33.2767659691492,1.07520106018206,-3.03810142073687));
#73522=CARTESIAN_POINT('Ctrl Pts',(33.2829158173644,1.1694051100967,-3.00476208135527));
#73523=CARTESIAN_POINT('Ctrl Pts',(33.2890656655796,1.26206844210807,-2.96703306339426));
#73524=CARTESIAN_POINT('Ctrl Pts',(33.2952155137948,1.35276137341589,-2.92509046511282));
#73525=CARTESIAN_POINT('Ctrl Pts',(33.301366322174,1.44346846443605,-2.88314131841446));
#73526=CARTESIAN_POINT('Ctrl Pts',(33.3075171305531,1.53220414941774,-2.83697746706725));
#73527=CARTESIAN_POINT('Ctrl Pts',(33.3136679389322,1.61856135924482,-2.78682196935139));
#73528=CARTESIAN_POINT('Ctrl Pts',(33.3198253252984,1.70501092386053,-2.73661283279751));
#73529=CARTESIAN_POINT('Ctrl Pts',(33.3259827116646,1.7890765575395,-2.68240374396516));
#73530=CARTESIAN_POINT('Ctrl Pts',(33.3321400980308,1.87037843184976,-2.62446224666525));
#73531=CARTESIAN_POINT('Ctrl Pts',(33.3383009207678,1.95172567985723,-2.56648841284203));
#73532=CARTESIAN_POINT('Ctrl Pts',(33.3444617435047,2.03030575514491,-2.50477829054302));
#73533=CARTESIAN_POINT('Ctrl Pts',(33.3506225662417,2.10577196599746,-2.43963972539373));
#73534=CARTESIAN_POINT('Ctrl Pts',(33.3567936891584,2.18136434758539,-2.37439225613261));
#73535=CARTESIAN_POINT('Ctrl Pts',(33.3629648120751,2.25383215046458,-2.30570519356653));
#73536=CARTESIAN_POINT('Ctrl Pts',(33.3691359349917,2.32286549967818,-2.23392332744542));
#73537=CARTESIAN_POINT('Ctrl Pts',(33.3738314569373,2.37539201885263,-2.1793054998282));
#73538=CARTESIAN_POINT('Ctrl Pts',(33.378526978883,2.42593093258027,-2.12289670773472));
#73539=CARTESIAN_POINT('Ctrl Pts',(33.3832225008286,2.47436211737472,-2.06486069133026));
#73540=CARTESIAN_POINT('Ctrl Pts',(33.3893947489213,2.53802474986598,-1.98857253940306));
#73541=CARTESIAN_POINT('Ctrl Pts',(33.3955669970141,2.59826801926057,-1.90920313734829));
#73542=CARTESIAN_POINT('Ctrl Pts',(33.4017392451069,2.65477918577529,-1.8270919619095));
#73543=CARTESIAN_POINT('Ctrl Pts',(33.4079031337595,2.71121381587955,-1.74509199448522));
#73544=CARTESIAN_POINT('Ctrl Pts',(33.4140670224121,2.76392614559788,-1.66035798903141));
#73545=CARTESIAN_POINT('Ctrl Pts',(33.4202309110647,2.81264295951523,-1.57326321535508));
#73546=CARTESIAN_POINT('Ctrl Pts',(33.4263882727233,2.86130818678425,-1.48626066707487));
#73547=CARTESIAN_POINT('Ctrl Pts',(33.4325456343818,2.90598609877098,-1.39690269749423));
#73548=CARTESIAN_POINT('Ctrl Pts',(33.4387029960404,2.94644672409517,-1.30559153818063));
#73549=CARTESIAN_POINT('Ctrl Pts',(33.4448558601867,2.98687779582682,-1.21434707513717));
#73550=CARTESIAN_POINT('Ctrl Pts',(33.451008724333,3.02309752986778,-1.12115265475232));
#73551=CARTESIAN_POINT('Ctrl Pts',(33.4571615884793,3.05492229806421,-1.02643427226983));
#73552=CARTESIAN_POINT('Ctrl Pts',(33.4633121216158,3.08673500946175,-0.931751773803268));
#73553=CARTESIAN_POINT('Ctrl Pts',(33.4694626547523,3.11415592522857,-0.83554687173272));
#73554=CARTESIAN_POINT('Ctrl Pts',(33.4756131878889,3.13705021961368,-0.738263829617687));
#73555=CARTESIAN_POINT('Ctrl Pts',(33.4817630361041,3.15994196449776,-0.640991620909962));
#73556=CARTESIAN_POINT('Ctrl Pts',(33.4879128843193,3.17830799068462,-0.542641933681937));
#73557=CARTESIAN_POINT('Ctrl Pts',(33.4940627325345,3.19206409970979,-0.443671439067201));
#73558=CARTESIAN_POINT('Ctrl Pts',(33.5002135409136,3.20582235644969,-0.344685492380201));
#73559=CARTESIAN_POINT('Ctrl Pts',(33.5063643492928,3.21496920663792,-0.245078976067287));
#73560=CARTESIAN_POINT('Ctrl Pts',(33.5125151576719,3.21947218244898,-0.145314930193683));
#73561=CARTESIAN_POINT('Ctrl Pts',(33.5186725440381,3.22397997397121,-0.0454441915796242));
#73562=CARTESIAN_POINT('Ctrl Pts',(33.5248299304043,3.22383395411364,0.0545839782330701));
#73563=CARTESIAN_POINT('Ctrl Pts',(33.5309873167704,3.2190538059926,0.154305400503576));
#73564=CARTESIAN_POINT('Ctrl Pts',(33.5371481395074,3.21427099012257,0.254082476221889));
#73565=CARTESIAN_POINT('Ctrl Pts',(33.5433089622444,3.20484893645769,0.353552031016853));
#73566=CARTESIAN_POINT('Ctrl Pts',(33.5494697849813,3.190859147722,0.452255969445233));
#73567=CARTESIAN_POINT('Ctrl Pts',(33.555640907898,3.17684596968515,0.551124929389278));
#73568=CARTESIAN_POINT('Ctrl Pts',(33.5618120308147,3.15824988339817,0.649225289189306));
#73569=CARTESIAN_POINT('Ctrl Pts',(33.5679831537314,3.13519337651014,0.746109947921181));
#73570=CARTESIAN_POINT('Ctrl Pts',(33.5726786756769,3.11764999979536,0.819828142714125));
#73571=CARTESIAN_POINT('Ctrl Pts',(33.5773741976225,3.09752532918172,0.892842738917816));
#73572=CARTESIAN_POINT('Ctrl Pts',(33.582069719568,3.07489215235679,0.964964151600781));
#73573=CARTESIAN_POINT('Ctrl Pts',(33.5882407086637,3.04514698472547,1.05974817271529));
#73574=CARTESIAN_POINT('Ctrl Pts',(33.5944116977594,3.01096277059836,1.15332235267896));
#73575=CARTESIAN_POINT('Ctrl Pts',(33.6005826868551,2.97245590277785,1.24524032561636));
#73576=CARTESIAN_POINT('Ctrl Pts',(33.6067458895631,2.93399762188527,1.33704231893298));
#73577=CARTESIAN_POINT('Ctrl Pts',(33.612909092271,2.89122768971275,1.42719186031542));
#73578=CARTESIAN_POINT('Ctrl Pts',(33.619072294979,2.84431230542675,1.51525742753433));
#73579=CARTESIAN_POINT('Ctrl Pts',(33.6252293704408,2.79744356281732,1.60323544296687));
#73580=CARTESIAN_POINT('Ctrl Pts',(33.6313864459026,2.74643776143771,1.68913322053688));
#73581=CARTESIAN_POINT('Ctrl Pts',(33.6375435213645,2.69150886839109,1.772539865242));
#73582=CARTESIAN_POINT('Ctrl Pts',(33.6436961230225,2.6366198873276,1.85588590569292));
#73583=CARTESIAN_POINT('Ctrl Pts',(33.6498487246805,2.57781371995906,1.93674405032632));
#73584=CARTESIAN_POINT('Ctrl Pts',(33.6560013263384,2.51534937764723,2.01472952796888));
#73585=CARTESIAN_POINT('Ctrl Pts',(33.66215179013,2.45290674004298,2.09268790771966));
#73586=CARTESIAN_POINT('Ctrl Pts',(33.6683022539216,2.38680872279129,2.16777526396096));
#73587=CARTESIAN_POINT('Ctrl Pts',(33.6744527177132,2.31735611603887,2.23963796046532));
#73588=CARTESIAN_POINT('Ctrl Pts',(33.680601990954,2.24791695328996,2.31148674644293));
#73589=CARTESIAN_POINT('Ctrl Pts',(33.6867512641947,2.1751247975078,2.38011180499616));
#73590=CARTESIAN_POINT('Ctrl Pts',(33.6929005374355,2.09931816608955,2.44519545231591));
#73591=CARTESIAN_POINT('Ctrl Pts',(33.6990516521312,2.02348883369676,2.5102985895166));
#73592=CARTESIAN_POINT('Ctrl Pts',(33.7052027668269,1.94464355533572,2.57185791788098));
#73593=CARTESIAN_POINT('Ctrl Pts',(33.7113538815226,1.86315432946049,2.62959569270879));
#73594=CARTESIAN_POINT('Ctrl Pts',(33.7131911939146,1.83881383640885,2.64684172605761));
#73595=CARTESIAN_POINT('Ctrl Pts',(33.7150285063065,1.81423765800748,2.6637470907295));
#73596=CARTESIAN_POINT('Ctrl Pts',(33.7168658186985,1.789436210378,2.68030513402635));
#73597=CARTESIAN_POINT('Ctrl Pts',(32.4670258968214,1.789436210378,2.68030513402635));
#73598=CARTESIAN_POINT('Ctrl Pts',(32.4731761355784,1.70635327281358,2.73577330257738));
#73599=CARTESIAN_POINT('Ctrl Pts',(32.4793263743353,1.62065793516169,2.78739544615674));
#73600=CARTESIAN_POINT('Ctrl Pts',(32.4854766130923,1.53274485189673,2.83492694464673));
#73601=CARTESIAN_POINT('Ctrl Pts',(32.4916265325084,1.44483633337075,2.88245597514362));
#73602=CARTESIAN_POINT('Ctrl Pts',(32.4977764519246,1.3547106804889,2.92589457653808));
#73603=CARTESIAN_POINT('Ctrl Pts',(32.5039263713407,1.26278750833372,2.96504389028161));
#73604=CARTESIAN_POINT('Ctrl Pts',(32.5100776164577,1.1708445208569,3.00420164320566));
#73605=CARTESIAN_POINT('Ctrl Pts',(32.5162288615748,1.07710364398436,3.03906810147295));
#73606=CARTESIAN_POINT('Ctrl Pts',(32.5223801066918,0.98200389695119,3.06949277713317));
#73607=CARTESIAN_POINT('Ctrl Pts',(32.5285381283277,0.886799383286437,3.09995097013581));
#73608=CARTESIAN_POINT('Ctrl Pts',(32.5346961499636,0.790233425364579,3.12595747949633));
#73609=CARTESIAN_POINT('Ctrl Pts',(32.5408541715995,0.692759459672458,3.14741193578698));
#73610=CARTESIAN_POINT('Ctrl Pts',(32.5470159581728,0.595225899617504,3.16887950906372));
#73611=CARTESIAN_POINT('Ctrl Pts',(32.5531777447461,0.496783654244963,3.18578941460701));
#73612=CARTESIAN_POINT('Ctrl Pts',(32.5593395313194,0.397893539858509,3.1980929150728));
#73613=CARTESIAN_POINT('Ctrl Pts',(32.5655112110428,0.298844650944925,3.21041616961089));
#73614=CARTESIAN_POINT('Ctrl Pts',(32.5716828907662,0.199346889868214,3.21811821901011));
#73615=CARTESIAN_POINT('Ctrl Pts',(32.5778545704896,0.0998633265283507,
3.22120239639093));
#73616=CARTESIAN_POINT('Ctrl Pts',(32.5811809222831,0.0462446450407157,
3.22286467625991));
#73617=CARTESIAN_POINT('Ctrl Pts',(32.5845072740765,-0.00736995105583313,
3.22318641425991));
#73618=CARTESIAN_POINT('Ctrl Pts',(32.58783362587,-0.0609086335585425,3.22217437468211));
#73619=CARTESIAN_POINT('Ctrl Pts',(32.5940058739627,-0.160252915668906,
3.22029647368372));
#73620=CARTESIAN_POINT('Ctrl Pts',(32.6001781220555,-0.259685125527568,
3.21381657148514));
#73621=CARTESIAN_POINT('Ctrl Pts',(32.6063503701483,-0.358743898115725,
3.20272077741172));
#73622=CARTESIAN_POINT('Ctrl Pts',(32.6125142588009,-0.457668509557358,
3.19164001102757));
#73623=CARTESIAN_POINT('Ctrl Pts',(32.6186781474535,-0.556220261123532,
3.17595582638922));
#73624=CARTESIAN_POINT('Ctrl Pts',(32.6248420361061,-0.653938148823915,
3.15570633298042));
#73625=CARTESIAN_POINT('Ctrl Pts',(32.6309993977646,-0.751552562222665,
3.13547828193227));
#73626=CARTESIAN_POINT('Ctrl Pts',(32.6371567594232,-0.848334444220762,
3.11069462070218));
#73627=CARTESIAN_POINT('Ctrl Pts',(32.6433141210817,-0.943829238858411,
3.08144510422885));
#73628=CARTESIAN_POINT('Ctrl Pts',(32.649466985228,-1.03925428137959,3.05221695243501));
#73629=CARTESIAN_POINT('Ctrl Pts',(32.6556198493743,-1.13339369159259,3.01852955761725));
#73630=CARTESIAN_POINT('Ctrl Pts',(32.6617727135206,-1.22580531920612,2.98052325639408));
#73631=CARTESIAN_POINT('Ctrl Pts',(32.6679232466572,-1.31818193671698,2.94253135384068));
#73632=CARTESIAN_POINT('Ctrl Pts',(32.6740737797937,-1.40883167097371,2.90022396106922));
#73633=CARTESIAN_POINT('Ctrl Pts',(32.6802243129303,-1.49733054031327,2.85379025430131));
#73634=CARTESIAN_POINT('Ctrl Pts',(32.6863741611455,-1.58581955444775,2.80736171837578));
#73635=CARTESIAN_POINT('Ctrl Pts',(32.6925240093607,-1.67215779521927,2.75680798383333));
#73636=CARTESIAN_POINT('Ctrl Pts',(32.6986738575759,-1.75594507307874,2.70236460582774));
#73637=CARTESIAN_POINT('Ctrl Pts',(32.704824665955,-1.83974543248441,2.64791272768247));
#73638=CARTESIAN_POINT('Ctrl Pts',(32.7109754743341,-1.92099367362728,2.58957023654973));
#73639=CARTESIAN_POINT('Ctrl Pts',(32.7171262827133,-1.99931868428552,2.52761594415901));
#73640=CARTESIAN_POINT('Ctrl Pts',(32.7232836690795,-2.0777274596903,2.46559539469975));
#73641=CARTESIAN_POINT('Ctrl Pts',(32.7294410554456,-2.15320642046319,2.39995560068344));
#73642=CARTESIAN_POINT('Ctrl Pts',(32.7355984418118,-2.22541775868719,2.33101552157417));
#73643=CARTESIAN_POINT('Ctrl Pts',(32.7417592645488,-2.2976693972786,2.26203696775185));
#73644=CARTESIAN_POINT('Ctrl Pts',(32.7479200872858,-2.36664948169988,2.18975477506497));
#73645=CARTESIAN_POINT('Ctrl Pts',(32.7540809100227,-2.43205874772026,2.11452306919015));
#73646=CARTESIAN_POINT('Ctrl Pts',(32.7602520329394,-2.49757737043281,2.03916558464512));
#73647=CARTESIAN_POINT('Ctrl Pts',(32.7664231558561,-2.559512980297,1.96084907777183));
#73648=CARTESIAN_POINT('Ctrl Pts',(32.7725942787728,-2.61760802055093,1.87995899243772));
#73649=CARTESIAN_POINT('Ctrl Pts',(32.7772898007184,-2.66181173195385,1.81841084698782));
#73650=CARTESIAN_POINT('Ctrl Pts',(32.7819853226639,-2.70379281926605,1.75537338245911));
#73651=CARTESIAN_POINT('Ctrl Pts',(32.7866808446095,-2.7434557287003,1.69102579139454));
#73652=CARTESIAN_POINT('Ctrl Pts',(32.7930369414377,-2.79714545601391,1.60392162614735));
#73653=CARTESIAN_POINT('Ctrl Pts',(32.7993930382659,-2.84676563256974,1.51412452493224));
#73654=CARTESIAN_POINT('Ctrl Pts',(32.8057491350941,-2.89204502204965,1.42203837955867));
#73655=CARTESIAN_POINT('Ctrl Pts',(32.8120949271868,-2.93725100293519,1.33010152759587));
#73656=CARTESIAN_POINT('Ctrl Pts',(32.8184407192795,-2.9781300244835,1.23588337090644));
#73657=CARTESIAN_POINT('Ctrl Pts',(32.8247865113722,-3.0144549709217,1.13981524414507));
#73658=CARTESIAN_POINT('Ctrl Pts',(32.8311205920994,-3.05071287849111,1.0439244142327));
#73659=CARTESIAN_POINT('Ctrl Pts',(32.8374546728266,-3.08243331286468,0.94619078659277));
#73660=CARTESIAN_POINT('Ctrl Pts',(32.8437887535538,-3.10943629476629,0.847067583661478));
#73661=CARTESIAN_POINT('Ctrl Pts',(32.8501159540983,-3.13640994558483,0.748052049983551));
#73662=CARTESIAN_POINT('Ctrl Pts',(32.8564431546429,-3.15867623335824,0.647650326955835));
#73663=CARTESIAN_POINT('Ctrl Pts',(32.8627703551874,-3.17610418537993,0.546333017592838));
#73664=CARTESIAN_POINT('Ctrl Pts',(32.8690905736384,-3.19351290558005,0.445127512325509));
#73665=CARTESIAN_POINT('Ctrl Pts',(32.8754107920893,-3.20609385586696,0.343008825151237));
#73666=CARTESIAN_POINT('Ctrl Pts',(32.8817310105403,-3.21376678477098,0.240459176582594));
#73667=CARTESIAN_POINT('Ctrl Pts',(32.8866784901179,-3.21977316878248,0.160183107658706));
#73668=CARTESIAN_POINT('Ctrl Pts',(32.8916259696955,-3.22277300950498,0.07964327837657));
#73669=CARTESIAN_POINT('Ctrl Pts',(32.8965734492731,-3.22274986705265,-0.000925695482814911));
#73670=CARTESIAN_POINT('',(32.6496983329207,-3.22274855022239,0.00295378027726991));
#73671=CARTESIAN_POINT('Ctrl Pts',(32.2229614699496,1.78943610001022,2.68030520771053));
#73672=CARTESIAN_POINT('Ctrl Pts',(32.2311765813675,1.6717578365648,2.75887004136827));
#73673=CARTESIAN_POINT('Ctrl Pts',(32.2390848340268,1.54896895161024,2.82964254777507));
#73674=CARTESIAN_POINT('Ctrl Pts',(32.2606380892181,1.20284676547122,2.99980551990526));
#73675=CARTESIAN_POINT('Ctrl Pts',(32.2742759836249,0.972351721218044,3.08223738364988));
#73676=CARTESIAN_POINT('Ctrl Pts',(32.2893277163545,0.727339594247371,3.13961032517539));
#73677=CARTESIAN_POINT('Ctrl Pts',(32.2897852986577,0.719898064168698,3.14132498398815));
#73678=CARTESIAN_POINT('Ctrl Pts',(32.2919298039605,0.685056870534286,3.14922270076477));
#73679=CARTESIAN_POINT('Ctrl Pts',(32.2936268976391,0.657583863789359,3.15507367912768));
#73680=CARTESIAN_POINT('Ctrl Pts',(32.2960147192698,0.619088017945855,3.16274758200143));
#73681=CARTESIAN_POINT('Ctrl Pts',(32.296695755128,0.608126341141233,3.16487355034997));
#73682=CARTESIAN_POINT('Ctrl Pts',(32.2977951229357,0.590461253158554,3.16820445294952));
#73683=CARTESIAN_POINT('Ctrl Pts',(32.2982123093913,0.583764619345555,3.16944519044626));
#73684=CARTESIAN_POINT('Ctrl Pts',(32.299078609013,0.569873470822747,3.17197339336959));
#73685=CARTESIAN_POINT('Ctrl Pts',(32.2995278224637,0.56267841483191,3.17325762916782));
#73686=CARTESIAN_POINT('Ctrl Pts',(32.3004199791209,0.548405145610037,3.1757551750335));
#73687=CARTESIAN_POINT('Ctrl Pts',(32.3008628927341,0.541327120505095,3.17696932354594));
#73688=CARTESIAN_POINT('Ctrl Pts',(32.3023299333626,0.517909826850498,3.18090574467427));
#73689=CARTESIAN_POINT('Ctrl Pts',(32.3033573074268,0.50155383542279,3.18352566801759));
#73690=CARTESIAN_POINT('Ctrl Pts',(32.3111678022377,0.377548903745032,3.20240959009859));
#73691=CARTESIAN_POINT('Ctrl Pts',(32.3181193383071,0.269169598260056,3.21333370976967));
#73692=CARTESIAN_POINT('Ctrl Pts',(32.3387473180987,-0.0465317649755937,
3.22907143515109));
#73693=CARTESIAN_POINT('Ctrl Pts',(32.3528084420133,-0.254012200876999,
3.21939860024077));
#73694=CARTESIAN_POINT('Ctrl Pts',(32.3741337676163,-0.566280805953381,
3.17445577017493));
#73695=CARTESIAN_POINT('Ctrl Pts',(32.3814158743773,-0.672623503361394,
3.15363661035685));
#73696=CARTESIAN_POINT('Ctrl Pts',(32.3893345942766,-0.789744375024898,
3.12451194039179));
#73697=CARTESIAN_POINT('Ctrl Pts',(32.3901450609702,-0.801749793785433,
3.12145291808912));
#73698=CARTESIAN_POINT('Ctrl Pts',(32.3944323840439,-0.86537017552225,3.10485096321226));
#73699=CARTESIAN_POINT('Ctrl Pts',(32.3978625638344,-0.916664051078385,
3.09009593110946));
#73700=CARTESIAN_POINT('Ctrl Pts',(32.4017791283241,-0.975973399836583,
3.07142818171962));
#73701=CARTESIAN_POINT('Ctrl Pts',(32.4023320924848,-0.984364795491938,
3.06874911100708));
#73702=CARTESIAN_POINT('Ctrl Pts',(32.4032125736964,-0.99775661690011,3.06441300137637));
#73703=CARTESIAN_POINT('Ctrl Pts',(32.4035413556762,-1.00276407480465,3.06277807240332));
#73704=CARTESIAN_POINT('Ctrl Pts',(32.4041218249331,-1.01161729386561,3.05986346756012));
#73705=CARTESIAN_POINT('Ctrl Pts',(32.4043738066516,-1.01546467428422,3.05858880619186));
#73706=CARTESIAN_POINT('Ctrl Pts',(32.4049032317049,-1.0235571911871,3.05589075155576));
#73707=CARTESIAN_POINT('Ctrl Pts',(32.4051805789702,-1.02780175767006,3.05446577269861));
#73708=CARTESIAN_POINT('Ctrl Pts',(32.4059166649045,-1.03908020774752,3.05065321853523));
#73709=CARTESIAN_POINT('Ctrl Pts',(32.4063744915315,-1.0461088810643,3.04825014548098));
#73710=CARTESIAN_POINT('Ctrl Pts',(32.4084570554354,-1.07813981431673,3.03717507125781));
#73711=CARTESIAN_POINT('Ctrl Pts',(32.4100655686224,-1.10304384824495,3.02821931957473));
#73712=CARTESIAN_POINT('Ctrl Pts',(32.4144178833676,-1.17077003623107,3.00291786663811));
#73713=CARTESIAN_POINT('Ctrl Pts',(32.4171305753043,-1.21335963659518,2.98596333271594));
#73714=CARTESIAN_POINT('Ctrl Pts',(32.4262678153603,-1.35739138226532,2.92503466593221));
#73715=CARTESIAN_POINT('Ctrl Pts',(32.4325209947079,-1.45693124112177,2.8767505783729));
#73716=CARTESIAN_POINT('Ctrl Pts',(32.4460187442791,-1.66771884737423,2.76074984021439));
#73717=CARTESIAN_POINT('Ctrl Pts',(32.453233833109,-1.77773956052826,2.69122048375457));
#73718=CARTESIAN_POINT('Ctrl Pts',(32.4705399405685,-2.02659577081193,2.51201646809973));
#73719=CARTESIAN_POINT('Ctrl Pts',(32.4807172636519,-2.16118457848172,2.39720366811364));
#73720=CARTESIAN_POINT('Ctrl Pts',(32.492456832024,-2.29823435826055,2.25932588892734));
#73721=CARTESIAN_POINT('Ctrl Pts',(32.4935366252251,-2.31068247137538,2.24659322857556));
#73722=CARTESIAN_POINT('Ctrl Pts',(32.4951772654397,-2.32935484968002,2.22717466022778));
#73723=CARTESIAN_POINT('Ctrl Pts',(32.4957347067265,-2.33565739310087,2.22056423510824));
#73724=CARTESIAN_POINT('Ctrl Pts',(32.4967066348567,-2.34657314692069,2.20901735571762));
#73725=CARTESIAN_POINT('Ctrl Pts',(32.4971205681824,-2.35119911371783,2.20409299673621));
#73726=CARTESIAN_POINT('Ctrl Pts',(32.4979860413732,-2.36082329750307,2.19378324021374));
#73727=CARTESIAN_POINT('Ctrl Pts',(32.4984377005421,-2.36581864616443,2.18839522918309));
#73728=CARTESIAN_POINT('Ctrl Pts',(32.4993366785394,-2.37570719293694,2.17765595883385));
#73729=CARTESIAN_POINT('Ctrl Pts',(32.4997839741521,-2.38060084324102,2.17230517317434));
#73730=CARTESIAN_POINT('Ctrl Pts',(32.5008306807971,-2.39199030138518,2.15976707389633));
#73731=CARTESIAN_POINT('Ctrl Pts',(32.5014306918399,-2.39847181570245,2.15256692378927));
#73732=CARTESIAN_POINT('Ctrl Pts',(32.5049324961434,-2.4360229292316,2.11047217585016));
#73733=CARTESIAN_POINT('Ctrl Pts',(32.5078646251329,-2.46636186623155,2.07493597288023));
#73734=CARTESIAN_POINT('Ctrl Pts',(32.5185346819283,-2.57277335540922,1.94466319719758));
#73735=CARTESIAN_POINT('Ctrl Pts',(32.5264496047245,-2.64423973926204,1.84631200858033));
#73736=CARTESIAN_POINT('Ctrl Pts',(32.5407152334136,-2.76048784073444,1.6656933844388));
#73737=CARTESIAN_POINT('Ctrl Pts',(32.5469954517289,-2.80756216939516,1.58506175453716));
#73738=CARTESIAN_POINT('Ctrl Pts',(32.563861270865,-2.92387393894476,1.36435501323778));
#73739=CARTESIAN_POINT('Ctrl Pts',(32.5744845067112,-2.98654361969685,1.22109147762472));
#73740=CARTESIAN_POINT('Ctrl Pts',(32.5898837124654,-3.06428734487769,1.00110557192209));
#73741=CARTESIAN_POINT('Ctrl Pts',(32.5948914002713,-3.08737577887558,0.927460139995997));
#73742=CARTESIAN_POINT('Ctrl Pts',(32.6004405126205,-3.11066466246883,0.842614992459523));
#73743=CARTESIAN_POINT('Ctrl Pts',(32.6011202106373,-3.11347654986578,0.832164917042117));
#73744=CARTESIAN_POINT('Ctrl Pts',(32.6021218754553,-3.11756072589531,0.816675998147852));
#73745=CARTESIAN_POINT('Ctrl Pts',(32.6024461335052,-3.11887351482204,0.811648054911674));
#73746=CARTESIAN_POINT('Ctrl Pts',(32.6030207746317,-3.12118349457647,0.802712537983304));
#73747=CARTESIAN_POINT('Ctrl Pts',(32.6032714363748,-3.12218551568387,0.79880625421403));
#73748=CARTESIAN_POINT('Ctrl Pts',(32.6038049884276,-3.12430644504244,0.790473053812531));
#73749=CARTESIAN_POINT('Ctrl Pts',(32.6040877570126,-3.12542327446057,0.786045652245447));
#73750=CARTESIAN_POINT('Ctrl Pts',(32.6048536823619,-3.12842864524872,0.77402391046774));
#73751=CARTESIAN_POINT('Ctrl Pts',(32.6053357921226,-3.13029895605099,0.766424980761924));
#73752=CARTESIAN_POINT('Ctrl Pts',(32.6063975800741,-3.1343700289073,0.749621009189221));
#73753=CARTESIAN_POINT('Ctrl Pts',(32.6069765464908,-3.13655796767299,0.740412895633103));
#73754=CARTESIAN_POINT('Ctrl Pts',(32.6087317352373,-3.14309199999781,0.712365113551878));
#73755=CARTESIAN_POINT('Ctrl Pts',(32.6099011504097,-3.14730923633366,0.693495483819581));
#73756=CARTESIAN_POINT('Ctrl Pts',(32.624621409482,-3.19860803990296,0.453851897613045));
#73757=CARTESIAN_POINT('Ctrl Pts',(32.6370704181691,-3.2225416427767,0.228738105582529));
#73758=CARTESIAN_POINT('Ctrl Pts',(32.6496981158975,-3.22274864554512,0.00295468053696055));
#73759=CARTESIAN_POINT('Ctrl Pts',(32.6496981667624,-3.22274864637881,0.00295377107196897));
#73760=CARTESIAN_POINT('Ctrl Pts',(32.6625673399754,-3.22295954265633,-0.227147234168067));
#73761=CARTESIAN_POINT('Ctrl Pts',(32.6755727780319,-3.19852845568629,-0.456583634416496));
#73762=CARTESIAN_POINT('Ctrl Pts',(32.6903769391481,-3.14658318365223,-0.696688345641234));
#73763=CARTESIAN_POINT('Ctrl Pts',(32.6913194246516,-3.1431778142581,-0.711894372415847));
#73764=CARTESIAN_POINT('Ctrl Pts',(32.692852679855,-3.13747999714007,-0.736498745073295));
#73765=CARTESIAN_POINT('Ctrl Pts',(32.6934412837706,-3.13525524884396,-0.7459126325254));
#73766=CARTESIAN_POINT('Ctrl Pts',(32.6944731721616,-3.13128997221173,-0.762360265232649));
#73767=CARTESIAN_POINT('Ctrl Pts',(32.6949158564687,-3.12956803396871,-0.769398455606417));
#73768=CARTESIAN_POINT('Ctrl Pts',(32.6958087967532,-3.12605296241245,-0.783558790866895));
#73769=CARTESIAN_POINT('Ctrl Pts',(32.6962590710462,-3.12425918945861,-0.790680730901383));
#73770=CARTESIAN_POINT('Ctrl Pts',(32.6971253287643,-3.12076758725303,-0.804346274904442));
#73771=CARTESIAN_POINT('Ctrl Pts',(32.697541189421,-3.11907348066985,-0.810890797008091));
#73772=CARTESIAN_POINT('Ctrl Pts',(32.6985214216944,-3.11503828859942,-0.82627944564835));
#73773=CARTESIAN_POINT('Ctrl Pts',(32.6990863457372,-3.11268011898487,-0.835118995023577));
#73774=CARTESIAN_POINT('Ctrl Pts',(32.7007581312009,-3.10560571050519,-0.861190997037086));
#73775=CARTESIAN_POINT('Ctrl Pts',(32.7018684207584,-3.10078383407627,-0.878394191755366));
#73776=CARTESIAN_POINT('Ctrl Pts',(32.7168056648685,-3.03427294972694,-1.1083135332806));
#73777=CARTESIAN_POINT('Ctrl Pts',(32.7313699228012,-2.95097145910775,-1.31411696454995));
#73778=CARTESIAN_POINT('Ctrl Pts',(32.7534126488163,-2.79770703594818,-1.60316549806046));
#73779=CARTESIAN_POINT('Ctrl Pts',(32.7605947883641,-2.74358964678818,-1.69411327258968));
#73780=CARTESIAN_POINT('Ctrl Pts',(32.7770267228811,-2.60890753017515,-1.89702426789483));
#73781=CARTESIAN_POINT('Ctrl Pts',(32.7862301965882,-2.52542421113345,-2.00682342387298));
#73782=CARTESIAN_POINT('Ctrl Pts',(32.7966196283592,-2.41896787912752,-2.12962979218792));
#73783=CARTESIAN_POINT('Ctrl Pts',(32.7981866898664,-2.40256077640483,-2.14812254219514));
#73784=CARTESIAN_POINT('Ctrl Pts',(32.8001978843017,-2.38102404029111,-2.17184152341822));
#73785=CARTESIAN_POINT('Ctrl Pts',(32.8006558081043,-2.37608766996993,-2.17724102257574));
#73786=CARTESIAN_POINT('Ctrl Pts',(32.8013901879191,-2.36811759528246,-2.18589945786128));
#73787=CARTESIAN_POINT('Ctrl Pts',(32.8016675124697,-2.36509548464485,-2.18916895968573));
#73788=CARTESIAN_POINT('Ctrl Pts',(32.8021967564606,-2.35930422671847,-2.19540830280771));
#73789=CARTESIAN_POINT('Ctrl Pts',(32.8024487590276,-2.35653625001467,-2.19837916492099));
#73790=CARTESIAN_POINT('Ctrl Pts',(32.8030297920326,-2.35013026558368,-2.20522869019298));
#73791=CARTESIAN_POINT('Ctrl Pts',(32.803358513664,-2.34648824400342,-2.20910361073875));
#73792=CARTESIAN_POINT('Ctrl Pts',(32.8044116432076,-2.33476370463092,-2.22151619923804));
#73793=CARTESIAN_POINT('Ctrl Pts',(32.8051332330779,-2.32664394032802,-2.23001878126695));
#73794=CARTESIAN_POINT('Ctrl Pts',(32.8174551558295,-2.18654799573593,-2.37512160650147));
#73795=CARTESIAN_POINT('Ctrl Pts',(32.8281727860812,-2.04277405890123,-2.49985834596524));
#73796=CARTESIAN_POINT('Ctrl Pts',(32.8458443071347,-1.78703973249849,-2.68484421110534));
#73797=CARTESIAN_POINT('Ctrl Pts',(32.8528257549029,-1.6810345315686,-2.75245739061293));
#73798=CARTESIAN_POINT('Ctrl Pts',(32.866414386939,-1.47130746000319,-2.86958244327393));
#73799=CARTESIAN_POINT('Ctrl Pts',(32.8729903885499,-1.36835839841498,-2.92007549617023));
#73800=CARTESIAN_POINT('Ctrl Pts',(32.8821132914348,-1.22599878212761,-2.98071421989086));
#73801=CARTESIAN_POINT('Ctrl Pts',(32.88450168693,-1.1887626386916,-2.99575924523463));
#73802=CARTESIAN_POINT('Ctrl Pts',(32.8885910343187,-1.1251547325655,-3.02008697511983));
#73803=CARTESIAN_POINT('Ctrl Pts',(32.8902799870072,-1.0989251319401,-3.02972968905458));
#73804=CARTESIAN_POINT('Ctrl Pts',(32.8924857299937,-1.06474134905322,-3.04179427568128));
#73805=CARTESIAN_POINT('Ctrl Pts',(32.8929921391112,-1.05689803484748,-3.04452838677206));
#73806=CARTESIAN_POINT('Ctrl Pts',(32.8939907721223,-1.04144121961344,-3.04984957110577));
#73807=CARTESIAN_POINT('Ctrl Pts',(32.8944829292796,-1.03382842934866,-3.05243853289476));
#73808=CARTESIAN_POINT('Ctrl Pts',(32.8954185069251,-1.0193663305556,-3.05729650305064));
#73809=CARTESIAN_POINT('Ctrl Pts',(32.8958617405345,-1.01251892547061,-3.05957105615339));
#73810=CARTESIAN_POINT('Ctrl Pts',(32.8968696750525,-0.996957235469488,
-3.06468233570964));
#73811=CARTESIAN_POINT('Ctrl Pts',(32.8974348390197,-0.988238401577048,
-3.0675049155683));
#73812=CARTESIAN_POINT('Ctrl Pts',(32.8991502205219,-0.961796756548136,
-3.07594053348342));
#73813=CARTESIAN_POINT('Ctrl Pts',(32.9003042466146,-0.944037542640087,
-3.08143736933901));
#73814=CARTESIAN_POINT('Ctrl Pts',(32.9091296214775,-0.808466047018551,
-3.12211751476472));
#73815=CARTESIAN_POINT('Ctrl Pts',(32.9170162020647,-0.688788843543406,
-3.15068223854805));
#73816=CARTESIAN_POINT('Ctrl Pts',(32.9314599585764,-0.472247384519792,
-3.18943877585619));
#73817=CARTESIAN_POINT('Ctrl Pts',(32.9379387836329,-0.375992536273159,
-3.20221247288937));
#73818=CARTESIAN_POINT('Ctrl Pts',(32.9608420599428,-0.0371575738424513,
-3.23168999983551));
#73819=CARTESIAN_POINT('Ctrl Pts',(32.977550850477,0.206613648715612,-3.22529444914199));
#73820=CARTESIAN_POINT('Ctrl Pts',(32.9948892937291,0.474515380555603,-3.18774290089363));
#73821=CARTESIAN_POINT('Ctrl Pts',(32.996631151341,0.501625462550799,-3.18358943069423));
#73822=CARTESIAN_POINT('Ctrl Pts',(32.9988505644776,0.536467328899358,-3.17779525501121));
#73823=CARTESIAN_POINT('Ctrl Pts',(32.9993450589931,0.544249699825903,-3.17647165028942));
#73824=CARTESIAN_POINT('Ctrl Pts',(33.000126233559,0.556576124547202,-3.1743285743681));
#73825=CARTESIAN_POINT('Ctrl Pts',(33.0004139666241,0.561123353245616,-3.17352792071334));
#73826=CARTESIAN_POINT('Ctrl Pts',(33.0009514570549,0.569631081768674,-3.17201106417824));
#73827=CARTESIAN_POINT('Ctrl Pts',(33.0012013422472,0.573591917240838,-3.17129722247786));
#73828=CARTESIAN_POINT('Ctrl Pts',(33.0017679268232,0.58258498537413,-3.16965904700639));
#73829=CARTESIAN_POINT('Ctrl Pts',(33.0020843621892,0.587616347875645,-3.16873015071057));
#73830=CARTESIAN_POINT('Ctrl Pts',(33.0030220665662,0.602551149917696,-3.16593607486007));
#73831=CARTESIAN_POINT('Ctrl Pts',(33.0036413972635,0.612448188572382,-3.16403640007377));
#73832=CARTESIAN_POINT('Ctrl Pts',(33.0080316727549,0.682824626315074,-3.1501854950853));
#73833=CARTESIAN_POINT('Ctrl Pts',(33.0117112728667,0.742963630229042,-3.13654656267067));
#73834=CARTESIAN_POINT('Ctrl Pts',(33.0191069477058,0.865140373449977,-3.10512627443492));
#73835=CARTESIAN_POINT('Ctrl Pts',(33.0228152423561,0.927109021745268,-3.08719075515475));
#73836=CARTESIAN_POINT('Ctrl Pts',(33.0407195724168,1.22681237450783,-2.99060853692969));
#73837=CARTESIAN_POINT('Ctrl Pts',(33.0543494304512,1.45535940758955,-2.88630259273302));
#73838=CARTESIAN_POINT('Ctrl Pts',(33.0730876525826,1.73351806602429,-2.71783527292491));
#73839=CARTESIAN_POINT('Ctrl Pts',(33.0774568399969,1.79613087213766,-2.67686872444748));
#73840=CARTESIAN_POINT('Ctrl Pts',(33.0836758988301,1.88161796906975,-2.61658552704864));
#73841=CARTESIAN_POINT('Ctrl Pts',(33.085459931725,1.90573711377358,-2.59907136632971));
#73842=CARTESIAN_POINT('Ctrl Pts',(33.0885870899223,1.94728587053142,-2.5680113665687));
#73843=CARTESIAN_POINT('Ctrl Pts',(33.0899243877882,1.96482590761348,-2.55461616604637));
#73844=CARTESIAN_POINT('Ctrl Pts',(33.0918730166724,1.99004740172076,-2.53494127857654));
#73845=CARTESIAN_POINT('Ctrl Pts',(33.0924786743277,1.99783987514487,-2.52880441646763));
#73846=CARTESIAN_POINT('Ctrl Pts',(33.093534101271,2.01133742319527,-2.5180732686481));
#73847=CARTESIAN_POINT('Ctrl Pts',(33.0939832142364,2.01705542463182,-2.51349530112615));
#73848=CARTESIAN_POINT('Ctrl Pts',(33.0948499540363,2.02804105958321,-2.50463831338046));
#73849=CARTESIAN_POINT('Ctrl Pts',(33.0952674674882,2.03331088636543,-2.5003620654761));
#73850=CARTESIAN_POINT('Ctrl Pts',(33.0962557923294,2.04573322928038,-2.49021660168074));
#73851=CARTESIAN_POINT('Ctrl Pts',(33.096827178751,2.05287402600598,-2.48433319004402));
#73852=CARTESIAN_POINT('Ctrl Pts',(33.0988274660231,2.07772835918137,-2.46367499712194));
#73853=CARTESIAN_POINT('Ctrl Pts',(33.100262865557,2.0953081989451,-2.44874113225818));
#73854=CARTESIAN_POINT('Ctrl Pts',(33.1026028708073,2.12354950326985,-2.42422369314495));
#73855=CARTESIAN_POINT('Ctrl Pts',(33.1035026695099,2.13431020096048,-2.4147552593629));
#73856=CARTESIAN_POINT('Ctrl Pts',(33.1206723618894,2.33775714586359,-2.2333182224323));
#73857=CARTESIAN_POINT('Ctrl Pts',(33.1379568320403,2.50910827342829,-2.03890729429591));
#73858=CARTESIAN_POINT('Ctrl Pts',(33.1680927302765,2.76139522866264,-1.67206561218137));
#73859=CARTESIAN_POINT('Ctrl Pts',(33.180763473198,2.85378188818997,-1.50898969179775));
#73860=CARTESIAN_POINT('Ctrl Pts',(33.1943201670744,2.94187816157787,-1.31609043810097));
#73861=CARTESIAN_POINT('Ctrl Pts',(33.1959031082151,2.9519880934302,-1.29325463324993));
#73862=CARTESIAN_POINT('Ctrl Pts',(33.197923379484,2.96467535282437,-1.26367308000243));
#73863=CARTESIAN_POINT('Ctrl Pts',(33.1983748617183,2.96749654443497,-1.25703375528059));
#73864=CARTESIAN_POINT('Ctrl Pts',(33.1991013913038,2.97201401083069,-1.24630249206975));
#73865=CARTESIAN_POINT('Ctrl Pts',(33.1993772746335,2.97372416430878,-1.24221647770628));
#73866=CARTESIAN_POINT('Ctrl Pts',(33.1999055373488,2.97698879100295,-1.23437103419365));
#73867=CARTESIAN_POINT('Ctrl Pts',(33.2001579930885,2.97854456632494,-1.23061219657944));
#73868=CARTESIAN_POINT('Ctrl Pts',(33.2007424553745,2.98213606198424,-1.22188823815869));
#73869=CARTESIAN_POINT('Ctrl Pts',(33.2010741413267,2.98416651555158,-1.2169209371141));
#73870=CARTESIAN_POINT('Ctrl Pts',(33.2021464407145,2.99070513343733,-1.20081008825158));
#73871=CARTESIAN_POINT('Ctrl Pts',(33.2028840899951,2.99516342474455,-1.18964622173422));
#73872=CARTESIAN_POINT('Ctrl Pts',(33.2133726722157,3.05796367663419,-1.0297990653307));
#73873=CARTESIAN_POINT('Ctrl Pts',(33.2225014479099,3.10524489560186,-0.876981685410832));
#73874=CARTESIAN_POINT('Ctrl Pts',(33.2428961464341,3.18636220784537,-0.523729532728325));
#73875=CARTESIAN_POINT('Ctrl Pts',(33.2540525353336,3.21298617662333,-0.322358940721574));
#73876=CARTESIAN_POINT('Ctrl Pts',(33.2704018987214,3.22357849386231,-0.0376640062154653));
#73877=CARTESIAN_POINT('Ctrl Pts',(33.2751871762806,3.22349009030975,0.0445758759698111));
#73878=CARTESIAN_POINT('Ctrl Pts',(33.2829377205287,3.21835522125058,0.175067017576471));
#73879=CARTESIAN_POINT('Ctrl Pts',(33.2858405490179,3.21536414677462,0.223364759904355));
#73880=CARTESIAN_POINT('Ctrl Pts',(33.2895833981433,3.21016848981178,0.284801733147738));
#73881=CARTESIAN_POINT('Ctrl Pts',(33.2903917233395,3.20896822566466,0.298021272088014));
#73882=CARTESIAN_POINT('Ctrl Pts',(33.29169315569,3.20691088673237,0.319225003160697));
#73883=CARTESIAN_POINT('Ctrl Pts',(33.292184628672,3.20610557096026,0.32721415632135));
#73884=CARTESIAN_POINT('Ctrl Pts',(33.2931196637426,3.20451970993939,0.342378568573353));
#73885=CARTESIAN_POINT('Ctrl Pts',(33.2935630420846,3.20374489993098,0.3495543883647));
#73886=CARTESIAN_POINT('Ctrl Pts',(33.2945723505152,3.20192939663249,0.365855231564391));
#73887=CARTESIAN_POINT('Ctrl Pts',(33.2951387484922,3.20087379209316,0.37497850041957));
#73888=CARTESIAN_POINT('Ctrl Pts',(33.2968615278343,3.19755173555575,0.402653399892398));
#73889=CARTESIAN_POINT('Ctrl Pts',(33.2980217662429,3.19516291953437,0.421189691110196));
#73890=CARTESIAN_POINT('Ctrl Pts',(33.3070499158732,3.17540885225935,0.564620533241722));
#73891=CARTESIAN_POINT('Ctrl Pts',(33.315144556927,3.15089044560091,0.688404056098711));
#73892=CARTESIAN_POINT('Ctrl Pts',(33.3239498031942,3.11720526846814,0.818053212493782));
#73893=CARTESIAN_POINT('Ctrl Pts',(33.3244688436758,3.11519430753084,0.82567800572603));
#73894=CARTESIAN_POINT('Ctrl Pts',(33.3251944440819,3.11234768496992,0.836312865180888));
#73895=CARTESIAN_POINT('Ctrl Pts',(33.3254004337965,3.11153559058599,0.839329249481283));
#73896=CARTESIAN_POINT('Ctrl Pts',(33.325817361759,3.10988385910074,0.845428978342795));
#73897=CARTESIAN_POINT('Ctrl Pts',(33.3260283046359,3.10904401899641,0.848512264099187));
#73898=CARTESIAN_POINT('Ctrl Pts',(33.3427134654385,3.04228588910754,1.09217006680701));
#73899=CARTESIAN_POINT('Ctrl Pts',(33.3598799716314,2.94867366654491,1.32425269373299));
#73900=CARTESIAN_POINT('Ctrl Pts',(33.3808531683655,2.79761035461309,1.60120531676256));
#73901=CARTESIAN_POINT('Ctrl Pts',(33.3851937538263,2.76419705173627,1.65822133550961));
#73902=CARTESIAN_POINT('Ctrl Pts',(33.3916646254845,2.71074173108212,1.743324962901));
#73903=CARTESIAN_POINT('Ctrl Pts',(33.3938573166705,2.69196420165102,1.77218272966235));
#73904=CARTESIAN_POINT('Ctrl Pts',(33.3965267526353,2.66822976206699,1.80741037928458));
#73905=CARTESIAN_POINT('Ctrl Pts',(33.3970309607682,2.66370750508744,1.81406854141633));
#73906=CARTESIAN_POINT('Ctrl Pts',(33.3978216837897,2.65655272630586,1.82451814953452));
#73907=CARTESIAN_POINT('Ctrl Pts',(33.3981093154309,2.65393695970833,1.82832094561003));
#73908=CARTESIAN_POINT('Ctrl Pts',(33.39864671759,2.6490248736206,1.8354293724626));
#73909=CARTESIAN_POINT('Ctrl Pts',(33.3988966154917,2.64673055639167,1.83873628464068));
#73910=CARTESIAN_POINT('Ctrl Pts',(33.3994633600774,2.64150427428559,1.84623913210516));
#73911=CARTESIAN_POINT('Ctrl Pts',(33.3997799421479,2.63856851149864,1.85043237514224));
#73912=CARTESIAN_POINT('Ctrl Pts',(33.4007394962038,2.62962096770244,1.86314784636808));
#73913=CARTESIAN_POINT('Ctrl Pts',(33.4013803450961,2.62357772554077,1.87164800543243));
#73914=CARTESIAN_POINT('Ctrl Pts',(33.4061089720623,2.57849537198935,1.93441146181875));
#73915=CARTESIAN_POINT('Ctrl Pts',(33.4100892074513,2.53781446909569,1.98748214447525));
#73916=CARTESIAN_POINT('Ctrl Pts',(33.4320365420117,2.30015895988496,2.27830991968861));
#73917=CARTESIAN_POINT('Ctrl Pts',(33.4485434396639,2.07146289119973,2.4880731197027));
#73918=CARTESIAN_POINT('Ctrl Pts',(33.4669551839278,1.8074385196177,2.66822058804784));
#73919=CARTESIAN_POINT('Ctrl Pts',(33.4675809300173,1.79845237115226,2.67428572812347));
#73920=CARTESIAN_POINT('Ctrl Pts',(33.4682079605267,1.78943620863048,2.68030513519304));
#73921=CARTESIAN_POINT('Origin',(-1.72497344927317,0.,0.));
#73922=CARTESIAN_POINT('',(34.9669226703048,1.78943621037804,2.68030513402632));
#73923=CARTESIAN_POINT('',(34.7184445309107,1.78943583648355,2.68030538364725));
#73924=CARTESIAN_POINT('',(-1.72497344927317,1.78943621037804,2.68030513402633));
#73925=CARTESIAN_POINT('',(34.1465734492326,-3.22274894896891,-0.00260277156147679));
#73926=CARTESIAN_POINT('Ctrl Pts',(34.1465734492731,-3.22274894896838,-0.00260277221528181));
#73927=CARTESIAN_POINT('Ctrl Pts',(34.1565886751657,-3.22261829689253,-0.164375991421163));
#73928=CARTESIAN_POINT('Ctrl Pts',(34.1666039010584,-3.21030412491819,-0.325671211582515));
#73929=CARTESIAN_POINT('Ctrl Pts',(34.1766191269511,-3.18603596446093,-0.485069475087369));
#73930=CARTESIAN_POINT('Ctrl Pts',(34.1772832098965,-3.18442680739871,-0.495638749255301));
#73931=CARTESIAN_POINT('Ctrl Pts',(34.1779472928418,-3.18276510569429,-0.506199695768205));
#73932=CARTESIAN_POINT('Ctrl Pts',(34.1786113757872,-3.18105093180358,-0.516751905435821));
#73933=CARTESIAN_POINT('Ctrl Pts',(34.18478362388,-3.16511872544068,-0.614828292505281));
#73934=CARTESIAN_POINT('Ctrl Pts',(34.1909558719727,-3.1446184722633,-0.712339794952678));
#73935=CARTESIAN_POINT('Ctrl Pts',(34.1971281200655,-3.11960177926634,-0.808827732770278));
#73936=CARTESIAN_POINT('Ctrl Pts',(34.2032920087181,-3.09461896785424,-0.905184991274903));
#73937=CARTESIAN_POINT('Ctrl Pts',(34.2094558973707,-3.06513198265442,-1.0005210237516));
#73938=CARTESIAN_POINT('Ctrl Pts',(34.2156197860234,-3.03124385526426,-1.09438487399209));
#73939=CARTESIAN_POINT('Ctrl Pts',(34.2217771476819,-2.99739161230016,-1.18814933100392));
#73940=CARTESIAN_POINT('Ctrl Pts',(34.2279345093405,-2.95914763916692,-1.280444298722));
#73941=CARTESIAN_POINT('Ctrl Pts',(34.234091870999,-2.91666517864518,-1.37083252010545));
#73942=CARTESIAN_POINT('Ctrl Pts',(34.2402447351453,-2.87421374852202,-1.4611547193588));
#73943=CARTESIAN_POINT('Ctrl Pts',(34.2463975992916,-2.827530170422,-1.54957254935167));
#73944=CARTESIAN_POINT('Ctrl Pts',(34.2525504634379,-2.77681600129492,-1.63566819907109));
#73945=CARTESIAN_POINT('Ctrl Pts',(34.2587009965745,-2.72612104520764,-1.72173123149298));
#73946=CARTESIAN_POINT('Ctrl Pts',(34.264851529711,-2.67139875242658,-1.8054734578587));
#73947=CARTESIAN_POINT('Ctrl Pts',(34.2710020628476,-2.61289645317398,-1.88650197123959));
#73948=CARTESIAN_POINT('Ctrl Pts',(34.2771519110628,-2.55440066871804,-1.96752146131206));
#73949=CARTESIAN_POINT('Ctrl Pts',(34.283301759278,-2.49212596895196,-2.04582748703674));
#73950=CARTESIAN_POINT('Ctrl Pts',(34.2894516074932,-2.42636222488437,-2.12105726376121));
#73951=CARTESIAN_POINT('Ctrl Pts',(34.2956024158723,-2.36058821325039,-2.19629878596546));
#73952=CARTESIAN_POINT('Ctrl Pts',(34.3017532242514,-2.29132436123661,-2.26846277812617));
#73953=CARTESIAN_POINT('Ctrl Pts',(34.3079040326306,-2.21889924105963,-2.33722136746287));
#73954=CARTESIAN_POINT('Ctrl Pts',(34.3140614189968,-2.14639666577862,-2.40605349072919));
#73955=CARTESIAN_POINT('Ctrl Pts',(34.320218805363,-2.07072638681877,-2.47147263899648));
#73956=CARTESIAN_POINT('Ctrl Pts',(34.3263761917292,-1.99225200131635,-2.53318959530293));
#73957=CARTESIAN_POINT('Ctrl Pts',(34.3325370144661,-1.91373382010764,-2.59494099517557));
#73958=CARTESIAN_POINT('Ctrl Pts',(34.3386978372031,-1.83240876936569,-2.65298583601607));
#73959=CARTESIAN_POINT('Ctrl Pts',(34.34485865994,-1.74866979764436,-2.70707803753539));
#73960=CARTESIAN_POINT('Ctrl Pts',(34.3510297828567,-1.66479082409277,-2.76126067493014));
#73961=CARTESIAN_POINT('Ctrl Pts',(34.3572009057734,-1.57849024380117,-2.81147725445752));
#73962=CARTESIAN_POINT('Ctrl Pts',(34.3633720286901,-1.49018609934024,-2.85752741926182));
#73963=CARTESIAN_POINT('Ctrl Pts',(34.3680675506356,-1.4229966990001,-2.89256635177913));
#73964=CARTESIAN_POINT('Ctrl Pts',(34.3727630725812,-1.35464785899063,-2.9251940960375));
#73965=CARTESIAN_POINT('Ctrl Pts',(34.3774585945267,-1.28533050100755,-2.9553414465472));
#73966=CARTESIAN_POINT('Ctrl Pts',(34.3836308426195,-1.19421306282511,-2.99497003924548));
#73967=CARTESIAN_POINT('Ctrl Pts',(34.3898030907122,-1.10110082093646,-3.03045051134412));
#73968=CARTESIAN_POINT('Ctrl Pts',(34.395975338805,-1.00640752548339,-3.06157826213056));
#73969=CARTESIAN_POINT('Ctrl Pts',(34.4021392274576,-0.911842478753034,
-3.09266385476568));
#73970=CARTESIAN_POINT('Ctrl Pts',(34.4083031161103,-0.815701043574529,
-3.11940830888991));
#73971=CARTESIAN_POINT('Ctrl Pts',(34.4144670047629,-0.718418278569851,
-3.14165445896215));
#73972=CARTESIAN_POINT('Ctrl Pts',(34.4206243664214,-0.621238527111895,
-3.16387705239699));
#73973=CARTESIAN_POINT('Ctrl Pts',(34.42678172808,-0.522920269676796,-3.18161071535755));
#73974=CARTESIAN_POINT('Ctrl Pts',(34.4329390897385,-0.423914190725676,
-3.19474792767777));
#73975=CARTESIAN_POINT('Ctrl Pts',(34.4390919538848,-0.324980428633079,
-3.20787554420413));
#73976=CARTESIAN_POINT('Ctrl Pts',(34.4452448180311,-0.225360273193283,
-3.21641332816805));
#73977=CARTESIAN_POINT('Ctrl Pts',(34.4513976821774,-0.125514174661367,
-3.22030491637967));
#73978=CARTESIAN_POINT('Ctrl Pts',(34.457548215314,-0.0257059027782921,
-3.22419503026487));
#73979=CARTESIAN_POINT('Ctrl Pts',(34.4636987484505,0.0743277085494085,
-3.22344242902527));
#73980=CARTESIAN_POINT('Ctrl Pts',(34.469849281587,0.174122408527278,-3.21804272024917));
#73981=CARTESIAN_POINT('Ctrl Pts',(34.4759991298022,0.273905995400481,-3.21264361278284));
#73982=CARTESIAN_POINT('Ctrl Pts',(34.4821489780174,0.373450290077414,-3.2025984501153));
#73983=CARTESIAN_POINT('Ctrl Pts',(34.4882988262326,0.472293378652133,-3.18795491294676));
#73984=CARTESIAN_POINT('Ctrl Pts',(34.4944496346118,0.571151899407579,-3.17330908951101));
#73985=CARTESIAN_POINT('Ctrl Pts',(34.5006004429909,0.669308566883421,-3.15406352923284));
#73986=CARTESIAN_POINT('Ctrl Pts',(34.5067512513701,0.766309909212199,-3.13031734582026));
#73987=CARTESIAN_POINT('Ctrl Pts',(34.5129086377362,0.863414989705747,-3.10654576703244));
#73988=CARTESIAN_POINT('Ctrl Pts',(34.5190660241024,0.9593618550203,-3.0782640571445));
#73989=CARTESIAN_POINT('Ctrl Pts',(34.5252234104686,1.05371061257495,-3.04562169473606));
#73990=CARTESIAN_POINT('Ctrl Pts',(34.5313842332056,1.1481120251513,-3.01296111497801));
#73991=CARTESIAN_POINT('Ctrl Pts',(34.5375450559425,1.2409131503258,-2.97593519712689));
#73992=CARTESIAN_POINT('Ctrl Pts',(34.5437058786795,1.33169451185914,-2.93474143487706));
#73993=CARTESIAN_POINT('Ctrl Pts',(34.5498770015962,1.42262764928017,-2.89347880144346));
#73994=CARTESIAN_POINT('Ctrl Pts',(34.5560481245129,1.51153389102886,-2.84803460273548));
#73995=CARTESIAN_POINT('Ctrl Pts',(34.5622192474295,1.59801865523376,-2.79865216488668));
#73996=CARTESIAN_POINT('Ctrl Pts',(34.5669147693752,1.66382371434022,-2.7610777519674));
#73997=CARTESIAN_POINT('Ctrl Pts',(34.5716102913208,1.7282273812905,-2.72122425388253));
#73998=CARTESIAN_POINT('Ctrl Pts',(34.5763058132664,1.79106820649395,-2.67921485554752));
#73999=CARTESIAN_POINT('Ctrl Pts',(34.5824780613592,1.8736722637217,-2.62399364015239));
#74000=CARTESIAN_POINT('Ctrl Pts',(34.5886503094519,1.95386549571327,-2.56485144681597));
#74001=CARTESIAN_POINT('Ctrl Pts',(34.5948225575447,2.03125207158727,-2.50202569614551));
#74002=CARTESIAN_POINT('Ctrl Pts',(34.6009864461973,2.10853383825101,-2.43928503409976));
#74003=CARTESIAN_POINT('Ctrl Pts',(34.60715033485,2.18301616987677,-2.37287100199665));
#74004=CARTESIAN_POINT('Ctrl Pts',(34.6133142235026,2.2543316167588,-2.30306459400982));
#74005=CARTESIAN_POINT('Ctrl Pts',(34.6194715851611,2.32557154710797,-2.23333210462176));
#74006=CARTESIAN_POINT('Ctrl Pts',(34.6256289468197,2.39365095096647,-2.16021468318641));
#74007=CARTESIAN_POINT('Ctrl Pts',(34.6317863084782,2.45823569170938,-2.08403331223523));
#74008=CARTESIAN_POINT('Ctrl Pts',(34.6379391726245,2.5227732579191,-2.00790758632606));
#74009=CARTESIAN_POINT('Ctrl Pts',(34.6440920367709,2.58382095597386,-1.92872269075188));
#74010=CARTESIAN_POINT('Ctrl Pts',(34.6502449009172,2.64108240248834,-1.84683548421791));
#74011=CARTESIAN_POINT('Ctrl Pts',(34.6563954340537,2.69832215552999,-1.76497930061469));
#74012=CARTESIAN_POINT('Ctrl Pts',(34.6625459671902,2.75177825856786,-1.68042319585627));
#74013=CARTESIAN_POINT('Ctrl Pts',(34.6686965003268,2.80119599150795,-1.59355532682734));
#74014=CARTESIAN_POINT('Ctrl Pts',(34.674846348542,2.85060822130569,-1.50669713137549));
#74015=CARTESIAN_POINT('Ctrl Pts',(34.6809961967572,2.8959827603119,-1.41752806103303));
#74016=CARTESIAN_POINT('Ctrl Pts',(34.6871460449724,2.93710995637808,-1.32646246333802));
#74017=CARTESIAN_POINT('Ctrl Pts',(34.6932968533515,2.97824357355398,-1.23538264774704));
#74018=CARTESIAN_POINT('Ctrl Pts',(34.6994476617307,3.01512835184066,-1.14240611258294));
#74019=CARTESIAN_POINT('Ctrl Pts',(34.7055984701098,3.04760246969089,-1.04796791421971));
#74020=CARTESIAN_POINT('Ctrl Pts',(34.711755856476,3.08011131701301,-0.953428718847997));
#74021=CARTESIAN_POINT('Ctrl Pts',(34.7179132428422,3.1081999430433,-0.857425150343363));
#74022=CARTESIAN_POINT('Ctrl Pts',(34.7240706292084,3.13175623607276,-0.760408074864664));
#74023=CARTESIAN_POINT('Ctrl Pts',(34.7302314519454,3.15532567561472,-0.663336855204869));
#74024=CARTESIAN_POINT('Ctrl Pts',(34.7363922746823,3.17435766205571,-0.565251428568188));
#74025=CARTESIAN_POINT('Ctrl Pts',(34.7425530974193,3.18879151375422,-0.466611448969114));
#74026=CARTESIAN_POINT('Ctrl Pts',(34.748724220336,3.20324949717556,-0.367806554786105));
#74027=CARTESIAN_POINT('Ctrl Pts',(34.7548953432527,3.21309394736921,-0.268445688150943));
#74028=CARTESIAN_POINT('Ctrl Pts',(34.7610664661694,3.21831619798967,-0.168992343783121));
#74029=CARTESIAN_POINT('Ctrl Pts',(34.7657619881149,3.2222897361487,-0.0933196716711029));
#74030=CARTESIAN_POINT('Ctrl Pts',(34.7704575100605,3.22358834046245,-0.0175935384480273));
#74031=CARTESIAN_POINT('Ctrl Pts',(34.775153032006,3.22222833773311,0.057983635706201));
#74032=CARTESIAN_POINT('Ctrl Pts',(34.7813254289543,3.22044057552189,0.157331977492349));
#74033=CARTESIAN_POINT('Ctrl Pts',(34.7874978259026,3.2140506716445,0.256772428979356));
#74034=CARTESIAN_POINT('Ctrl Pts',(34.7936702228509,3.20304431621291,0.355843604517699));
#74035=CARTESIAN_POINT('Ctrl Pts',(34.7998342219306,3.19205293550307,0.454779988544348));
#74036=CARTESIAN_POINT('Ctrl Pts',(34.8059982210103,3.17645763513739,0.553347667295676));
#74037=CARTESIAN_POINT('Ctrl Pts',(34.81216222009,3.15629610985148,0.651085577659667));
#74038=CARTESIAN_POINT('Ctrl Pts',(34.8186105721823,3.13520450810396,0.75333226047749));
#74039=CARTESIAN_POINT('Ctrl Pts',(34.8250589242746,3.10911525674017,0.854670299241264));
#74040=CARTESIAN_POINT('Ctrl Pts',(34.8315072763669,3.07813236972921,0.954577747973023));
#74041=CARTESIAN_POINT('Ctrl Pts',(34.8376598941505,3.04857041981027,1.04990324152348));
#74042=CARTESIAN_POINT('Ctrl Pts',(34.8438125119341,3.01455391332712,1.14392599391152));
#74043=CARTESIAN_POINT('Ctrl Pts',(34.8499651297178,2.97622513545598,1.23620447563502));
#74044=CARTESIAN_POINT('Ctrl Pts',(34.8561154399878,2.93791073263305,1.32844834869898));
#74045=CARTESIAN_POINT('Ctrl Pts',(34.8622657502578,2.89528743899897,1.41894885049804));
#74046=CARTESIAN_POINT('Ctrl Pts',(34.8684160605278,2.84854628670866,1.50728285831768));
#74047=CARTESIAN_POINT('Ctrl Pts',(34.8745657092847,2.80181016178826,1.59560736513635));
#74048=CARTESIAN_POINT('Ctrl Pts',(34.8807153580415,2.75095726247121,1.68176545766543));
#74049=CARTESIAN_POINT('Ctrl Pts',(34.8868650067984,2.69622487749183,1.76535802954929));
#74050=CARTESIAN_POINT('Ctrl Pts',(34.8930156390435,2.64148373938572,1.84896397005169));
#74051=CARTESIAN_POINT('Ctrl Pts',(34.8991662712886,2.58286212168719,1.9300032119258));
#74052=CARTESIAN_POINT('Ctrl Pts',(34.9053169035337,2.52064041971634,2.00810593271178));
#74053=CARTESIAN_POINT('Ctrl Pts',(34.9114734788998,2.45835859529171,2.08628412117337));
#74054=CARTESIAN_POINT('Ctrl Pts',(34.9176300542659,2.39247001439353,2.16151978498113));
#74055=CARTESIAN_POINT('Ctrl Pts',(34.923786629632,2.32329494304472,2.23347670015222));
#74056=CARTESIAN_POINT('Ctrl Pts',(34.9299466888311,2.25408072746688,2.30547433371958));
#74057=CARTESIAN_POINT('Ctrl Pts',(34.9361067480301,2.18157663311518,2.37418922553548));
#74058=CARTESIAN_POINT('Ctrl Pts',(34.9422668072292,2.10613788409193,2.43932383575711));
#74059=CARTESIAN_POINT('Ctrl Pts',(34.9484355437554,2.0305928687687,2.50455019742104));
#74060=CARTESIAN_POINT('Ctrl Pts',(34.9546042802815,1.95210528873003,2.56618594352339));
#74061=CARTESIAN_POINT('Ctrl Pts',(34.9607730168077,1.87106114828943,2.62397556045437));
#74062=CARTESIAN_POINT('Ctrl Pts',(34.9628229013067,1.84413000501173,2.64317917523849));
#74063=CARTESIAN_POINT('Ctrl Pts',(34.9648727858058,1.81691676947684,2.66195845143838));
#74064=CARTESIAN_POINT('Ctrl Pts',(34.9669226703048,1.78943621037804,2.68030513402632));
#74065=CARTESIAN_POINT('Ctrl Pts',(33.7168658186985,1.789436210378,2.68030513402635));
#74066=CARTESIAN_POINT('Ctrl Pts',(33.7230240742904,1.7063073672797,2.73580395021653));
#74067=CARTESIAN_POINT('Ctrl Pts',(33.7291823298824,1.6206459620611,2.78739728776321));
#74068=CARTESIAN_POINT('Ctrl Pts',(33.7353405854743,1.53286051683291,2.83486440565237));
#74069=CARTESIAN_POINT('Ctrl Pts',(33.741502718378,1.44501980083312,2.88236140940956));
#74070=CARTESIAN_POINT('Ctrl Pts',(33.7476648512817,1.35505277321614,2.92572683291559));
#74071=CARTESIAN_POINT('Ctrl Pts',(33.7538269841854,1.2633891756319,2.96478757306424));
#74072=CARTESIAN_POINT('Ctrl Pts',(33.7599988749213,1.17158042733207,3.00391016649526));
#74073=CARTESIAN_POINT('Ctrl Pts',(33.7661707656571,1.07807015233765,3.03871431759347));
#74074=CARTESIAN_POINT('Ctrl Pts',(33.772342656393,0.983304446662363,3.06907639651965));
#74075=CARTESIAN_POINT('Ctrl Pts',(33.7752007503646,0.939420116285148,3.08313654088349));
#74076=CARTESIAN_POINT('Ctrl Pts',(33.7780588443362,0.895266726279772,3.09624481987067));
#74077=CARTESIAN_POINT('Ctrl Pts',(33.7809169383078,0.850889225077483,3.10839268580195));
#74078=CARTESIAN_POINT('Ctrl Pts',(33.7870891864005,0.75505299650007,3.13462682753091));
#74079=CARTESIAN_POINT('Ctrl Pts',(33.7932614344933,0.657833694385125,3.15647083783526));
#74080=CARTESIAN_POINT('Ctrl Pts',(33.7994336825861,0.559670010758543,3.17378118993064));
#74081=CARTESIAN_POINT('Ctrl Pts',(33.8055975712387,0.461639276006399,3.1910680975938));
#74082=CARTESIAN_POINT('Ctrl Pts',(33.8117614598913,0.362667125967397,3.20383347660308));
#74083=CARTESIAN_POINT('Ctrl Pts',(33.817925348544,0.263206581153961,3.21198378858568));
#74084=CARTESIAN_POINT('Ctrl Pts',(33.8240827102025,0.163851355956706,3.22012547013367));
#74085=CARTESIAN_POINT('Ctrl Pts',(33.8302400718611,0.0640091946955882,
3.22366176506024));
#74086=CARTESIAN_POINT('Ctrl Pts',(33.8363974335196,-0.0358584933163507,
3.22255050091648));
#74087=CARTESIAN_POINT('Ctrl Pts',(33.8425502976659,-0.135653235125919,
3.2214400484717));
#74088=CARTESIAN_POINT('Ctrl Pts',(33.8487031618122,-0.235473033576979,
3.21568879103823));
#74089=CARTESIAN_POINT('Ctrl Pts',(33.8548560259586,-0.334854106241301,
3.2053065828456));
#74090=CARTESIAN_POINT('Ctrl Pts',(33.8610065590951,-0.434197528431681,
3.1949283079478));
#74091=CARTESIAN_POINT('Ctrl Pts',(33.8671570922316,-0.533102123551234,
3.17992261342375));
#74092=CARTESIAN_POINT('Ctrl Pts',(33.8733076253682,-0.631107756398591,
3.16035133526536));
#74093=CARTESIAN_POINT('Ctrl Pts',(33.8794574735834,-0.729102475371115,
3.14078223655803));
#74094=CARTESIAN_POINT('Ctrl Pts',(33.8856073217986,-0.826198005135701,
3.1166486500967));
#74095=CARTESIAN_POINT('Ctrl Pts',(33.8917571700138,-0.921943947047824,
3.08806361997318));
#74096=CARTESIAN_POINT('Ctrl Pts',(33.8979079783929,-1.01770483758911,3.05947412692407));
#74097=CARTESIAN_POINT('Ctrl Pts',(33.9040587867721,-1.11211530549546,3.02643193404758));
#74098=CARTESIAN_POINT('Ctrl Pts',(33.9102095951512,-1.20474064021909,2.98909978961969));
#74099=CARTESIAN_POINT('Ctrl Pts',(33.9163669815174,-1.29746503318267,2.95172772029943));
#74100=CARTESIAN_POINT('Ctrl Pts',(33.9225243678836,-1.38840007699535,2.91005670057734));
#74101=CARTESIAN_POINT('Ctrl Pts',(33.9286817542498,-1.47713168170983,2.86429739332163));
#74102=CARTESIAN_POINT('Ctrl Pts',(33.9348425769867,-1.56591280657373,2.8185125482912));
#74103=CARTESIAN_POINT('Ctrl Pts',(33.9410033997237,-1.65248766698527,2.76863508874169));
#74104=CARTESIAN_POINT('Ctrl Pts',(33.9471642224607,-1.73646922583916,2.71492029168695));
#74105=CARTESIAN_POINT('Ctrl Pts',(33.9533353453774,-1.8205911921008,2.66111568973319));
#74106=CARTESIAN_POINT('Ctrl Pts',(33.9595064682941,-1.90211084157241,2.60346118628263));
#74107=CARTESIAN_POINT('Ctrl Pts',(33.9656775912107,-1.98067231111727,2.54225387372571));
#74108=CARTESIAN_POINT('Ctrl Pts',(33.9703731131563,-2.04044864506884,2.49568207743832));
#74109=CARTESIAN_POINT('Ctrl Pts',(33.9750686351019,-2.09851299431253,2.44705425646063));
#74110=CARTESIAN_POINT('Ctrl Pts',(33.9797641570475,-2.15472311950254,2.39651535375454));
#74111=CARTESIAN_POINT('Ctrl Pts',(33.9858444085629,-2.22750985180378,2.33107231178245));
#74112=CARTESIAN_POINT('Ctrl Pts',(33.9919246600783,-2.29745886960337,2.26217825259532));
#74113=CARTESIAN_POINT('Ctrl Pts',(33.9980049115937,-2.36421738820502,2.19011271486402));
#74114=CARTESIAN_POINT('Ctrl Pts',(34.0041952673286,-2.43218480327599,2.11674217852059));
#74115=CARTESIAN_POINT('Ctrl Pts',(34.0103856230635,-2.49684463175334,2.04008441524718));
#74116=CARTESIAN_POINT('Ctrl Pts',(34.0165759787985,-2.55785923176369,1.96047792973583));
#74117=CARTESIAN_POINT('Ctrl Pts',(34.022640822498,-2.617636735399,1.88248549880549));
#74118=CARTESIAN_POINT('Ctrl Pts',(34.0287056661975,-2.67391512789858,1.80166315333502));
#74119=CARTESIAN_POINT('Ctrl Pts',(34.034770509897,-2.72641465857697,1.71836569798068));
#74120=CARTESIAN_POINT('Ctrl Pts',(34.0408315863062,-2.77888157819644,1.63511998438839));
#74121=CARTESIAN_POINT('Ctrl Pts',(34.0468926627153,-2.82757405851386,1.54940259201758));
#74122=CARTESIAN_POINT('Ctrl Pts',(34.0529537391245,-2.87225467075501,1.46159866886435));
#74123=CARTESIAN_POINT('Ctrl Pts',(34.0590127840448,-2.91692030741171,1.3738241749199));
#74124=CARTESIAN_POINT('Ctrl Pts',(34.0650718289652,-2.95757654445578,1.28396493903239));
#74125=CARTESIAN_POINT('Ctrl Pts',(34.0711308738856,-2.99403166642841,1.1924311061541));
#74126=CARTESIAN_POINT('Ctrl Pts',(34.0774177551645,-3.03185759887512,1.09745535537644));
#74127=CARTESIAN_POINT('Ctrl Pts',(34.0837046364434,-3.06516000806082,1.00067704311448));
#74128=CARTESIAN_POINT('Ctrl Pts',(34.0899915177224,-3.09377983211648,0.902576264306415));
#74129=CARTESIAN_POINT('Ctrl Pts',(34.0960543632788,-3.12137977641379,0.80797134900856));
#74130=CARTESIAN_POINT('Ctrl Pts',(34.1021172088352,-3.14462512716138,0.712137083011762));
#74131=CARTESIAN_POINT('Ctrl Pts',(34.1081800543917,-3.16342477300057,0.61551707374071));
#74132=CARTESIAN_POINT('Ctrl Pts',(34.1142454973404,-3.18223247282267,0.51885567135453));
#74133=CARTESIAN_POINT('Ctrl Pts',(34.1203109402891,-3.19659061145951,0.421408298975774));
#74134=CARTESIAN_POINT('Ctrl Pts',(34.1263763832378,-3.20645977270616,0.323625228493059));
#74135=CARTESIAN_POINT('Ctrl Pts',(34.1324486615409,-3.21634005584711,0.225731962934236));
#74136=CARTESIAN_POINT('Ctrl Pts',(34.1385209398441,-3.22172124882492,0.127502691283429));
#74137=CARTESIAN_POINT('Ctrl Pts',(34.1445932181473,-3.22261599848899,0.0293885825244143));
#74138=CARTESIAN_POINT('Ctrl Pts',(34.1452532951757,-3.22271326078001,0.0187232496582979));
#74139=CARTESIAN_POINT('Ctrl Pts',(34.1459133722042,-3.22275755989923,0.00805927310546678));
#74140=CARTESIAN_POINT('Ctrl Pts',(34.1465734492326,-3.22274894896891,-0.00260277156152148));
#74141=CARTESIAN_POINT('Ctrl Pts',(33.4682079605267,1.78943620863048,2.68030513519304));
#74142=CARTESIAN_POINT('Ctrl Pts',(33.4719380796925,1.73580028482111,2.71611376865332));
#74143=CARTESIAN_POINT('Ctrl Pts',(33.4757140711437,1.68110222134406,2.7503039548369));
#74144=CARTESIAN_POINT('Ctrl Pts',(33.4822462518313,1.58621665213048,2.80572540357671));
#74145=CARTESIAN_POINT('Ctrl Pts',(33.4849724197114,1.54654012316622,2.82778917906105));
#74146=CARTESIAN_POINT('Ctrl Pts',(33.4885168940229,1.49493702531806,2.85507431585235));
#74147=CARTESIAN_POINT('Ctrl Pts',(33.4893075168186,1.48342536161371,2.86107239466536));
#74148=CARTESIAN_POINT('Ctrl Pts',(33.4905872050483,1.4647927675562,2.87063810685974));
#74149=CARTESIAN_POINT('Ctrl Pts',(33.4910747334261,1.45769422095793,2.87424921480799));
#74150=CARTESIAN_POINT('Ctrl Pts',(33.4920067407488,1.44412439818775,2.88108913212089));
#74151=CARTESIAN_POINT('Ctrl Pts',(33.4924510542796,1.43765548808053,2.88432254799983));
#74152=CARTESIAN_POINT('Ctrl Pts',(33.4934687704669,1.42283905956801,2.89166615425891));
#74153=CARTESIAN_POINT('Ctrl Pts',(33.4940426704232,1.41448454374745,2.89576200847203));
#74154=CARTESIAN_POINT('Ctrl Pts',(33.4958108007527,1.38874798984052,2.90824156572417));
#74155=CARTESIAN_POINT('Ctrl Pts',(33.4970091921931,1.3713085358095,2.91650524727887));
#74156=CARTESIAN_POINT('Ctrl Pts',(33.5140033041706,1.12409660014393,3.03093910101488));
#74157=CARTESIAN_POINT('Ctrl Pts',(33.5307812868111,0.882719776687108,3.10981336198634));
#74158=CARTESIAN_POINT('Ctrl Pts',(33.5579610837558,0.488602770142272,3.18897767916929));
#74159=CARTESIAN_POINT('Ctrl Pts',(33.5680903139525,0.340681186009445,3.2081538041494));
#74160=CARTESIAN_POINT('Ctrl Pts',(33.5817012053634,0.135288220629928,3.22040955632333));
#74161=CARTESIAN_POINT('Ctrl Pts',(33.5854134154499,0.0785340083628635,
3.22229325493868));
#74162=CARTESIAN_POINT('Ctrl Pts',(33.5910489641831,-0.00920999557223865,
3.2228856165061));
#74163=CARTESIAN_POINT('Ctrl Pts',(33.5930180482641,-0.0401791499890595,
3.22264834064953));
#74164=CARTESIAN_POINT('Ctrl Pts',(33.5954518694566,-0.0789131415843825,
3.22179308891856));
#74165=CARTESIAN_POINT('Ctrl Pts',(33.5959387058417,-0.0866843200401143,
3.22159336716264));
#74166=CARTESIAN_POINT('Ctrl Pts',(33.5967083012373,-0.0990073252826235,
3.22123203998006));
#74167=CARTESIAN_POINT('Ctrl Pts',(33.5969920808811,-0.103559601571538,
3.22108890212455));
#74168=CARTESIAN_POINT('Ctrl Pts',(33.597526233037,-0.11214425999312,3.22080075574038));
#74169=CARTESIAN_POINT('Ctrl Pts',(33.597776715927,-0.116176625634615,3.2206578264498));
#74170=CARTESIAN_POINT('Ctrl Pts',(33.5983500099586,-0.125420942573093,
3.22031277272218));
#74171=CARTESIAN_POINT('Ctrl Pts',(33.598672532392,-0.130632669263656,3.22010556870806));
#74172=CARTESIAN_POINT('Ctrl Pts',(33.5996681584257,-0.146754592217182,
3.21942540012344));
#74173=CARTESIAN_POINT('Ctrl Pts',(33.600338897959,-0.157663043697437,3.21890962749139));
#74174=CARTESIAN_POINT('Ctrl Pts',(33.6059002209114,-0.248479205585574,
3.21415289479418));
#74175=CARTESIAN_POINT('Ctrl Pts',(33.6106361461237,-0.328213636123482,
3.20699219837407));
#74176=CARTESIAN_POINT('Ctrl Pts',(33.6171305017668,-0.439300996965171,
3.19282838734028));
#74177=CARTESIAN_POINT('Ctrl Pts',(33.618967983285,-0.470935095321453,3.18831596815152));
#74178=CARTESIAN_POINT('Ctrl Pts',(33.6291419685417,-0.646804281906092,
3.16055455472443));
#74179=CARTESIAN_POINT('Ctrl Pts',(33.63724217855,-0.789400686117254,3.1279883233347));
#74180=CARTESIAN_POINT('Ctrl Pts',(33.6577556065832,-1.14033063572142,3.02230644677379));
#74181=CARTESIAN_POINT('Ctrl Pts',(33.6702485155395,-1.34425361407535,2.93728671015791));
#74182=CARTESIAN_POINT('Ctrl Pts',(33.684924566749,-1.55835455903518,2.82102652742668));
#74183=CARTESIAN_POINT('Ctrl Pts',(33.6863346669472,-1.57869298209044,2.8096953615356));
#74184=CARTESIAN_POINT('Ctrl Pts',(33.6883643495246,-1.60762599536752,2.79316255833346));
#74185=CARTESIAN_POINT('Ctrl Pts',(33.6889774921215,-1.61632212697993,2.78813937895873));
#74186=CARTESIAN_POINT('Ctrl Pts',(33.6900417201285,-1.63133875618909,2.77937140294921));
#74187=CARTESIAN_POINT('Ctrl Pts',(33.69049211775,-1.63767022433886,2.7756454686923));
#74188=CARTESIAN_POINT('Ctrl Pts',(33.6913583345557,-1.64980111489311,2.76845074172262));
#74189=CARTESIAN_POINT('Ctrl Pts',(33.6917740300083,-1.65560248133948,2.7649852894219));
#74190=CARTESIAN_POINT('Ctrl Pts',(33.692753447977,-1.66922325877094,2.75679066726143));
#74191=CARTESIAN_POINT('Ctrl Pts',(33.6933177206522,-1.67703350890455,2.7520464527282));
#74192=CARTESIAN_POINT('Ctrl Pts',(33.6949863123481,-1.70001885209107,2.7379501838192));
#74193=CARTESIAN_POINT('Ctrl Pts',(33.6960940411091,-1.71513646251771,2.72850548852349));
#74194=CARTESIAN_POINT('Ctrl Pts',(33.7112833465532,-1.9204797640668,2.59783680653195));
#74195=CARTESIAN_POINT('Ctrl Pts',(33.7261316492658,-2.0975066086757,2.45711771452616));
#74196=CARTESIAN_POINT('Ctrl Pts',(33.7518921242362,-2.37011219506015,2.18934252252009));
#74197=CARTESIAN_POINT('Ctrl Pts',(33.7625696361211,-2.47370592503951,2.07157734027799));
#74198=CARTESIAN_POINT('Ctrl Pts',(33.77767879054,-2.61071967280842,1.89081611880131));
#74199=CARTESIAN_POINT('Ctrl Pts',(33.7822989206574,-2.65127772735827,1.83351318076555));
#74200=CARTESIAN_POINT('Ctrl Pts',(33.7891357767719,-2.70969811537775,1.74497604168268));
#74201=CARTESIAN_POINT('Ctrl Pts',(33.7914230139312,-2.728960886787,1.71469472549758));
#74202=CARTESIAN_POINT('Ctrl Pts',(33.7941913451706,-2.75197679645455,1.67714274692081));
#74203=CARTESIAN_POINT('Ctrl Pts',(33.7947023364444,-2.75621244538718,1.67017275785686));
#74204=CARTESIAN_POINT('Ctrl Pts',(33.7955013003503,-2.76281585073487,1.65921296404043));
#74205=CARTESIAN_POINT('Ctrl Pts',(33.7957904282399,-2.76520149351232,1.65523405778063));
#74206=CARTESIAN_POINT('Ctrl Pts',(33.7963291454886,-2.76963924894492,1.64779615505152));
#74207=CARTESIAN_POINT('Ctrl Pts',(33.7965788687404,-2.77169345683387,1.64433850514248));
#74208=CARTESIAN_POINT('Ctrl Pts',(33.797143312002,-2.77632983038721,1.63650117134253));
#74209=CARTESIAN_POINT('Ctrl Pts',(33.7974577760024,-2.77890810102189,1.63211922904628));
#74210=CARTESIAN_POINT('Ctrl Pts',(33.7983843036132,-2.78649010781804,1.61916305394649));
#74211=CARTESIAN_POINT('Ctrl Pts',(33.7989944968837,-2.79146466324536,1.61057168611753));
#74212=CARTESIAN_POINT('Ctrl Pts',(33.8031770606525,-2.82542481065391,1.55129036973048));
#74213=CARTESIAN_POINT('Ctrl Pts',(33.8066676030247,-2.85306989054627,1.49984011774334));
#74214=CARTESIAN_POINT('Ctrl Pts',(33.8249994655882,-2.99323991185709,1.22105152298918));
#74215=CARTESIAN_POINT('Ctrl Pts',(33.8387685968133,-3.08003661397099,0.981760544420308));
#74216=CARTESIAN_POINT('Ctrl Pts',(33.8626163546827,-3.17630043159713,0.57064695878151));
#74217=CARTESIAN_POINT('Ctrl Pts',(33.8723315943972,-3.20178845264642,0.403809028733365));
#74218=CARTESIAN_POINT('Ctrl Pts',(33.883861381671,-3.21578592624298,0.2129790190033));
#74219=CARTESIAN_POINT('Ctrl Pts',(33.8852449534423,-3.21721447936017,0.190184485174906));
#74220=CARTESIAN_POINT('Ctrl Pts',(33.8872431221123,-3.21891813768289,0.157425799412396));
#74221=CARTESIAN_POINT('Ctrl Pts',(33.8878515543184,-3.21938950802269,0.147472206019382));
#74222=CARTESIAN_POINT('Ctrl Pts',(33.8889102380269,-3.22012759809292,0.130190568843589));
#74223=CARTESIAN_POINT('Ctrl Pts',(33.889359821574,-3.22041548554441,0.122863465972389));
#74224=CARTESIAN_POINT('Ctrl Pts',(33.8902263439641,-3.22092126585149,0.108764286047468));
#74225=CARTESIAN_POINT('Ctrl Pts',(33.890643165549,-3.22114281359467,0.101992372470458));
#74226=CARTESIAN_POINT('Ctrl Pts',(33.891628114379,-3.22161509829806,0.0860147060581472));
#74227=CARTESIAN_POINT('Ctrl Pts',(33.8921968072082,-3.22184773391983,0.0768085141895613));
#74228=CARTESIAN_POINT('Ctrl Pts',(33.8941787487881,-3.22251948245932,0.0447914674210797));
#74229=CARTESIAN_POINT('Ctrl Pts',(33.8955983401279,-3.22275581429867,0.0219774571189312));
#74230=CARTESIAN_POINT('Ctrl Pts',(33.9108867291927,-3.22269236757379,-0.222409689435768));
#74231=CARTESIAN_POINT('Ctrl Pts',(33.9254886145542,-3.19978513449874,-0.443342263224991));
#74232=CARTESIAN_POINT('Ctrl Pts',(33.9504104189607,-3.1240733957462,-0.805123469020129));
#74233=CARTESIAN_POINT('Ctrl Pts',(33.9605006650502,-3.08377248928053,-0.947843055054371));
#74234=CARTESIAN_POINT('Ctrl Pts',(33.9721730153332,-3.02479159950525,-1.11241445468042));
#74235=CARTESIAN_POINT('Ctrl Pts',(33.9739480628578,-3.01547352190336,-1.13743115704715));
#74236=CARTESIAN_POINT('Ctrl Pts',(33.9811360105444,-2.97627737508921,-1.23879444698446));
#74237=CARTESIAN_POINT('Ctrl Pts',(33.9864675844489,-2.94379925103353,-1.31411082859061));
#74238=CARTESIAN_POINT('Ctrl Pts',(33.9923332731715,-2.9037485989655,-1.39802801640957));
#74239=CARTESIAN_POINT('Ctrl Pts',(33.9930234146757,-2.89896580791011,-1.40791885896994));
#74240=CARTESIAN_POINT('Ctrl Pts',(33.9940339776451,-2.89185678254053,-1.42243054999275));
#74241=CARTESIAN_POINT('Ctrl Pts',(33.9943567868124,-2.88956991485426,-1.42707043566162));
#74242=CARTESIAN_POINT('Ctrl Pts',(33.9949304697766,-2.88547704674999,-1.43532438763105));
#74243=CARTESIAN_POINT('Ctrl Pts',(33.9951816145403,-2.88367541347753,-1.43894058093007));
#74244=CARTESIAN_POINT('Ctrl Pts',(33.9957133814653,-2.87983965191445,-1.44660348909123));
#74245=CARTESIAN_POINT('Ctrl Pts',(33.9959938924046,-2.8778037984006,-1.45064929390348));
#74246=CARTESIAN_POINT('Ctrl Pts',(33.9967473774967,-2.87230191772499,-1.46152589040197));
#74247=CARTESIAN_POINT('Ctrl Pts',(33.9972193618536,-2.86882002888239,-1.46834869141606));
#74248=CARTESIAN_POINT('Ctrl Pts',(33.9995106975204,-2.85174542602477,-1.50151399233557));
#74249=CARTESIAN_POINT('Ctrl Pts',(34.0013094608905,-2.8378135070946,-1.52768154079737));
#74250=CARTESIAN_POINT('Ctrl Pts',(34.0062942755146,-2.79778922692071,-1.60041936893558));
#74251=CARTESIAN_POINT('Ctrl Pts',(34.0094373440646,-2.7708971243481,-1.64654076885814));
#74252=CARTESIAN_POINT('Ctrl Pts',(34.0172331602429,-2.7004133406762,-1.76080240005062));
#74253=CARTESIAN_POINT('Ctrl Pts',(34.0218274655985,-2.65537865515775,-1.8280106233033));
#74254=CARTESIAN_POINT('Ctrl Pts',(34.0375782712077,-2.49102974793326,-2.05436867573003));
#74255=CARTESIAN_POINT('Ctrl Pts',(34.0485229735838,-2.35955981635353,-2.20411811531303));
#74256=CARTESIAN_POINT('Ctrl Pts',(34.062319302285,-2.18453738827689,-2.3697442260397));
#74257=CARTESIAN_POINT('Ctrl Pts',(34.064747572999,-2.15338359315616,-2.39808886705959));
#74258=CARTESIAN_POINT('Ctrl Pts',(34.0675486660572,-2.11713261360311,-2.42979497522419));
#74259=CARTESIAN_POINT('Ctrl Pts',(34.0679007827238,-2.11256998412559,-2.43376296849092));
#74260=CARTESIAN_POINT('Ctrl Pts',(34.0730991300267,-2.04513115690436,-2.49208012778898));
#74261=CARTESIAN_POINT('Ctrl Pts',(34.0780270488176,-1.98019140265298,-2.54398605067792));
#74262=CARTESIAN_POINT('Ctrl Pts',(34.0839663727014,-1.90123248354936,-2.60224102056088));
#74263=CARTESIAN_POINT('Ctrl Pts',(34.0848789899186,-1.88908065921275,-2.61107593468888));
#74264=CARTESIAN_POINT('Ctrl Pts',(34.0863637079333,-1.86928283909061,-2.62525927978279));
#74265=CARTESIAN_POINT('Ctrl Pts',(34.0869337834369,-1.8616745195216,-2.63066010709916));
#74266=CARTESIAN_POINT('Ctrl Pts',(34.0879481934027,-1.84812483077425,-2.64019024357382));
#74267=CARTESIAN_POINT('Ctrl Pts',(34.0883920179623,-1.84219278316576,-2.64433274394175));
#74268=CARTESIAN_POINT('Ctrl Pts',(34.0893251830207,-1.82971273657552,-2.65298550366578));
#74269=CARTESIAN_POINT('Ctrl Pts',(34.0898146793625,-1.8231619033622,-2.65749157164531));
#74270=CARTESIAN_POINT('Ctrl Pts',(34.0911020894005,-1.80592184261346,-2.66925660304347));
#74271=CARTESIAN_POINT('Ctrl Pts',(34.0919015128902,-1.79520559901843,-2.6764755489184));
#74272=CARTESIAN_POINT('Ctrl Pts',(34.0954843561959,-1.74713238270632,-2.70844123829686));
#74273=CARTESIAN_POINT('Ctrl Pts',(34.0982945017097,-1.70930660578123,-2.73247069606748));
#74274=CARTESIAN_POINT('Ctrl Pts',(34.1058237651811,-1.60769913970024,-2.79408308342598));
#74275=CARTESIAN_POINT('Ctrl Pts',(34.1105911047565,-1.5431055586311,-2.83026865217769));
#74276=CARTESIAN_POINT('Ctrl Pts',(34.1350940527639,-1.20977322716755,-3.00219855800697));
#74277=CARTESIAN_POINT('Ctrl Pts',(34.1559505400123,-0.924254100659246,
-3.10200905282167));
#74278=CARTESIAN_POINT('Ctrl Pts',(34.1772913978078,-0.606969066619641,
-3.1651561847723));
#74279=CARTESIAN_POINT('Ctrl Pts',(34.1787703826077,-0.584827328114436,
-3.1693220354944));
#74280=CARTESIAN_POINT('Ctrl Pts',(34.1838265784864,-0.508544881713805,
-3.18284751520198));
#74281=CARTESIAN_POINT('Ctrl Pts',(34.1873607449368,-0.45420606974951,-3.19105529844832));
#74282=CARTESIAN_POINT('Ctrl Pts',(34.1913822789209,-0.390861605494726,
-3.19897229603057));
#74283=CARTESIAN_POINT('Ctrl Pts',(34.1919402298768,-0.382038338056251,
-3.20003800884452));
#74284=CARTESIAN_POINT('Ctrl Pts',(34.1928271238649,-0.36795562183618,-3.20167990492449));
#74285=CARTESIAN_POINT('Ctrl Pts',(34.1931573605453,-0.362699044396027,
-3.20227965009078));
#74286=CARTESIAN_POINT('Ctrl Pts',(34.1937394973898,-0.353409609686988,
-3.20331635411682));
#74287=CARTESIAN_POINT('Ctrl Pts',(34.193991697711,-0.34937737694337,-3.20375864664951));
#74288=CARTESIAN_POINT('Ctrl Pts',(34.194520621874,-0.340904351111182,-3.20467185959086));
#74289=CARTESIAN_POINT('Ctrl Pts',(34.1947972531571,-0.33646342250337,-3.2051411622821));
#74290=CARTESIAN_POINT('Ctrl Pts',(34.1955294039,-0.324685144208438,-3.20636110242637));
#74291=CARTESIAN_POINT('Ctrl Pts',(34.1959840285445,-0.317346115838568,
-3.20709579016687));
#74292=CARTESIAN_POINT('Ctrl Pts',(34.1980705665225,-0.283550136825774,
-3.21036185720309));
#74293=CARTESIAN_POINT('Ctrl Pts',(34.199686075999,-0.257064107710861,-3.21259117942451));
#74294=CARTESIAN_POINT('Ctrl Pts',(34.21409152433,-0.0183803925095439,-3.2297102528033));
#74295=CARTESIAN_POINT('Ctrl Pts',(34.2258931363999,0.194808855475423,-3.22388609181496));
#74296=CARTESIAN_POINT('Ctrl Pts',(34.2518266971885,0.655173114240783,-3.16543964946339));
#74297=CARTESIAN_POINT('Ctrl Pts',(34.2659535153078,0.899856969521382,-3.10475341768069));
#74298=CARTESIAN_POINT('Ctrl Pts',(34.2822982124249,1.15309804491474,-3.00946117669203));
#74299=CARTESIAN_POINT('Ctrl Pts',(34.2834719114789,1.17113881898752,-3.00248655560916));
#74300=CARTESIAN_POINT('Ctrl Pts',(34.2852188387614,1.19777140328748,-2.99191376251029));
#74301=CARTESIAN_POINT('Ctrl Pts',(34.2857878707302,1.20641237946928,-2.98843997172863));
#74302=CARTESIAN_POINT('Ctrl Pts',(34.2868011038135,1.22173745400303,-2.98220178289296));
#74303=CARTESIAN_POINT('Ctrl Pts',(34.2872447992585,1.22842755825503,-2.97945223374505));
#74304=CARTESIAN_POINT('Ctrl Pts',(34.2881783850816,1.24246039339101,-2.97362961591066));
#74305=CARTESIAN_POINT('Ctrl Pts',(34.2886684338232,1.24980109980339,-2.97055182262154));
#74306=CARTESIAN_POINT('Ctrl Pts',(34.2899588616555,1.26906423405284,-2.9623911814377));
#74307=CARTESIAN_POINT('Ctrl Pts',(34.2907607634599,1.2809674422033,-2.95726359091311));
#74308=CARTESIAN_POINT('Ctrl Pts',(34.294370348991,1.33424200458382,-2.93393230933178));
#74309=CARTESIAN_POINT('Ctrl Pts',(34.2972052509489,1.37525690619207,-2.91493201110783));
#74310=CARTESIAN_POINT('Ctrl Pts',(34.3048161715812,1.48313836262008,-2.86217183828571));
#74311=CARTESIAN_POINT('Ctrl Pts',(34.30964170965,1.54924744292296,-2.82693437403859));
#74312=CARTESIAN_POINT('Ctrl Pts',(34.3345583713122,1.87919669710098,-2.63601368599455));
#74313=CARTESIAN_POINT('Ctrl Pts',(34.3558101807841,2.12105464443564,-2.4456150849873));
#74314=CARTESIAN_POINT('Ctrl Pts',(34.3805446715954,2.38055917866903,-2.17345975217112));
#74315=CARTESIAN_POINT('Ctrl Pts',(34.3850620962195,2.4270762221431,-2.12138916657322));
#74316=CARTESIAN_POINT('Ctrl Pts',(34.3901286790484,2.47863766626281,-2.05975342278005));
#74317=CARTESIAN_POINT('Ctrl Pts',(34.3907911039627,2.48536664892809,-2.05162897985243));
#74318=CARTESIAN_POINT('Ctrl Pts',(34.3917722350599,2.49531654551626,-2.03949487538844));
#74319=CARTESIAN_POINT('Ctrl Pts',(34.3920931003489,2.4985678677454,-2.03551040778731));
#74320=CARTESIAN_POINT('Ctrl Pts',(34.392663993498,2.50434824582372,-2.02839188620047));
#74321=CARTESIAN_POINT('Ctrl Pts',(34.3929142863809,2.50688097057737,-2.02526086723646));
#74322=CARTESIAN_POINT('Ctrl Pts',(34.393449541339,2.512294015095,-2.0185434110434));
#74323=CARTESIAN_POINT('Ctrl Pts',(34.3937343722852,2.51517251721996,-2.01495556521726));
#74324=CARTESIAN_POINT('Ctrl Pts',(34.3945116892489,2.52302221940756,-2.00512844564018));
#74325=CARTESIAN_POINT('Ctrl Pts',(34.3950030746773,2.52797799056766,-1.9988768059891));
#74326=CARTESIAN_POINT('Ctrl Pts',(34.3975492816733,2.55361970908719,-1.96628222627942));
#74327=CARTESIAN_POINT('Ctrl Pts',(34.399577594593,2.57391818456463,-1.93963522352443));
#74328=CARTESIAN_POINT('Ctrl Pts',(34.4053830945387,2.63148526249179,-1.86156792582208));
#74329=CARTESIAN_POINT('Ctrl Pts',(34.4090982417231,2.66765582003833,-1.80935438767603));
#74330=CARTESIAN_POINT('Ctrl Pts',(34.4330602878244,2.89416807216864,-1.46080108700049));
#74331=CARTESIAN_POINT('Ctrl Pts',(34.4518113554724,3.03637594754524,-1.13604757613463));
#74332=CARTESIAN_POINT('Ctrl Pts',(34.4738388306347,3.12800406265096,-0.775939869479387));
#74333=CARTESIAN_POINT('Ctrl Pts',(34.4749910462281,3.13260716192307,-0.757142286912593));
#74334=CARTESIAN_POINT('Ctrl Pts',(34.4765962884021,3.13875594932679,-0.731016222123901));
#74335=CARTESIAN_POINT('Ctrl Pts',(34.4770448809079,3.14044587520714,-0.723721859513328));
#74336=CARTESIAN_POINT('Ctrl Pts',(34.4791967128837,3.14841617263775,-0.688765417767764));
#74337=CARTESIAN_POINT('Ctrl Pts',(34.480910366545,3.15435641672236,-0.661027771455983));
#74338=CARTESIAN_POINT('Ctrl Pts',(34.4833178010663,3.16213275926679,-0.622221589080528));
#74339=CARTESIAN_POINT('Ctrl Pts',(34.4840016766316,3.16427850150988,-0.611215880881014));
#74340=CARTESIAN_POINT('Ctrl Pts',(34.4851044326133,3.1676368019304,-0.593499081402116));
#74341=CARTESIAN_POINT('Ctrl Pts',(34.4855221539621,3.168885582184,-0.586794882785151));
#74342=CARTESIAN_POINT('Ctrl Pts',(34.4863886381031,3.17142762870947,-0.572902867409919));
#74343=CARTESIAN_POINT('Ctrl Pts',(34.4868374982169,3.17271775873012,-0.565714523118713));
#74344=CARTESIAN_POINT('Ctrl Pts',(34.4878898824897,3.17568006867618,-0.548880227709062));
#74345=CARTESIAN_POINT('Ctrl Pts',(34.4884940239807,3.17733274505393,-0.539230958658211));
#74346=CARTESIAN_POINT('Ctrl Pts',(34.4904520581129,3.18253436628835,-0.508006546438726));
#74347=CARTESIAN_POINT('Ctrl Pts',(34.491811513763,3.18590765657875,-0.486403134856993));
#74348=CARTESIAN_POINT('Ctrl Pts',(34.4950023192994,3.19327052644359,-0.435881874109262));
#74349=CARTESIAN_POINT('Ctrl Pts',(34.496839005377,3.1970874933311,-0.406941191132162));
#74350=CARTESIAN_POINT('Ctrl Pts',(34.5032898435442,3.20903120086238,-0.305801833587352));
#74351=CARTESIAN_POINT('Ctrl Pts',(34.5079661539453,3.21510884141991,-0.233387719814971));
#74352=CARTESIAN_POINT('Ctrl Pts',(34.5317643456143,3.23330240527779,0.130715023243514));
#74353=CARTESIAN_POINT('Ctrl Pts',(34.5519386052257,3.20819256489968,0.422837264813661));
#74354=CARTESIAN_POINT('Ctrl Pts',(34.5719223956567,3.14198504625179,0.717036866251241));
#74355=CARTESIAN_POINT('Ctrl Pts',(34.5725648380975,3.13980976651225,0.726502946845154));
#74356=CARTESIAN_POINT('Ctrl Pts',(34.5783167751819,3.11991039252752,0.811339330235586));
#74357=CARTESIAN_POINT('Ctrl Pts',(34.5833430977989,3.09951658942662,0.88606518541743));
#74358=CARTESIAN_POINT('Ctrl Pts',(34.5889104651749,3.07322226182184,0.970329741651132));
#74359=CARTESIAN_POINT('Ctrl Pts',(34.5895907786374,3.06994370432798,0.980653118201075));
#74360=CARTESIAN_POINT('Ctrl Pts',(34.5905931741331,3.06501467198019,0.995906444367906));
#74361=CARTESIAN_POINT('Ctrl Pts',(34.5909175521902,3.06340425631236,1.00084911385299));
#74362=CARTESIAN_POINT('Ctrl Pts',(34.5914923265982,3.06052323347696,1.00961941566585));
#74363=CARTESIAN_POINT('Ctrl Pts',(34.5917430020978,3.05925739641625,1.01344857308127));
#74364=CARTESIAN_POINT('Ctrl Pts',(34.5922764972188,3.0565434218592,1.02160692593387));
#74365=CARTESIAN_POINT('Ctrl Pts',(34.5925591954394,3.05509327814732,1.02593540891315));
#74366=CARTESIAN_POINT('Ctrl Pts',(34.5933247326321,3.05113387133929,1.03767086332361));
#74367=CARTESIAN_POINT('Ctrl Pts',(34.5938065264061,3.04860681656638,1.04507186470845));
#74368=CARTESIAN_POINT('Ctrl Pts',(34.5962230110933,3.0357563017489,1.08226397634098));
#74369=CARTESIAN_POINT('Ctrl Pts',(34.5981343063317,3.02502256985817,1.11191288583828));
#74370=CARTESIAN_POINT('Ctrl Pts',(34.6035158791671,2.99322841875114,1.19586495752777));
#74371=CARTESIAN_POINT('Ctrl Pts',(34.6069344403413,2.97112800012848,1.24976341932747));
#74372=CARTESIAN_POINT('Ctrl Pts',(34.6267367759753,2.83274271150433,1.5628025391476));
#74373=CARTESIAN_POINT('Ctrl Pts',(34.6420328778033,2.6840707846814,1.80625876471057));
#74374=CARTESIAN_POINT('Ctrl Pts',(34.6592125547122,2.49606351048983,2.03862817651479));
#74375=CARTESIAN_POINT('Ctrl Pts',(34.6600679475698,2.48664755277495,2.05010288296596));
#74376=CARTESIAN_POINT('Ctrl Pts',(34.6669095603765,2.41092169336804,2.14109654099073));
#74377=CARTESIAN_POINT('Ctrl Pts',(34.6730105519655,2.34089994481689,2.21743589382977));
#74378=CARTESIAN_POINT('Ctrl Pts',(34.680239664614,2.25595243793691,2.30153264586878));
#74379=CARTESIAN_POINT('Ctrl Pts',(34.6812116344691,2.24449032281051,2.31271206567245));
#74380=CARTESIAN_POINT('Ctrl Pts',(34.682767615086,2.22607946068685,2.3304030700112));
#74381=CARTESIAN_POINT('Ctrl Pts',(34.683349207277,2.21918423713549,2.33697016510572));
#74382=CARTESIAN_POINT('Ctrl Pts',(34.6843782107073,2.20696122235134,2.34850863830448));
#74383=CARTESIAN_POINT('Ctrl Pts',(34.6848250702172,2.20164546124089,2.35349270718351));
#74384=CARTESIAN_POINT('Ctrl Pts',(34.6857512738721,2.19061182638981,2.36376777139543));
#74385=CARTESIAN_POINT('Ctrl Pts',(34.6862307259954,2.1848915848346,2.36905614366219));
#74386=CARTESIAN_POINT('Ctrl Pts',(34.6874631207535,2.17016643487082,2.38257087380289));
#74387=CARTESIAN_POINT('Ctrl Pts',(34.6882173449824,2.16113396010438,2.39076689027765));
#74388=CARTESIAN_POINT('Ctrl Pts',(34.6913454025323,2.12358988007634,2.42444755781927));
#74389=CARTESIAN_POINT('Ctrl Pts',(34.6937383177986,2.09467326617776,2.44947415665856));
#74390=CARTESIAN_POINT('Ctrl Pts',(34.7034148302954,1.97701218882663,2.54769957885559));
#74391=CARTESIAN_POINT('Ctrl Pts',(34.7108594538666,1.88491167208578,2.61656343737978));
#74392=CARTESIAN_POINT('Ctrl Pts',(34.7184445309107,1.78943583648355,2.68030538364725));
#74393=CARTESIAN_POINT('Origin',(-1.72497344927317,0.,0.));
#74394=CARTESIAN_POINT('',(36.2170783832723,1.78943621037801,2.68030513402635));
#74395=CARTESIAN_POINT('',(35.9732071344081,1.7894362098569,2.68030513437425));
#74396=CARTESIAN_POINT('',(-1.72497344927317,1.78943621037804,2.68030513402633));
#74397=CARTESIAN_POINT('',(35.3965734493253,-3.22274924894224,0.0022002141326696));
#74398=CARTESIAN_POINT('Ctrl Pts',(35.3965734493253,-3.22274924894224,0.00220021413262451));
#74399=CARTESIAN_POINT('Ctrl Pts',(35.4026541762509,-3.22281622665231,-0.0959049482773073));
#74400=CARTESIAN_POINT('Ctrl Pts',(35.4087349031765,-3.21839931530627,-0.194185885337791));
#74401=CARTESIAN_POINT('Ctrl Pts',(35.4148156301021,-3.20947683880307,-0.292191689968481));
#74402=CARTESIAN_POINT('Ctrl Pts',(35.4208892708103,-3.20056476016993,-0.390083282853154));
#74403=CARTESIAN_POINT('Ctrl Pts',(35.4269629115185,-3.18715758731565,-0.487699937740014));
#74404=CARTESIAN_POINT('Ctrl Pts',(35.4330365522267,-3.16928567806029,-0.584590329497458));
#74405=CARTESIAN_POINT('Ctrl Pts',(35.4391050586173,-3.15142887672161,-0.681398815514107));
#74406=CARTESIAN_POINT('Ctrl Pts',(35.4451735650079,-3.12911491984515,-0.777481819955843));
#74407=CARTESIAN_POINT('Ctrl Pts',(35.4512420713985,-3.10242590709074,-0.872393863752045));
#74408=CARTESIAN_POINT('Ctrl Pts',(35.4573079117998,-3.07574861923517,-0.967264211209651));
#74409=CARTESIAN_POINT('Ctrl Pts',(35.4633737522011,-3.04470021267832,-1.06096418915499));
#74410=CARTESIAN_POINT('Ctrl Pts',(35.4694395926024,-3.00941350713223,-1.15306023502247));
#74411=CARTESIAN_POINT('Ctrl Pts',(35.4755044967244,-2.97413224818665,-1.24514206561079));
#74412=CARTESIAN_POINT('Ctrl Pts',(35.4815694008465,-2.93461415028325,-1.33562003807765));
#74413=CARTESIAN_POINT('Ctrl Pts',(35.4876343049685,-2.89104095423344,-1.42407856645798));
#74414=CARTESIAN_POINT('Ctrl Pts',(35.493700001277,-2.84746206673425,-1.51254864912586));
#74415=CARTESIAN_POINT('Ctrl Pts',(35.4997656975855,-2.79982722847961,-1.59899836299989));
#74416=CARTESIAN_POINT('Ctrl Pts',(35.505831393894,-2.74836456137673,-1.68303588799185));
#74417=CARTESIAN_POINT('Ctrl Pts',(35.5119033144651,-2.69684908629595,-1.76715964737491));
#74418=CARTESIAN_POINT('Ctrl Pts',(35.5179752350362,-2.64149817683487,-1.84886589519704));
#74419=CARTESIAN_POINT('Ctrl Pts',(35.5240471556074,-2.58258360470976,-1.92779134949411));
#74420=CARTESIAN_POINT('Ctrl Pts',(35.5301225189983,-2.52363562762575,-2.00676155505496));
#74421=CARTESIAN_POINT('Ctrl Pts',(35.5361978823893,-2.46112025182293,-2.08294748478473));
#74422=CARTESIAN_POINT('Ctrl Pts',(35.5422732457803,-2.39534846607981,-2.15602024307499));
#74423=CARTESIAN_POINT('Ctrl Pts',(35.5483582611303,-2.32947218838389,-2.22920909240829));
#74424=CARTESIAN_POINT('Ctrl Pts',(35.5544432764804,-2.26032948940595,-2.29927458140149));
#74425=CARTESIAN_POINT('Ctrl Pts',(35.5605282918304,-2.18826682920184,-2.3659260019525));
#74426=CARTESIAN_POINT('Ctrl Pts',(35.5638661635418,-2.14873760846764,-2.40248694360725));
#74427=CARTESIAN_POINT('Ctrl Pts',(35.5672040352532,-2.10833035019661,-2.4380213303225));
#74428=CARTESIAN_POINT('Ctrl Pts',(35.5705419069646,-2.06710597654784,-2.4724866924253));
#74429=CARTESIAN_POINT('Ctrl Pts',(35.5767141550573,-1.99087564667602,-2.53621855029738));
#74430=CARTESIAN_POINT('Ctrl Pts',(35.5828864031501,-1.91156096397265,-2.59653384352848));
#74431=CARTESIAN_POINT('Ctrl Pts',(35.5890586512429,-1.8295011211476,-2.65311952429959));
#74432=CARTESIAN_POINT('Ctrl Pts',(35.5952225398955,-1.7475524168143,-2.70962856774117));
#74433=CARTESIAN_POINT('Ctrl Pts',(35.6013864285481,-1.66286629660897,-2.7624177941908));
#74434=CARTESIAN_POINT('Ctrl Pts',(35.6075503172008,-1.57581578216981,-2.81121364950524));
#74435=CARTESIAN_POINT('Ctrl Pts',(35.6137076788593,-1.48885744626015,-2.85995783447381));
#74436=CARTESIAN_POINT('Ctrl Pts',(35.6198650405179,-1.39954007048067,-2.90471684396876));
#74437=CARTESIAN_POINT('Ctrl Pts',(35.6260224021764,-1.30826567747346,-2.94526034157337));
#74438=CARTESIAN_POINT('Ctrl Pts',(35.6321752663227,-1.21705795388129,-2.98577422505315));
#74439=CARTESIAN_POINT('Ctrl Pts',(35.6383281304691,-1.1238964508519,-3.02207854267777));
#74440=CARTESIAN_POINT('Ctrl Pts',(35.6444809946154,-1.02920699676254,-3.05398927966603));
#74441=CARTESIAN_POINT('Ctrl Pts',(35.6506315277519,-0.934553415729537,
-3.08588792728618));
#74442=CARTESIAN_POINT('Ctrl Pts',(35.6567820608884,-0.838373445007394,
-3.11339616306775));
#74443=CARTESIAN_POINT('Ctrl Pts',(35.662932594025,-0.741111225582647,-3.13637875802898));
#74444=CARTESIAN_POINT('Ctrl Pts',(35.6690824422402,-0.643859837246461,
-3.15935879365603));
#74445=CARTESIAN_POINT('Ctrl Pts',(35.6752322904554,-0.545526862551012,
-3.17781409054637));
#74446=CARTESIAN_POINT('Ctrl Pts',(35.6813821386706,-0.446568896009425,
-3.19166003572074));
#74447=CARTESIAN_POINT('Ctrl Pts',(35.6875329470498,-0.347595479351526,
-3.20550814263581));
#74448=CARTESIAN_POINT('Ctrl Pts',(35.6936837554289,-0.247997307256176,
-3.2147454082297));
#74449=CARTESIAN_POINT('Ctrl Pts',(35.699834563808,-0.148237390124708,-3.21933894435939));
#74450=CARTESIAN_POINT('Ctrl Pts',(35.7059919501742,-0.0483707846683332,
-3.22393739305004));
#74451=CARTESIAN_POINT('Ctrl Pts',(35.7121493365404,0.0516574764825923,
-3.22388217518866));
#74452=CARTESIAN_POINT('Ctrl Pts',(35.7183067229066,0.151383196910882,-3.21919255251888));
#74453=CARTESIAN_POINT('Ctrl Pts',(35.7244675456436,0.251164573185612,-3.21450031262139));
#74454=CARTESIAN_POINT('Ctrl Pts',(35.7306283683805,0.350642639995108,-3.2051685576842));
#74455=CARTESIAN_POINT('Ctrl Pts',(35.7367891911175,0.44935923717731,-3.19126837455947));
#74456=CARTESIAN_POINT('Ctrl Pts',(35.7429603140342,0.548240877039232,-3.17734495194374));
#74457=CARTESIAN_POINT('Ctrl Pts',(35.7491314369508,0.646358077271314,-3.15883792525885));
#74458=CARTESIAN_POINT('Ctrl Pts',(35.7553025598675,0.743263625943796,-3.13586937624144));
#74459=CARTESIAN_POINT('Ctrl Pts',(35.7599980818131,0.816997715603227,-3.11839292545202));
#74460=CARTESIAN_POINT('Ctrl Pts',(35.7646936037587,0.890030550168058,-3.09833454312605));
#74461=CARTESIAN_POINT('Ctrl Pts',(35.7693891257042,0.962172478710912,-3.07576684482282));
#74462=CARTESIAN_POINT('Ctrl Pts',(35.775561373797,1.05700280556683,-3.04610167992207));
#74463=CARTESIAN_POINT('Ctrl Pts',(35.7817336218897,1.15062682894838,-3.0119945584408));
#74464=CARTESIAN_POINT('Ctrl Pts',(35.7879058699825,1.24259780526836,-2.97356154414908));
#74465=CARTESIAN_POINT('Ctrl Pts',(35.7940697586351,1.33444421986316,-2.93518058195853));
#74466=CARTESIAN_POINT('Ctrl Pts',(35.8002336472878,1.42464164003634,-2.89248553799921));
#74467=CARTESIAN_POINT('Ctrl Pts',(35.8063975359404,1.51275825298489,-2.84564228787213));
#74468=CARTESIAN_POINT('Ctrl Pts',(35.812554897599,1.60078155850296,-2.79884864046079));
#74469=CARTESIAN_POINT('Ctrl Pts',(35.8187122592575,1.68672805590052,-2.74791572249858));
#74470=CARTESIAN_POINT('Ctrl Pts',(35.824869620916,1.77018660637164,-2.69305717375671));
#74471=CARTESIAN_POINT('Ctrl Pts',(35.8310224850623,1.85358419634174,-2.63823869526046));
#74472=CARTESIAN_POINT('Ctrl Pts',(35.8371753492086,1.93449709053669,-2.57950052472488));
#74473=CARTESIAN_POINT('Ctrl Pts',(35.843328213355,2.0125402443185,-2.51710137410046));
#74474=CARTESIAN_POINT('Ctrl Pts',(35.8494787464915,2.09055383148716,-2.45472586336575));
#74475=CARTESIAN_POINT('Ctrl Pts',(35.855629279628,2.16569949961442,-2.38869239938264));
#74476=CARTESIAN_POINT('Ctrl Pts',(35.8617798127646,2.2376233412963,-2.31930147781309));
#74477=CARTESIAN_POINT('Ctrl Pts',(35.8679296609798,2.30953917356318,-2.2499182835934));
#74478=CARTESIAN_POINT('Ctrl Pts',(35.874079509195,2.37823358008963,-2.17717867672222));
#74479=CARTESIAN_POINT('Ctrl Pts',(35.8802293574102,2.44338849835483,-2.10142099746989));
#74480=CARTESIAN_POINT('Ctrl Pts',(35.8863801657894,2.5085535891317,-2.02565149031726));
#74481=CARTESIAN_POINT('Ctrl Pts',(35.8925309741685,2.57017781074956,-1.9468633042078));
#74482=CARTESIAN_POINT('Ctrl Pts',(35.8986817825477,2.62798314294445,-1.86542814466273));
#74483=CARTESIAN_POINT('Ctrl Pts',(35.9048391689139,2.68585029509895,-1.78390589421993));
#74484=CARTESIAN_POINT('Ctrl Pts',(35.9109965552801,2.73989015035574,-1.69973137241133));
#74485=CARTESIAN_POINT('Ctrl Pts',(35.9171539416463,2.7898679161095,-1.61330548042299));
#74486=CARTESIAN_POINT('Ctrl Pts',(35.9233147643832,2.83987357391408,-1.52683135507855));
#74487=CARTESIAN_POINT('Ctrl Pts',(35.9294755871202,2.8858124277765,-1.4381037430731));
#74488=CARTESIAN_POINT('Ctrl Pts',(35.9356364098571,2.92749654469965,-1.3475464902079));
#74489=CARTESIAN_POINT('Ctrl Pts',(35.9418075327738,2.96925035262258,-1.2568378361387));
#74490=CARTESIAN_POINT('Ctrl Pts',(35.9479786556905,3.00673505160855,-1.1642938338478));
#74491=CARTESIAN_POINT('Ctrl Pts',(35.9541497786072,3.03981152583318,-1.07035669284203));
#74492=CARTESIAN_POINT('Ctrl Pts',(35.9588453005528,3.06497895689897,-0.998881223457837));
#74493=CARTESIAN_POINT('Ctrl Pts',(35.9635408224984,3.08759526833057,-0.926599579291563));
#74494=CARTESIAN_POINT('Ctrl Pts',(35.968236344444,3.10761899878544,-0.853710560370323));
#74495=CARTESIAN_POINT('Ctrl Pts',(35.9744085925367,3.1339401263496,-0.75789818567932));
#74496=CARTESIAN_POINT('Ctrl Pts',(35.9805808406295,3.15587237980187,-0.660698752818934));
#74497=CARTESIAN_POINT('Ctrl Pts',(35.9867530887222,3.17327183418831,-0.562550823345912));
#74498=CARTESIAN_POINT('Ctrl Pts',(35.9929169773749,3.19064772346603,-0.464535821410606));
#74499=CARTESIAN_POINT('Ctrl Pts',(35.9990808660275,3.2035029405354,-0.365575300096989));
#74500=CARTESIAN_POINT('Ctrl Pts',(36.0052447546801,3.21174353582663,-0.266122194820102));
#74501=CARTESIAN_POINT('Ctrl Pts',(36.0114021163387,3.21997540508147,-0.166774401281577));
#74502=CARTESIAN_POINT('Ctrl Pts',(36.0175594779972,3.22360233163526,-0.0669354912772715));
#74503=CARTESIAN_POINT('Ctrl Pts',(36.0237168396557,3.22258172420588,0.0329331643525058));
#74504=CARTESIAN_POINT('Ctrl Pts',(36.029869703802,3.22156186225722,0.132728873073168));
#74505=CARTESIAN_POINT('Ctrl Pts',(36.0360225679483,3.21590121997748,0.232553851179046));
#74506=CARTESIAN_POINT('Ctrl Pts',(36.0421754320946,3.2056092305873,0.331944307487699));
#74507=CARTESIAN_POINT('Ctrl Pts',(36.0483259652312,3.19532114031261,0.431297109767358));
#74508=CARTESIAN_POINT('Ctrl Pts',(36.0544764983677,3.18040523396699,0.530215285760309));
#74509=CARTESIAN_POINT('Ctrl Pts',(36.0606270315042,3.16092292982288,0.628238644322294));
#74510=CARTESIAN_POINT('Ctrl Pts',(36.0667768797195,3.14144279522168,0.726251087035697));
#74511=CARTESIAN_POINT('Ctrl Pts',(36.0729267279347,3.11739735849586,0.823368484387686));
#74512=CARTESIAN_POINT('Ctrl Pts',(36.0790765761499,3.08889925483512,0.91914033530199));
#74513=CARTESIAN_POINT('Ctrl Pts',(36.085227384529,3.06039670182045,1.01492713889055));
#74514=CARTESIAN_POINT('Ctrl Pts',(36.0913781929082,3.02744022494843,1.1093675623996));
#74515=CARTESIAN_POINT('Ctrl Pts',(36.0975290012873,2.99019217781354,1.20202674772349));
#74516=CARTESIAN_POINT('Ctrl Pts',(36.1036863876535,2.95290429572424,1.29478502748874));
#74517=CARTESIAN_POINT('Ctrl Pts',(36.1098437740197,2.91131584069827,1.38575786127123));
#74518=CARTESIAN_POINT('Ctrl Pts',(36.1160011603858,2.86563709962124,1.47453096806218));
#74519=CARTESIAN_POINT('Ctrl Pts',(36.1221619831228,2.81993286573246,1.56335361816466));
#74520=CARTESIAN_POINT('Ctrl Pts',(36.1283228058598,2.77013401624417,1.64997371985045));
#74521=CARTESIAN_POINT('Ctrl Pts',(36.1344836285967,2.71649547672681,1.73400400444255));
#74522=CARTESIAN_POINT('Ctrl Pts',(36.1406547515134,2.66276725980429,1.81817477790597));
#74523=CARTESIAN_POINT('Ctrl Pts',(36.1468258744301,2.60518678068265,1.8997467304522));
#74524=CARTESIAN_POINT('Ctrl Pts',(36.1529969973468,2.54405080859028,1.97836372940144));
#74525=CARTESIAN_POINT('Ctrl Pts',(36.1576925192924,2.49753329427433,2.0381823149074));
#74526=CARTESIAN_POINT('Ctrl Pts',(36.1623880412379,2.44895820203773,2.09629078279533));
#74527=CARTESIAN_POINT('Ctrl Pts',(36.1670835631835,2.39847034566298,2.15254676220409));
#74528=CARTESIAN_POINT('Ctrl Pts',(36.173255787853,2.33210447702427,2.22649478075079));
#74529=CARTESIAN_POINT('Ctrl Pts',(36.1794280125225,2.26219872041211,2.29750085817463));
#74530=CARTESIAN_POINT('Ctrl Pts',(36.1856002371921,2.18904417262736,2.36520679281668));
#74531=CARTESIAN_POINT('Ctrl Pts',(36.191763242266,2.11599889749356,2.43281159352808));
#74532=CARTESIAN_POINT('Ctrl Pts',(36.1979262473398,2.03971479775672,2.49712576225517));
#74533=CARTESIAN_POINT('Ctrl Pts',(36.2040892524137,1.9605219423884,2.55782549754936));
#74534=CARTESIAN_POINT('Ctrl Pts',(36.2084189626999,1.90488640154891,2.60046902373868));
#74535=CARTESIAN_POINT('Ctrl Pts',(36.2127486729861,1.8478160898422,2.64132932155466));
#74536=CARTESIAN_POINT('Ctrl Pts',(36.2170783832723,1.78943621037801,2.68030513402635));
#74537=CARTESIAN_POINT('Ctrl Pts',(34.9669226703048,1.78943621037804,2.68030513402632));
#74538=CARTESIAN_POINT('Ctrl Pts',(34.9692818637851,1.75780908412248,2.70142016463737));
#74539=CARTESIAN_POINT('Ctrl Pts',(34.9716410572654,1.72582786777747,2.72196218169318));
#74540=CARTESIAN_POINT('Ctrl Pts',(34.9740002507457,1.69351550403383,2.74191954661275));
#74541=CARTESIAN_POINT('Ctrl Pts',(34.9801724988385,1.60897817076503,2.79413307152716));
#74542=CARTESIAN_POINT('Ctrl Pts',(34.9863447469312,1.52187505275975,2.84252522299456));
#74543=CARTESIAN_POINT('Ctrl Pts',(34.992516995024,1.43258650633541,2.88683450588455));
#74544=CARTESIAN_POINT('Ctrl Pts',(34.9986808836766,1.34341888866301,2.93108377809575));
#74545=CARTESIAN_POINT('Ctrl Pts',(35.0048447723292,1.25207211128199,2.97126098116774));
#74546=CARTESIAN_POINT('Ctrl Pts',(35.0110086609819,1.15895438370155,3.00714853291269));
#74547=CARTESIAN_POINT('Ctrl Pts',(35.0171660226404,1.06593525927433,3.04299808302407));
#74548=CARTESIAN_POINT('Ctrl Pts',(35.023323384299,0.971149315950608,3.07456685707849));
#74549=CARTESIAN_POINT('Ctrl Pts',(35.0294807459575,0.875027306918201,3.10168418357632));
#74550=CARTESIAN_POINT('Ctrl Pts',(35.0356336101038,0.778975508137488,3.12878170280693));
#74551=CARTESIAN_POINT('Ctrl Pts',(35.0417864742501,0.681590000702285,3.1514341213634));
#74552=CARTESIAN_POINT('Ctrl Pts',(35.0479393383964,0.583318496780982,3.16952001000359));
#74553=CARTESIAN_POINT('Ctrl Pts',(35.054089871533,0.485084222974071,3.18759904681313));
#74554=CARTESIAN_POINT('Ctrl Pts',(35.0602404046695,0.38596504636087,3.20111491272747));
#74555=CARTESIAN_POINT('Ctrl Pts',(35.066390937806,0.286419849779324,3.20999707665792));
#74556=CARTESIAN_POINT('Ctrl Pts',(35.0725407860212,0.186885738517858,3.21887825147354));
#74557=CARTESIAN_POINT('Ctrl Pts',(35.0786906342364,0.0869261342653877,
3.22312671159877));
#74558=CARTESIAN_POINT('Ctrl Pts',(35.0848404824516,-0.0129949696231923,
3.22272380033792));
#74559=CARTESIAN_POINT('Ctrl Pts',(35.0909912908308,-0.11293167400092,3.22232082617132));
#74560=CARTESIAN_POINT('Ctrl Pts',(35.0971420992099,-0.21282943166276,3.2172650399304));
#74561=CARTESIAN_POINT('Ctrl Pts',(35.1032929075891,-0.312225272783111,
3.20758989609575));
#74562=CARTESIAN_POINT('Ctrl Pts',(35.1094502939552,-0.41172741286698,3.19790440517061));
#74563=CARTESIAN_POINT('Ctrl Pts',(35.1156076803214,-0.510726131350203,
3.18358973379608));
#74564=CARTESIAN_POINT('Ctrl Pts',(35.1217650666876,-0.608764718986963,
3.16473112276805));
#74565=CARTESIAN_POINT('Ctrl Pts',(35.1279258894246,-0.706858020899713,
3.14586198695307));
#74566=CARTESIAN_POINT('Ctrl Pts',(35.1340867121615,-0.803989702561212,
3.12244396304012));
#74567=CARTESIAN_POINT('Ctrl Pts',(35.1402475348985,-0.899716417509094,
3.09461272707339));
#74568=CARTESIAN_POINT('Ctrl Pts',(35.1464186578152,-0.995603176400935,
3.06673496051411));
#74569=CARTESIAN_POINT('Ctrl Pts',(35.1525897807319,-1.09007986543974,3.0344293844264));
#74570=CARTESIAN_POINT('Ctrl Pts',(35.1587609036486,-1.18272124439707,2.99788058810751));
#74571=CARTESIAN_POINT('Ctrl Pts',(35.1634564255942,-1.25321078638775,2.97007111525829));
#74572=CARTESIAN_POINT('Ctrl Pts',(35.1681519475398,-1.32263815591294,2.93980605310689));
#74573=CARTESIAN_POINT('Ctrl Pts',(35.1728474694854,-1.39082599117186,2.9071843121448));
#74574=CARTESIAN_POINT('Ctrl Pts',(35.1790197175782,-1.48045867546171,2.86430314136796));
#74575=CARTESIAN_POINT('Ctrl Pts',(35.1851919656709,-1.56826413242229,2.81719735384842));
#74576=CARTESIAN_POINT('Ctrl Pts',(35.1913642137637,-1.65381672746355,2.76604551561643));
#74577=CARTESIAN_POINT('Ctrl Pts',(35.1975281024163,-1.7392534535725,2.71496295534004));
#74578=CARTESIAN_POINT('Ctrl Pts',(35.203691991069,-1.82244301278988,2.65984545701312));
#74579=CARTESIAN_POINT('Ctrl Pts',(35.2098558797216,-1.90298164997837,2.60091876119682));
#74580=CARTESIAN_POINT('Ctrl Pts',(35.2160132413801,-1.98343500411945,2.54205446335953));
#74581=CARTESIAN_POINT('Ctrl Pts',(35.2221706030387,-2.06124266835014,2.4793892422711));
#74582=CARTESIAN_POINT('Ctrl Pts',(35.2283279646973,-2.13602815962436,2.41319316752551));
#74583=CARTESIAN_POINT('Ctrl Pts',(35.2344808288436,-2.21075902544674,2.34704544427739));
#74584=CARTESIAN_POINT('Ctrl Pts',(35.2406336929899,-2.2824717828834,2.27737228197147));
#74585=CARTESIAN_POINT('Ctrl Pts',(35.2467865571362,-2.35082220201975,2.20448464204017));
#74586=CARTESIAN_POINT('Ctrl Pts',(35.2529370902727,-2.41914672663102,2.13162461555799));
#74587=CARTESIAN_POINT('Ctrl Pts',(35.2590876234092,-2.48411114721659,2.05555284772074));
#74588=CARTESIAN_POINT('Ctrl Pts',(35.2652381565458,-2.54540800974684,1.97661721798042));
#74589=CARTESIAN_POINT('Ctrl Pts',(35.271388004761,-2.60669804627883,1.89769037848562));
#74590=CARTESIAN_POINT('Ctrl Pts',(35.2775378529762,-2.66432107033355,1.81590065422547));
#74591=CARTESIAN_POINT('Ctrl Pts',(35.2836877011914,-2.71801050177438,1.73162827267985));
#74592=CARTESIAN_POINT('Ctrl Pts',(35.2898385095706,-2.7717083156425,1.64734273384997));
#74593=CARTESIAN_POINT('Ctrl Pts',(35.2959893179497,-2.82147108362984,1.56057413421501));
#74594=CARTESIAN_POINT('Ctrl Pts',(35.3021401263288,-2.86707661541854,1.47173001729943));
#74595=CARTESIAN_POINT('Ctrl Pts',(35.308297512695,-2.91273092008052,1.38279088597034));
#74596=CARTESIAN_POINT('Ctrl Pts',(35.3144548990612,-2.95421891166921,1.29177219211118));
#74597=CARTESIAN_POINT('Ctrl Pts',(35.3206122854274,-2.99136534813643,1.19910421418184));
#74598=CARTESIAN_POINT('Ctrl Pts',(35.3267731081644,-3.02853251562831,1.1063845192557));
#74599=CARTESIAN_POINT('Ctrl Pts',(35.3329339309013,-3.06135315998669,1.01201411748536));
#74600=CARTESIAN_POINT('Ctrl Pts',(35.3390947536383,-3.08970169113766,0.916439317293331));
#74601=CARTESIAN_POINT('Ctrl Pts',(35.345265876555,-3.11809761773861,0.820704727141216));
#74602=CARTESIAN_POINT('Ctrl Pts',(35.3514369994717,-3.14200639228661,0.723762138369761));
#74603=CARTESIAN_POINT('Ctrl Pts',(35.3576081223884,-3.16135336119834,0.626069076172855));
#74604=CARTESIAN_POINT('Ctrl Pts',(35.3623036443339,-3.17607420185096,0.551735778381997));
#74605=CARTESIAN_POINT('Ctrl Pts',(35.3669991662794,-3.18815505136534,0.47696822725851));
#74606=CARTESIAN_POINT('Ctrl Pts',(35.3716946882249,-3.1975832127869,0.401969103045743));
#74607=CARTESIAN_POINT('Ctrl Pts',(35.3799876085743,-3.21423460801356,0.269510609487901));
#74608=CARTESIAN_POINT('Ctrl Pts',(35.3882805289237,-3.2226579044307,0.135996438299877));
#74609=CARTESIAN_POINT('Ctrl Pts',(35.3965734492731,-3.22274924894167,0.00220021497454528));
#74610=CARTESIAN_POINT('',(35.1510759787713,-3.2227488984055,-0.00266464371426724));
#74611=CARTESIAN_POINT('Ctrl Pts',(34.7184445309107,1.78943583648354,2.68030538364725));
#74612=CARTESIAN_POINT('Ctrl Pts',(34.7284778164623,1.6631436028897,2.7646210926113));
#74613=CARTESIAN_POINT('Ctrl Pts',(34.7387622824405,1.53094595801515,2.83997492085281));
#74614=CARTESIAN_POINT('Ctrl Pts',(34.7619414468197,1.22213078041361,2.98810412560491));
#74615=CARTESIAN_POINT('Ctrl Pts',(34.7747870808691,1.04347616301321,3.05508516657453));
#74616=CARTESIAN_POINT('Ctrl Pts',(34.7875527957726,0.848617770828407,3.10903575152029));
#74617=CARTESIAN_POINT('Ctrl Pts',(34.7882908352342,0.837284743590831,3.11210695403658));
#74618=CARTESIAN_POINT('Ctrl Pts',(34.7893578671172,0.820797499870536,3.11647834515815));
#74619=CARTESIAN_POINT('Ctrl Pts',(34.789689639538,0.815656613366819,3.11782778576215));
#74620=CARTESIAN_POINT('Ctrl Pts',(34.790273542617,0.806582816664488,3.12018560447348));
#74621=CARTESIAN_POINT('Ctrl Pts',(34.7905259794676,0.802651311122227,3.12119927591796));
#74622=CARTESIAN_POINT('Ctrl Pts',(34.79101149322,0.795072951781387,3.12313796020713));
#74623=CARTESIAN_POINT('Ctrl Pts',(34.7912446315174,0.791426410539952,3.12406401249833));
#74624=CARTESIAN_POINT('Ctrl Pts',(34.7918800931694,0.781466912184462,3.12657470593548));
#74625=CARTESIAN_POINT('Ctrl Pts',(34.7922816817834,0.775150720267577,3.12814662208265));
#74626=CARTESIAN_POINT('Ctrl Pts',(34.7938430515433,0.750509310741564,3.13419993459638));
#74627=CARTESIAN_POINT('Ctrl Pts',(34.7949948929898,0.732149202625317,3.13853963496172));
#74628=CARTESIAN_POINT('Ctrl Pts',(34.8028754721779,0.605377675591414,3.16733107376819));
#74629=CARTESIAN_POINT('Ctrl Pts',(34.8093240711907,0.495790826396426,3.18632470560624));
#74630=CARTESIAN_POINT('Ctrl Pts',(34.8254589396022,0.214336675417558,3.22022907094288));
#74631=CARTESIAN_POINT('Ctrl Pts',(34.8349585888802,0.0418611685172514,
3.22708334719831));
#74632=CARTESIAN_POINT('Ctrl Pts',(34.8552830121383,-0.318953711024702,
3.21247873457031));
#74633=CARTESIAN_POINT('Ctrl Pts',(34.8661175392745,-0.506504546755326,
3.18828939790886));
#74634=CARTESIAN_POINT('Ctrl Pts',(34.8785953490578,-0.708348592382026,
3.14399124136648));
#74635=CARTESIAN_POINT('Ctrl Pts',(34.879681888505,-0.725818446321938,3.14000417468881));
#74636=CARTESIAN_POINT('Ctrl Pts',(34.8813310645041,-0.752169131473583,
3.13375862296668));
#74637=CARTESIAN_POINT('Ctrl Pts',(34.8818902445693,-0.761075264011493,
3.13160756627395));
#74638=CARTESIAN_POINT('Ctrl Pts',(34.8828643525772,-0.776539824538581,
3.12780261695751));
#74639=CARTESIAN_POINT('Ctrl Pts',(34.8832787207512,-0.783102474530881,
3.12616599415625));
#74640=CARTESIAN_POINT('Ctrl Pts',(34.8841442721017,-0.796777818220816,
3.12270981232525));
#74641=CARTESIAN_POINT('Ctrl Pts',(34.8845955719299,-0.803889536606635,
3.12088658478861));
#74642=CARTESIAN_POINT('Ctrl Pts',(34.8856644341053,-0.820688572717468,
3.11651859435406));
#74643=CARTESIAN_POINT('Ctrl Pts',(34.8862826708766,-0.830370337315541,
3.11395295109271));
#74644=CARTESIAN_POINT('Ctrl Pts',(34.8883334632527,-0.862369637508156,
3.10531337151894));
#74645=CARTESIAN_POINT('Ctrl Pts',(34.8897723436963,-0.884633342258211,
3.09904442237034));
#74646=CARTESIAN_POINT('Ctrl Pts',(34.8931786461193,-0.936889090710098,
3.08372142356578));
#74647=CARTESIAN_POINT('Ctrl Pts',(34.8951524302891,-0.966819975411211,
3.07446873626558));
#74648=CARTESIAN_POINT('Ctrl Pts',(34.9022306333465,-1.0728993418802,3.03997368300715));
#74649=CARTESIAN_POINT('Ctrl Pts',(34.9074112900613,-1.14822969579944,3.01232797092583));
#74650=CARTESIAN_POINT('Ctrl Pts',(34.9279205739658,-1.43770784080941,2.89365500312409));
#74651=CARTESIAN_POINT('Ctrl Pts',(34.9438283067615,-1.64276786542543,2.78236157455301));
#74652=CARTESIAN_POINT('Ctrl Pts',(34.9683962912241,-1.94333728080291,2.57434031387165));
#74653=CARTESIAN_POINT('Ctrl Pts',(34.9772017762032,-2.04787128812812,2.4919911341095));
#74654=CARTESIAN_POINT('Ctrl Pts',(34.9862787882194,-2.15506093622227,2.3962357750216));
#74655=CARTESIAN_POINT('Ctrl Pts',(34.9869561011829,-2.16305599863747,2.38902119764158));
#74656=CARTESIAN_POINT('Ctrl Pts',(34.9879623650819,-2.17493151774676,2.37819648916721));
#74657=CARTESIAN_POINT('Ctrl Pts',(34.9882935294953,-2.17883937728659,2.37461673053001));
#74658=CARTESIAN_POINT('Ctrl Pts',(34.9888618403155,-2.18554527553861,2.36844336354522));
#74659=CARTESIAN_POINT('Ctrl Pts',(34.9890993373077,-2.18834755619136,2.36585441044548));
#74660=CARTESIAN_POINT('Ctrl Pts',(34.9895916685124,-2.19415659740547,2.36046843914858));
#74661=CARTESIAN_POINT('Ctrl Pts',(34.9898464379053,-2.19716260816482,2.35767065121706));
#74662=CARTESIAN_POINT('Ctrl Pts',(34.9903536503233,-2.20314691579528,2.35207948481872));
#74663=CARTESIAN_POINT('Ctrl Pts',(34.9906060987866,-2.20612527484871,2.34928616979587));
#74664=CARTESIAN_POINT('Ctrl Pts',(34.9914615306586,-2.21621671301815,2.33978559402886));
#74665=CARTESIAN_POINT('Ctrl Pts',(34.9920624849962,-2.22330466482923,2.33305154640913));
#74666=CARTESIAN_POINT('Ctrl Pts',(34.9973176682873,-2.2852602306074,2.27365068924023));
#74667=CARTESIAN_POINT('Ctrl Pts',(35.0018309455731,-2.33828320461286,2.21908439305163));
#74668=CARTESIAN_POINT('Ctrl Pts',(35.0132013204803,-2.4694762310012,2.07414280623862));
#74669=CARTESIAN_POINT('Ctrl Pts',(35.0199206852879,-2.54464392427288,1.98120475746244));
#74670=CARTESIAN_POINT('Ctrl Pts',(35.0417498132851,-2.772675819174,1.66480899495109));
#74671=CARTESIAN_POINT('Ctrl Pts',(35.056732507421,-2.90258060168324,1.42629876383573));
#74672=CARTESIAN_POINT('Ctrl Pts',(35.0748970024127,-3.01318745895865,1.14363812459064));
#74673=CARTESIAN_POINT('Ctrl Pts',(35.0768870989167,-3.02474093199921,1.11272143610757));
#74674=CARTESIAN_POINT('Ctrl Pts',(35.0796184495736,-3.03982259703606,1.07039177998368));
#74675=CARTESIAN_POINT('Ctrl Pts',(35.0803458859634,-3.04376543881535,1.05912791086658));
#74676=CARTESIAN_POINT('Ctrl Pts',(35.0815008272551,-3.04990835125389,1.04126127572589));
#74677=CARTESIAN_POINT('Ctrl Pts',(35.0819269576981,-3.05214977867479,1.03467276116999));
#74678=CARTESIAN_POINT('Ctrl Pts',(35.0827976850688,-3.05667857196086,1.0212179240933));
#74679=CARTESIAN_POINT('Ctrl Pts',(35.0832423371441,-3.05896418299751,1.01435105685925));
#74680=CARTESIAN_POINT('Ctrl Pts',(35.0842629349958,-3.064148168375,0.998599470976569));
#74681=CARTESIAN_POINT('Ctrl Pts',(35.0848393881054,-3.0670310549673,0.989709758519929));
#74682=CARTESIAN_POINT('Ctrl Pts',(35.0866231039322,-3.07581218487464,0.962225295630317));
#74683=CARTESIAN_POINT('Ctrl Pts',(35.0878346349083,-3.08158020615633,0.943589700153594));
#74684=CARTESIAN_POINT('Ctrl Pts',(35.1038102468562,-3.15506376297686,0.698313372654338));
#74685=CARTESIAN_POINT('Ctrl Pts',(35.1194225230371,-3.19778273799733,0.464985913026927));
#74686=CARTESIAN_POINT('Ctrl Pts',(35.1406054601478,-3.22009290535345,0.151989361175707));
#74687=CARTESIAN_POINT('Ctrl Pts',(35.145849298648,-3.22281284297365,0.0746730076407296));
#74688=CARTESIAN_POINT('Ctrl Pts',(35.1510759787713,-3.2227488984055,-0.00266464371426724));
#74689=CARTESIAN_POINT('Ctrl Pts',(35.1510761725173,-3.22274889603389,-0.00266751051583289));
#74690=CARTESIAN_POINT('Ctrl Pts',(35.1619186355403,-3.22261610378722,-0.163100267507248));
#74691=CARTESIAN_POINT('Ctrl Pts',(35.1726751749668,-3.21050356731146,-0.323323489996479));
#74692=CARTESIAN_POINT('Ctrl Pts',(35.1836396978217,-3.18469468457042,-0.493946725074042));
#74693=CARTESIAN_POINT('Ctrl Pts',(35.1844042266867,-3.18282006570918,-0.505885402975079));
#74694=CARTESIAN_POINT('Ctrl Pts',(35.185590766742,-3.17979244483891,-0.524483786703438));
#74695=CARTESIAN_POINT('Ctrl Pts',(35.1860152095985,-3.17868559656821,-0.53115074588874));
#74696=CARTESIAN_POINT('Ctrl Pts',(35.1867253485776,-3.17679349744505,-0.542329799525009));
#74697=CARTESIAN_POINT('Ctrl Pts',(35.1870116660491,-3.17601959156579,-0.54684375416133));
#74698=CARTESIAN_POINT('Ctrl Pts',(35.1875738124882,-3.1744783170012,-0.555719888449237));
#74699=CARTESIAN_POINT('Ctrl Pts',(35.187849675962,-3.17371157297722,-0.56008216508376));
#74700=CARTESIAN_POINT('Ctrl Pts',(35.1883779254982,-3.1722233160601,-0.568448190912915));
#74701=CARTESIAN_POINT('Ctrl Pts',(35.1886303878206,-3.17150321685426,-0.572452145013885));
#74702=CARTESIAN_POINT('Ctrl Pts',(35.1892148988959,-3.16981555422855,-0.581735092873558));
#74703=CARTESIAN_POINT('Ctrl Pts',(35.1895466268871,-3.16884237758759,-0.587013077455503));
#74704=CARTESIAN_POINT('Ctrl Pts',(35.1906191997119,-3.16564608459058,-0.60410845141004));
#74705=CARTESIAN_POINT('Ctrl Pts',(35.1913570782785,-3.16336998101465,-0.615916007076254));
#74706=CARTESIAN_POINT('Ctrl Pts',(35.2017150564923,-3.13033552276273,-0.782271034266164));
#74707=CARTESIAN_POINT('Ctrl Pts',(35.2107296928083,-3.08834382341957,-0.934395614647729));
#74708=CARTESIAN_POINT('Ctrl Pts',(35.2229259068031,-3.01555139663591,-1.13844214108711));
#74709=CARTESIAN_POINT('Ctrl Pts',(35.2262256114441,-2.99419755406352,-1.19347472122739));
#74710=CARTESIAN_POINT('Ctrl Pts',(35.2324329478645,-2.95118760173036,-1.29588545677335));
#74711=CARTESIAN_POINT('Ctrl Pts',(35.2353399305116,-2.92987106400019,-1.34338485903844));
#74712=CARTESIAN_POINT('Ctrl Pts',(35.2452770916432,-2.85338841379238,-1.5033209881666));
#74713=CARTESIAN_POINT('Ctrl Pts',(35.2523552413528,-2.79282754015025,-1.61304385644462));
#74714=CARTESIAN_POINT('Ctrl Pts',(35.2644373740046,-2.68185930772172,-1.78902469339391));
#74715=CARTESIAN_POINT('Ctrl Pts',(35.2693265013199,-2.63499651587901,-1.85735573684857));
#74716=CARTESIAN_POINT('Ctrl Pts',(35.275714643997,-2.571695293704,-1.94243148472485));
#74717=CARTESIAN_POINT('Ctrl Pts',(35.2771210796786,-2.55763327006465,-1.96091018890047));
#74718=CARTESIAN_POINT('Ctrl Pts',(35.27914641218,-2.53721197019249,-1.98715213852997));
#74719=CARTESIAN_POINT('Ctrl Pts',(35.2797589075699,-2.53101399694575,-1.9950404374439));
#74720=CARTESIAN_POINT('Ctrl Pts',(35.2808223726937,-2.52021479204133,-2.00865350598104));
#74721=CARTESIAN_POINT('Ctrl Pts',(35.2812726573704,-2.51563061000929,-2.01439175377605));
#74722=CARTESIAN_POINT('Ctrl Pts',(35.2821389115726,-2.50678949345152,-2.02538137053575));
#74723=CARTESIAN_POINT('Ctrl Pts',(35.2825547582483,-2.50253556835076,-2.03063511951808));
#74724=CARTESIAN_POINT('Ctrl Pts',(35.2835349216485,-2.49248629412709,-2.04296679345692));
#74725=CARTESIAN_POINT('Ctrl Pts',(35.2840997906074,-2.48667729879733,-2.05003347642359));
#74726=CARTESIAN_POINT('Ctrl Pts',(35.2857713058927,-2.4694366033465,-2.07082580176271));
#74727=CARTESIAN_POINT('Ctrl Pts',(35.2868813787977,-2.45792092855606,-2.08448106910328));
#74728=CARTESIAN_POINT('Ctrl Pts',(35.2993592257815,-2.32775899610887,-2.23624853271456));
#74729=CARTESIAN_POINT('Ctrl Pts',(35.3112142879728,-2.19774735677507,-2.36413955524367));
#74730=CARTESIAN_POINT('Ctrl Pts',(35.3302774196647,-1.97829108725116,-2.54619632976771));
#74731=CARTESIAN_POINT('Ctrl Pts',(35.3372550672089,-1.89581365979886,-2.6081872249002));
#74732=CARTESIAN_POINT('Ctrl Pts',(35.3539780663021,-1.69142004017044,-2.74698714086701));
#74733=CARTESIAN_POINT('Ctrl Pts',(35.3637106042693,-1.5670374361554,-2.81979421102691));
#74734=CARTESIAN_POINT('Ctrl Pts',(35.3755913348369,-1.4042216184317,-2.90098612572683));
#74735=CARTESIAN_POINT('Ctrl Pts',(35.3780460684144,-1.36994889415371,-2.91732739926484));
#74736=CARTESIAN_POINT('Ctrl Pts',(35.3819399525753,-1.31442912741162,-2.942605012417));
#74737=CARTESIAN_POINT('Ctrl Pts',(35.3833987176301,-1.29336194231337,-2.95192532907449));
#74738=CARTESIAN_POINT('Ctrl Pts',(35.3852833763351,-1.26576731740669,-2.96378130377405));
#74739=CARTESIAN_POINT('Ctrl Pts',(35.3857212183762,-1.25932965607741,-2.96652243172272));
#74740=CARTESIAN_POINT('Ctrl Pts',(35.386394066545,-1.24939423049461,-2.97071472179452));
#74741=CARTESIAN_POINT('Ctrl Pts',(35.386629965975,-1.24590280008205,-2.97218070018979));
#74742=CARTESIAN_POINT('Ctrl Pts',(35.3871157713353,-1.23869574655169,-2.97519185989066));
#74743=CARTESIAN_POINT('Ctrl Pts',(35.3873656214303,-1.23497985548337,-2.97673621815444));
#74744=CARTESIAN_POINT('Ctrl Pts',(35.3879317586139,-1.22653899885447,-2.98022578928774));
#74745=CARTESIAN_POINT('Ctrl Pts',(35.388247783352,-1.22181230584003,-2.98216672253603));
#74746=CARTESIAN_POINT('Ctrl Pts',(35.3891831544763,-1.20777877409992,-2.98789037958972));
#74747=CARTESIAN_POINT('Ctrl Pts',(35.3898005768387,-1.19845873694612,-2.9916408791332));
#74748=CARTESIAN_POINT('Ctrl Pts',(35.3941468799826,-1.13246377650996,-3.01784017551127));
#74749=CARTESIAN_POINT('Ctrl Pts',(35.3977864750939,-1.0751752243457,-3.03872224836789));
#74750=CARTESIAN_POINT('Ctrl Pts',(35.4022265879943,-1.00334178480227,-3.06261979052757));
#74751=CARTESIAN_POINT('Ctrl Pts',(35.4030870938265,-0.989327105896628,
-3.0671756728886));
#74752=CARTESIAN_POINT('Ctrl Pts',(35.4065544973521,-0.932506101081867,
-3.08521703111218));
#74753=CARTESIAN_POINT('Ctrl Pts',(35.4091329354071,-0.889450192956968,
-3.09790419263125));
#74754=CARTESIAN_POINT('Ctrl Pts',(35.4260760431206,-0.602516370728571,
-3.17597849379441));
#74755=CARTESIAN_POINT('Ctrl Pts',(35.4398053805642,-0.351946954142931,
-3.21341035213004));
#74756=CARTESIAN_POINT('Ctrl Pts',(35.4609886234768,0.0159826061019054,
-3.22478327776359));
#74757=CARTESIAN_POINT('Ctrl Pts',(35.4677803679812,0.131631623585466,-3.22213458006225));
#74758=CARTESIAN_POINT('Ctrl Pts',(35.4758258847611,0.264234804030499,-3.21194652834045));
#74759=CARTESIAN_POINT('Ctrl Pts',(35.4768831839327,0.281578333453512,-3.2104725752219));
#74760=CARTESIAN_POINT('Ctrl Pts',(35.4784892248803,0.307793913794964,-3.20803056394151));
#74761=CARTESIAN_POINT('Ctrl Pts',(35.4790347043618,0.316675468334443,-3.20716601344246));
#74762=CARTESIAN_POINT('Ctrl Pts',(35.4800179034934,0.332643161557032,-3.20554470795251));
#74763=CARTESIAN_POINT('Ctrl Pts',(35.4804551989288,0.339730622306593,-3.20480131218513));
#74764=CARTESIAN_POINT('Ctrl Pts',(35.481395504283,0.354939228024015,-3.20315508130235));
#74765=CARTESIAN_POINT('Ctrl Pts',(35.4818987447456,0.363059507725923,-3.20224485671336));
#74766=CARTESIAN_POINT('Ctrl Pts',(35.4832613080726,0.384993352690459,-3.19970173011544));
#74767=CARTESIAN_POINT('Ctrl Pts',(35.4841224755046,0.398799832331221,-3.19801027629641));
#74768=CARTESIAN_POINT('Ctrl Pts',(35.4867809858683,0.441246170580943,-3.19253096495631));
#74769=CARTESIAN_POINT('Ctrl Pts',(35.4885876307851,0.469845772670512,-3.18844742899992));
#74770=CARTESIAN_POINT('Ctrl Pts',(35.507637912639,0.768783809597302,-3.14165489459676));
#74771=CARTESIAN_POINT('Ctrl Pts',(35.5260248103655,1.0326371498629,-3.06506506031414));
#74772=CARTESIAN_POINT('Ctrl Pts',(35.55268024069,1.39392490682922,-2.90818884758759));
#74773=CARTESIAN_POINT('Ctrl Pts',(35.5608028844359,1.50150592627978,-2.85413246914246));
#74774=CARTESIAN_POINT('Ctrl Pts',(35.5719355347804,1.64814583285149,-2.76985853927283));
#74775=CARTESIAN_POINT('Ctrl Pts',(35.5751136288798,1.68991843646663,-2.74457232164209));
#74776=CARTESIAN_POINT('Ctrl Pts',(35.5794232953742,1.74665404528642,-2.70844182810834));
#74777=CARTESIAN_POINT('Ctrl Pts',(35.5805974204871,1.76212064698642,-2.6984047789682));
#74778=CARTESIAN_POINT('Ctrl Pts',(35.5823419444932,1.78512859667937,-2.68319158470917));
#74779=CARTESIAN_POINT('Ctrl Pts',(35.5829183468193,1.79273514110954,-2.67811536447158));
#74780=CARTESIAN_POINT('Ctrl Pts',(35.5839647097358,1.80655389755418,-2.66880817339567));
#74781=CARTESIAN_POINT('Ctrl Pts',(35.5844353381918,1.8127730822346,-2.66458773662323));
#74782=CARTESIAN_POINT('Ctrl Pts',(35.5851838539894,1.82267157812968,-2.65781976558723));
#74783=CARTESIAN_POINT('Ctrl Pts',(35.5854626793158,1.82636039944118,-2.65528628964999));
#74784=CARTESIAN_POINT('Ctrl Pts',(35.5859917611571,1.83336335498208,-2.65045517474856));
#74785=CARTESIAN_POINT('Ctrl Pts',(35.5862421096316,1.83667841470282,-2.64815902579592));
#74786=CARTESIAN_POINT('Ctrl Pts',(35.5868140096072,1.84425451551665,-2.64289043200747));
#74787=CARTESIAN_POINT('Ctrl Pts',(35.5871352774869,1.84851267618509,-2.63991390777859));
#74788=CARTESIAN_POINT('Ctrl Pts',(35.5881232234822,1.86161325689899,-2.63070914817417));
#74789=CARTESIAN_POINT('Ctrl Pts',(35.5887875899389,1.87043164752207,-2.62444660838729));
#74790=CARTESIAN_POINT('Ctrl Pts',(35.5941572573658,1.94175587741265,-2.57325231492583));
#74791=CARTESIAN_POINT('Ctrl Pts',(35.5987195271814,2.00267073561076,-2.52613448806674));
#74792=CARTESIAN_POINT('Ctrl Pts',(35.6047616711685,2.0826110855344,-2.45958913330616));
#74793=CARTESIAN_POINT('Ctrl Pts',(35.6063199416966,2.10315973829833,-2.44204152643267));
#74794=CARTESIAN_POINT('Ctrl Pts',(35.6237749902183,2.33215990364585,-2.24145118054918));
#74795=CARTESIAN_POINT('Ctrl Pts',(35.6387662671737,2.51636259911403,-2.03248790616208));
#74796=CARTESIAN_POINT('Ctrl Pts',(35.658890701615,2.71128307532589,-1.74359181342733));
#74797=CARTESIAN_POINT('Ctrl Pts',(35.6630490833056,2.74907040725976,-1.68338325866498));
#74798=CARTESIAN_POINT('Ctrl Pts',(35.6698653824782,2.80671948699116,-1.58440337404542));
#74799=CARTESIAN_POINT('Ctrl Pts',(35.6724784229749,2.82784047241329,-1.54639138517793));
#74800=CARTESIAN_POINT('Ctrl Pts',(35.6758954238782,2.85416655670975,-1.49666771048175));
#74801=CARTESIAN_POINT('Ctrl Pts',(35.6766741227786,2.8600805708126,-1.48533500939412));
#74802=CARTESIAN_POINT('Ctrl Pts',(35.6779391693011,2.86954939238842,-1.4669241896655));
#74803=CARTESIAN_POINT('Ctrl Pts',(35.6784240439373,2.87314584181258,-1.45986754998023));
#74804=CARTESIAN_POINT('Ctrl Pts',(35.6793541197731,2.87998152516894,-1.44633206588444));
#74805=CARTESIAN_POINT('Ctrl Pts',(35.6797991681869,2.88322500452995,-1.439855410105));
#74806=CARTESIAN_POINT('Ctrl Pts',(35.6808134902275,2.89055477241374,-1.42509508001197));
#74807=CARTESIAN_POINT('Ctrl Pts',(35.6813832404057,2.89462732432263,-1.41680469008169));
#74808=CARTESIAN_POINT('Ctrl Pts',(35.6831574655498,2.90717058841364,-1.39099085410641));
#74809=CARTESIAN_POINT('Ctrl Pts',(35.6843662132921,2.91551811245241,-1.37340834988258));
#74810=CARTESIAN_POINT('Ctrl Pts',(35.7009476070123,3.02732062719227,-1.13230397110782));
#74811=CARTESIAN_POINT('Ctrl Pts',(35.717245886225,3.10495694190771,-0.897762264905472));
#74812=CARTESIAN_POINT('Ctrl Pts',(35.7442841419308,3.18649195883906,-0.506039312820335));
#74813=CARTESIAN_POINT('Ctrl Pts',(35.754758986728,3.20702199870698,-0.353298352941245));
#74814=CARTESIAN_POINT('Ctrl Pts',(35.7687787635256,3.22014467818334,-0.141901427182443));
#74815=CARTESIAN_POINT('Ctrl Pts',(35.772565735669,3.22217404457667,-0.0840418297419472));
#74816=CARTESIAN_POINT('Ctrl Pts',(35.7783016471311,3.22289863767436,0.00523574299113315));
#74817=CARTESIAN_POINT('Ctrl Pts',(35.7802981966691,3.22269474554549,0.0366305350771588));
#74818=CARTESIAN_POINT('Ctrl Pts',(35.7827610966504,3.22186730775691,0.075826090997907));
#74819=CARTESIAN_POINT('Ctrl Pts',(35.7832501753731,3.22167411116111,0.0836329441804956));
#74820=CARTESIAN_POINT('Ctrl Pts',(35.7840224995579,3.22132308875262,0.0959996654043833));
#74821=CARTESIAN_POINT('Ctrl Pts',(35.7843067778593,3.22118395481501,0.100559970901961));
#74822=CARTESIAN_POINT('Ctrl Pts',(35.7848413388266,3.220903572792,0.109151298472018));
#74823=CARTESIAN_POINT('Ctrl Pts',(35.7850917340939,3.22076444303738,0.113182303575542));
#74824=CARTESIAN_POINT('Ctrl Pts',(35.7856641252704,3.22042852499624,0.122412189675962));
#74825=CARTESIAN_POINT('Ctrl Pts',(35.7859858357635,3.22022671562632,0.127610852440287));
#74826=CARTESIAN_POINT('Ctrl Pts',(35.7869764874582,3.2195650855084,0.143652358469452));
#74827=CARTESIAN_POINT('Ctrl Pts',(35.7876430986058,3.21906307787263,0.154493522368231));
#74828=CARTESIAN_POINT('Ctrl Pts',(35.7930796772694,3.21450271169469,0.243269780588717));
#74829=CARTESIAN_POINT('Ctrl Pts',(35.7977026066793,3.20766910592091,0.321043645601942));
#74830=CARTESIAN_POINT('Ctrl Pts',(35.803761805331,3.19476370753438,0.424611395409422));
#74831=CARTESIAN_POINT('Ctrl Pts',(35.8052788302377,3.1911901855223,0.450683083871293));
#74832=CARTESIAN_POINT('Ctrl Pts',(35.8145419605233,3.16728853908643,0.610490690108467));
#74833=CARTESIAN_POINT('Ctrl Pts',(35.8220678377394,3.13887537559548,0.742886507228558));
#74834=CARTESIAN_POINT('Ctrl Pts',(35.8433012124546,3.03596051382057,1.10855066781525));
#74835=CARTESIAN_POINT('Ctrl Pts',(35.8570829529927,2.94312241202374,1.33564526553336));
#74836=CARTESIAN_POINT('Ctrl Pts',(35.8730327844104,2.81610925627517,1.56717194329522));
#74837=CARTESIAN_POINT('Ctrl Pts',(35.8742181785233,2.8065573374075,1.58421435701194));
#74838=CARTESIAN_POINT('Ctrl Pts',(35.8759791993935,2.79220526021841,1.60928393739835));
#74839=CARTESIAN_POINT('Ctrl Pts',(35.8765505298628,2.78752404393566,1.61737896237576));
#74840=CARTESIAN_POINT('Ctrl Pts',(35.8775663575245,2.77915707303021,1.63170337832467));
#74841=CARTESIAN_POINT('Ctrl Pts',(35.8780103397202,2.77548542390749,1.6379409671076));
#74842=CARTESIAN_POINT('Ctrl Pts',(35.8788825942787,2.76824337690093,1.65014986372986));
#74843=CARTESIAN_POINT('Ctrl Pts',(35.8793108059672,2.76467459224511,1.65612208617163));
#74844=CARTESIAN_POINT('Ctrl Pts',(35.8804748286046,2.75493714414894,1.67229813876974));
#74845=CARTESIAN_POINT('Ctrl Pts',(35.881212005277,2.7487311913592,1.68247929100381));
#74846=CARTESIAN_POINT('Ctrl Pts',(35.8839931462954,2.72517237336327,1.72065035759566));
#74847=CARTESIAN_POINT('Ctrl Pts',(35.8860508051543,2.70744779033035,1.74840740401792));
#74848=CARTESIAN_POINT('Ctrl Pts',(35.9052476929829,2.5394394191109,2.0028296290539));
#74849=CARTESIAN_POINT('Ctrl Pts',(35.923510490241,2.36148212710625,2.20984651698626));
#74850=CARTESIAN_POINT('Ctrl Pts',(35.9501514007285,2.0693086690558,2.47364362567509));
#74851=CARTESIAN_POINT('Ctrl Pts',(35.9583776039676,1.97435077787986,2.55007713701945));
#74852=CARTESIAN_POINT('Ctrl Pts',(35.9686858107573,1.84699442295384,2.64120041730075));
#74853=CARTESIAN_POINT('Ctrl Pts',(35.970958031864,1.81837287744804,2.66098631872296));
#74854=CARTESIAN_POINT('Ctrl Pts',(35.9732071344081,1.7894362098569,2.68030513437425));
#74855=CARTESIAN_POINT('Origin',(-1.72497344927317,0.,0.));
#74856=CARTESIAN_POINT('',(37.4669394326166,1.78943621037803,2.68030513402633));
#74857=CARTESIAN_POINT('',(37.2205445093424,1.78943610171058,2.68030520657533));
#74858=CARTESIAN_POINT('',(-1.72497344927317,1.78943621037804,2.68030513402633));
#74859=CARTESIAN_POINT('',(36.6465734492396,-3.22274964508592,0.00151248092928333));
#74860=CARTESIAN_POINT('Ctrl Pts',(36.6465734492731,-3.22274964508618,0.00151248038429142));
#74861=CARTESIAN_POINT('Ctrl Pts',(36.6528250213268,-3.222797401118,-0.100244696904469));
#74862=CARTESIAN_POINT('Ctrl Pts',(36.6590765933804,-3.21802138921175,-0.201988221218814));
#74863=CARTESIAN_POINT('Ctrl Pts',(36.6653281654341,-3.20845189099051,-0.303239221901459));
#74864=CARTESIAN_POINT('Ctrl Pts',(36.6715822484097,-3.19887854921391,-0.404530889693085));
#74865=CARTESIAN_POINT('Ctrl Pts',(36.6778363313853,-3.18450792857277,-0.505329227822775));
#74866=CARTESIAN_POINT('Ctrl Pts',(36.684090414361,-3.1654220506495,-0.605161799655191));
#74867=CARTESIAN_POINT('Ctrl Pts',(36.6903484556982,-3.14632409280857,-0.705057557957362));
#74868=CARTESIAN_POINT('Ctrl Pts',(36.6966064970355,-3.12250501607544,-0.803985927111695));
#74869=CARTESIAN_POINT('Ctrl Pts',(36.7028645383728,-3.0940974981539,-0.901486680111143));
#74870=CARTESIAN_POINT('Ctrl Pts',(36.7091322606066,-3.06564603513406,-0.999138262203995));
#74871=CARTESIAN_POINT('Ctrl Pts',(36.7153999828405,-3.03259207630555,-1.0953574213286));
#74872=CARTESIAN_POINT('Ctrl Pts',(36.7216677050743,-2.99511760116889,-1.18970085217601));
#74873=CARTESIAN_POINT('Ctrl Pts',(36.7279411298304,-2.95760903086611,-1.284130118914));
#74874=CARTESIAN_POINT('Ctrl Pts',(36.7342145545865,-2.91567210274627,-1.3766798814995));
#74875=CARTESIAN_POINT('Ctrl Pts',(36.7404879793427,-2.86953532638981,-1.46693032319225));
#74876=CARTESIAN_POINT('Ctrl Pts',(36.7467724924765,-2.82331700255023,-1.55734028397047));
#74877=CARTESIAN_POINT('Ctrl Pts',(36.7530570056102,-2.7728842156572,-1.64544245211922));
#74878=CARTESIAN_POINT('Ctrl Pts',(36.759341518744,-2.71850948289369,-1.7308448093105));
#74879=CARTESIAN_POINT('Ctrl Pts',(36.7607694189635,-2.70615503455451,-1.75024902439975));
#74880=CARTESIAN_POINT('Ctrl Pts',(36.762197319183,-2.69359725225644,-1.7695139980812));
#74881=CARTESIAN_POINT('Ctrl Pts',(36.7636252194025,-2.68083961826775,-1.78863537469939));
#74882=CARTESIAN_POINT('Ctrl Pts',(36.7697974674953,-2.62569341058482,-1.87128952570457));
#74883=CARTESIAN_POINT('Ctrl Pts',(36.775969715588,-2.56662403811661,-1.95153641178811));
#74884=CARTESIAN_POINT('Ctrl Pts',(36.7821419636808,-2.50386856205166,-2.02897998670991));
#74885=CARTESIAN_POINT('Ctrl Pts',(36.7883058523334,-2.44119807943436,-2.10631867522429));
#74886=CARTESIAN_POINT('Ctrl Pts',(36.7944697409861,-2.37485168704783,-2.1808612644059));
#74887=CARTESIAN_POINT('Ctrl Pts',(36.8006336296387,-2.30511004539246,-2.2522400496241));
#74888=CARTESIAN_POINT('Ctrl Pts',(36.8067909912972,-2.23544225375432,-2.32354325123983));
#74889=CARTESIAN_POINT('Ctrl Pts',(36.8129483529558,-2.16238666245251,-2.39168900038535));
#74890=CARTESIAN_POINT('Ctrl Pts',(36.8191057146143,-2.08626395056914,-2.45634286919714));
#74891=CARTESIAN_POINT('Ctrl Pts',(36.8252585787606,-2.01019684088149,-2.52094951298267));
#74892=CARTESIAN_POINT('Ctrl Pts',(36.831411442907,-1.93106739481383,-2.58206906705413));
#74893=CARTESIAN_POINT('Ctrl Pts',(36.8375643070533,-1.84923220187827,-2.63940482420497));
#74894=CARTESIAN_POINT('Ctrl Pts',(36.8437148401898,-1.76742801216814,-2.69671885973042));
#74895=CARTESIAN_POINT('Ctrl Pts',(36.8498653733263,-1.6829204677553,-2.75025169770129));
#74896=CARTESIAN_POINT('Ctrl Pts',(36.8560159064629,-1.59609749413888,-2.79974826577383));
#74897=CARTESIAN_POINT('Ctrl Pts',(36.8621657546781,-1.50928418910006,-2.84923932192494));
#74898=CARTESIAN_POINT('Ctrl Pts',(36.8683156028933,-1.42015634485385,-2.89469478667634));
#74899=CARTESIAN_POINT('Ctrl Pts',(36.8744654511085,-1.32912811845297,-2.93590463183627));
#74900=CARTESIAN_POINT('Ctrl Pts',(36.8806162594876,-1.23808567999067,-2.97712091100985));
#74901=CARTESIAN_POINT('Ctrl Pts',(36.8867670678668,-1.14514266579525,-3.01409007481787));
#74902=CARTESIAN_POINT('Ctrl Pts',(36.8929178762459,-1.05073398516574,-3.04664990685141));
#74903=CARTESIAN_POINT('Ctrl Pts',(36.8990752626121,-0.956224339095592,
-3.07924456002393));
#74904=CARTESIAN_POINT('Ctrl Pts',(36.9052326489783,-0.860246307979682,
-3.10742032303051));
#74905=CARTESIAN_POINT('Ctrl Pts',(36.9113900353445,-0.763250656020162,
-3.13106467492845));
#74906=CARTESIAN_POINT('Ctrl Pts',(36.9175508580815,-0.666200871835899,
-3.15472222248356));
#74907=CARTESIAN_POINT('Ctrl Pts',(36.9237116808184,-0.568132762157658,
-3.17384323946745));
#74908=CARTESIAN_POINT('Ctrl Pts',(36.9298725035554,-0.469505925725956,
-3.18836662700641));
#74909=CARTESIAN_POINT('Ctrl Pts',(36.9360436264721,-0.370714196684077,
-3.20291429596173));
#74910=CARTESIAN_POINT('Ctrl Pts',(36.9422147493888,-0.271362307421376,
-3.21284893828179));
#74911=CARTESIAN_POINT('Ctrl Pts',(36.9483858723055,-0.171913744599385,
-3.21816146688102));
#74912=CARTESIAN_POINT('Ctrl Pts',(36.953081394251,-0.0962447106994679,
-3.22220369630358));
#74913=CARTESIAN_POINT('Ctrl Pts',(36.9577769161965,-0.0205197875028225,
-3.22357104151303));
#74914=CARTESIAN_POINT('Ctrl Pts',(36.9624724381421,0.0550585900731698,
-3.22227964555517));
#74915=CARTESIAN_POINT('Ctrl Pts',(36.9686446862348,0.154406117836357,-3.22058210983277));
#74916=CARTESIAN_POINT('Ctrl Pts',(36.9748169343276,0.253849928258262,-3.21428274012976));
#74917=CARTESIAN_POINT('Ctrl Pts',(36.9809891824204,0.352928682299329,-3.20336680817393));
#74918=CARTESIAN_POINT('Ctrl Pts',(36.987153071073,0.451873248132202,-3.19246566030945));
#74919=CARTESIAN_POINT('Ctrl Pts',(36.9933169597256,0.550453312332139,-3.17696042484048));
#74920=CARTESIAN_POINT('Ctrl Pts',(36.9994808483783,0.648207802479794,-3.156888374223));
#74921=CARTESIAN_POINT('Ctrl Pts',(37.0056382100368,0.745858779566933,-3.13683757807052));
#74922=CARTESIAN_POINT('Ctrl Pts',(37.0117955716954,0.84268549745669,-3.1122296677612));
#74923=CARTESIAN_POINT('Ctrl Pts',(37.0179529333539,0.938233237985931,-3.08315357282741));
#74924=CARTESIAN_POINT('Ctrl Pts',(37.0241057975002,1.0337111877254,-3.05409871590111));
#74925=CARTESIAN_POINT('Ctrl Pts',(37.0302586616465,1.12791160314956,-3.02058228920045));
#74926=CARTESIAN_POINT('Ctrl Pts',(37.0364115257928,1.22039207991097,-2.98274382637708));
#74927=CARTESIAN_POINT('Ctrl Pts',(37.0425620589294,1.31283752048611,-2.94491969863802));
#74928=CARTESIAN_POINT('Ctrl Pts',(37.0487125920659,1.40356391554019,-2.90277695259075));
#74929=CARTESIAN_POINT('Ctrl Pts',(37.0548631252025,1.49214694065446,-2.85650399439517));
#74930=CARTESIAN_POINT('Ctrl Pts',(37.0610129734177,1.58072010119239,-2.81023618914088));
#74931=CARTESIAN_POINT('Ctrl Pts',(37.0671628216329,1.66714998131957,-2.75983928728214));
#74932=CARTESIAN_POINT('Ctrl Pts',(37.0733126698481,1.7510359644898,-2.70554811702976));
#74933=CARTESIAN_POINT('Ctrl Pts',(37.0794634782272,1.83493504461644,-2.65124847040191));
#74934=CARTESIAN_POINT('Ctrl Pts',(37.0856142866063,1.91628907419751,-2.59305358376017));
#74935=CARTESIAN_POINT('Ctrl Pts',(37.0917650949854,1.9947264354327,-2.53124159461043));
#74936=CARTESIAN_POINT('Ctrl Pts',(37.0979224813516,2.07324768156821,-2.46936350057819));
#74937=CARTESIAN_POINT('Ctrl Pts',(37.1040798677178,2.14884568873491,-2.40386084879743));
#74938=CARTESIAN_POINT('Ctrl Pts',(37.110237254084,2.22118207049317,-2.33505198490733));
#74939=CARTESIAN_POINT('Ctrl Pts',(37.1163980768209,2.29355882240419,-2.26620471953406));
#74940=CARTESIAN_POINT('Ctrl Pts',(37.1225588995579,2.36267002338088,-2.19404788114744));
#74941=CARTESIAN_POINT('Ctrl Pts',(37.1287197222949,2.42821576676111,-2.11893505151828));
#74942=CARTESIAN_POINT('Ctrl Pts',(37.1348908452116,2.49387109500778,-2.04369664196617));
#74943=CARTESIAN_POINT('Ctrl Pts',(37.1410619681282,2.55594878849473,-1.96549270990756));
#74944=CARTESIAN_POINT('Ctrl Pts',(37.1472330910449,2.61419059110094,-1.88470823097351));
#74945=CARTESIAN_POINT('Ctrl Pts',(37.1519286129905,2.65850597194506,-1.82324043997018));
#74946=CARTESIAN_POINT('Ctrl Pts',(37.1566241349361,2.70060143625978,-1.7602792971095));
#74947=CARTESIAN_POINT('Ctrl Pts',(37.1613196568817,2.74038110508653,-1.69600382115864));
#74948=CARTESIAN_POINT('Ctrl Pts',(37.1674919049745,2.79267134840589,-1.61151392026039));
#74949=CARTESIAN_POINT('Ctrl Pts',(37.1736641530672,2.84114254897881,-1.52445476677892));
#74950=CARTESIAN_POINT('Ctrl Pts',(37.17983640116,2.885532866509,-1.43520647949916));
#74951=CARTESIAN_POINT('Ctrl Pts',(37.1860002898126,2.92986306361038,-1.34607906644603));
#74952=CARTESIAN_POINT('Ctrl Pts',(37.1921641784653,2.97012317141227,-1.2547687981058));
#74953=CARTESIAN_POINT('Ctrl Pts',(37.1983280671179,3.00609523725876,-1.1616836863063));
#74954=CARTESIAN_POINT('Ctrl Pts',(37.2044854287765,3.04202921197908,-1.06869714312258));
#74955=CARTESIAN_POINT('Ctrl Pts',(37.210642790435,3.07368401626014,-0.973939895837431));
#74956=CARTESIAN_POINT('Ctrl Pts',(37.2168001520936,3.10088858765053,-0.87784254253181));
#74957=CARTESIAN_POINT('Ctrl Pts',(37.2229530162399,3.12807328804748,-0.781815381468874));
#74958=CARTESIAN_POINT('Ctrl Pts',(37.2291058803862,3.15081410029398,-0.684450477200166));
#74959=CARTESIAN_POINT('Ctrl Pts',(37.2352587445325,3.16898918878107,-0.586195431480566));
#74960=CARTESIAN_POINT('Ctrl Pts',(37.2414092776691,3.1871573916442,-0.487977609640144));
#74961=CARTESIAN_POINT('Ctrl Pts',(37.2475598108056,3.20076322877482,-0.388870743077388));
#74962=CARTESIAN_POINT('Ctrl Pts',(37.2537103439421,3.20973575255615,-0.289333650415608));
#74963=CARTESIAN_POINT('Ctrl Pts',(37.2598601921574,3.2187072771602,-0.18980764217155));
#74964=CARTESIAN_POINT('Ctrl Pts',(37.2660100403726,3.22304647522968,-0.0898519357018265));
#74965=CARTESIAN_POINT('Ctrl Pts',(37.2721598885878,3.2227342688803,0.0100694927657119));
#74966=CARTESIAN_POINT('Ctrl Pts',(37.2783106969669,3.22242201378675,0.110006521772982));
#74967=CARTESIAN_POINT('Ctrl Pts',(37.284461505346,3.21745691318152,0.209908827734067));
#74968=CARTESIAN_POINT('Ctrl Pts',(37.2906123137252,3.20787200126423,0.30931341064534));
#74969=CARTESIAN_POINT('Ctrl Pts',(37.2967697000914,3.19827683875502,0.408824301869322));
#74970=CARTESIAN_POINT('Ctrl Pts',(37.3029270864576,3.18405204071588,0.507835973901786));
#74971=CARTESIAN_POINT('Ctrl Pts',(37.3090844728238,3.16528243332354,0.605891640306602));
#74972=CARTESIAN_POINT('Ctrl Pts',(37.3152452955607,3.14650235081623,0.704002030518734));
#74973=CARTESIAN_POINT('Ctrl Pts',(37.3214061182977,3.12317250916127,0.801154930191059));
#74974=CARTESIAN_POINT('Ctrl Pts',(37.3275669410347,3.09542818189315,0.896906869882096));
#74975=CARTESIAN_POINT('Ctrl Pts',(37.3337380639514,3.0676374693337,0.992818895689989));
#74976=CARTESIAN_POINT('Ctrl Pts',(37.3399091868681,3.03541766905999,1.08732487163034));
#74977=CARTESIAN_POINT('Ctrl Pts',(37.3460803097848,2.99895298427561,1.17999939008645));
#74978=CARTESIAN_POINT('Ctrl Pts',(37.3507758317303,2.97120751072827,1.25051414746174));
#74979=CARTESIAN_POINT('Ctrl Pts',(37.3554713536758,2.94100548468902,1.3199689619039));
#74980=CARTESIAN_POINT('Ctrl Pts',(37.3601668756214,2.90844565560598,1.38818638189787));
#74981=CARTESIAN_POINT('Ctrl Pts',(37.3663388278917,2.86564791909001,1.47785365746173));
#74982=CARTESIAN_POINT('Ctrl Pts',(37.3725107801621,2.81862431437544,1.56569771632256));
#74983=CARTESIAN_POINT('Ctrl Pts',(37.3786827324324,2.76755299425081,1.65129282276444));
#74984=CARTESIAN_POINT('Ctrl Pts',(37.384846680592,2.71654790608681,1.7367769249929));
#74985=CARTESIAN_POINT('Ctrl Pts',(37.3910106287516,2.66150575392245,1.82001750060698));
#74986=CARTESIAN_POINT('Ctrl Pts',(37.3971745769113,2.60265191622203,1.90061057702145));
#74987=CARTESIAN_POINT('Ctrl Pts',(37.4033313459559,2.54386662524833,1.98110978714272));
#74988=CARTESIAN_POINT('Ctrl Pts',(37.4094881150005,2.48127873417071,2.05896728283734));
#74989=CARTESIAN_POINT('Ctrl Pts',(37.4156448840451,2.41515788910051,2.13380644230342));
#74990=CARTESIAN_POINT('Ctrl Pts',(37.4217974226011,2.34908247751702,2.2085941776845));
#74991=CARTESIAN_POINT('Ctrl Pts',(37.427949961157,2.27947922316048,2.28036737424976));
#74992=CARTESIAN_POINT('Ctrl Pts',(37.434102499713,2.20665871918159,2.34878156914599));
#74993=CARTESIAN_POINT('Ctrl Pts',(37.4402531847559,2.13386015309898,2.41717515359008));
#74994=CARTESIAN_POINT('Ctrl Pts',(37.4464038697989,2.05784657591176,2.48221144628947));
#74995=CARTESIAN_POINT('Ctrl Pts',(37.4525545548418,1.97896560744366,2.54358264797021));
#74996=CARTESIAN_POINT('Ctrl Pts',(37.4573495141001,1.91747147672217,2.59142649132029));
#74997=CARTESIAN_POINT('Ctrl Pts',(37.4621444733583,1.85423549402089,2.63704357283874));
#74998=CARTESIAN_POINT('Ctrl Pts',(37.4669394326166,1.78943621037803,2.68030513402633));
#74999=CARTESIAN_POINT('Ctrl Pts',(36.2170783832723,1.78943621037801,2.68030513402635));
#75000=CARTESIAN_POINT('Ctrl Pts',(36.2232805665494,1.70580874151773,2.7361368447749));
#75001=CARTESIAN_POINT('Ctrl Pts',(36.2294827498265,1.61949287711907,2.78809966004317));
#75002=CARTESIAN_POINT('Ctrl Pts',(36.2356849331037,1.53088469535462,2.83593187718411));
#75003=CARTESIAN_POINT('Ctrl Pts',(36.241835971149,1.44300720563696,2.88336965421863));
#75004=CARTESIAN_POINT('Ctrl Pts',(36.2479870091944,1.35287545759231,2.92674450276665));
#75005=CARTESIAN_POINT('Ctrl Pts',(36.2541380472397,1.26090307854026,2.96584574599349));
#75006=CARTESIAN_POINT('Ctrl Pts',(36.260287924438,1.16894805686143,3.00493960988669));
#75007=CARTESIAN_POINT('Ctrl Pts',(36.2664378016363,1.07515349425653,3.03976130157094));
#75008=CARTESIAN_POINT('Ctrl Pts',(36.2725876788347,0.979954194461434,3.07014777156694));
#75009=CARTESIAN_POINT('Ctrl Pts',(36.2787380404257,0.884747396330164,3.10053663494154));
#75010=CARTESIAN_POINT('Ctrl Pts',(36.2848884020167,0.788136055225419,3.12648945097924));
#75011=CARTESIAN_POINT('Ctrl Pts',(36.2910387636077,0.69057040552706,3.14789295839458));
#75012=CARTESIAN_POINT('Ctrl Pts',(36.297279765134,0.591566898226102,3.16961189645539));
#75013=CARTESIAN_POINT('Ctrl Pts',(36.3035207666603,0.491581175418993,3.18664624558934));
#75014=CARTESIAN_POINT('Ctrl Pts',(36.3097617681866,0.391093102908749,3.19893165718763));
#75015=CARTESIAN_POINT('Ctrl Pts',(36.315921497213,0.291913621147141,3.21105708386872));
#75016=CARTESIAN_POINT('Ctrl Pts',(36.3220812262394,0.192245238270418,3.21855655792975));
#75017=CARTESIAN_POINT('Ctrl Pts',(36.3282409552658,0.0925517978440608,
3.22142076221282));
#75018=CARTESIAN_POINT('Ctrl Pts',(36.3345225930421,-0.00911470059073392,
3.22434165268482));
#75019=CARTESIAN_POINT('Ctrl Pts',(36.3408042308183,-0.110806781691359,
3.22244185568611));
#75020=CARTESIAN_POINT('Ctrl Pts',(36.3470858685945,-0.212036920502237,
3.2157670790721));
#75021=CARTESIAN_POINT('Ctrl Pts',(36.3533675063707,-0.313267059313115,
3.2090923024581));
#75022=CARTESIAN_POINT('Ctrl Pts',(36.3596491441469,-0.414034794378422,
3.19764266511839));
#75023=CARTESIAN_POINT('Ctrl Pts',(36.3659307819232,-0.51386405013367,3.18151870974857));
#75024=CARTESIAN_POINT('Ctrl Pts',(36.3721030300159,-0.611954859471789,
3.16567554012869));
#75025=CARTESIAN_POINT('Ctrl Pts',(36.3782752781087,-0.709484931127417,
3.14526381279472));
#75026=CARTESIAN_POINT('Ctrl Pts',(36.3844475262015,-0.805995538434842,
3.12033471834724));
#75027=CARTESIAN_POINT('Ctrl Pts',(36.3906114148541,-0.902375435726782,
3.09543938684471));
#75028=CARTESIAN_POINT('Ctrl Pts',(36.3967753035068,-0.997738196136775,
3.06603895637837));
#75029=CARTESIAN_POINT('Ctrl Pts',(36.4029391921594,-1.09163277011398,3.0322360491415));
#75030=CARTESIAN_POINT('Ctrl Pts',(36.4090965538179,-1.18542791832857,2.99846893609048));
#75031=CARTESIAN_POINT('Ctrl Pts',(36.4152539154765,-1.27775756450784,2.96030876073085));
#75032=CARTESIAN_POINT('Ctrl Pts',(36.421411277135,-1.36818431268288,2.91790836885405));
#75033=CARTESIAN_POINT('Ctrl Pts',(36.4275641412813,-1.45854501058682,2.87553894743051));
#75034=CARTESIAN_POINT('Ctrl Pts',(36.4337170054276,-1.547005181805,2.82893565105665));
#75035=CARTESIAN_POINT('Ctrl Pts',(36.4398698695739,-1.63314683253052,2.7782996573256));
#75036=CARTESIAN_POINT('Ctrl Pts',(36.4460204027105,-1.71925584853101,2.72768284701764));
#75037=CARTESIAN_POINT('Ctrl Pts',(36.452170935847,-1.8030477153014,2.67303659493187));
#75038=CARTESIAN_POINT('Ctrl Pts',(36.4583214689835,-1.8841293015575,2.614607874522));
#75039=CARTESIAN_POINT('Ctrl Pts',(36.4644713171987,-1.96520185859486,2.55618566071519));
#75040=CARTESIAN_POINT('Ctrl Pts',(36.4706211654139,-2.04356438276439,2.49398206997094));
#75041=CARTESIAN_POINT('Ctrl Pts',(36.4767710136291,-2.11885382642875,2.42828664385575));
#75042=CARTESIAN_POINT('Ctrl Pts',(36.4829218220083,-2.19415502488912,2.36258096084006));
#75043=CARTESIAN_POINT('Ctrl Pts',(36.4890726303874,-2.26638186252413,2.29338264521252));
#75044=CARTESIAN_POINT('Ctrl Pts',(36.4952234387666,-2.33520616842251,2.22101997142337));
#75045=CARTESIAN_POINT('Ctrl Pts',(36.5013808251327,-2.40410407853083,2.14857990931386));
#75046=CARTESIAN_POINT('Ctrl Pts',(36.5075382114989,-2.46959189057255,2.07296904665602));
#75047=CARTESIAN_POINT('Ctrl Pts',(36.5136955978651,-2.53138005764479,1.9945507178957));
#75048=CARTESIAN_POINT('Ctrl Pts',(36.5198564206021,-2.5932027080252,1.91608862471373));
#75049=CARTESIAN_POINT('Ctrl Pts',(36.526017243339,-2.65132134887475,1.83481629847544));
#75050=CARTESIAN_POINT('Ctrl Pts',(36.532178066076,-2.70548954330138,1.75112646419008));
#75051=CARTESIAN_POINT('Ctrl Pts',(36.5383491889927,-2.75974830065476,1.66729671022655));
#75052=CARTESIAN_POINT('Ctrl Pts',(36.5445203119094,-2.81004320002142,1.58104175027761));
#75053=CARTESIAN_POINT('Ctrl Pts',(36.5506914348261,-2.85617350514434,1.49277944486502));
#75054=CARTESIAN_POINT('Ctrl Pts',(36.5553869567716,-2.8912734153203,1.42562187927663));
#75055=CARTESIAN_POINT('Ctrl Pts',(36.5600824787172,-2.9239631907279,1.35730268570755));
#75056=CARTESIAN_POINT('Ctrl Pts',(36.5647780006628,-2.95417345259417,1.28801272295263));
#75057=CARTESIAN_POINT('Ctrl Pts',(36.5715942880442,-2.99802839122183,1.18742746230242));
#75058=CARTESIAN_POINT('Ctrl Pts',(36.5784105754256,-3.03678939838922,1.08449244505177));
#75059=CARTESIAN_POINT('Ctrl Pts',(36.585226862807,-3.07022405146555,0.979715181214655));
#75060=CARTESIAN_POINT('Ctrl Pts',(36.5920141814928,-3.10351660984527,0.875383212666901));
#75061=CARTESIAN_POINT('Ctrl Pts',(36.5988015001786,-3.13152785282194,0.769224872399252));
#75062=CARTESIAN_POINT('Ctrl Pts',(36.6055888188644,-3.15407435744704,0.661764693977453));
#75063=CARTESIAN_POINT('Ctrl Pts',(36.6124195905936,-3.17676520688476,0.553616545532031));
#75064=CARTESIAN_POINT('Ctrl Pts',(36.6192503623228,-3.19392090784062,0.444150068994009));
#75065=CARTESIAN_POINT('Ctrl Pts',(36.626081134052,-3.20540400980987,0.333920194649572));
#75066=CARTESIAN_POINT('Ctrl Pts',(36.6329119057812,-3.21688711177912,0.223690320305166));
#75067=CARTESIAN_POINT('Ctrl Pts',(36.6397426775104,-3.22269746450369,0.112697322741449));
#75068=CARTESIAN_POINT('Ctrl Pts',(36.6465734492396,-3.22274964508592,0.00151248092933596));
#75069=CARTESIAN_POINT('Ctrl Pts',(35.9732071344081,1.7894362098569,2.68030513437425));
#75070=CARTESIAN_POINT('Ctrl Pts',(35.9741186123143,1.77770925091503,2.68813433437576));
#75071=CARTESIAN_POINT('Ctrl Pts',(35.9750262904335,1.76593053683883,2.69588682130556));
#75072=CARTESIAN_POINT('Ctrl Pts',(35.977713407941,1.73074853339878,2.71871329221958));
#75073=CARTESIAN_POINT('Ctrl Pts',(35.9794806339119,1.70719996623789,2.7335619348491));
#75074=CARTESIAN_POINT('Ctrl Pts',(35.9816994319375,1.67706897147055,2.75201987975685));
#75075=CARTESIAN_POINT('Ctrl Pts',(35.9821687391261,1.67066319774735,2.75591332156977));
#75076=CARTESIAN_POINT('Ctrl Pts',(35.9829169893021,1.66039664631732,2.7621044010783));
#75077=CARTESIAN_POINT('Ctrl Pts',(35.9831968595434,1.65654459551128,2.76441634874886));
#75078=CARTESIAN_POINT('Ctrl Pts',(35.9837279472292,1.64921170208059,2.76879661912018));
#75079=CARTESIAN_POINT('Ctrl Pts',(35.9839792573544,1.6457318381304,2.7708664120543));
#75080=CARTESIAN_POINT('Ctrl Pts',(35.9845547304197,1.63774067685999,2.77559912091324));
#75081=CARTESIAN_POINT('Ctrl Pts',(35.9848786015888,1.63322678629941,2.77825759606472));
#75082=CARTESIAN_POINT('Ctrl Pts',(35.9857390824225,1.62119064508468,2.78530686227322));
#75083=CARTESIAN_POINT('Ctrl Pts',(35.9862744496421,1.61365697967995,2.78967822172077));
#75084=CARTESIAN_POINT('Ctrl Pts',(35.9899584042047,1.56151310223042,2.819652452902));
#75085=CARTESIAN_POINT('Ctrl Pts',(35.9930433553004,1.51631034154117,2.84421637318373));
#75086=CARTESIAN_POINT('Ctrl Pts',(35.9969485933205,1.45743587726204,2.87440688941287));
#75087=CARTESIAN_POINT('Ctrl Pts',(35.9978135079042,1.44428969406905,2.88103481324579));
#75088=CARTESIAN_POINT('Ctrl Pts',(36.00874552682,1.27685295158687,2.96401747259804));
#75089=CARTESIAN_POINT('Ctrl Pts',(36.0183107427117,1.11671679414589,3.02798725712601));
#75090=CARTESIAN_POINT('Ctrl Pts',(36.0417314686228,0.716370608426992,3.15180566743302));
#75091=CARTESIAN_POINT('Ctrl Pts',(36.0556251678948,0.472954110497661,3.19739850834578));
#75092=CARTESIAN_POINT('Ctrl Pts',(36.071743569953,0.206626242784038,3.21618244905141));
#75093=CARTESIAN_POINT('Ctrl Pts',(36.0729663480509,0.186504645184643,3.21741199391175));
#75094=CARTESIAN_POINT('Ctrl Pts',(36.0747723446459,0.156914524420469,3.2189416117457));
#75095=CARTESIAN_POINT('Ctrl Pts',(36.07535093949,0.147453836660584,3.21938885983645));
#75096=CARTESIAN_POINT('Ctrl Pts',(36.0763750215052,0.130743654033602,3.22010501158632));
#75097=CARTESIAN_POINT('Ctrl Pts',(36.0768199641124,0.123494933816185,3.2203911546066));
#75098=CARTESIAN_POINT('Ctrl Pts',(36.0776905465913,0.109334797373467,3.22090224667221));
#75099=CARTESIAN_POINT('Ctrl Pts',(36.078116113773,0.102423497296265,3.22112943026915));
#75100=CARTESIAN_POINT('Ctrl Pts',(36.0792641296717,0.0838084266371843,
3.22168136132579));
#75101=CARTESIAN_POINT('Ctrl Pts',(36.0799878784939,0.07210361306308,3.22196457296839));
#75102=CARTESIAN_POINT('Ctrl Pts',(36.0826646126157,0.0289299351166631,
3.22277383408107));
#75103=CARTESIAN_POINT('Ctrl Pts',(36.0846300027322,-0.00254377873521497,
3.22290265795043));
#75104=CARTESIAN_POINT('Ctrl Pts',(36.1050154321242,-0.326576889170818,
3.21948256643101));
#75105=CARTESIAN_POINT('Ctrl Pts',(36.124761157141,-0.617302373908438,3.17656804775269));
#75106=CARTESIAN_POINT('Ctrl Pts',(36.1510765088031,-0.991124842285462,
3.06808695714326));
#75107=CARTESIAN_POINT('Ctrl Pts',(36.1575919963022,-1.08282312691447,3.03693627969966));
#75108=CARTESIAN_POINT('Ctrl Pts',(36.1674949724734,-1.22255751294971,2.98233188702151));
#75109=CARTESIAN_POINT('Ctrl Pts',(36.1709684349362,-1.27164646387149,2.96173366495804));
#75110=CARTESIAN_POINT('Ctrl Pts',(36.1762815803382,-1.3471912260389,2.92780949680161));
#75111=CARTESIAN_POINT('Ctrl Pts',(36.1781612735046,-1.37401008024242,2.91531972480208));
#75112=CARTESIAN_POINT('Ctrl Pts',(36.1805001655199,-1.40754799390382,2.89913518104887));
#75113=CARTESIAN_POINT('Ctrl Pts',(36.1809794746948,-1.41442992974098,2.89578385412785));
#75114=CARTESIAN_POINT('Ctrl Pts',(36.1817399068793,-1.42536374128204,2.89041109007756));
#75115=CARTESIAN_POINT('Ctrl Pts',(36.1820220099817,-1.42942335674865,2.88840560385652));
#75116=CARTESIAN_POINT('Ctrl Pts',(36.182554816216,-1.43709748504238,2.8845943746037));
#75117=CARTESIAN_POINT('Ctrl Pts',(36.1828056221963,-1.44071278531366,2.88279041172217));
#75118=CARTESIAN_POINT('Ctrl Pts',(36.1833766784246,-1.44895080290288,2.87866043713634));
#75119=CARTESIAN_POINT('Ctrl Pts',(36.1836966523751,-1.45357130889051,2.87633009100585));
#75120=CARTESIAN_POINT('Ctrl Pts',(36.1846944441557,-1.46799313462403,2.86901283598748));
#75121=CARTESIAN_POINT('Ctrl Pts',(36.1853698443605,-1.47777468214032,2.86398681794658));
#75122=CARTESIAN_POINT('Ctrl Pts',(36.1910752975701,-1.5605470088626,2.82091924096549));
#75123=CARTESIAN_POINT('Ctrl Pts',(36.1959416432411,-1.63208845255928,2.78014068176321));
#75124=CARTESIAN_POINT('Ctrl Pts',(36.2150917285888,-1.91284886304389,2.60552909192817));
#75125=CARTESIAN_POINT('Ctrl Pts',(36.2285735826886,-2.10785151510612,2.45045970750694));
#75126=CARTESIAN_POINT('Ctrl Pts',(36.2513750221016,-2.3912753237818,2.16596448068789));
#75127=CARTESIAN_POINT('Ctrl Pts',(36.2602676108545,-2.49153302444539,2.04984236909523));
#75128=CARTESIAN_POINT('Ctrl Pts',(36.270706176967,-2.59488306678859,1.91130448774902));
#75129=CARTESIAN_POINT('Ctrl Pts',(36.2718972951471,-2.60647772350059,1.89546216678164));
#75130=CARTESIAN_POINT('Ctrl Pts',(36.2736652099258,-2.62339113340421,1.87190392767963));
#75131=CARTESIAN_POINT('Ctrl Pts',(36.2742376608647,-2.62882228363083,1.86426895898914));
#75132=CARTESIAN_POINT('Ctrl Pts',(36.2752547564251,-2.63839121034164,1.85069225101053));
#75133=CARTESIAN_POINT('Ctrl Pts',(36.2756988814986,-2.64254242012419,1.84476002321267));
#75134=CARTESIAN_POINT('Ctrl Pts',(36.2765708572543,-2.65063936271733,1.83310579106032));
#75135=CARTESIAN_POINT('Ctrl Pts',(36.2769986453726,-2.654586647,1.82738490876055));
#75136=CARTESIAN_POINT('Ctrl Pts',(36.2781601109579,-2.66523568974777,1.81184371093194));
#75137=CARTESIAN_POINT('Ctrl Pts',(36.2788951435894,-2.67190161295433,1.80199907862279));
#75138=CARTESIAN_POINT('Ctrl Pts',(36.2816595673455,-2.696696129648,1.76494100805202));
#75139=CARTESIAN_POINT('Ctrl Pts',(36.2837024423475,-2.71446418660161,1.73748980719753));
#75140=CARTESIAN_POINT('Ctrl Pts',(36.3031422435098,-2.8782876996376,1.47573888429936));
#75141=CARTESIAN_POINT('Ctrl Pts',(36.3217015072401,-2.99405455496806,1.22389558357841));
#75142=CARTESIAN_POINT('Ctrl Pts',(36.348437615209,-3.1118041741739,0.846747939731584));
#75143=CARTESIAN_POINT('Ctrl Pts',(36.3564771865748,-3.140975310928,0.731152899988543));
#75144=CARTESIAN_POINT('Ctrl Pts',(36.3674813859943,-3.17285187458381,0.566960714525288));
#75145=CARTESIAN_POINT('Ctrl Pts',(36.3706128447901,-3.18096469716936,0.519516680882692));
#75146=CARTESIAN_POINT('Ctrl Pts',(36.3754587973901,-3.1920421341892,0.444681886771678));
#75147=CARTESIAN_POINT('Ctrl Pts',(36.3772056850026,-3.19572329295198,0.417405944967495));
#75148=CARTESIAN_POINT('Ctrl Pts',(36.379402682816,-3.19995846515099,0.382673660444147));
#75149=CARTESIAN_POINT('Ctrl Pts',(36.3798701138288,-3.20083645387982,0.375258986886533));
#75150=CARTESIAN_POINT('Ctrl Pts',(36.3806160782755,-3.20220069430102,0.363384643795507));
#75151=CARTESIAN_POINT('Ctrl Pts',(36.380895529182,-3.20270340990713,0.358926948953006));
#75152=CARTESIAN_POINT('Ctrl Pts',(36.381426304326,-3.20364235307471,0.350442069681884));
#75153=CARTESIAN_POINT('Ctrl Pts',(36.381677719315,-3.20408029034524,0.346415161029705));
#75154=CARTESIAN_POINT('Ctrl Pts',(36.3822540678485,-3.20506851836765,0.337166025535612));
#75155=CARTESIAN_POINT('Ctrl Pts',(36.3825787065722,-3.20561363823906,0.331943277488954));
#75156=CARTESIAN_POINT('Ctrl Pts',(36.3836057837671,-3.20730155176934,0.315379520007084));
#75157=CARTESIAN_POINT('Ctrl Pts',(36.384305596644,-3.20839696043669,0.304033614835384));
#75158=CARTESIAN_POINT('Ctrl Pts',(36.3909303954768,-3.21824106154852,0.196087170189352));
#75159=CARTESIAN_POINT('Ctrl Pts',(36.3966274657522,-3.22268558048147,0.0991332467784455));
#75160=CARTESIAN_POINT('Ctrl Pts',(36.4161689540792,-3.22290883677749,-0.240760994970365));
#75161=CARTESIAN_POINT('Ctrl Pts',(36.4293750420992,-3.19561283972274,-0.482885890304909));
#75162=CARTESIAN_POINT('Ctrl Pts',(36.4466838645332,-3.12773851163942,-0.779163845548733));
#75163=CARTESIAN_POINT('Ctrl Pts',(36.450192317602,-3.11241845861492,-0.838269228512858));
#75164=CARTESIAN_POINT('Ctrl Pts',(36.4587881355566,-3.07132427767243,-0.980095396770234));
#75165=CARTESIAN_POINT('Ctrl Pts',(36.463918368936,-3.04387670006028,-1.06227699931576));
#75166=CARTESIAN_POINT('Ctrl Pts',(36.4700803365586,-3.00775729576546,-1.15747358376793));
#75167=CARTESIAN_POINT('Ctrl Pts',(36.4710044139286,-3.00225941727521,-1.17166011556708));
#75168=CARTESIAN_POINT('Ctrl Pts',(36.472497995361,-2.99324417153111,-1.19444260767364));
#75169=CARTESIAN_POINT('Ctrl Pts',(36.4730653786993,-2.98978969638818,-1.20306333247977));
#75170=CARTESIAN_POINT('Ctrl Pts',(36.4740779774849,-2.98357199555874,-1.21838757430831));
#75171=CARTESIAN_POINT('Ctrl Pts',(36.4745226980718,-2.98082330790142,-1.22509695110969));
#75172=CARTESIAN_POINT('Ctrl Pts',(36.4754532961702,-2.97503427778503,-1.23909279093215));
#75173=CARTESIAN_POINT('Ctrl Pts',(36.4759393134086,-2.97198975695754,-1.2463774634127));
#75174=CARTESIAN_POINT('Ctrl Pts',(36.4772077062024,-2.96398958325967,-1.26532361923962));
#75175=CARTESIAN_POINT('Ctrl Pts',(36.4779915111077,-2.95899190717012,-1.27696710882121));
#75176=CARTESIAN_POINT('Ctrl Pts',(36.4814103401889,-2.93696042318549,-1.32747179849471));
#75177=CARTESIAN_POINT('Ctrl Pts',(36.4840691744175,-2.91922938776033,-1.36602247690401));
#75178=CARTESIAN_POINT('Ctrl Pts',(36.4911051830736,-2.87078292973119,-1.46610058839102));
#75179=CARTESIAN_POINT('Ctrl Pts',(36.4955231519047,-2.83885165664463,-1.52701202041522));
#75180=CARTESIAN_POINT('Ctrl Pts',(36.5104689705668,-2.72586286112991,-1.72673661569493));
#75181=CARTESIAN_POINT('Ctrl Pts',(36.5212580308052,-2.63638182239187,-1.86049154480157));
#75182=CARTESIAN_POINT('Ctrl Pts',(36.5403038706459,-2.46279362454057,-2.08215557903536));
#75183=CARTESIAN_POINT('Ctrl Pts',(36.5485062104486,-2.38298239156801,-2.17304412523397));
#75184=CARTESIAN_POINT('Ctrl Pts',(36.5583654369076,-2.2792765405919,-2.27854092800775));
#75185=CARTESIAN_POINT('Ctrl Pts',(36.5601615420715,-2.2600573257729,-2.29760554892307));
#75186=CARTESIAN_POINT('Ctrl Pts',(36.5635008379472,-2.2236744754282,-2.33279743531597));
#75187=CARTESIAN_POINT('Ctrl Pts',(36.5650464290956,-2.20656983617779,-2.34898311153141));
#75188=CARTESIAN_POINT('Ctrl Pts',(36.5701131039918,-2.14957312713693,-2.4017456092113));
#75189=CARTESIAN_POINT('Ctrl Pts',(36.5735931962215,-2.10893459104393,-2.43750739995751));
#75190=CARTESIAN_POINT('Ctrl Pts',(36.5775601725571,-2.06062544531364,-2.47790609138502));
#75191=CARTESIAN_POINT('Ctrl Pts',(36.5781155445077,-2.05381567615525,-2.4835533004731));
#75192=CARTESIAN_POINT('Ctrl Pts',(36.5789991226391,-2.04290550799125,-2.49252532837804));
#75193=CARTESIAN_POINT('Ctrl Pts',(36.5793286075796,-2.03882010328936,-2.49586818853822));
#75194=CARTESIAN_POINT('Ctrl Pts',(36.5799098819954,-2.03158215701297,-2.50176096816193));
#75195=CARTESIAN_POINT('Ctrl Pts',(36.5801619686742,-2.02843299594842,-2.50431499300444));
#75196=CARTESIAN_POINT('Ctrl Pts',(36.5806911484843,-2.02180064737811,-2.50967322579763));
#75197=CARTESIAN_POINT('Ctrl Pts',(36.5809681472508,-2.01831645036655,-2.51247612223156));
#75198=CARTESIAN_POINT('Ctrl Pts',(36.581702317734,-2.00904894645256,-2.51989973814567));
#75199=CARTESIAN_POINT('Ctrl Pts',(36.5821585858103,-2.00325549195663,-2.52450783243841));
#75200=CARTESIAN_POINT('Ctrl Pts',(36.5842636651153,-1.97637216857509,-2.54573992133799));
#75201=CARTESIAN_POINT('Ctrl Pts',(36.5858957145302,-1.95509017481341,-2.56212045281473));
#75202=CARTESIAN_POINT('Ctrl Pts',(36.6006000762666,-1.75963092139697,-2.70870957509641));
#75203=CARTESIAN_POINT('Ctrl Pts',(36.6126415570292,-1.57287101304347,-2.82126080471715));
#75204=CARTESIAN_POINT('Ctrl Pts',(36.6385496285038,-1.15372929339507,-3.01919566061869));
#75205=CARTESIAN_POINT('Ctrl Pts',(36.6524045964157,-0.920026144731918,
-3.09841289139467));
#75206=CARTESIAN_POINT('Ctrl Pts',(36.6684364760453,-0.660571862011332,
-3.15438448002207));
#75207=CARTESIAN_POINT('Ctrl Pts',(36.6696178495064,-0.641503477908418,
-3.15831757345088));
#75208=CARTESIAN_POINT('Ctrl Pts',(36.6713740264031,-0.613238650201305,
-3.16388102185212));
#75209=CARTESIAN_POINT('Ctrl Pts',(36.6719445680677,-0.604068637852739,
-3.16564461688406));
#75210=CARTESIAN_POINT('Ctrl Pts',(36.6729595043423,-0.587779199927651,
-3.16870407879051));
#75211=CARTESIAN_POINT('Ctrl Pts',(36.673403387158,-0.580662802089373,-3.17001587310287));
#75212=CARTESIAN_POINT('Ctrl Pts',(36.6743363670786,-0.565721861057963,
-3.17271799798426));
#75213=CARTESIAN_POINT('Ctrl Pts',(36.6748256189075,-0.557896481754156,
-3.17410337460058));
#75214=CARTESIAN_POINT('Ctrl Pts',(36.676111693057,-0.537352039781101,-3.17766216675373));
#75215=CARTESIAN_POINT('Ctrl Pts',(36.6769100194652,-0.524625004724335,
-3.17978814660827));
#75216=CARTESIAN_POINT('Ctrl Pts',(36.6804810888713,-0.467813515088797,
-3.18892783010006));
#75217=CARTESIAN_POINT('Ctrl Pts',(36.683280342245,-0.423600684910258,-3.1951013015825));
#75218=CARTESIAN_POINT('Ctrl Pts',(36.6907737645373,-0.30614901441594,-3.20902055904293));
#75219=CARTESIAN_POINT('Ctrl Pts',(36.6955155916123,-0.23275193445757,-3.21517734078655));
#75220=CARTESIAN_POINT('Ctrl Pts',(36.7198306769412,0.139059342776081,-3.23356830881318));
#75221=CARTESIAN_POINT('Ctrl Pts',(36.7405066947731,0.437878540012598,-3.20679320487276));
#75222=CARTESIAN_POINT('Ctrl Pts',(36.7654356679086,0.80552593068938,-3.12145216151649));
#75223=CARTESIAN_POINT('Ctrl Pts',(36.7705575909788,0.881665581068449,-3.10080695499617));
#75224=CARTESIAN_POINT('Ctrl Pts',(36.7762185304869,0.967367511749989,-3.0741561519716));
#75225=CARTESIAN_POINT('Ctrl Pts',(36.7769019718869,0.977741066551706,-3.07087257375926));
#75226=CARTESIAN_POINT('Ctrl Pts',(36.7779080799732,0.993055155222298,-3.06593968378723));
#75227=CARTESIAN_POINT('Ctrl Pts',(36.7782330670231,0.998008507813227,-3.06433087397199));
#75228=CARTESIAN_POINT('Ctrl Pts',(36.7788085185025,1.00679167227465,-3.06145461577495));
#75229=CARTESIAN_POINT('Ctrl Pts',(36.7790592645278,1.01062301867689,-3.06019197937034));
#75230=CARTESIAN_POINT('Ctrl Pts',(36.7795924740823,1.01877939006166,-3.05748702406157));
#75231=CARTESIAN_POINT('Ctrl Pts',(36.7798748178459,1.02310371362859,-3.05604272543634));
#75232=CARTESIAN_POINT('Ctrl Pts',(36.7806384001787,1.03481264310518,-3.05210437373569));
#75233=CARTESIAN_POINT('Ctrl Pts',(36.781118602623,1.04219134777408,-3.04959267970297));
#75234=CARTESIAN_POINT('Ctrl Pts',(36.783514286236,1.07907397612567,-3.03688842042406));
#75235=CARTESIAN_POINT('Ctrl Pts',(36.7854068516727,1.10843904017133,-3.02629393632444));
#75236=CARTESIAN_POINT('Ctrl Pts',(36.7907216554301,1.19136712430015,-2.99500561239376));
#75237=CARTESIAN_POINT('Ctrl Pts',(36.7940937095598,1.24453953762948,-2.97330395112609));
#75238=CARTESIAN_POINT('Ctrl Pts',(36.8062303632827,1.43645302021816,-2.88892561515328));
#75239=CARTESIAN_POINT('Ctrl Pts',(36.8146984536009,1.57129273925118,-2.81785976672978));
#75240=CARTESIAN_POINT('Ctrl Pts',(36.8371070735987,1.91187990190257,-2.60627945583568));
#75241=CARTESIAN_POINT('Ctrl Pts',(36.8511018884129,2.1072127423579,-2.45104231029528));
#75242=CARTESIAN_POINT('Ctrl Pts',(36.8672952836862,2.29645224480173,-2.26115052309472));
#75243=CARTESIAN_POINT('Ctrl Pts',(36.868473517801,2.3100340070721,-2.24727333926551));
#75244=CARTESIAN_POINT('Ctrl Pts',(36.8702198136267,2.32988396084766,-2.22662153160806));
#75245=CARTESIAN_POINT('Ctrl Pts',(36.8707836136004,2.3362499543421,-2.21994118482476));
#75246=CARTESIAN_POINT('Ctrl Pts',(36.8717921224686,2.34756073599831,-2.20796933925305));
#75247=CARTESIAN_POINT('Ctrl Pts',(36.872236350756,2.35251656297532,-2.20268831927018));
#75248=CARTESIAN_POINT('Ctrl Pts',(36.8731682884187,2.36285792177073,-2.19159366810999));
#75249=CARTESIAN_POINT('Ctrl Pts',(36.8736561460994,2.36823988871201,-2.18577679379563));
#75250=CARTESIAN_POINT('Ctrl Pts',(36.8749346018162,2.38226067001499,-2.170510443237));
#75251=CARTESIAN_POINT('Ctrl Pts',(36.8757266715596,2.39086465997479,-2.16102930433224));
#75252=CARTESIAN_POINT('Ctrl Pts',(36.8792313350736,2.42856868390872,-2.11898068880317));
#75253=CARTESIAN_POINT('Ctrl Pts',(36.8819692422436,2.45706030939448,-2.08587615776834));
#75254=CARTESIAN_POINT('Ctrl Pts',(36.8892617740853,2.53039459505167,-1.99708084030475));
#75255=CARTESIAN_POINT('Ctrl Pts',(36.8938609679564,2.57406992716853,-1.9404616563029));
#75256=CARTESIAN_POINT('Ctrl Pts',(36.9169210528835,2.78054479582112,-1.65354584610455));
#75257=CARTESIAN_POINT('Ctrl Pts',(36.9363631304863,2.91450025964948,-1.40402766612287));
#75258=CARTESIAN_POINT('Ctrl Pts',(36.9616399474412,3.04889490221409,-1.04877961788107));
#75259=CARTESIAN_POINT('Ctrl Pts',(36.9680439700766,3.07934484495578,-0.955687336357353));
#75260=CARTESIAN_POINT('Ctrl Pts',(36.9749438467709,3.10856379660807,-0.850340562763089));
#75261=CARTESIAN_POINT('Ctrl Pts',(36.9756614120413,3.11155723581187,-0.839320872941894));
#75262=CARTESIAN_POINT('Ctrl Pts',(36.97670435262,3.11584266434413,-0.823206940842209));
#75263=CARTESIAN_POINT('Ctrl Pts',(36.9770323368395,3.11718082319363,-0.818125230539963));
#75264=CARTESIAN_POINT('Ctrl Pts',(36.9776118939201,3.11952859825246,-0.809120077199282));
#75265=CARTESIAN_POINT('Ctrl Pts',(36.9778637580884,3.12054325234113,-0.805197979152317));
#75266=CARTESIAN_POINT('Ctrl Pts',(36.9783934688462,3.12266536032122,-0.796930809661828));
#75267=CARTESIAN_POINT('Ctrl Pts',(36.9786712174125,3.12377113961956,-0.792585349222883));
#75268=CARTESIAN_POINT('Ctrl Pts',(36.9794095091452,3.12669182348375,-0.78100666845305));
#75269=CARTESIAN_POINT('Ctrl Pts',(36.9798691305563,3.12849071041146,-0.773769379519499));
#75270=CARTESIAN_POINT('Ctrl Pts',(36.9820125721864,3.1367877872471,-0.73988657479942));
#75271=CARTESIAN_POINT('Ctrl Pts',(36.9836788768371,3.1429710245235,-0.713164092144977));
#75272=CARTESIAN_POINT('Ctrl Pts',(36.988209932356,3.15901296840076,-0.639569018783328));
#75273=CARTESIAN_POINT('Ctrl Pts',(36.9910406057058,3.16816944705662,-0.592548998008233));
#75274=CARTESIAN_POINT('Ctrl Pts',(37.0007336137894,3.19629145107302,-0.428755341376519));
#75275=CARTESIAN_POINT('Ctrl Pts',(37.0074020685398,3.20987547092154,-0.311148706877908));
#75276=CARTESIAN_POINT('Ctrl Pts',(37.0295626247875,3.23357570264587,0.0837801909215586));
#75277=CARTESIAN_POINT('Ctrl Pts',(37.044884553195,3.21438708930145,0.361565071211477));
#75278=CARTESIAN_POINT('Ctrl Pts',(37.0619370300203,3.15839107534176,0.640890675631692));
#75279=CARTESIAN_POINT('Ctrl Pts',(37.0623916430659,3.15687463751017,0.648319029873952));
#75280=CARTESIAN_POINT('Ctrl Pts',(37.0644690880412,3.14983780741904,0.682179203614099));
#75281=CARTESIAN_POINT('Ctrl Pts',(37.0661012904997,3.14401169270617,0.708545755175215));
#75282=CARTESIAN_POINT('Ctrl Pts',(37.0684123474123,3.13535080339916,0.745529025225156));
#75283=CARTESIAN_POINT('Ctrl Pts',(37.0690823240132,3.13279190056873,0.756209687104703));
#75284=CARTESIAN_POINT('Ctrl Pts',(37.070168517851,3.12856601318455,0.773458584215435));
#75285=CARTESIAN_POINT('Ctrl Pts',(37.0705836419275,3.12693280558143,0.780035068838096));
#75286=CARTESIAN_POINT('Ctrl Pts',(37.0714493542964,3.12348922551498,0.793716815164936));
#75287=CARTESIAN_POINT('Ctrl Pts',(37.071900054716,3.12167532328016,0.800821140574469));
#75288=CARTESIAN_POINT('Ctrl Pts',(37.0729649536656,3.11733985957578,0.81756284136249));
#75289=CARTESIAN_POINT('Ctrl Pts',(37.0735798128605,3.11479783700592,0.827194796095611));
#75290=CARTESIAN_POINT('Ctrl Pts',(37.0756081157084,3.10628524859561,0.858854101788282));
#75291=CARTESIAN_POINT('Ctrl Pts',(37.0770276947857,3.10012546085512,0.880829437268086));
#75292=CARTESIAN_POINT('Ctrl Pts',(37.0884058372798,3.04916199250557,1.0554842380729));
#75293=CARTESIAN_POINT('Ctrl Pts',(37.0987283662029,2.99334713802395,1.20469712668627));
#75294=CARTESIAN_POINT('Ctrl Pts',(37.1215802222119,2.84957042113543,1.51659379870485));
#75295=CARTESIAN_POINT('Ctrl Pts',(37.1341637674022,2.75816436501057,1.67709019465128));
#75296=CARTESIAN_POINT('Ctrl Pts',(37.1555686746182,2.57747707362098,1.93925200526032));
#75297=CARTESIAN_POINT('Ctrl Pts',(37.1644515391825,2.49458384830556,2.044785266828));
#75298=CARTESIAN_POINT('Ctrl Pts',(37.1735989676574,2.39818285805468,2.15289396878105));
#75299=CARTESIAN_POINT('Ctrl Pts',(37.1742760834683,2.39097759215961,2.16089324654482));
#75300=CARTESIAN_POINT('Ctrl Pts',(37.1752821031806,2.3801662523534,2.17277570195034));
#75301=CARTESIAN_POINT('Ctrl Pts',(37.1756132191062,2.37659055540104,2.17668623663545));
#75302=CARTESIAN_POINT('Ctrl Pts',(37.1761814687019,2.37042392839877,2.18339701288422));
#75303=CARTESIAN_POINT('Ctrl Pts',(37.1764189527889,2.36783765517095,2.18620149009971));
#75304=CARTESIAN_POINT('Ctrl Pts',(37.1769112799696,2.36245699275374,2.19201537055341));
#75305=CARTESIAN_POINT('Ctrl Pts',(37.177166058175,2.35966183218356,2.1950240238465));
#75306=CARTESIAN_POINT('Ctrl Pts',(37.1777728490376,2.35297946720843,2.20218926904811));
#75307=CARTESIAN_POINT('Ctrl Pts',(37.1781244559008,2.34908696505018,2.20634094863468));
#75308=CARTESIAN_POINT('Ctrl Pts',(37.1793085879291,2.33590991201172,2.22032097745005));
#75309=CARTESIAN_POINT('Ctrl Pts',(37.1801372710837,2.32657436194683,2.23010136837593));
#75310=CARTESIAN_POINT('Ctrl Pts',(37.1821077759072,2.3041112438841,2.25334027173706));
#75311=CARTESIAN_POINT('Ctrl Pts',(37.1832454875708,2.29092676943774,2.26674338604494));
#75312=CARTESIAN_POINT('Ctrl Pts',(37.197057997158,2.1283476524747,2.4291509929166));
#75313=CARTESIAN_POINT('Ctrl Pts',(37.2087592672923,1.96482590108901,2.5632107659461));
#75314=CARTESIAN_POINT('Ctrl Pts',(37.2205445093424,1.78943610171065,2.68030520657529));
#75315=CARTESIAN_POINT('Origin',(-1.72497344927317,0.,0.));
#75316=CARTESIAN_POINT('',(38.7168453967856,1.78943621037805,2.68030513402632));
#75317=CARTESIAN_POINT('',(38.470402238185,1.78943621037805,2.68030513402632));
#75318=CARTESIAN_POINT('',(-1.72497344927317,1.78943621037804,2.68030513402633));
#75319=CARTESIAN_POINT('',(37.8965734493324,-3.22274881024213,-0.00276922063369994));
#75320=CARTESIAN_POINT('Ctrl Pts',(37.8965734493324,-3.22274881024213,-0.00276922063374366));
#75321=CARTESIAN_POINT('Ctrl Pts',(37.903965412188,-3.22264570243583,-0.122763473181237));
#75322=CARTESIAN_POINT('Ctrl Pts',(37.9113573750437,-3.2158370897087,-0.242465150599442));
#75323=CARTESIAN_POINT('Ctrl Pts',(37.9187493378993,-3.20244346561688,-0.361211035307264));
#75324=CARTESIAN_POINT('Ctrl Pts',(37.9262403139818,-3.18887043776371,-0.481547487154726));
#75325=CARTESIAN_POINT('Ctrl Pts',(37.9337312900642,-3.16853487915056,-0.600902356567945));
#75326=CARTESIAN_POINT('Ctrl Pts',(37.9412222661466,-3.14161120691717,-0.718607394251148));
#75327=CARTESIAN_POINT('Ctrl Pts',(37.9463843547112,-3.12305789970835,-0.799718830508165));
#75328=CARTESIAN_POINT('Ctrl Pts',(37.9515464432757,-3.10137711637387,-0.880047272850072));
#75329=CARTESIAN_POINT('Ctrl Pts',(37.9567085318403,-3.07663900274975,-0.95938001295578));
#75330=CARTESIAN_POINT('Ctrl Pts',(37.9628807799331,-3.04705993359477,-1.05423722969816));
#75331=CARTESIAN_POINT('Ctrl Pts',(37.9690530280258,-3.01303781465099,-1.14789217570988));
#75332=CARTESIAN_POINT('Ctrl Pts',(37.9752252761186,-2.97468830410308,-1.23989800222935));
#75333=CARTESIAN_POINT('Ctrl Pts',(37.9813891647712,-2.93639073256224,-1.33177921982407));
#75334=CARTESIAN_POINT('Ctrl Pts',(37.9875530534238,-2.89377758413291,-1.42201535984317));
#75335=CARTESIAN_POINT('Ctrl Pts',(37.9937169420765,-2.8470143423638,-1.51017445908571));
#75336=CARTESIAN_POINT('Ctrl Pts',(37.999874303735,-2.80030061858893,-1.59824020590862));
#75337=CARTESIAN_POINT('Ctrl Pts',(38.0060316653936,-2.74944574071772,-1.68423290294603));
#75338=CARTESIAN_POINT('Ctrl Pts',(38.0121890270521,-2.69466297521651,-1.76774121762698));
#75339=CARTESIAN_POINT('Ctrl Pts',(38.0183418911984,-2.6399202246067,-1.85118853545768));
#75340=CARTESIAN_POINT('Ctrl Pts',(38.0244947553447,-2.58125552805605,-1.93215471669091));
#75341=CARTESIAN_POINT('Ctrl Pts',(38.030647619491,-2.51892724787893,-2.01025448199801));
#75342=CARTESIAN_POINT('Ctrl Pts',(38.0367981526276,-2.45662258074225,-2.08832465924473));
#75343=CARTESIAN_POINT('Ctrl Pts',(38.0429486857641,-2.39065735847169,-2.16353023918866));
#75344=CARTESIAN_POINT('Ctrl Pts',(38.0490992189006,-2.32133175534108,-2.2355170417926));
#75345=CARTESIAN_POINT('Ctrl Pts',(38.0552490671158,-2.25201387228662,-2.30749582797009));
#75346=CARTESIAN_POINT('Ctrl Pts',(38.0613989153311,-2.17933665367041,-2.37625623656383));
#75347=CARTESIAN_POINT('Ctrl Pts',(38.0675487635463,-2.10363815089778,-2.44147989805105));
#75348=CARTESIAN_POINT('Ctrl Pts',(38.0736995719254,-2.02792782946396,-2.50671374278271));
#75349=CARTESIAN_POINT('Ctrl Pts',(38.0798503803046,-1.94919561604475,-2.56840946006127));
#75350=CARTESIAN_POINT('Ctrl Pts',(38.0860011886837,-1.86781296363155,-2.62628869231658));
#75351=CARTESIAN_POINT('Ctrl Pts',(38.0921585750499,-1.78634327647428,-2.68422982356409));
#75352=CARTESIAN_POINT('Ctrl Pts',(38.0983159614161,-1.702217844763,-2.73834606712631));
#75353=CARTESIAN_POINT('Ctrl Pts',(38.1044733477823,-1.6158373563824,-2.78840226657115));
#75354=CARTESIAN_POINT('Ctrl Pts',(38.1106341705192,-1.52940865998501,-2.83848640183979));
#75355=CARTESIAN_POINT('Ctrl Pts',(38.1167949932562,-1.44072278615831,-2.88450578047512));
#75356=CARTESIAN_POINT('Ctrl Pts',(38.1229558159932,-1.3502034099302,-2.92627208480566));
#75357=CARTESIAN_POINT('Ctrl Pts',(38.1291269389099,-1.25953269582335,-2.96810821754381));
#75358=CARTESIAN_POINT('Ctrl Pts',(38.1352980618266,-1.16702275890909,-3.00567690916634));
#75359=CARTESIAN_POINT('Ctrl Pts',(38.1414691847433,-1.07311568222778,-3.03883864248446));
#75360=CARTESIAN_POINT('Ctrl Pts',(38.1461647066888,-1.00166308837199,-3.06407094601336));
#75361=CARTESIAN_POINT('Ctrl Pts',(38.1508602286344,-0.929402004252621,
-3.08675286277535));
#75362=CARTESIAN_POINT('Ctrl Pts',(38.1555557505799,-0.856531192177784,
-3.10684275098153));
#75363=CARTESIAN_POINT('Ctrl Pts',(38.1617279986727,-0.760742750325845,
-3.13325084269148));
#75364=CARTESIAN_POINT('Ctrl Pts',(38.1679002467655,-0.66356326681565,-3.15527132121878));
#75365=CARTESIAN_POINT('Ctrl Pts',(38.1740724948582,-0.565431172373414,
-3.17275986355861));
#75366=CARTESIAN_POINT('Ctrl Pts',(38.1802363835109,-0.467431984022516,
-3.19022472013264));
#75367=CARTESIAN_POINT('Ctrl Pts',(38.1864002721635,-0.368483172980994,
-3.20316976466903));
#75368=CARTESIAN_POINT('Ctrl Pts',(38.1925641608161,-0.269037589193264,
-3.21150063647839));
#75369=CARTESIAN_POINT('Ctrl Pts',(38.1987215224747,-0.169697309179329,
-3.21982268665679));
#75370=CARTESIAN_POINT('Ctrl Pts',(38.2048788841332,-0.0698617327023847,
-3.22354024184912));
#75371=CARTESIAN_POINT('Ctrl Pts',(38.2110362457918,0.030007808250163,-3.22261029197513));
#75372=CARTESIAN_POINT('Ctrl Pts',(38.2171891099381,0.1298044016469,-3.221681021363));
#75373=CARTESIAN_POINT('Ctrl Pts',(38.2233419740844,0.229634477148471,-3.21611099890156));
#75374=CARTESIAN_POINT('Ctrl Pts',(38.2294948382307,0.329034235200374,-3.20590923679478));
#75375=CARTESIAN_POINT('Ctrl Pts',(38.2356453713673,0.428396335699355,-3.19571133962092));
#75376=CARTESIAN_POINT('Ctrl Pts',(38.2417959045038,0.527328011053883,-3.18088523374493));
#75377=CARTESIAN_POINT('Ctrl Pts',(38.2479464376403,0.62536901455604,-3.16149191966913));
#75378=CARTESIAN_POINT('Ctrl Pts',(38.2540962858555,0.723399100244558,-3.14210076522636));
#75379=CARTESIAN_POINT('Ctrl Pts',(38.2602461340708,0.820538285155734,-3.11814349805032));
#75380=CARTESIAN_POINT('Ctrl Pts',(38.266395982286,0.916335966152786,-3.08973234433581));
#75381=CARTESIAN_POINT('Ctrl Pts',(38.2725467906651,1.01214860385687,-3.0613167548427));
#75382=CARTESIAN_POINT('Ctrl Pts',(38.2786975990443,1.10661890514633,-3.02844602113245));
#75383=CARTESIAN_POINT('Ctrl Pts',(38.2848484074234,1.199311864716,-2.99128210198427));
#75384=CARTESIAN_POINT('Ctrl Pts',(38.2910057937896,1.29210395484706,-2.95407843785237));
#75385=CARTESIAN_POINT('Ctrl Pts',(38.2971631801558,1.38311450363477,-2.91257258179275));
#75386=CARTESIAN_POINT('Ctrl Pts',(38.303320566522,1.47192903935023,-2.86697444453513));
#75387=CARTESIAN_POINT('Ctrl Pts',(38.3094813892589,1.56079314149801,-2.82135085945001));
#75388=CARTESIAN_POINT('Ctrl Pts',(38.3156422119959,1.64745841307979,-2.77163066105908));
#75389=CARTESIAN_POINT('Ctrl Pts',(38.3218030347328,1.73153735416595,-2.71806842327929));
#75390=CARTESIAN_POINT('Ctrl Pts',(38.3279741576495,1.81575686547165,-2.66441663566187));
#75391=CARTESIAN_POINT('Ctrl Pts',(38.3341452805662,1.89738105387448,-2.60691022831736));
#75392=CARTESIAN_POINT('Ctrl Pts',(38.3403164034829,1.97605351744507,-2.54584564706758));
#75393=CARTESIAN_POINT('Ctrl Pts',(38.3450119254285,2.03591430521375,-2.4993824530544));
#75394=CARTESIAN_POINT('Ctrl Pts',(38.3497074473741,2.09406684386339,-2.45086012958568));
#75395=CARTESIAN_POINT('Ctrl Pts',(38.3544029693197,2.15036863113482,-2.40042336114515));
#75396=CARTESIAN_POINT('Ctrl Pts',(38.3605752174125,2.2243771445932,-2.33412439557355));
#75397=CARTESIAN_POINT('Ctrl Pts',(38.3667474655052,2.29544690919835,-2.26428284598557));
#75398=CARTESIAN_POINT('Ctrl Pts',(38.372919713598,2.36321945516923,-2.19118948728987));
#75399=CARTESIAN_POINT('Ctrl Pts',(38.3790836022506,2.43090021277835,-2.11819512324686));
#75400=CARTESIAN_POINT('Ctrl Pts',(38.3852474909033,2.49529233492339,-2.0419580194834));
#75401=CARTESIAN_POINT('Ctrl Pts',(38.3914113795559,2.55607158394951,-1.96280809561858));
#75402=CARTESIAN_POINT('Ctrl Pts',(38.3975687412144,2.61678647331225,-1.88374198428087));
#75403=CARTESIAN_POINT('Ctrl Pts',(38.403726102873,2.67389583231662,-1.80176952755802));
#75404=CARTESIAN_POINT('Ctrl Pts',(38.4098834645315,2.72711403357044,-1.71725554603943));
#75405=CARTESIAN_POINT('Ctrl Pts',(38.4160363286778,2.78029336273509,-1.63280329593881));
#75406=CARTESIAN_POINT('Ctrl Pts',(38.4221891928241,2.82958695419273,-1.54581357835062));
#75407=CARTESIAN_POINT('Ctrl Pts',(38.4283420569704,2.87475160792161,-1.45668141858544));
#75408=CARTESIAN_POINT('Ctrl Pts',(38.434492590107,2.91989915104207,-1.36758302649827));
#75409=CARTESIAN_POINT('Ctrl Pts',(38.4406431232435,2.960920668463,-1.27634419204506));
#75410=CARTESIAN_POINT('Ctrl Pts',(38.44679365638,2.9976186142432,-1.18338506245544));
#75411=CARTESIAN_POINT('Ctrl Pts',(38.4529435045952,3.03431247335233,-1.09043628476366));
#75412=CARTESIAN_POINT('Ctrl Pts',(38.4590933528104,3.06668355855487,-0.99576799683915));
#75413=CARTESIAN_POINT('Ctrl Pts',(38.4652432010256,3.0945826297964,-0.899819931909951));
#75414=CARTESIAN_POINT('Ctrl Pts',(38.4713940094048,3.12248605686606,-0.803856886794599));
#75415=CARTESIAN_POINT('Ctrl Pts',(38.4775448177839,3.14591596186266,-0.706614084941657));
#75416=CARTESIAN_POINT('Ctrl Pts',(38.483695626163,3.1647733741324,-0.608545029461781));
#75417=CARTESIAN_POINT('Ctrl Pts',(38.4898530125292,3.18365095347711,-0.510371093950314));
#75418=CARTESIAN_POINT('Ctrl Pts',(38.4960103988954,3.19794619297597,-0.411369567671443));
#75419=CARTESIAN_POINT('Ctrl Pts',(38.5021677852616,3.20761156229836,-0.312002608819048));
#75420=CARTESIAN_POINT('Ctrl Pts',(38.5083286079985,3.21728232575888,-0.212580194341048));
#75421=CARTESIAN_POINT('Ctrl Pts',(38.5144894307355,3.22231805138747,-0.112792374975328));
#75422=CARTESIAN_POINT('Ctrl Pts',(38.5206502534724,3.22272336385277,-0.0131027698404472));
#75423=CARTESIAN_POINT('Ctrl Pts',(38.5268213763891,3.22312935395341,0.0867535047302972));
#75424=CARTESIAN_POINT('Ctrl Pts',(38.5329924993058,3.21888948591141,0.186510802894764));
#75425=CARTESIAN_POINT('Ctrl Pts',(38.5391636222225,3.21006042242216,0.285709024881714));
#75426=CARTESIAN_POINT('Ctrl Pts',(38.5438591441681,3.20334251031245,0.361187577908209));
#75427=CARTESIAN_POINT('Ctrl Pts',(38.5485546661136,3.19396877235967,0.436342528928671));
#75428=CARTESIAN_POINT('Ctrl Pts',(38.5532501880592,3.18198386601061,0.510975771390588));
#75429=CARTESIAN_POINT('Ctrl Pts',(38.5594232188451,3.16622774843368,0.609093362728268));
#75430=CARTESIAN_POINT('Ctrl Pts',(38.565596249631,3.14590140604225,0.706654222548105));
#75431=CARTESIAN_POINT('Ctrl Pts',(38.571769280417,3.12105563561883,0.803199403555509));
#75432=CARTESIAN_POINT('Ctrl Pts',(38.5779319860937,3.09625142262508,0.899583101561941));
#75433=CARTESIAN_POINT('Ctrl Pts',(38.5840946917705,3.06694292998563,0.994954083968358));
#75434=CARTESIAN_POINT('Ctrl Pts',(38.5902573974472,3.03323231316575,1.08886146817085));
#75435=CARTESIAN_POINT('Ctrl Pts',(38.596414199088,2.99955399201324,1.18267888660201));
#75436=CARTESIAN_POINT('Ctrl Pts',(38.6025710007288,2.96148207180857,1.27503508647626));
#75437=CARTESIAN_POINT('Ctrl Pts',(38.6087278023696,2.91916895414155,1.36549265090522));
#75438=CARTESIAN_POINT('Ctrl Pts',(38.6148803527234,2.87688505378917,1.45588775415739));
#75439=CARTESIAN_POINT('Ctrl Pts',(38.6210329030771,2.8303659597981,1.54438643542387));
#75440=CARTESIAN_POINT('Ctrl Pts',(38.6271854534308,2.77981243089773,1.63057057851736));
#75441=CARTESIAN_POINT('Ctrl Pts',(38.6333354012549,2.72928028614738,1.71671826570591));
#75442=CARTESIAN_POINT('Ctrl Pts',(38.6394853490789,2.67471731938183,1.80055298741101));
#75443=CARTESIAN_POINT('Ctrl Pts',(38.6456352969029,2.61637006536727,1.88168149365138));
#75444=CARTESIAN_POINT('Ctrl Pts',(38.6517864454348,2.55801141971113,1.96282583931522));
#75445=CARTESIAN_POINT('Ctrl Pts',(38.6579375939666,2.49586725562134,2.04126255476866));
#75446=CARTESIAN_POINT('Ctrl Pts',(38.6640887424984,2.43022696041206,2.1166280928369));
#75447=CARTESIAN_POINT('Ctrl Pts',(38.670240264458,2.36458268027065,2.19199820624339));
#75448=CARTESIAN_POINT('Ctrl Pts',(38.6763917864175,2.29544213822753,2.26429644875661));
#75449=CARTESIAN_POINT('Ctrl Pts',(38.6825433083771,2.22313342363478,2.33319423606735));
#75450=CARTESIAN_POINT('Ctrl Pts',(38.6887005649325,2.15075730112979,2.40215625154238));
#75451=CARTESIAN_POINT('Ctrl Pts',(38.694857821488,2.07520742646403,2.46771118470814));
#75452=CARTESIAN_POINT('Ctrl Pts',(38.7010150780434,1.99684684859484,2.5295691778951));
#75453=CARTESIAN_POINT('Ctrl Pts',(38.7062918509574,1.92969178186814,2.58258151870483));
#75454=CARTESIAN_POINT('Ctrl Pts',(38.7115686238715,1.86047308150388,2.63287920932439));
#75455=CARTESIAN_POINT('Ctrl Pts',(38.7168453967856,1.78943621037806,2.68030513402632));
#75456=CARTESIAN_POINT('Ctrl Pts',(37.4669394326166,1.78943621037803,2.68030513402633));
#75457=CARTESIAN_POINT('Ctrl Pts',(37.4730898879459,1.70631869509735,2.73579638749286));
#75458=CARTESIAN_POINT('Ctrl Pts',(37.4792403432753,1.62062842594005,2.78741050688953));
#75459=CARTESIAN_POINT('Ctrl Pts',(37.4853907986046,1.53276716638739,2.83491487987643));
#75460=CARTESIAN_POINT('Ctrl Pts',(37.491547626715,1.44481486957995,2.88246847441704));
#75461=CARTESIAN_POINT('Ctrl Pts',(37.4977044548254,1.35468747199566,2.92590360943848));
#75462=CARTESIAN_POINT('Ctrl Pts',(37.5038612829358,1.26281076315955,2.96503398613716));
#75463=CARTESIAN_POINT('Ctrl Pts',(37.5100212215073,1.17088763773931,3.00418413170266));
#75464=CARTESIAN_POINT('Ctrl Pts',(37.5161811600788,1.07721384803234,3.03902503514212));
#75465=CARTESIAN_POINT('Ctrl Pts',(37.5223410986503,0.982232556778373,3.06941961401575));
#75466=CARTESIAN_POINT('Ctrl Pts',(37.5285117579066,0.887085961198498,3.09986709125817));
#75467=CARTESIAN_POINT('Ctrl Pts',(37.534682417163,0.790627737122123,3.12585266730446));
#75468=CARTESIAN_POINT('Ctrl Pts',(37.5408530764194,0.693313810752102,3.14728986944647));
#75469=CARTESIAN_POINT('Ctrl Pts',(37.5469067490666,0.597844813067353,3.16832065381625));
#75470=CARTESIAN_POINT('Ctrl Pts',(37.5529604217139,0.501552670685782,3.18497403493035));
#75471=CARTESIAN_POINT('Ctrl Pts',(37.5590140943611,0.40487158721871,3.19721700238864));
#75472=CARTESIAN_POINT('Ctrl Pts',(37.5651863424538,0.306296776882969,3.20969977721769));
#75473=CARTESIAN_POINT('Ctrl Pts',(37.5713585905466,0.206970630375115,3.21764144642235));
#75474=CARTESIAN_POINT('Ctrl Pts',(37.5775308386393,0.107347675039233,3.22096166372152));
#75475=CARTESIAN_POINT('Ctrl Pts',(37.583694727292,0.00785964495559124,
3.2242773842543));
#75476=CARTESIAN_POINT('Ctrl Pts',(37.5898586159446,-0.0919239646534392,
3.22298407920088));
#75477=CARTESIAN_POINT('Ctrl Pts',(37.5960225045972,-0.191541477122879,
3.21705290989153));
#75478=CARTESIAN_POINT('Ctrl Pts',(37.6021798662558,-0.291053503761449,
3.21112802114779));
#75479=CARTESIAN_POINT('Ctrl Pts',(37.6083372279143,-0.390399351713373,
3.20057505750116));
#75480=CARTESIAN_POINT('Ctrl Pts',(37.6144945895728,-0.489116269441735,
3.18541721560417));
#75481=CARTESIAN_POINT('Ctrl Pts',(37.6206474537191,-0.587761081523434,
3.17027044542636));
#75482=CARTESIAN_POINT('Ctrl Pts',(37.6268003178654,-0.68577744867549,3.15052555000574));
#75483=CARTESIAN_POINT('Ctrl Pts',(37.6329531820117,-0.7827075932881,3.12625756870881));
#75484=CARTESIAN_POINT('Ctrl Pts',(37.6391037151483,-0.87960101595968,3.10199878132552));
#75485=CARTESIAN_POINT('Ctrl Pts',(37.6452542482848,-0.975408612867861,
3.07322041829767));
#75486=CARTESIAN_POINT('Ctrl Pts',(37.6514047814213,-1.06968353440715,3.04004846979752));
#75487=CARTESIAN_POINT('Ctrl Pts',(37.6575546296365,-1.16394795752231,3.00688021531459));
#75488=CARTESIAN_POINT('Ctrl Pts',(37.6637044778517,-1.25667963485141,2.96931949227251));
#75489=CARTESIAN_POINT('Ctrl Pts',(37.6698543260669,-1.34744856459123,2.92754161853953));
#75490=CARTESIAN_POINT('Ctrl Pts',(37.676005134446,-1.43823166590896,2.88575722210771));
#75491=CARTESIAN_POINT('Ctrl Pts',(37.6821559428252,-1.5270510163454,2.83975454883317));
#75492=CARTESIAN_POINT('Ctrl Pts',(37.6883067512043,-1.61349914248706,2.78975591758375));
#75493=CARTESIAN_POINT('Ctrl Pts',(37.6944641375705,-1.70003972064795,2.73970381525722));
#75494=CARTESIAN_POINT('Ctrl Pts',(37.7006215239367,-1.78420363382053,2.68564743915454));
#75495=CARTESIAN_POINT('Ctrl Pts',(37.7067789103029,-1.86561056846591,2.62785364305707));
#75496=CARTESIAN_POINT('Ctrl Pts',(37.7129397330398,-1.9470629354412,2.57002759286696));
#75497=CARTESIAN_POINT('Ctrl Pts',(37.7191005557767,-2.02575491758814,2.50846023648324));
#75498=CARTESIAN_POINT('Ctrl Pts',(37.7252613785137,-2.10133926486082,2.44345878959605));
#75499=CARTESIAN_POINT('Ctrl Pts',(37.7314325014303,-2.1770499803795,2.37834866784261));
#75500=CARTESIAN_POINT('Ctrl Pts',(37.737603624347,-2.24964236701193,2.30979328569732));
#75501=CARTESIAN_POINT('Ctrl Pts',(37.7437747472637,-2.31880592433699,2.23813686975566));
#75502=CARTESIAN_POINT('Ctrl Pts',(37.7484702692093,-2.37143151706016,2.18361449544191));
#75503=CARTESIAN_POINT('Ctrl Pts',(37.753165791155,-2.42207275915576,2.12729755105307));
#75504=CARTESIAN_POINT('Ctrl Pts',(37.7578613131006,-2.47060923006076,2.06934955839718));
#75505=CARTESIAN_POINT('Ctrl Pts',(37.7639979307526,-2.53404195757667,1.99361683288795));
#75506=CARTESIAN_POINT('Ctrl Pts',(37.7701345484046,-2.59410897624073,1.91482168154805));
#75507=CARTESIAN_POINT('Ctrl Pts',(37.7762711660567,-2.65049770048539,1.83329743964848));
#75508=CARTESIAN_POINT('Ctrl Pts',(37.7823999093046,-2.70681406767217,1.75187780827821));
#75509=CARTESIAN_POINT('Ctrl Pts',(37.7885286525526,-2.75946126721234,1.66773639906458));
#75510=CARTESIAN_POINT('Ctrl Pts',(37.7946573958006,-2.80816578952707,1.58124079792731));
#75511=CARTESIAN_POINT('Ctrl Pts',(37.8007799602126,-2.8568212092377,1.49483239935476));
#75512=CARTESIAN_POINT('Ctrl Pts',(37.8069025246246,-2.90154163422463,1.40607490455059));
#75513=CARTESIAN_POINT('Ctrl Pts',(37.8130250890366,-2.94209648297818,1.31536529046019));
#75514=CARTESIAN_POINT('Ctrl Pts',(37.8191431641036,-2.98262159505624,1.22472218882001));
#75515=CARTESIAN_POINT('Ctrl Pts',(37.8252612391705,-3.01898702253225,1.13213021254061));
#75516=CARTESIAN_POINT('Ctrl Pts',(37.8313793142374,-3.05100834218173,1.03801043272093));
#75517=CARTESIAN_POINT('Ctrl Pts',(37.8374955154327,-3.08301985419687,0.943919480332296));
#75518=CARTESIAN_POINT('Ctrl Pts',(37.843611716628,-3.11068975499154,0.848302067816363));
#75519=CARTESIAN_POINT('Ctrl Pts',(37.8497279178233,-3.13388228014506,0.75159790891994));
#75520=CARTESIAN_POINT('Ctrl Pts',(37.8558429582643,-3.1570704037392,0.654912102880492));
#75521=CARTESIAN_POINT('Ctrl Pts',(37.8619579987053,-3.17578274326909,0.557140389035435));
#75522=CARTESIAN_POINT('Ctrl Pts',(37.8680730391463,-3.18993413181391,0.458734996690495));
#75523=CARTESIAN_POINT('Ctrl Pts',(37.8741906184604,-3.20409139580304,0.360288747902387));
#75524=CARTESIAN_POINT('Ctrl Pts',(37.8803081977745,-3.21368386707593,0.261208730973718));
#75525=CARTESIAN_POINT('Ctrl Pts',(37.8864257770886,-3.21867805973883,0.161954037479339));
#75526=CARTESIAN_POINT('Ctrl Pts',(37.8898083344834,-3.2214394695148,0.107073719593024));
#75527=CARTESIAN_POINT('Ctrl Pts',(37.8931908918782,-3.22279599229166,0.0521400722480563));
#75528=CARTESIAN_POINT('Ctrl Pts',(37.8965734492731,-3.22274881024296,-0.0027692196713569));
#75529=CARTESIAN_POINT('',(37.6500265507268,-3.22274952462855,0.00175043035796299));
#75530=CARTESIAN_POINT('Ctrl Pts',(37.2205445093424,1.78943610171065,2.68030520657528));
#75531=CARTESIAN_POINT('Ctrl Pts',(37.2224802418693,1.76062823012852,2.69953803323102));
#75532=CARTESIAN_POINT('Ctrl Pts',(37.2244175279826,1.73150014886572,2.71831319089206));
#75533=CARTESIAN_POINT('Ctrl Pts',(37.2384264205786,1.51921349350945,2.85034643710809));
#75534=CARTESIAN_POINT('Ctrl Pts',(37.2506793919992,1.32545670170221,2.94544219845531));
#75535=CARTESIAN_POINT('Ctrl Pts',(37.2647609238842,1.10688342938587,3.02675533842266));
#75536=CARTESIAN_POINT('Ctrl Pts',(37.2658477158002,1.09003339531374,3.03286431974323));
#75537=CARTESIAN_POINT('Ctrl Pts',(37.2674972111626,1.06449314932949,3.04188360462719));
#75538=CARTESIAN_POINT('Ctrl Pts',(37.2680564562156,1.0558398564875,3.04489798249388));
#75539=CARTESIAN_POINT('Ctrl Pts',(37.2690306457383,1.04077698163362,3.05007321025528));
#75540=CARTESIAN_POINT('Ctrl Pts',(37.2694450302053,1.03437320372013,3.05225087234579));
#75541=CARTESIAN_POINT('Ctrl Pts',(37.2703015797915,1.02114369817172,3.05670326905425));
#75542=CARTESIAN_POINT('Ctrl Pts',(37.2707438303974,1.01431711874152,3.05897533639165));
#75543=CARTESIAN_POINT('Ctrl Pts',(37.2717805726071,0.998323800657221,3.06423891524433));
#75544=CARTESIAN_POINT('Ctrl Pts',(37.2723756628899,0.989151167606897,3.06721217150673));
#75545=CARTESIAN_POINT('Ctrl Pts',(37.2736387725998,0.969698526896517,3.07342129844191));
#75546=CARTESIAN_POINT('Ctrl Pts',(37.2743071240318,0.959415373500202,3.07664685125373));
#75547=CARTESIAN_POINT('Ctrl Pts',(37.276111827541,0.931676248972311,3.08519528912247));
#75548=CARTESIAN_POINT('Ctrl Pts',(37.2772513277758,0.914191124048758,3.09042152003924));
#75549=CARTESIAN_POINT('Ctrl Pts',(37.2863239427167,0.77522387491839,3.13067569978891));
#75550=CARTESIAN_POINT('Ctrl Pts',(37.2944837783438,0.651835218281041,3.15867160826862));
#75551=CARTESIAN_POINT('Ctrl Pts',(37.3181729803099,0.297772103565216,3.21737505629345));
#75552=CARTESIAN_POINT('Ctrl Pts',(37.3341202738711,0.0649749300655654,
3.23046947168723));
#75553=CARTESIAN_POINT('Ctrl Pts',(37.3519510734052,-0.201284597353794,
3.21663938647263));
#75554=CARTESIAN_POINT('Ctrl Pts',(37.3542244585613,-0.235368656332999,
3.21432514663897));
#75555=CARTESIAN_POINT('Ctrl Pts',(37.3617845294849,-0.349358402603648,
3.2047625414042));
#75556=CARTESIAN_POINT('Ctrl Pts',(37.3669985083002,-0.429036130022836,
3.19507193941178));
#75557=CARTESIAN_POINT('Ctrl Pts',(37.372749432629,-0.519066802190178,3.18069279046842));
#75558=CARTESIAN_POINT('Ctrl Pts',(37.3734358475626,-0.529848876295111,
3.17891446076409));
#75559=CARTESIAN_POINT('Ctrl Pts',(37.3744454834247,-0.545765125500566,
3.17620610307979));
#75560=CARTESIAN_POINT('Ctrl Pts',(37.3747710479647,-0.55090628356377,3.17531841696218));
#75561=CARTESIAN_POINT('Ctrl Pts',(37.3753471425832,-0.560019848654505,
3.17372204411346));
#75562=CARTESIAN_POINT('Ctrl Pts',(37.375597956577,-0.563993095990223,3.17301837885143));
#75563=CARTESIAN_POINT('Ctrl Pts',(37.3761309004313,-0.572447472313028,
3.17150472013617));
#75564=CARTESIAN_POINT('Ctrl Pts',(37.3764129120629,-0.576928194224971,
3.1706926936749));
#75565=CARTESIAN_POINT('Ctrl Pts',(37.3771746633321,-0.589049673858524,
3.1684694122481));
#75566=CARTESIAN_POINT('Ctrl Pts',(37.3776533753126,-0.596687133366817,
3.16704000644736));
#75567=CARTESIAN_POINT('Ctrl Pts',(37.3800297551351,-0.634694316697665,
3.15978431927256));
#75568=CARTESIAN_POINT('Ctrl Pts',(37.3819049479015,-0.664985483264241,
3.15354852399911));
#75569=CARTESIAN_POINT('Ctrl Pts',(37.3871580840239,-0.750508238316349,
3.13465550720659));
#75570=CARTESIAN_POINT('Ctrl Pts',(37.3904872358269,-0.80550446203134,3.1209759854939));
#75571=CARTESIAN_POINT('Ctrl Pts',(37.4033504534745,-1.01951930941039,3.06170811072668));
#75572=CARTESIAN_POINT('Ctrl Pts',(37.4125221773342,-1.17529979136804,3.00535422246439));
#75573=CARTESIAN_POINT('Ctrl Pts',(37.4349834602705,-1.54137475376134,2.84008520820448));
#75574=CARTESIAN_POINT('Ctrl Pts',(37.4483321848952,-1.74530262894262,2.71952509482192));
#75575=CARTESIAN_POINT('Ctrl Pts',(37.4637830694739,-1.94994091559425,2.56597633369436));
#75576=CARTESIAN_POINT('Ctrl Pts',(37.4649759369321,-1.96555858143066,2.55403280242161));
#75577=CARTESIAN_POINT('Ctrl Pts',(37.4667398217267,-1.98838112619948,2.5362460604074));
#75578=CARTESIAN_POINT('Ctrl Pts',(37.4673064511329,-1.99567182320074,2.53051329836606));
#75579=CARTESIAN_POINT('Ctrl Pts',(37.4683181876895,-2.00861644488968,2.52024405271185));
#75580=CARTESIAN_POINT('Ctrl Pts',(37.4687628029808,-2.01428002359491,2.51571979622008));
#75581=CARTESIAN_POINT('Ctrl Pts',(37.4692132547213,-2.01999251602909,2.51112480862423));
#75582=CARTESIAN_POINT('Ctrl Pts',(37.4692183221494,-2.02005677636714,2.51107311513518));
#75583=CARTESIAN_POINT('Ctrl Pts',(37.4692282303718,-2.02018241673396,2.5109720372448));
#75584=CARTESIAN_POINT('Ctrl Pts',(37.4692330711804,-2.02024379722798,2.51092265282469));
#75585=CARTESIAN_POINT('Ctrl Pts',(37.4692425379801,-2.02036382857398,2.51082607290054));
#75586=CARTESIAN_POINT('Ctrl Pts',(37.4692471639705,-2.02042247967589,2.5107788775174));
#75587=CARTESIAN_POINT('Ctrl Pts',(37.4692562121854,-2.02053719311496,2.5106865632567));
#75588=CARTESIAN_POINT('Ctrl Pts',(37.4692606344171,-2.02059325577748,2.5106414444092));
#75589=CARTESIAN_POINT('Ctrl Pts',(37.4692692855023,-2.02070292471747,2.51055317754345));
#75590=CARTESIAN_POINT('Ctrl Pts',(37.4692735143618,-2.02075653128325,2.51051002955799));
#75591=CARTESIAN_POINT('Ctrl Pts',(37.4692817884481,-2.02086141219338,2.51042560525908));
#75592=CARTESIAN_POINT('Ctrl Pts',(37.4692858336875,-2.02091268688959,2.51038432890291));
#75593=CARTESIAN_POINT('Ctrl Pts',(37.4692937497061,-2.02101302089148,2.5103035545236));
#75594=CARTESIAN_POINT('Ctrl Pts',(37.4692976204973,-2.02106208052516,2.51026405645501));
#75595=CARTESIAN_POINT('Ctrl Pts',(37.4693051962382,-2.02115809415445,2.51018675093464));
#75596=CARTESIAN_POINT('Ctrl Pts',(37.4693089012057,-2.02120504853464,2.51014894337206));
#75597=CARTESIAN_POINT('Ctrl Pts',(37.4693161534218,-2.02129695506833,2.51007493618464));
#75598=CARTESIAN_POINT('Ctrl Pts',(37.4693197006877,-2.02134190758624,2.51003873644738));
#75599=CARTESIAN_POINT('Ctrl Pts',(37.4693266451485,-2.02142990773995,2.50996786705512));
#75600=CARTESIAN_POINT('Ctrl Pts',(37.4693300423638,-2.02147295576501,2.50993319725155));
#75601=CARTESIAN_POINT('Ctrl Pts',(37.4693366939325,-2.021557238675,2.5098653143274));
#75602=CARTESIAN_POINT('Ctrl Pts',(37.4693399483097,-2.0215984739818,2.5098321010174));
#75603=CARTESIAN_POINT('Ctrl Pts',(37.4693463209997,-2.02167921793681,2.50976706186766));
#75604=CARTESIAN_POINT('Ctrl Pts',(37.4693494393407,-2.0217187270525,2.50973523578854));
#75605=CARTESIAN_POINT('Ctrl Pts',(37.4693555463853,-2.02179610037984,2.50967290564978));
#75606=CARTESIAN_POINT('Ctrl Pts',(37.469358535115,-2.02183396502238,2.50964240136828));
#75607=CARTESIAN_POINT('Ctrl Pts',(37.4693643889991,-2.02190812650292,2.50958265308271));
#75608=CARTESIAN_POINT('Ctrl Pts',(37.4693672541842,-2.02194442382091,2.50955340880635));
#75609=CARTESIAN_POINT('Ctrl Pts',(37.4693728667073,-2.02201552348668,2.50949612218786));
#75610=CARTESIAN_POINT('Ctrl Pts',(37.4693756140804,-2.02205032636458,2.50946807952319));
#75611=CARTESIAN_POINT('Ctrl Pts',(37.4693809964028,-2.02211850609953,2.50941314088107));
#75612=CARTESIAN_POINT('Ctrl Pts',(37.4693836313867,-2.02215188347209,2.50938624458392));
#75613=CARTESIAN_POINT('Ctrl Pts',(37.4693887940676,-2.02221727749147,2.50933354634355));
#75614=CARTESIAN_POINT('Ctrl Pts',(37.4693913217974,-2.02224929462391,2.5093077440966));
#75615=CARTESIAN_POINT('Ctrl Pts',(37.4693962748219,-2.02231202982677,2.5092571845217));
#75616=CARTESIAN_POINT('Ctrl Pts',(37.4693987001561,-2.02234274846107,2.50923242681953));
#75617=CARTESIAN_POINT('Ctrl Pts',(37.4694038885212,-2.02240846131369,2.50917946351515));
#75618=CARTESIAN_POINT('Ctrl Pts',(37.4694066516036,-2.02244345596416,2.5091512572877));
#75619=CARTESIAN_POINT('Ctrl Pts',(37.4694121526349,-2.02251312502412,2.50909510054678));
#75620=CARTESIAN_POINT('Ctrl Pts',(37.4694148901303,-2.02254779370764,2.50906715467144));
#75621=CARTESIAN_POINT('Ctrl Pts',(37.4694203397855,-2.02261680832958,2.50901152072062));
#75622=CARTESIAN_POINT('Ctrl Pts',(37.4694230519556,-2.02265115441582,2.50898383254784));
#75623=CARTESIAN_POINT('Ctrl Pts',(37.469428451374,-2.02271952913357,2.50892870980267));
#75624=CARTESIAN_POINT('Ctrl Pts',(37.4694311386296,-2.02275355787464,2.50890127516327));
#75625=CARTESIAN_POINT('Ctrl Pts',(37.469436488617,-2.02282130299522,2.50884665544236));
#75626=CARTESIAN_POINT('Ctrl Pts',(37.4694391513584,-2.02285501951226,2.50881947027076));
#75627=CARTESIAN_POINT('Ctrl Pts',(37.469444452708,-2.02292214517852,2.50876534552119));
#75628=CARTESIAN_POINT('Ctrl Pts',(37.4694470913267,-2.02295555447622,2.50873840584376));
#75629=CARTESIAN_POINT('Ctrl Pts',(37.469952018084,-2.0293485980074,2.50358314718528));
#75630=CARTESIAN_POINT('Ctrl Pts',(37.4704552800458,-2.03568866190087,2.49843070285088));
#75631=CARTESIAN_POINT('Ctrl Pts',(37.4718285307259,-2.0529015338585,2.48433312741732));
#75632=CARTESIAN_POINT('Ctrl Pts',(37.4727004337053,-2.06373532776098,2.47534084168917));
#75633=CARTESIAN_POINT('Ctrl Pts',(37.4746403731667,-2.08762805515924,2.45524347402416));
#75634=CARTESIAN_POINT('Ctrl Pts',(37.47570978232,-2.10065793828163,2.44410466662851));
#75635=CARTESIAN_POINT('Ctrl Pts',(37.4789689293492,-2.13993726725661,2.40997996257231));
#75636=CARTESIAN_POINT('Ctrl Pts',(37.4811719476923,-2.16590218476488,2.38667184598604));
#75637=CARTESIAN_POINT('Ctrl Pts',(37.4893402062464,-2.2600127153569,2.29939034352748));
#75638=CARTESIAN_POINT('Ctrl Pts',(37.4954097320415,-2.32573944324816,2.23288754040933));
#75639=CARTESIAN_POINT('Ctrl Pts',(37.5158149635961,-2.53331939408569,2.00373520968703));
#75640=CARTESIAN_POINT('Ctrl Pts',(37.53056655816,-2.66173139669831,1.82970878571906));
#75641=CARTESIAN_POINT('Ctrl Pts',(37.5494371625395,-2.80506226468721,1.58808011082096));
#75642=CARTESIAN_POINT('Ctrl Pts',(37.5537863979906,-2.83663282956752,1.53097607877595));
#75643=CARTESIAN_POINT('Ctrl Pts',(37.5624805230061,-2.89712487501739,1.4132549517848));
#75644=CARTESIAN_POINT('Ctrl Pts',(37.5668196693968,-2.92593040517308,1.35261039452751));
#75645=CARTESIAN_POINT('Ctrl Pts',(37.5717096171271,-2.95700568357344,1.28153967994256));
#75646=CARTESIAN_POINT('Ctrl Pts',(37.5723651612951,-2.96114189045629,1.27195333075637));
#75647=CARTESIAN_POINT('Ctrl Pts',(37.5733380984812,-2.96723738164278,1.25763512506905));
#75648=CARTESIAN_POINT('Ctrl Pts',(37.5736575989741,-2.96923204169334,1.25291854095699));
#75649=CARTESIAN_POINT('Ctrl Pts',(37.5742269959283,-2.97277441280395,1.24448626120758));
#75650=CARTESIAN_POINT('Ctrl Pts',(37.5744771519168,-2.97432640799353,1.24077241389976));
#75651=CARTESIAN_POINT('Ctrl Pts',(37.575013145255,-2.97764257128531,1.2327950233224));
#75652=CARTESIAN_POINT('Ctrl Pts',(37.5752988475505,-2.97940453591041,1.22853061170287));
#75653=CARTESIAN_POINT('Ctrl Pts',(37.5760809870765,-2.98421229836944,1.21682340220248));
#75654=CARTESIAN_POINT('Ctrl Pts',(37.5765763006831,-2.98723943096725,1.20937290329058));
#75655=CARTESIAN_POINT('Ctrl Pts',(37.5791778911401,-3.00304407218191,1.17005248170601));
#75656=CARTESIAN_POINT('Ctrl Pts',(37.5812562671334,-3.01534011683228,1.13798976877865));
#75657=CARTESIAN_POINT('Ctrl Pts',(37.5872467707994,-3.04970386362609,1.04391366794094));
#75658=CARTESIAN_POINT('Ctrl Pts',(37.5910920291017,-3.07038817643195,0.981410716644376));
#75659=CARTESIAN_POINT('Ctrl Pts',(37.612746686303,-3.17759684509134,0.620768231487759));
#75660=CARTESIAN_POINT('Ctrl Pts',(37.6294005054505,-3.22259519032419,0.312020770992711));
#75661=CARTESIAN_POINT('Ctrl Pts',(37.6474995143151,-3.22274960128745,0.00160309126306275));
#75662=CARTESIAN_POINT('Ctrl Pts',(37.6500265507268,-3.22274952462855,0.00175043035796299));
#75663=CARTESIAN_POINT('Ctrl Pts',(37.6562525068647,-3.22280455179977,-0.0995611065815355));
#75664=CARTESIAN_POINT('Ctrl Pts',(37.6624784630026,-3.21807793497928,-0.200873595969597));
#75665=CARTESIAN_POINT('Ctrl Pts',(37.6687044191406,-3.20859589316742,-0.301711711488305));
#75666=CARTESIAN_POINT('Ctrl Pts',(37.6749320374216,-3.19911131993544,-0.402576747752343));
#75667=CARTESIAN_POINT('Ctrl Pts',(37.6811596557026,-3.18486883519379,-0.502966740616681));
#75668=CARTESIAN_POINT('Ctrl Pts',(37.6873872739837,-3.16594645797127,-0.602412307111318));
#75669=CARTESIAN_POINT('Ctrl Pts',(37.6936180596769,-3.14701445668942,-0.701908452347799));
#75670=CARTESIAN_POINT('Ctrl Pts',(37.6998488453701,-3.12339790591718,-0.800458803920177));
#75671=CARTESIAN_POINT('Ctrl Pts',(37.7060796310633,-3.09522558791562,-0.897605772270008));
#75672=CARTESIAN_POINT('Ctrl Pts',(37.7123194068227,-3.06701262158846,-0.994892908766438));
#75673=CARTESIAN_POINT('Ctrl Pts',(37.7185591825822,-3.03423088150391,-1.09077221623046));
#75674=CARTESIAN_POINT('Ctrl Pts',(37.7247989583417,-2.99705858694311,-1.18480267932284));
#75675=CARTESIAN_POINT('Ctrl Pts',(37.7310438467765,-2.95985583457685,-1.27891018801024));
#75676=CARTESIAN_POINT('Ctrl Pts',(37.7372887352114,-2.91825553415589,-1.37116545338473));
#75677=CARTESIAN_POINT('Ctrl Pts',(37.7435336236463,-2.87248259932717,-1.46115066952817));
#75678=CARTESIAN_POINT('Ctrl Pts',(37.7497896545153,-2.82662799419841,-1.55129644167768));
#75679=CARTESIAN_POINT('Ctrl Pts',(37.7560456853843,-2.77658609542278,-1.63916371321967));
#75680=CARTESIAN_POINT('Ctrl Pts',(37.7623017162533,-2.72262606332809,-1.72436216665369));
#75681=CARTESIAN_POINT('Ctrl Pts',(37.7649444456067,-2.69983177670908,-1.76035247080442));
#75682=CARTESIAN_POINT('Ctrl Pts',(37.7675871749601,-2.67633881719068,-1.79586692679338));
#75683=CARTESIAN_POINT('Ctrl Pts',(37.7702299043134,-2.65216960257468,-1.8308779210201));
#75684=CARTESIAN_POINT('Ctrl Pts',(37.7764021524062,-2.59572099627804,-1.91264813410139));
#75685=CARTESIAN_POINT('Ctrl Pts',(37.782574400499,-2.5353878507564,-1.99194923775924));
#75686=CARTESIAN_POINT('Ctrl Pts',(37.7887466485917,-2.47141347119128,-2.06838899071579));
#75687=CARTESIAN_POINT('Ctrl Pts',(37.7949105372444,-2.40752573590673,-2.14472521680037));
#75688=CARTESIAN_POINT('Ctrl Pts',(37.801074425897,-2.34000684488508,-2.21820746458734));
#75689=CARTESIAN_POINT('Ctrl Pts',(37.8072383145497,-2.26914324819176,-2.2884725215055));
#75690=CARTESIAN_POINT('Ctrl Pts',(37.8133956762082,-2.1983546895634,-2.35866317415756));
#75691=CARTESIAN_POINT('Ctrl Pts',(37.8195530378668,-2.12422877332027,-2.42564310464567));
#75692=CARTESIAN_POINT('Ctrl Pts',(37.8257103995253,-2.04709143595346,-2.48908300692163));
#75693=CARTESIAN_POINT('Ctrl Pts',(37.8318632636716,-1.97001044189372,-2.55247657088702));
#75694=CARTESIAN_POINT('Ctrl Pts',(37.8380161278179,-1.88992273442372,-2.612334972445));
#75695=CARTESIAN_POINT('Ctrl Pts',(37.8441689919642,-1.80718955842861,-2.66836719032569));
#75696=CARTESIAN_POINT('Ctrl Pts',(37.8503195251008,-1.72448772585939,-2.72437818042625));
#75697=CARTESIAN_POINT('Ctrl Pts',(37.8564700582373,-1.63914277545373,-2.77656562378353));
#75698=CARTESIAN_POINT('Ctrl Pts',(37.8626205913738,-1.55154662461723,-2.82468062515727));
#75699=CARTESIAN_POINT('Ctrl Pts',(37.868770439589,-1.46396022845918,-2.87279026846034));
#75700=CARTESIAN_POINT('Ctrl Pts',(37.8749202878042,-1.37412351100675,-2.91682816229175));
#75701=CARTESIAN_POINT('Ctrl Pts',(37.8810701360194,-1.28245390438678,-2.95659086544336));
#75702=CARTESIAN_POINT('Ctrl Pts',(37.8872209443986,-1.19076998556788,-2.99635977666914));
#75703=CARTESIAN_POINT('Ctrl Pts',(37.8933717527777,-1.09725300772172,-3.03185199856225));
#75704=CARTESIAN_POINT('Ctrl Pts',(37.8995225611569,-1.00234039523467,-3.06291222443295));
#75705=CARTESIAN_POINT('Ctrl Pts',(37.905679947523,-0.907326278376747,-3.09400566768756));
#75706=CARTESIAN_POINT('Ctrl Pts',(37.9118373338892,-0.810913960021141,
-3.12065751466234));
#75707=CARTESIAN_POINT('Ctrl Pts',(37.9179947202554,-0.713555930245918,
-3.14276239905451));
#75708=CARTESIAN_POINT('Ctrl Pts',(37.9241555429924,-0.616143566006662,
-3.16487961994373));
#75709=CARTESIAN_POINT('Ctrl Pts',(37.9303163657293,-0.517784866882843,
-3.18244474826779));
#75710=CARTESIAN_POINT('Ctrl Pts',(37.9364771884663,-0.418940341809283,
-3.195403973288));
#75711=CARTESIAN_POINT('Ctrl Pts',(37.942648311383,-0.319930560175463,-3.20838486462658));
#75712=CARTESIAN_POINT('Ctrl Pts',(37.9488194342997,-0.220433763210126,
-3.21674443469551));
#75713=CARTESIAN_POINT('Ctrl Pts',(37.9549905572163,-0.120913523366501,
-3.22048093960624));
#75714=CARTESIAN_POINT('Ctrl Pts',(37.9596860791619,-0.0451899514139525,
-3.22332399443513));
#75715=CARTESIAN_POINT('Ctrl Pts',(37.9643816011074,0.0305471301858255,
-3.22349161534475));
#75716=CARTESIAN_POINT('Ctrl Pts',(37.9690771230529,0.1060955676368,-3.22100315011144));
#75717=CARTESIAN_POINT('Ctrl Pts',(37.9752493711457,0.205403739204771,-3.21773207077918));
#75718=CARTESIAN_POINT('Ctrl Pts',(37.9814216192384,0.304735284049323,-3.20985820967658));
#75719=CARTESIAN_POINT('Ctrl Pts',(37.9875938673312,0.403628687708124,-3.19737414841601));
#75720=CARTESIAN_POINT('Ctrl Pts',(37.9937577559838,0.50238815418949,-3.18490699505694));
#75721=CARTESIAN_POINT('Ctrl Pts',(37.9999216446364,0.600710231773359,-3.16784210583526));
#75722=CARTESIAN_POINT('Ctrl Pts',(38.0060855332891,0.698134496323708,-3.1462240523432));
#75723=CARTESIAN_POINT('Ctrl Pts',(38.0122428949476,0.795455597492531,-3.12462889039166));
#75724=CARTESIAN_POINT('Ctrl Pts',(38.0184002566062,0.891880353990418,-3.09849024311563));
#75725=CARTESIAN_POINT('Ctrl Pts',(38.0245576182647,0.986955513436086,-3.06790423204475));
#75726=CARTESIAN_POINT('Ctrl Pts',(38.030710482411,1.08196122727859,-3.03734056186712));
#75727=CARTESIAN_POINT('Ctrl Pts',(38.0368633465573,1.17561889171836,-3.00233611905558));
#75728=CARTESIAN_POINT('Ctrl Pts',(38.0430162107036,1.2674883682607,-2.96303742784728));
#75729=CARTESIAN_POINT('Ctrl Pts',(38.0491667438402,1.3593230400939,-2.92375362493015));
#75730=CARTESIAN_POINT('Ctrl Pts',(38.0553172769767,1.44937047120064,-2.88017897685373));
#75731=CARTESIAN_POINT('Ctrl Pts',(38.0614678101132,1.53720937493199,-2.83250858782833));
#75732=CARTESIAN_POINT('Ctrl Pts',(38.0676176583285,1.62503849695214,-2.78484350736164));
#75733=CARTESIAN_POINT('Ctrl Pts',(38.0737675065437,1.71065919878597,-2.73308379993163));
#75734=CARTESIAN_POINT('Ctrl Pts',(38.0799173547589,1.79367463405055,-2.67747061042015));
#75735=CARTESIAN_POINT('Ctrl Pts',(38.086068163138,1.87670303035475,-2.62184873812875));
#75736=CARTESIAN_POINT('Ctrl Pts',(38.0922189715171,1.95712499125445,-2.56237243053142));
#75737=CARTESIAN_POINT('Ctrl Pts',(38.0983697798963,2.03457335153321,-2.49932567700389));
#75738=CARTESIAN_POINT('Ctrl Pts',(38.1045271662624,2.11210453902418,-2.43621149807425));
#75739=CARTESIAN_POINT('Ctrl Pts',(38.1106845526286,2.18665543799785,-2.36951952299409));
#75740=CARTESIAN_POINT('Ctrl Pts',(38.1168419389948,2.25789274736271,-2.29957341781185));
#75741=CARTESIAN_POINT('Ctrl Pts',(38.1230027617318,2.32916981349981,-2.22958827646447));
#75742=CARTESIAN_POINT('Ctrl Pts',(38.1291635844687,2.39712931175495,-2.15634570671666));
#75743=CARTESIAN_POINT('Ctrl Pts',(38.1353244072057,2.46147697415873,-2.08020399677204));
#75744=CARTESIAN_POINT('Ctrl Pts',(38.1414955301223,2.52593221837693,-2.00393498673598));
#75745=CARTESIAN_POINT('Ctrl Pts',(38.147666653039,2.58676330012441,-1.92475749933256));
#75746=CARTESIAN_POINT('Ctrl Pts',(38.1538377759557,2.64371809405453,-1.84306055290343));
#75747=CARTESIAN_POINT('Ctrl Pts',(38.1585332979013,2.68705420782473,-1.78089847802216));
#75748=CARTESIAN_POINT('Ctrl Pts',(38.163228819847,2.72814702753737,-1.7172784041907));
#75749=CARTESIAN_POINT('Ctrl Pts',(38.1679243417926,2.76690352208694,-1.65238084652507));
#75750=CARTESIAN_POINT('Ctrl Pts',(38.1740965898854,2.81784880619728,-1.56707322126721));
#75751=CARTESIAN_POINT('Ctrl Pts',(38.1802688379781,2.86493482742254,-1.47925716296869));
#75752=CARTESIAN_POINT('Ctrl Pts',(38.1864410860709,2.9079057997536,-1.38931689051108));
#75753=CARTESIAN_POINT('Ctrl Pts',(38.1926049747235,2.95081857395892,-1.29949842947641));
#75754=CARTESIAN_POINT('Ctrl Pts',(38.1987688633762,2.98962719111635,-1.20756186102319));
#75755=CARTESIAN_POINT('Ctrl Pts',(38.2049327520288,3.02412018920187,-1.11391859835521));
#75756=CARTESIAN_POINT('Ctrl Pts',(38.2110901136874,3.05857666235845,-1.02037449533425));
#75757=CARTESIAN_POINT('Ctrl Pts',(38.2172474753459,3.08872645241741,-0.925127696404006));
#75758=CARTESIAN_POINT('Ctrl Pts',(38.2234048370044,3.11440533946282,-0.828611455403252));
#75759=CARTESIAN_POINT('Ctrl Pts',(38.2295577011507,3.14006546991815,-0.732165712612355));
#75760=CARTESIAN_POINT('Ctrl Pts',(38.2357105652971,3.16126107873318,-0.63445278976262));
#75761=CARTESIAN_POINT('Ctrl Pts',(38.2418634294434,3.17787743601157,-0.535922162434538));
#75762=CARTESIAN_POINT('Ctrl Pts',(38.2480139625799,3.1944874981906,-0.437428863389572));
#75763=CARTESIAN_POINT('Ctrl Pts',(38.2541644957165,3.20652168381173,-0.338118903262951));
#75764=CARTESIAN_POINT('Ctrl Pts',(38.260315028853,3.21391632227115,-0.238452166983385));
#75765=CARTESIAN_POINT('Ctrl Pts',(38.2664648770682,3.2213101372661,-0.138796529558336));
#75766=CARTESIAN_POINT('Ctrl Pts',(38.2726147252834,3.22406540015222,-0.0387846281554028));
#75767=CARTESIAN_POINT('Ctrl Pts',(38.2787645734986,3.22217038525106,0.0611193170038219));
#75768=CARTESIAN_POINT('Ctrl Pts',(38.2849153818778,3.22027507448489,0.161038859973051));
#75769=CARTESIAN_POINT('Ctrl Pts',(38.2910661902569,3.21372805206935,0.26084997888216));
#75770=CARTESIAN_POINT('Ctrl Pts',(38.2972169986361,3.20256968240682,0.360090255114835));
#75771=CARTESIAN_POINT('Ctrl Pts',(38.3033743850023,3.19139937941675,0.45943666394197));
#75772=CARTESIAN_POINT('Ctrl Pts',(38.3095317713685,3.17560792989481,0.558210578514013));
#75773=CARTESIAN_POINT('Ctrl Pts',(38.3156891577347,3.15528738529323,0.655956613435232));
#75774=CARTESIAN_POINT('Ctrl Pts',(38.3218499804716,3.13495550001538,0.753757199361873));
#75775=CARTESIAN_POINT('Ctrl Pts',(38.3280108032086,3.1100895940069,0.850528342502538));
#75776=CARTESIAN_POINT('Ctrl Pts',(38.3341716259455,3.08083194879438,0.945828771917954));
#75777=CARTESIAN_POINT('Ctrl Pts',(38.3403427488622,3.05152538819874,1.04128853257763));
#75778=CARTESIAN_POINT('Ctrl Pts',(38.3465138717789,3.01781256875866,1.13527225895367));
#75779=CARTESIAN_POINT('Ctrl Pts',(38.3526849946956,2.97988440941438,1.22735751475645));
#75780=CARTESIAN_POINT('Ctrl Pts',(38.3573805166412,2.9510253983464,1.29742391034098));
#75781=CARTESIAN_POINT('Ctrl Pts',(38.3620760385867,2.91972693349835,1.36639158192843));
#75782=CARTESIAN_POINT('Ctrl Pts',(38.3667715605322,2.88609056292363,1.43408466455198));
#75783=CARTESIAN_POINT('Ctrl Pts',(38.372943637077,2.84187689375485,1.52306452501239));
#75784=CARTESIAN_POINT('Ctrl Pts',(38.3791157136217,2.79346659890682,1.61015437971099));
#75785=CARTESIAN_POINT('Ctrl Pts',(38.3852877901665,2.7410445645196,1.69493134309847));
#75786=CARTESIAN_POINT('Ctrl Pts',(38.3914518381726,2.68869071987752,1.77959802996588));
#75787=CARTESIAN_POINT('Ctrl Pts',(38.3976158861788,2.63233573177939,1.86195743777999));
#75788=CARTESIAN_POINT('Ctrl Pts',(38.4037799341849,2.57221136227819,1.94160919607088));
#75789=CARTESIAN_POINT('Ctrl Pts',(38.4099367118373,2.51215790809682,2.0211670069331));
#75790=CARTESIAN_POINT('Ctrl Pts',(38.4160934894897,2.44834417686357,2.09802317649368));
#75791=CARTESIAN_POINT('Ctrl Pts',(38.4222502671421,2.38104574964331,2.17180540118252));
#75792=CARTESIAN_POINT('Ctrl Pts',(38.4284028046021,2.31379367106477,2.24553681181761));
#75793=CARTESIAN_POINT('Ctrl Pts',(38.434555342062,2.24306195790413,2.31619816520041));
#75794=CARTESIAN_POINT('Ctrl Pts',(38.440707879522,2.16916662225259,2.38344996326864));
#75795=CARTESIAN_POINT('Ctrl Pts',(38.4468582812357,2.09529693807963,2.45067841604664));
#75796=CARTESIAN_POINT('Ctrl Pts',(38.4530086829495,2.0182661329439,2.51449937172952));
#75797=CARTESIAN_POINT('Ctrl Pts',(38.4591590846632,1.93842661068593,2.57461061861491));
#75798=CARTESIAN_POINT('Ctrl Pts',(38.4629068025038,1.88977678001197,2.61123911913531));
#75799=CARTESIAN_POINT('Ctrl Pts',(38.4666545203444,1.84008476533747,2.64649093985225));
#75800=CARTESIAN_POINT('Ctrl Pts',(38.470402238185,1.78943621037805,2.68030513402632));
#75801=CARTESIAN_POINT('Origin',(-1.72497344927317,0.,0.));
#75802=CARTESIAN_POINT('',(39.9670570335907,1.78943621037801,2.68030513402635));
#75803=CARTESIAN_POINT('',(39.7209886430068,1.78943588752244,2.68030534957246));
#75804=CARTESIAN_POINT('',(-1.72497344927317,1.78943621037804,2.68030513402633));
#75805=CARTESIAN_POINT('',(39.1465734492125,-3.22274998364956,-0.000324633233694736));
#75806=CARTESIAN_POINT('Ctrl Pts',(39.1465734492731,-3.22274998364947,-0.000324634210066948));
#75807=CARTESIAN_POINT('Ctrl Pts',(39.1476462476081,-3.22274824391556,-0.0175955417198468));
#75808=CARTESIAN_POINT('Ctrl Pts',(39.1487190459431,-3.22260767174683,-0.0348656462574428));
#75809=CARTESIAN_POINT('Ctrl Pts',(39.1497918442782,-3.22232829810597,-0.0521334990721938));
#75810=CARTESIAN_POINT('Ctrl Pts',(39.1559640923709,-3.22072094715689,-0.151482526863611));
#75811=CARTESIAN_POINT('Ctrl Pts',(39.1621363404637,-3.21451185152515,-0.250932014651666));
#75812=CARTESIAN_POINT('Ctrl Pts',(39.1683085885565,-3.20368586415779,-0.350020636956677));
#75813=CARTESIAN_POINT('Ctrl Pts',(39.1744724772091,-3.19287453906453,-0.44897505768811));
#75814=CARTESIAN_POINT('Ctrl Pts',(39.1806363658617,-3.17745879738243,-0.547569156360143));
#75815=CARTESIAN_POINT('Ctrl Pts',(39.1868002545143,-3.15747549300735,-0.645341826908817));
#75816=CARTESIAN_POINT('Ctrl Pts',(39.1929576161729,-3.13751334912308,-0.743010965145803));
#75817=CARTESIAN_POINT('Ctrl Pts',(39.1991149778314,-3.11299334472704,-0.839859981307581));
#75818=CARTESIAN_POINT('Ctrl Pts',(39.20527233949,-3.08400399653836,-0.935434076691369));
#75819=CARTESIAN_POINT('Ctrl Pts',(39.2114252036363,-3.05503582299486,-1.03093836203507));
#75820=CARTESIAN_POINT('Ctrl Pts',(39.2175780677826,-3.02160492181605,-1.12516916364069));
#75821=CARTESIAN_POINT('Ctrl Pts',(39.2237309319289,-2.98385042499748,-1.21768395067947));
#75822=CARTESIAN_POINT('Ctrl Pts',(39.2298814650654,-2.9461102314528,-1.3101636885334));
#75823=CARTESIAN_POINT('Ctrl Pts',(39.236031998202,-2.90404986089225,-1.40092830185925));
#75824=CARTESIAN_POINT('Ctrl Pts',(39.2421825313385,-2.8578573342118,-1.48955329538484));
#75825=CARTESIAN_POINT('Ctrl Pts',(39.2483323795537,-2.8116699515158,-1.57816841966054));
#75826=CARTESIAN_POINT('Ctrl Pts',(39.2544822277689,-2.76135152832458,-1.66464401265235));
#75827=CARTESIAN_POINT('Ctrl Pts',(39.2606320759841,-2.70713652908706,-1.74857924481062));
#75828=CARTESIAN_POINT('Ctrl Pts',(39.2667828843632,-2.65291306536636,-1.83252758161467));
#75829=CARTESIAN_POINT('Ctrl Pts',(39.2729336927423,-2.59479205293229,-1.91393440487903));
#75830=CARTESIAN_POINT('Ctrl Pts',(39.2790845011215,-2.53305129183504,-1.99242784447339));
#75831=CARTESIAN_POINT('Ctrl Pts',(39.2852418874877,-2.47124450203038,-2.07100522894084));
#75832=CARTESIAN_POINT('Ctrl Pts',(39.2913992738538,-2.40581050236054,-2.14666266588568));
#75833=CARTESIAN_POINT('Ctrl Pts',(39.29755666022,-2.33706733115862,-2.21906148002508));
#75834=CARTESIAN_POINT('Ctrl Pts',(39.303717482957,-2.26828579513588,-2.29150069916012));
#75835=CARTESIAN_POINT('Ctrl Pts',(39.3098783056939,-2.19619172311498,-2.36067737301636));
#75836=CARTESIAN_POINT('Ctrl Pts',(39.3160391284309,-2.12113842447668,-2.42629127408656));
#75837=CARTESIAN_POINT('Ctrl Pts',(39.3222102513476,-2.04595964544425,-2.49201487397503));
#75838=CARTESIAN_POINT('Ctrl Pts',(39.3283813742643,-1.96781209748039,-2.55416353257134));
#75839=CARTESIAN_POINT('Ctrl Pts',(39.3345524971809,-1.88708052162202,-2.61247864439401));
#75840=CARTESIAN_POINT('Ctrl Pts',(39.3392480191266,-1.82565298383554,-2.65684980520591));
#75841=CARTESIAN_POINT('Ctrl Pts',(39.3439435410722,-1.76273007964743,-2.69900240601355));
#75842=CARTESIAN_POINT('Ctrl Pts',(39.3486390630179,-1.69849074071571,-2.73884040539112));
#75843=CARTESIAN_POINT('Ctrl Pts',(39.3548113111106,-1.61404834181067,-2.79120732402636));
#75844=CARTESIAN_POINT('Ctrl Pts',(39.3609835592034,-1.52703322459284,-2.83975753376277));
#75845=CARTESIAN_POINT('Ctrl Pts',(39.3671558072962,-1.4378252700014,-2.88422884935391));
#75846=CARTESIAN_POINT('Ctrl Pts',(39.3733196959488,-1.3487381350116,-2.92863993481582));
#75847=CARTESIAN_POINT('Ctrl Pts',(39.3794835846014,-1.25746445095498,-2.96898291417187));
#75848=CARTESIAN_POINT('Ctrl Pts',(39.3856474732541,-1.16441203164176,-3.00503946447762));
#75849=CARTESIAN_POINT('Ctrl Pts',(39.3918048349126,-1.07145814632625,-3.04105783419578));
#75850=CARTESIAN_POINT('Ctrl Pts',(39.3979621965712,-0.976729673163516,
-3.0727986426186));
#75851=CARTESIAN_POINT('Ctrl Pts',(39.4041195582297,-0.880657054772842,
-3.10009043648388));
#75852=CARTESIAN_POINT('Ctrl Pts',(39.410272422376,-0.784654610557619,-3.12736229564599));
#75853=CARTESIAN_POINT('Ctrl Pts',(39.4164252865223,-0.687310389687696,
-3.15019148284326));
#75854=CARTESIAN_POINT('Ctrl Pts',(39.4225781506686,-0.589071883135591,
-3.16845575620034));
#75855=CARTESIAN_POINT('Ctrl Pts',(39.4287286838052,-0.49087059419678,-3.18671311014582));
#75856=CARTESIAN_POINT('Ctrl Pts',(39.4348792169417,-0.391776119352182,
-3.20040890728105));
#75857=CARTESIAN_POINT('Ctrl Pts',(39.4410297500782,-0.292247212632413,
-3.20947178351962));
#75858=CARTESIAN_POINT('Ctrl Pts',(39.4471795982934,-0.19272938941863,-3.21853365051929));
#75859=CARTESIAN_POINT('Ctrl Pts',(39.4533294465087,-0.0927776630986046,
-3.22296358295743));
#75860=CARTESIAN_POINT('Ctrl Pts',(39.4594792947239,0.00714400760919167,
-3.22274208177683));
#75861=CARTESIAN_POINT('Ctrl Pts',(39.465630103103,0.107081278894509,-3.22252054601369));
#75862=CARTESIAN_POINT('Ctrl Pts',(39.4717809114821,0.206988050831943,-3.21764613513559));
#75863=CARTESIAN_POINT('Ctrl Pts',(39.4779317198613,0.306401293621398,-3.20815146303399));
#75864=CARTESIAN_POINT('Ctrl Pts',(39.4840891062275,0.405920853984631,-3.19864663684755));
#75865=CARTESIAN_POINT('Ctrl Pts',(39.4902464925936,0.504945397976867,-3.18451172386564));
#75866=CARTESIAN_POINT('Ctrl Pts',(39.4964038789598,0.603018062348049,-3.16583113557593));
#75867=CARTESIAN_POINT('Ctrl Pts',(39.5025647016968,0.701145460013106,-3.14714012185183));
#75868=CARTESIAN_POINT('Ctrl Pts',(39.5087255244338,0.798319497638805,-3.12389848167956));
#75869=CARTESIAN_POINT('Ctrl Pts',(39.5148863471707,0.894096583169992,-3.09624108597243));
#75870=CARTESIAN_POINT('Ctrl Pts',(39.5210574700874,0.990033796858899,-3.06853745031347));
#75871=CARTESIAN_POINT('Ctrl Pts',(39.5272285930041,1.08456898182438,-3.03640345240416));
#75872=CARTESIAN_POINT('Ctrl Pts',(39.5333997159208,1.17727656341207,-3.00002290920264));
#75873=CARTESIAN_POINT('Ctrl Pts',(39.5380952378663,1.24781647806625,-2.97234145782015));
#75874=CARTESIAN_POINT('Ctrl Pts',(39.5427907598119,1.31729868019305,-2.94220249278023));
#75875=CARTESIAN_POINT('Ctrl Pts',(39.5474862817574,1.38554562870939,-2.90970460240628));
#75876=CARTESIAN_POINT('Ctrl Pts',(39.5536585298502,1.47525601718202,-2.86698623281809));
#75877=CARTESIAN_POINT('Ctrl Pts',(39.5598307779429,1.56314685124062,-2.82003993606994));
#75878=CARTESIAN_POINT('Ctrl Pts',(39.5660030260357,1.64879217280522,-2.7690435051469));
#75879=CARTESIAN_POINT('Ctrl Pts',(39.5721669146883,1.73432149985249,-2.71811614170219));
#75880=CARTESIAN_POINT('Ctrl Pts',(39.578330803341,1.81761098924881,-2.66314976706568));
#75881=CARTESIAN_POINT('Ctrl Pts',(39.5844946919936,1.89825647668429,-2.6043693883983));
#75882=CARTESIAN_POINT('Ctrl Pts',(39.5906520536521,1.97881656792768,-2.5456512527735));
#75883=CARTESIAN_POINT('Ctrl Pts',(39.5968094153107,2.05673787429803,-2.4831273968415));
#75884=CARTESIAN_POINT('Ctrl Pts',(39.6029667769692,2.13164342305119,-2.41706720623622));
#75885=CARTESIAN_POINT('Ctrl Pts',(39.6091196411155,2.20649425865922,-2.3510552678747));
#75886=CARTESIAN_POINT('Ctrl Pts',(39.6152725052618,2.27833339138376,-2.28151241680965));
#75887=CARTESIAN_POINT('Ctrl Pts',(39.6214253694081,2.34681602731882,-2.20874898900249));
#75888=CARTESIAN_POINT('Ctrl Pts',(39.6275759025447,2.41527271863851,-2.13601312758673));
#75889=CARTESIAN_POINT('Ctrl Pts',(39.6337264356812,2.48037514247187,-2.06005942975104));
#75890=CARTESIAN_POINT('Ctrl Pts',(39.6398769688177,2.54181521371162,-1.98123521618312));
#75891=CARTESIAN_POINT('Ctrl Pts',(39.6460268170329,2.60324844300542,-1.90241978045346));
#75892=CARTESIAN_POINT('Ctrl Pts',(39.6521766652481,2.66101986350874,-1.8207348071182));
#75893=CARTESIAN_POINT('Ctrl Pts',(39.6583265134633,2.7148622052112,-1.73656003904725));
#75894=CARTESIAN_POINT('Ctrl Pts',(39.6644773218425,2.76871295321453,-1.65237212893226));
#75895=CARTESIAN_POINT('Ctrl Pts',(39.6706281302216,2.81863316988512,-1.5656940179242));
#75896=CARTESIAN_POINT('Ctrl Pts',(39.6767789386008,2.8643999253652,-1.47693284548345));
#75897=CARTESIAN_POINT('Ctrl Pts',(39.6829363249669,2.91021562613935,-1.38807674733426));
#75898=CARTESIAN_POINT('Ctrl Pts',(39.6890937113331,2.95186879620757,-1.29713352603029));
#75899=CARTESIAN_POINT('Ctrl Pts',(39.6952510976993,2.98918341262852,-1.20453314116572));
#75900=CARTESIAN_POINT('Ctrl Pts',(39.7014119204363,3.02651885393352,-1.11188107702733));
#75901=CARTESIAN_POINT('Ctrl Pts',(39.7075727431732,3.05951077617051,-1.01757041753712));
#75902=CARTESIAN_POINT('Ctrl Pts',(39.7137335659102,3.08803277918776,-0.922047242369904));
#75903=CARTESIAN_POINT('Ctrl Pts',(39.7199046888269,3.1166024676798,-0.826364363553567));
#75904=CARTESIAN_POINT('Ctrl Pts',(39.7260758117436,3.1406872046676,-0.729465341565102));
#75905=CARTESIAN_POINT('Ctrl Pts',(39.7322469346602,3.16021150604174,-0.631807565308799));
#75906=CARTESIAN_POINT('Ctrl Pts',(39.7369424566059,3.17506727650892,-0.557501116099729));
#75907=CARTESIAN_POINT('Ctrl Pts',(39.7416379785515,3.18728384858711,-0.482755621299704));
#75908=CARTESIAN_POINT('Ctrl Pts',(39.7463335004971,3.19684815737126,-0.4077737377664));
#75909=CARTESIAN_POINT('Ctrl Pts',(39.7525057485899,3.20942040968641,-0.309210299454161));
#75910=CARTESIAN_POINT('Ctrl Pts',(39.7586779966826,3.21745224028383,-0.209891403028772));
#75911=CARTESIAN_POINT('Ctrl Pts',(39.7648502447754,3.22086289031212,-0.110271502711622));
#75912=CARTESIAN_POINT('Ctrl Pts',(39.771014133428,3.22426892109563,-0.0107865235091495));
#75913=CARTESIAN_POINT('Ctrl Pts',(39.7771780220807,3.22306619650828,0.0889982190027945));
#75914=CARTESIAN_POINT('Ctrl Pts',(39.7833419107333,3.21722545879891,0.188621074528142));
#75915=CARTESIAN_POINT('Ctrl Pts',(39.7894992723919,3.21139090589634,0.288138438565025));
#75916=CARTESIAN_POINT('Ctrl Pts',(39.7956566340504,3.20092812914673,0.38749382518187));
#75917=CARTESIAN_POINT('Ctrl Pts',(39.8018139957089,3.18585990512401,0.486224461975343));
#75918=CARTESIAN_POINT('Ctrl Pts',(39.8079668598553,3.17080268736108,0.584882983101115));
#75919=CARTESIAN_POINT('Ctrl Pts',(39.8141197240016,3.15114677577036,0.682917233567107));
#75920=CARTESIAN_POINT('Ctrl Pts',(39.8202725881479,3.12696679413358,0.779869367834104));
#75921=CARTESIAN_POINT('Ctrl Pts',(39.8264231212844,3.1027959730718,0.876784771829329));
#75922=CARTESIAN_POINT('Ctrl Pts',(39.832573654421,3.07410459255443,0.972618453214989));
#75923=CARTESIAN_POINT('Ctrl Pts',(39.8387241875575,3.041018237068,1.0669234482004));
#75924=CARTESIAN_POINT('Ctrl Pts',(39.8448740357727,3.00793556606715,1.16121794141284));
#75925=CARTESIAN_POINT('Ctrl Pts',(39.8510238839879,2.97045903694599,1.25398367679397));
#75926=CARTESIAN_POINT('Ctrl Pts',(39.8571737322032,2.92876357716053,1.34479049357059));
#75927=CARTESIAN_POINT('Ctrl Pts',(39.8633245405823,2.88706160754345,1.43561148784018));
#75928=CARTESIAN_POINT('Ctrl Pts',(39.8694753489614,2.84113958019999,1.52447256123594));
#75929=CARTESIAN_POINT('Ctrl Pts',(39.8756261573406,2.79121944401683,1.61096603869927));
#75930=CARTESIAN_POINT('Ctrl Pts',(39.8817835437068,2.74124592070318,1.69755201668283));
#75931=CARTESIAN_POINT('Ctrl Pts',(39.887940930073,2.68726596781312,1.78176496559147));
#75932=CARTESIAN_POINT('Ctrl Pts',(39.8940983164391,2.62954609378327,1.86322432980281));
#75933=CARTESIAN_POINT('Ctrl Pts',(39.9002591391761,2.57179400691569,1.94472915560474));
#75934=CARTESIAN_POINT('Ctrl Pts',(39.9064199619131,2.51029810961894,2.02347699393736));
#75935=CARTESIAN_POINT('Ctrl Pts',(39.91258078465,2.44536530223564,2.0991203160186));
#75936=CARTESIAN_POINT('Ctrl Pts',(39.9187519075667,2.38032393474356,2.17489010494463));
#75937=CARTESIAN_POINT('Ctrl Pts',(39.9249230304834,2.31183447757354,2.24754469375133));
#75938=CARTESIAN_POINT('Ctrl Pts',(39.9310941534001,2.24024087531824,2.31677326966913));
#75939=CARTESIAN_POINT('Ctrl Pts',(39.9357896753457,2.1857662950696,2.36944833413767));
#75940=CARTESIAN_POINT('Ctrl Pts',(39.9404851972912,2.12949534416398,2.42014067784178));
#75941=CARTESIAN_POINT('Ctrl Pts',(39.9451807192367,2.07159143502863,2.46872973182891));
#75942=CARTESIAN_POINT('Ctrl Pts',(39.9513534852644,1.99547055063582,2.5326052424212));
#75943=CARTESIAN_POINT('Ctrl Pts',(39.9575262512921,1.91625859641018,2.59306922074264));
#75944=CARTESIAN_POINT('Ctrl Pts',(39.9636990173197,1.83429428297196,2.6498079262385));
#75945=CARTESIAN_POINT('Ctrl Pts',(39.9648183560767,1.81943128114891,2.66009664150796));
#75946=CARTESIAN_POINT('Ctrl Pts',(39.9659376948337,1.80447787411704,2.67026295732891));
#75947=CARTESIAN_POINT('Ctrl Pts',(39.9670570335907,1.78943621037801,2.68030513402635));
#75948=CARTESIAN_POINT('Ctrl Pts',(38.7168453967856,1.78943621037806,2.68030513402632));
#75949=CARTESIAN_POINT('Ctrl Pts',(38.7230162077639,1.70636363716969,2.73576638308381));
#75950=CARTESIAN_POINT('Ctrl Pts',(38.7291870187422,1.6208043826183,2.78729911578586));
#75951=CARTESIAN_POINT('Ctrl Pts',(38.7353578297205,1.53317310434257,2.83469536187234));
#75952=CARTESIAN_POINT('Ctrl Pts',(38.7409376887467,1.45393389562647,2.87755267389499));
#75953=CARTESIAN_POINT('Ctrl Pts',(38.7465175477728,1.37300103670098,2.91702834418697));
#75954=CARTESIAN_POINT('Ctrl Pts',(38.7520974067989,1.29069388353065,2.95300302429858));
#75955=CARTESIAN_POINT('Ctrl Pts',(38.7582696548917,1.19964854227786,2.9927969778137));
#75956=CARTESIAN_POINT('Ctrl Pts',(38.7644419029845,1.10660086958338,3.02844643918464));
#75957=CARTESIAN_POINT('Ctrl Pts',(38.7706141510772,1.0119642434491,3.05974605686166));
#75958=CARTESIAN_POINT('Ctrl Pts',(38.7767780397299,0.917455789287036,3.09100328361784));
#75959=CARTESIAN_POINT('Ctrl Pts',(38.7829419283825,0.821363067822642,3.1179222409927));
#75960=CARTESIAN_POINT('Ctrl Pts',(38.7891058170351,0.724120851622665,3.14034497384368));
#75961=CARTESIAN_POINT('Ctrl Pts',(38.7952631786937,0.626981606031848,3.16274396307228));
#75962=CARTESIAN_POINT('Ctrl Pts',(38.8014205403522,0.528695706567802,3.18065609621248));
#75963=CARTESIAN_POINT('Ctrl Pts',(38.8075779020108,0.429713641743179,3.19397303504582));
#75964=CARTESIAN_POINT('Ctrl Pts',(38.8137307661571,0.330803876236448,3.20728024680794));
#75965=CARTESIAN_POINT('Ctrl Pts',(38.8198836303034,0.231199385550903,3.21599887973733));
#75966=CARTESIAN_POINT('Ctrl Pts',(38.8260364944497,0.131360516853901,3.22007173477733));
#75967=CARTESIAN_POINT('Ctrl Pts',(38.8321870275863,0.03155947206669,3.22414304681806));
#75968=CARTESIAN_POINT('Ctrl Pts',(38.8383375607228,-0.0684753407663051,
3.22357206049524));
#75969=CARTESIAN_POINT('Ctrl Pts',(38.8444880938593,-0.168279679590285,
3.21835354054476));
#75970=CARTESIAN_POINT('Ctrl Pts',(38.8506379420745,-0.26807290423622,3.21313560172693));
#75971=CARTESIAN_POINT('Ctrl Pts',(38.8567877902898,-0.367635272116785,
3.20327118092356));
#75972=CARTESIAN_POINT('Ctrl Pts',(38.862937638505,-0.466504783521725,3.18880712013934));
#75973=CARTESIAN_POINT('Ctrl Pts',(38.8690884468841,-0.565389731232556,
3.17434080110924));
#75974=CARTESIAN_POINT('Ctrl Pts',(38.8752392552632,-0.663581177764809,
3.15527347858415));
#75975=CARTESIAN_POINT('Ctrl Pts',(38.8813900636424,-0.760625472054809,
3.13170344281853));
#75976=CARTESIAN_POINT('Ctrl Pts',(38.8875474500086,-0.857773550444737,
3.10810820005887));
#75977=CARTESIAN_POINT('Ctrl Pts',(38.8937048363748,-0.953771603827205,
3.0800007308617));
#75978=CARTESIAN_POINT('Ctrl Pts',(38.8998622227409,-1.04817946896395,3.04752971492362));
#75979=CARTESIAN_POINT('Ctrl Pts',(38.9060230454779,-1.14264002210968,3.01504057726256));
#75980=CARTESIAN_POINT('Ctrl Pts',(38.9121838682149,-1.2355082158781,2.97818320333855));
#75981=CARTESIAN_POINT('Ctrl Pts',(38.9183446909518,-1.32636421616619,2.93715432495023));
#75982=CARTESIAN_POINT('Ctrl Pts',(38.9245158138685,-1.41737211712934,2.89605685104478));
#75983=CARTESIAN_POINT('Ctrl Pts',(38.9306869367852,-1.50636071750334,2.85077413887356));
#75984=CARTESIAN_POINT('Ctrl Pts',(38.9368580597019,-1.59293499430201,2.80154879779526));
#75985=CARTESIAN_POINT('Ctrl Pts',(38.9415535816474,-1.65880816230022,2.76409391763309));
#75986=CARTESIAN_POINT('Ctrl Pts',(38.946249103593,-1.72328407819148,2.72435741179683));
#75987=CARTESIAN_POINT('Ctrl Pts',(38.9509446255386,-1.78620106900576,2.68246217188289));
#75988=CARTESIAN_POINT('Ctrl Pts',(38.9570996536215,-1.86867450856015,2.6275446608586));
#75989=CARTESIAN_POINT('Ctrl Pts',(38.9632546817044,-1.94876206316078,2.56872070059939));
#75990=CARTESIAN_POINT('Ctrl Pts',(38.9694097097873,-2.02606874386555,2.5062248517703));
#75991=CARTESIAN_POINT('Ctrl Pts',(38.9755563907508,-2.10327058539179,2.44381375646308));
#75992=CARTESIAN_POINT('Ctrl Pts',(38.9817030717144,-2.17769871098348,2.37774094112655));
#75993=CARTESIAN_POINT('Ctrl Pts',(38.987849752678,-2.24898631620097,2.3082846687618));
#75994=CARTESIAN_POINT('Ctrl Pts',(38.9939899412545,-2.32019862440445,2.23890175907908));
#75995=CARTESIAN_POINT('Ctrl Pts',(39.0001301298311,-2.38827669489437,2.16614279976821));
#75996=CARTESIAN_POINT('Ctrl Pts',(39.0062703184076,-2.45288688390502,2.09032617006694));
#75997=CARTESIAN_POINT('Ctrl Pts',(39.0124060784873,-2.51745047401732,2.01456422170115));
#75998=CARTESIAN_POINT('Ctrl Pts',(39.0185418385669,-2.5785508720124,1.93574931853243));
#75999=CARTESIAN_POINT('Ctrl Pts',(39.0246775986465,-2.63589207408145,1.85423583621249));
#76000=CARTESIAN_POINT('Ctrl Pts',(39.0308110992547,-2.69321216045984,1.77275237093813));
#76001=CARTESIAN_POINT('Ctrl Pts',(39.0369445998628,-2.74677554998505,1.68857265798243));
#76002=CARTESIAN_POINT('Ctrl Pts',(39.043078100471,-2.79632782779313,1.6020824704146));
#76003=CARTESIAN_POINT('Ctrl Pts',(39.0492110074707,-2.84587530986541,1.51560065348296));
#76004=CARTESIAN_POINT('Ctrl Pts',(39.0553439144704,-2.89141223479319,1.42680918583746));
#76005=CARTESIAN_POINT('Ctrl Pts',(39.0614768214701,-2.93272921113104,1.33612010563375));
#76006=CARTESIAN_POINT('Ctrl Pts',(39.0676107997968,-2.97405340492551,1.24541518340671));
#76007=CARTESIAN_POINT('Ctrl Pts',(39.0737447781235,-3.01115600500093,1.15281238812868));
#76008=CARTESIAN_POINT('Ctrl Pts',(39.0798787564502,-3.04387542830063,1.05874451095988));
#76009=CARTESIAN_POINT('Ctrl Pts',(39.0860193054742,-3.07662990053854,0.96457586859163));
#76010=CARTESIAN_POINT('Ctrl Pts',(39.0921598544982,-3.10499167842174,0.868939424699028));
#76011=CARTESIAN_POINT('Ctrl Pts',(39.0983004035222,-3.12884888736368,0.772283757787963));
#76012=CARTESIAN_POINT('Ctrl Pts',(39.1044445273219,-3.15271998499353,0.67557182191448));
#76013=CARTESIAN_POINT('Ctrl Pts',(39.1105886511215,-3.17208120795575,0.577839910274741));
#76014=CARTESIAN_POINT('Ctrl Pts',(39.1167327749211,-3.186872104492,0.479545359805227));
#76015=CARTESIAN_POINT('Ctrl Pts',(39.1228868640422,-3.20168699078554,0.381091382731454));
#76016=CARTESIAN_POINT('Ctrl Pts',(39.1290409531633,-3.21191670436259,0.282073379134371));
#76017=CARTESIAN_POINT('Ctrl Pts',(39.1351950422844,-3.2175527969399,0.18295234735923));
#76018=CARTESIAN_POINT('Ctrl Pts',(39.1389878445938,-3.22102635484947,0.12186345657096));
#76019=CARTESIAN_POINT('Ctrl Pts',(39.1427806469031,-3.22275613433671,0.0607354334618325));
#76020=CARTESIAN_POINT('Ctrl Pts',(39.1465734492125,-3.22274998364956,-0.000324633233696488));
#76021=CARTESIAN_POINT('',(38.9000265507268,-3.22274891038197,-0.0026501192081339));
#76022=CARTESIAN_POINT('Ctrl Pts',(38.470402238185,1.78943621037805,2.68030513402632));
#76023=CARTESIAN_POINT('Ctrl Pts',(38.476552475551,1.70631879105963,2.73579632342613));
#76024=CARTESIAN_POINT('Ctrl Pts',(38.482702712917,1.62062405282665,2.78741343758364));
#76025=CARTESIAN_POINT('Ctrl Pts',(38.488852950283,1.53275302880884,2.83492252366398));
#76026=CARTESIAN_POINT('Ctrl Pts',(38.4952501026987,1.44135422578376,2.88433896838047));
#76027=CARTESIAN_POINT('Ctrl Pts',(38.5016472551144,1.3476011671571,2.92931035327353));
#76028=CARTESIAN_POINT('Ctrl Pts',(38.5080444075302,1.25197141895709,2.96962710261989));
#76029=CARTESIAN_POINT('Ctrl Pts',(38.5142038541353,1.15989508723702,3.00844575953955));
#76030=CARTESIAN_POINT('Ctrl Pts',(38.5203633007404,1.0660794941757,3.04294945474506));
#76031=CARTESIAN_POINT('Ctrl Pts',(38.5265227473455,0.970968081115809,3.07300155352292));
#76032=CARTESIAN_POINT('Ctrl Pts',(38.5326865903696,0.875788780523907,3.10307510254268));
#76033=CARTESIAN_POINT('Ctrl Pts',(38.5388504333938,0.779312237762846,3.12869061971578));
#76034=CARTESIAN_POINT('Ctrl Pts',(38.5450142764179,0.681993285611378,3.14976232768141));
#76035=CARTESIAN_POINT('Ctrl Pts',(38.5511872779008,0.584529733474962,3.17086534474549));
#76036=CARTESIAN_POINT('Ctrl Pts',(38.5573602793837,0.486221701546851,3.18741101349978));
#76037=CARTESIAN_POINT('Ctrl Pts',(38.5635332808666,0.387530032000321,3.19936525529641));
#76038=CARTESIAN_POINT('Ctrl Pts',(38.5642284470017,0.376415972384852,3.20071146979045));
#76039=CARTESIAN_POINT('Ctrl Pts',(38.5649236131368,0.365297047613253,3.20199951063944));
#76040=CARTESIAN_POINT('Ctrl Pts',(38.565618779272,0.354173915195078,3.20322937054083));
#76041=CARTESIAN_POINT('Ctrl Pts',(38.5717910273647,0.255413734879611,3.21414906303909));
#76042=CARTESIAN_POINT('Ctrl Pts',(38.5779632754575,0.155974247973943,3.22051631785057));
#76043=CARTESIAN_POINT('Ctrl Pts',(38.5841355235503,0.0563111975495212,
3.22225799890861));
#76044=CARTESIAN_POINT('Ctrl Pts',(38.5902994122029,-0.0432168733195461,
3.22399732110514));
#76045=CARTESIAN_POINT('Ctrl Pts',(38.5964633008555,-0.142967475403352,
3.22112351378161));
#76046=CARTESIAN_POINT('Ctrl Pts',(38.6026271895082,-0.242478533134772,
3.21361505527168));
#76047=CARTESIAN_POINT('Ctrl Pts',(38.6087845511667,-0.34188421776127,3.20611454753229));
#76048=CARTESIAN_POINT('Ctrl Pts',(38.6149419128253,-0.441050431570951,
3.19398917802298));
#76049=CARTESIAN_POINT('Ctrl Pts',(38.6210992744838,-0.539514848547188,
3.17726947089747));
#76050=CARTESIAN_POINT('Ctrl Pts',(38.6272521386301,-0.637907344310258,
3.16056197632201));
#76051=CARTESIAN_POINT('Ctrl Pts',(38.6334050027764,-0.735598635446793,
3.13926688860308));
#76052=CARTESIAN_POINT('Ctrl Pts',(38.6395578669228,-0.832132190479647,
3.1134664893118));
#76053=CARTESIAN_POINT('Ctrl Pts',(38.6457084000593,-0.928629173819252,
3.08767586449001));
#76054=CARTESIAN_POINT('Ctrl Pts',(38.6518589331958,-1.02396887338675,3.05738343160187));
#76055=CARTESIAN_POINT('Ctrl Pts',(38.6580094663324,-1.11770649144595,3.02272224352149));
#76056=CARTESIAN_POINT('Ctrl Pts',(38.6641593145476,-1.21143367091506,2.98806491529953));
#76057=CARTESIAN_POINT('Ctrl Pts',(38.6703091627628,-1.30355871616046,2.94903994977381));
#76058=CARTESIAN_POINT('Ctrl Pts',(38.676459010978,-1.39365445653052,2.90582945444027));
#76059=CARTESIAN_POINT('Ctrl Pts',(38.6826098193571,-1.48376426337474,2.86261221273544));
#76060=CARTESIAN_POINT('Ctrl Pts',(38.6887606277363,-1.57184374433822,2.81520833110536));
#76061=CARTESIAN_POINT('Ctrl Pts',(38.6949114361154,-1.65748899887154,2.76384655527759));
#76062=CARTESIAN_POINT('Ctrl Pts',(38.7010688224816,-1.74322584679221,2.71242985055675));
#76063=CARTESIAN_POINT('Ctrl Pts',(38.7072262088478,-1.8265228965419,2.657047023066));
#76064=CARTESIAN_POINT('Ctrl Pts',(38.713383595214,-1.90700410951207,2.59797091762092));
#76065=CARTESIAN_POINT('Ctrl Pts',(38.7195444179509,-1.98753023817731,2.53886184243992));
#76066=CARTESIAN_POINT('Ctrl Pts',(38.7257052406879,-2.06523706262828,2.47605565755229));
#76067=CARTESIAN_POINT('Ctrl Pts',(38.7318660634249,-2.13978224297069,2.40986504086169));
#76068=CARTESIAN_POINT('Ctrl Pts',(38.7380371863416,-2.21445205419244,2.34356376115138));
#76069=CARTESIAN_POINT('Ctrl Pts',(38.7442083092582,-2.28594935169415,2.27386705055432));
#76070=CARTESIAN_POINT('Ctrl Pts',(38.7503794321749,-2.35396912688206,2.20112401108755));
#76071=CARTESIAN_POINT('Ctrl Pts',(38.7550749541204,-2.40572443161908,2.14577483998694));
#76072=CARTESIAN_POINT('Ctrl Pts',(38.7597704760659,-2.45546720706799,2.08866275793249));
#76073=CARTESIAN_POINT('Ctrl Pts',(38.7644659980114,-2.50307963811206,2.02995317378722));
#76074=CARTESIAN_POINT('Ctrl Pts',(38.770617892004,-2.56545963162721,1.95303411298838));
#76075=CARTESIAN_POINT('Ctrl Pts',(38.7767697859965,-2.62440669444763,1.87309396875357));
#76076=CARTESIAN_POINT('Ctrl Pts',(38.7829216799891,-2.67961273722208,1.79047288195526));
#76077=CARTESIAN_POINT('Ctrl Pts',(38.7890655633465,-2.73474689392971,1.7079593794841));
#76078=CARTESIAN_POINT('Ctrl Pts',(38.795209446704,-2.78614946672464,1.6227722284766));
#76079=CARTESIAN_POINT('Ctrl Pts',(38.8013533300615,-2.83355202996752,1.53528513832675));
#76080=CARTESIAN_POINT('Ctrl Pts',(38.8074908818402,-2.88090574250036,1.44788820799485));
#76081=CARTESIAN_POINT('Ctrl Pts',(38.8136284336188,-2.92426742931672,1.3581964298393));
#76082=CARTESIAN_POINT('Ctrl Pts',(38.8197659853975,-2.96341207728283,1.26661218323301));
#76083=CARTESIAN_POINT('Ctrl Pts',(38.8258988786077,-3.00252701339788,1.1750974515575));
#76084=CARTESIAN_POINT('Ctrl Pts',(38.8320317718178,-3.03743110192722,1.081693507172));
#76085=CARTESIAN_POINT('Ctrl Pts',(38.838164665028,-3.06794586854737,0.986826078984108));
#76086=CARTESIAN_POINT('Ctrl Pts',(38.8442952427761,-3.09844911437588,0.891994467811846));
#76087=CARTESIAN_POINT('Ctrl Pts',(38.8504258205242,-3.12456619503217,0.795700885438159));
#76088=CARTESIAN_POINT('Ctrl Pts',(38.8565563982723,-3.14616759141027,0.698388895429812));
#76089=CARTESIAN_POINT('Ctrl Pts',(38.8626856552264,-3.16776433390495,0.601097870670672));
#76090=CARTESIAN_POINT('Ctrl Pts',(38.8688149121805,-3.18484723621972,0.502789302088776));
#76091=CARTESIAN_POINT('Ctrl Pts',(38.8749441691346,-3.19733754636273,0.403918527823539));
#76092=CARTESIAN_POINT('Ctrl Pts',(38.8810752541797,-3.20983158182246,0.305018264703097));
#76093=CARTESIAN_POINT('Ctrl Pts',(38.8872063392248,-3.21773023802526,0.205555895204617));
#76094=CARTESIAN_POINT('Ctrl Pts',(38.8933374242699,-3.22100653419584,0.105992778846848));
#76095=CARTESIAN_POINT('Ctrl Pts',(38.8955671330889,-3.22219803397303,0.0697843822980494));
#76096=CARTESIAN_POINT('Ctrl Pts',(38.8977968419078,-3.22277868876192,0.0335626825532226));
#76097=CARTESIAN_POINT('Ctrl Pts',(38.9000265507268,-3.22274891038197,-0.0026501192081339));
#76098=CARTESIAN_POINT('Ctrl Pts',(38.8985201488241,-3.22274882644913,-0.00275029466297132));
#76099=CARTESIAN_POINT('Ctrl Pts',(38.9060646964583,-3.22265200588648,-0.116202994426138));
#76100=CARTESIAN_POINT('Ctrl Pts',(38.9137273955404,-3.21656432972955,-0.229568442334264));
#76101=CARTESIAN_POINT('Ctrl Pts',(38.9342509370667,-3.18435131639635,-0.531072642175193));
#76102=CARTESIAN_POINT('Ctrl Pts',(38.9471159326192,-3.14756042191507,-0.717641260126694));
#76103=CARTESIAN_POINT('Ctrl Pts',(38.9608598654036,-3.08753583555694,-0.924052271636377));
#76104=CARTESIAN_POINT('Ctrl Pts',(38.9624543148532,-3.08023007553678,-0.948120726273012));
#76105=CARTESIAN_POINT('Ctrl Pts',(38.9644870520352,-3.07046149605965,-0.97899748198622));
#76106=CARTESIAN_POINT('Ctrl Pts',(38.9649397043297,-3.06825673625823,-0.98588562791305));
#76107=CARTESIAN_POINT('Ctrl Pts',(38.9656676598682,-3.06466302342795,-0.996984338830863));
#76108=CARTESIAN_POINT('Ctrl Pts',(38.9659438049694,-3.06328855223262,-1.00119951326819));
#76109=CARTESIAN_POINT('Ctrl Pts',(38.9664722423174,-3.06063669072522,-1.00927555579891));
#76110=CARTESIAN_POINT('Ctrl Pts',(38.9667246121572,-3.059360694359,-1.01313683286044));
#76111=CARTESIAN_POINT('Ctrl Pts',(38.9673084352517,-3.05638682379991,-1.02207917769647));
#76112=CARTESIAN_POINT('Ctrl Pts',(38.9676395701081,-3.05468357482492,-1.02715846920368));
#76113=CARTESIAN_POINT('Ctrl Pts',(38.9687082890737,-3.04913324897155,-1.04357429444997));
#76114=CARTESIAN_POINT('Ctrl Pts',(38.9694429366095,-3.04523561314486,-1.05489380931277));
#76115=CARTESIAN_POINT('Ctrl Pts',(38.9785458355029,-2.99592728416941,-1.1955441310358));
#76116=CARTESIAN_POINT('Ctrl Pts',(38.9864568303832,-2.94236691354503,-1.32188994192928));
#76117=CARTESIAN_POINT('Ctrl Pts',(39.0028115940323,-2.81287013402245,-1.58016675697157));
#76118=CARTESIAN_POINT('Ctrl Pts',(39.0112054661125,-2.73532043748411,-1.71090307810846));
#76119=CARTESIAN_POINT('Ctrl Pts',(39.0267281531353,-2.57809726251247,-1.93777140170975));
#76120=CARTESIAN_POINT('Ctrl Pts',(39.0337946066843,-2.50151456522588,-2.03567301473938));
#76121=CARTESIAN_POINT('Ctrl Pts',(39.0439903946623,-2.38644791646327,-2.16644504998062));
#76122=CARTESIAN_POINT('Ctrl Pts',(39.0469478315879,-2.35254913044546,-2.20320902624393));
#76123=CARTESIAN_POINT('Ctrl Pts',(39.0519244990418,-2.29478016659834,-2.26300689593011));
#76124=CARTESIAN_POINT('Ctrl Pts',(39.0539236213976,-2.27138455005892,-2.28648820800489));
#76125=CARTESIAN_POINT('Ctrl Pts',(39.0566366021057,-2.23940584424875,-2.31760884744372));
#76126=CARTESIAN_POINT('Ctrl Pts',(39.0573363451112,-2.23113750439746,-2.32556976591372));
#76127=CARTESIAN_POINT('Ctrl Pts',(39.0584497265335,-2.21795047446691,-2.33813143608706));
#76128=CARTESIAN_POINT('Ctrl Pts',(39.0588621018268,-2.21305953287834,-2.34276128157625));
#76129=CARTESIAN_POINT('Ctrl Pts',(39.0597184350409,-2.20288941492897,-2.35232821530745));
#76130=CARTESIAN_POINT('Ctrl Pts',(39.0601624911539,-2.19760807407725,-2.35726293788632));
#76131=CARTESIAN_POINT('Ctrl Pts',(39.0611779641854,-2.18551370124927,-2.36848757744297));
#76132=CARTESIAN_POINT('Ctrl Pts',(39.0617498705785,-2.17869005764982,-2.37476591955278));
#76133=CARTESIAN_POINT('Ctrl Pts',(39.0632399616886,-2.1608802763392,-2.39101108865657));
#76134=CARTESIAN_POINT('Ctrl Pts',(39.0641600961901,-2.14985234712002,-2.40093158346605));
#76135=CARTESIAN_POINT('Ctrl Pts',(39.0700523123043,-2.07904657484831,-2.46374801164275));
#76136=CARTESIAN_POINT('Ctrl Pts',(39.0751135767923,-2.01739402072552,-2.5144797611));
#76137=CARTESIAN_POINT('Ctrl Pts',(39.0816576877401,-1.93671581623818,-2.57598869790745));
#76138=CARTESIAN_POINT('Ctrl Pts',(39.0830598303985,-1.91937402482795,-2.58893592885779));
#76139=CARTESIAN_POINT('Ctrl Pts',(39.095158199764,-1.76925727623235,-2.69867447022444));
#76140=CARTESIAN_POINT('Ctrl Pts',(39.1061877187551,-1.62940319134005,-2.78534556118557));
#76141=CARTESIAN_POINT('Ctrl Pts',(39.1310554276237,-1.30307727624624,-2.95456318157637));
#76142=CARTESIAN_POINT('Ctrl Pts',(39.144890819654,-1.11411962683837,-3.0308754908564));
#76143=CARTESIAN_POINT('Ctrl Pts',(39.1595655495452,-0.894286465908746,
-3.09629550326156));
#76144=CARTESIAN_POINT('Ctrl Pts',(39.1612152681434,-0.869266249104422,
-3.10341270501232));
#76145=CARTESIAN_POINT('Ctrl Pts',(39.1633077428594,-0.837097675294885,
-3.11214373391211));
#76146=CARTESIAN_POINT('Ctrl Pts',(39.1637659048934,-0.830027083431778,
-3.11403695895987));
#76147=CARTESIAN_POINT('Ctrl Pts',(39.1645005750268,-0.818644567928665,
-3.11704322457693));
#76148=CARTESIAN_POINT('Ctrl Pts',(39.164777952878,-0.814336731143821,-3.11817143232451));
#76149=CARTESIAN_POINT('Ctrl Pts',(39.1653072340641,-0.806096638369069,
-3.12031124372292));
#76150=CARTESIAN_POINT('Ctrl Pts',(39.1655592207741,-0.802164820393485,
-3.12132434219196));
#76151=CARTESIAN_POINT('Ctrl Pts',(39.1661401310563,-0.793080681372778,
-3.12364672387928));
#76152=CARTESIAN_POINT('Ctrl Pts',(39.1664687462443,-0.787926995002609,
-3.1249506994953));
#76153=CARTESIAN_POINT('Ctrl Pts',(39.1675211914722,-0.771374672504296,
-3.12909518440884));
#76154=CARTESIAN_POINT('Ctrl Pts',(39.1682422086155,-0.75996356322609,-3.13188616506836));
#76155=CARTESIAN_POINT('Ctrl Pts',(39.1806045765768,-0.563140756821354,
-3.17888690149245));
#76156=CARTESIAN_POINT('Ctrl Pts',(39.1913569285077,-0.374150769360753,
-3.2066312026352));
#76157=CARTESIAN_POINT('Ctrl Pts',(39.2122694844599,-0.00121749177307916,
-3.2279340295954));
#76158=CARTESIAN_POINT('Ctrl Pts',(39.2224054714749,0.181903165602953,-3.22280421356543));
#76159=CARTESIAN_POINT('Ctrl Pts',(39.2372713190132,0.438304764730845,-3.19369061386641));
#76160=CARTESIAN_POINT('Ctrl Pts',(39.2416620380048,0.512688559534677,-3.18259643223032));
#76161=CARTESIAN_POINT('Ctrl Pts',(39.2479097065956,0.6160283649675,-3.16346669759801));
#76162=CARTESIAN_POINT('Ctrl Pts',(39.2497001187966,0.645365995493569,-3.15761225238062));
#76163=CARTESIAN_POINT('Ctrl Pts',(39.2528364200477,0.69624236187107,-3.14672102609189));
#76164=CARTESIAN_POINT('Ctrl Pts',(39.2541764172686,0.717818903528417,-3.14186928860523));
#76165=CARTESIAN_POINT('Ctrl Pts',(39.2561215146016,0.748897947416826,-3.13454395213167));
#76166=CARTESIAN_POINT('Ctrl Pts',(39.2567208830823,0.758442074818032,-3.13224832018168));
#76167=CARTESIAN_POINT('Ctrl Pts',(39.2577709951808,0.775105787075725,-3.12815960006328));
#76168=CARTESIAN_POINT('Ctrl Pts',(39.2582211157141,0.782230044702907,-3.12638571202832));
#76169=CARTESIAN_POINT('Ctrl Pts',(39.2590874270533,0.795905698927279,-3.12293090332341));
#76170=CARTESIAN_POINT('Ctrl Pts',(39.2595034963001,0.802457994069226,-3.12125367042773));
#76171=CARTESIAN_POINT('Ctrl Pts',(39.2604847552606,0.817873446638981,-3.11725592919275));
#76172=CARTESIAN_POINT('Ctrl Pts',(39.2610505002606,0.826732049784069,-3.11491823614743));
#76173=CARTESIAN_POINT('Ctrl Pts',(39.2627263144103,0.85288540520665,-3.10789721351607));
#76174=CARTESIAN_POINT('Ctrl Pts',(39.2638398349749,0.87015098637429,-3.10310744967131));
#76175=CARTESIAN_POINT('Ctrl Pts',(39.2784167370843,1.09468522842714,-3.03879660971757));
#76176=CARTESIAN_POINT('Ctrl Pts',(39.2925765874064,1.29547090309156,-2.95877390785682));
#76177=CARTESIAN_POINT('Ctrl Pts',(39.3236060632252,1.70446215143974,-2.7461154021794));
#76178=CARTESIAN_POINT('Ctrl Pts',(39.3404844841917,1.90855728384211,-2.60840224484998));
#76179=CARTESIAN_POINT('Ctrl Pts',(39.3580334495631,2.11659345332662,-2.43042249535349));
#76180=CARTESIAN_POINT('Ctrl Pts',(39.3598338094991,2.13789326882415,-2.41170766382542));
#76181=CARTESIAN_POINT('Ctrl Pts',(39.362088067794,2.16454501255764,-2.38765980814599));
#76182=CARTESIAN_POINT('Ctrl Pts',(39.3625603862631,2.17012814276729,-2.38258647639716));
#76183=CARTESIAN_POINT('Ctrl Pts',(39.3633123046844,2.17901559178365,-2.37445338808269));
#76184=CARTESIAN_POINT('Ctrl Pts',(39.3635928476753,2.18233135854243,-2.37140626707652));
#76185=CARTESIAN_POINT('Ctrl Pts',(39.3641244437186,2.18861425477795,-2.36560807787784));
#76186=CARTESIAN_POINT('Ctrl Pts',(39.364375592533,2.1915825543244,-2.36285840500009));
#76187=CARTESIAN_POINT('Ctrl Pts',(39.3649496923495,2.19836757908613,-2.35654933867806));
#76188=CARTESIAN_POINT('Ctrl Pts',(39.3652723563752,2.20218083717264,-2.35298626423987));
#76189=CARTESIAN_POINT('Ctrl Pts',(39.3662869752354,2.21417037657158,-2.34172866957656));
#76190=CARTESIAN_POINT('Ctrl Pts',(39.3669763940253,2.22231522198972,-2.33400057437667));
#76191=CARTESIAN_POINT('Ctrl Pts',(39.3731745779831,2.2955022818334,-2.26382786535447));
#76192=CARTESIAN_POINT('Ctrl Pts',(39.378486609106,2.35794427168836,-2.19871541235758));
#76193=CARTESIAN_POINT('Ctrl Pts',(39.4000428827543,2.60505184109672,-1.91838491640368));
#76194=CARTESIAN_POINT('Ctrl Pts',(39.4153219986218,2.76364748371816,-1.68189455695802));
#76195=CARTESIAN_POINT('Ctrl Pts',(39.4360117104762,2.92279468129681,-1.35982318984196));
#76196=CARTESIAN_POINT('Ctrl Pts',(39.4404311777144,2.95392593481961,-1.29080138369009));
#76197=CARTESIAN_POINT('Ctrl Pts',(39.4467170348712,2.99398351238235,-1.19293080652955));
#76198=CARTESIAN_POINT('Ctrl Pts',(39.4485159481675,3.00497999541645,-1.1649533547499));
#76199=CARTESIAN_POINT('Ctrl Pts',(39.4516768941388,3.02347859342186,-1.11588338236529));
#76200=CARTESIAN_POINT('Ctrl Pts',(39.4530330784389,3.03115539313289,-1.09485865373304));
#76201=CARTESIAN_POINT('Ctrl Pts',(39.4549986572776,3.04190535397881,-1.06443743835153));
#76202=CARTESIAN_POINT('Ctrl Pts',(39.4556021649113,3.04515536944266,-1.05510379359517));
#76203=CARTESIAN_POINT('Ctrl Pts',(39.4566550729737,3.05073726565942,-1.03883264459062));
#76204=CARTESIAN_POINT('Ctrl Pts',(39.4571038260695,3.05308855496693,-1.03190183722951));
#76205=CARTESIAN_POINT('Ctrl Pts',(39.4579707542821,3.05757739782353,-1.01852059176025));
#76206=CARTESIAN_POINT('Ctrl Pts',(39.4583888190526,3.05971820046875,-1.01207127817765));
#76207=CARTESIAN_POINT('Ctrl Pts',(39.4593798229488,3.06473633371996,-0.996792359630693));
#76208=CARTESIAN_POINT('Ctrl Pts',(39.4599533446228,3.06759591682979,-0.987957029224714));
#76209=CARTESIAN_POINT('Ctrl Pts',(39.4619682508713,3.07748604416483,-0.956942299578186));
#76210=CARTESIAN_POINT('Ctrl Pts',(39.4634162599488,3.08431441993459,-0.934699646918499));
#76211=CARTESIAN_POINT('Ctrl Pts',(39.4657510162797,3.0948771344825,-0.898916188733655));
#76212=CARTESIAN_POINT('Ctrl Pts',(39.4666327019952,3.09876491676096,-0.885421240144417));
#76213=CARTESIAN_POINT('Ctrl Pts',(39.483775701864,3.17240055600699,-0.623397018444148));
#76214=CARTESIAN_POINT('Ctrl Pts',(39.5010505570153,3.21211432778571,-0.367449694747811));
#76215=CARTESIAN_POINT('Ctrl Pts',(39.5311854738334,3.22725053041123,0.0774996261143986));
#76216=CARTESIAN_POINT('Ctrl Pts',(39.5438648346921,3.21730558876417,0.2647845740104));
#76217=CARTESIAN_POINT('Ctrl Pts',(39.5574298419839,3.18766600581436,0.474896824223559));
#76218=CARTESIAN_POINT('Ctrl Pts',(39.5590132968879,3.18388915199246,0.499591350544052));
#76219=CARTESIAN_POINT('Ctrl Pts',(39.5610341248735,3.17865181998118,0.531358843038604));
#76220=CARTESIAN_POINT('Ctrl Pts',(39.5614856595138,3.17745431937394,0.538473456559237));
#76221=CARTESIAN_POINT('Ctrl Pts',(39.5622122529664,3.1754830282558,0.549949744264628));
#76222=CARTESIAN_POINT('Ctrl Pts',(39.5624881480203,3.17472412741696,0.554313899627152));
#76223=CARTESIAN_POINT('Ctrl Pts',(39.5630164185219,3.17325101821033,0.562682936220123));
#76224=CARTESIAN_POINT('Ctrl Pts',(39.5632688703792,3.17253822659056,0.566688020208856));
#76225=CARTESIAN_POINT('Ctrl Pts',(39.5638533038773,3.17086766034932,0.575972772740443));
#76226=CARTESIAN_POINT('Ctrl Pts',(39.5641849650229,3.16990427541127,0.581251443099394));
#76227=CARTESIAN_POINT('Ctrl Pts',(39.5652571030804,3.16674036201778,0.598345626927872));
#76228=CARTESIAN_POINT('Ctrl Pts',(39.565994617083,3.16448688921343,0.610151414228941));
#76229=CARTESIAN_POINT('Ctrl Pts',(39.5757634998126,3.13361763792488,0.767100682506316));
#76230=CARTESIAN_POINT('Ctrl Pts',(39.5842616995361,3.09510262022304,0.910140041574776));
#76231=CARTESIAN_POINT('Ctrl Pts',(39.6047211540041,2.97697262499853,1.25291531162425));
#76232=CARTESIAN_POINT('Ctrl Pts',(39.6164973752005,2.88697295120931,1.44829215009111));
#76233=CARTESIAN_POINT('Ctrl Pts',(39.6335266825743,2.73659168282322,1.70409264763878));
#76234=CARTESIAN_POINT('Ctrl Pts',(39.6383081810283,2.69226987087226,1.77328712380675));
#76235=CARTESIAN_POINT('Ctrl Pts',(39.6460531284891,2.6177357392548,1.88040304191996));
#76236=CARTESIAN_POINT('Ctrl Pts',(39.648954254884,2.58922717117262,1.91946822815361));
#76237=CARTESIAN_POINT('Ctrl Pts',(39.6526951964302,2.55178911319659,1.96841713291518));
#76238=CARTESIAN_POINT('Ctrl Pts',(39.6535033561351,2.54366168844175,1.97890851074509));
#76239=CARTESIAN_POINT('Ctrl Pts',(39.6548045851885,2.53051358668526,1.99566605820484));
#76240=CARTESIAN_POINT('Ctrl Pts',(39.6552960212839,2.52553383161893,2.00196425836531));
#76241=CARTESIAN_POINT('Ctrl Pts',(39.6562310272417,2.51603296095574,2.01388872501931));
#76242=CARTESIAN_POINT('Ctrl Pts',(39.6566744135268,2.51151637221115,2.01951854860044));
#76243=CARTESIAN_POINT('Ctrl Pts',(39.6576837967055,2.50120905207499,2.03227832962638));
#76244=CARTESIAN_POINT('Ctrl Pts',(39.65825026175,2.49540669349987,2.0393987747592));
#76245=CARTESIAN_POINT('Ctrl Pts',(39.6597170765945,2.48033640508947,2.05773188190855));
#76246=CARTESIAN_POINT('Ctrl Pts',(39.6606192771946,2.4710229309074,2.0689066784153));
#76247=CARTESIAN_POINT('Ctrl Pts',(39.6662001699113,2.41314484376644,2.13740353205753));
#76248=CARTESIAN_POINT('Ctrl Pts',(39.6709576181331,2.3626672442439,2.19307178784247));
#76249=CARTESIAN_POINT('Ctrl Pts',(39.6776383145208,2.29030238348289,2.26747761828332));
#76250=CARTESIAN_POINT('Ctrl Pts',(39.679494840397,2.27003778255748,2.28776487958639));
#76251=CARTESIAN_POINT('Ctrl Pts',(39.682332450524,2.23882797620103,2.31818661798342));
#76252=CARTESIAN_POINT('Ctrl Pts',(39.6833060080094,2.2280783252365,2.32852031749382));
#76253=CARTESIAN_POINT('Ctrl Pts',(39.6909930169581,2.14286885525137,2.40930235810437));
#76254=CARTESIAN_POINT('Ctrl Pts',(39.6978264002758,2.06516308126227,2.47623172528963));
#76255=CARTESIAN_POINT('Ctrl Pts',(39.7101288006093,1.92114834567543,2.58877417296029));
#76256=CARTESIAN_POINT('Ctrl Pts',(39.7155639546189,1.85611072403138,2.63579163576638));
#76257=CARTESIAN_POINT('Ctrl Pts',(39.7209886430068,1.78943588752252,2.68030534957241));
#76258=CARTESIAN_POINT('Origin',(-1.72497344927317,0.,0.));
#76259=CARTESIAN_POINT('',(41.2170239499866,1.789436210378,2.68030513402635));
#76260=CARTESIAN_POINT('',(40.972917806056,1.78943621030417,2.68030513407564));
#76261=CARTESIAN_POINT('',(-1.72497344927317,1.78943621037804,2.68030513402633));
#76262=CARTESIAN_POINT('',(40.3965734492378,-3.22274866702434,0.00293115895939317));
#76263=CARTESIAN_POINT('Ctrl Pts',(40.3965734492731,-3.22274866702486,0.0029311583875785));
#76264=CARTESIAN_POINT('Ctrl Pts',(40.4026689406047,-3.22283856608011,-0.0959110132575726));
#76265=CARTESIAN_POINT('Ctrl Pts',(40.4087644319364,-3.21837696149856,-0.194856635371052));
#76266=CARTESIAN_POINT('Ctrl Pts',(40.414859923268,-3.20936208299301,-0.293449455182281));
#76267=CARTESIAN_POINT('Ctrl Pts',(40.4209523799394,-3.20035169257419,-0.391993190235922));
#76268=CARTESIAN_POINT('Ctrl Pts',(40.4270448366108,-3.18679257004819,-0.490184030980883));
#76269=CARTESIAN_POINT('Ctrl Pts',(40.4331372932821,-3.16873499236898,-0.587567962568068));
#76270=CARTESIAN_POINT('Ctrl Pts',(40.4392284227892,-3.15068134830373,-0.684930680302494));
#76271=CARTESIAN_POINT('Ctrl Pts',(40.4453195522962,-3.12813127669672,-0.781486402120908));
#76272=CARTESIAN_POINT('Ctrl Pts',(40.4514106818033,-3.10118648075366,-0.876789583703369));
#76273=CARTESIAN_POINT('Ctrl Pts',(40.4575021900668,-3.07424000933875,-0.972098691394826));
#76274=CARTESIAN_POINT('Ctrl Pts',(40.4635936983303,-3.04289839255802,-1.06615467758334));
#76275=CARTESIAN_POINT('Ctrl Pts',(40.4696852065938,-3.00731337428556,-1.15852657774571));
#76276=CARTESIAN_POINT('Ctrl Pts',(40.4757828570208,-2.97169247508056,-1.25099161794506));
#76277=CARTESIAN_POINT('Ctrl Pts',(40.4818805074477,-2.93181978869112,-1.34176876585871));
#76278=CARTESIAN_POINT('Ctrl Pts',(40.4879781578746,-2.88789538548396,-1.43044671519091));
#76279=CARTESIAN_POINT('Ctrl Pts',(40.4940788340213,-2.84394918651556,-1.5191686674752));
#76280=CARTESIAN_POINT('Ctrl Pts',(40.5001795101679,-2.79594748334401,-1.6057889593936));
#76281=CARTESIAN_POINT('Ctrl Pts',(40.5062801863146,-2.74413544236778,-1.68992255338551));
#76282=CARTESIAN_POINT('Ctrl Pts',(40.5123914223628,-2.69223371788128,-1.77420177754172));
#76283=CARTESIAN_POINT('Ctrl Pts',(40.518502658411,-2.63650873011724,-1.85598533823604));
#76284=CARTESIAN_POINT('Ctrl Pts',(40.5246138944592,-2.57724802975836,-1.93491864314928));
#76285=CARTESIAN_POINT('Ctrl Pts',(40.530316721458,-2.5219476749181,-2.00857689801266));
#76286=CARTESIAN_POINT('Ctrl Pts',(40.5360195484569,-2.46356899750457,-2.07975324295799));
#76287=CARTESIAN_POINT('Ctrl Pts',(40.5417223754557,-2.4023743985966,-2.14818872808411));
#76288=CARTESIAN_POINT('Ctrl Pts',(40.5478946235485,-2.33614264257929,-2.2222573948404));
#76289=CARTESIAN_POINT('Ctrl Pts',(40.5540668716413,-2.26636563631585,-2.29339052978325));
#76290=CARTESIAN_POINT('Ctrl Pts',(40.560239119734,-2.19333382918926,-2.36122939932442));
#76291=CARTESIAN_POINT('Ctrl Pts',(40.5664030083867,-2.1204009333524,-2.42897639067795));
#76292=CARTESIAN_POINT('Ctrl Pts',(40.5725668970393,-2.04422231382743,-2.4934376915636));
#76293=CARTESIAN_POINT('Ctrl Pts',(40.5787307856919,-1.96512759576635,-2.55428876497109));
#76294=CARTESIAN_POINT('Ctrl Pts',(40.5848881473505,-1.88611663177433,-2.61507540265988));
#76295=CARTESIAN_POINT('Ctrl Pts',(40.591045509009,-1.80419605062523,-2.67225914975049));
#76296=CARTESIAN_POINT('Ctrl Pts',(40.5972028706676,-1.71973041347598,-2.72555404779758));
#76297=CARTESIAN_POINT('Ctrl Pts',(40.6033557348139,-1.63532647243283,-2.77881001773382));
#76298=CARTESIAN_POINT('Ctrl Pts',(40.6095085989602,-1.54838153761617,-2.82818255498478));
#76299=CARTESIAN_POINT('Ctrl Pts',(40.6156614631065,-1.45929041340567,-2.8734281010393));
#76300=CARTESIAN_POINT('Ctrl Pts',(40.6218119962431,-1.37023304132688,-2.91865650583936));
#76301=CARTESIAN_POINT('Ctrl Pts',(40.6279625293796,-1.27903148230783,-2.95976082965567));
#76302=CARTESIAN_POINT('Ctrl Pts',(40.6341130625161,-1.18610570407999,-2.99654314523401));
#76303=CARTESIAN_POINT('Ctrl Pts',(40.6402629107313,-1.09319027403589,-3.03332136474592));
#76304=CARTESIAN_POINT('Ctrl Pts',(40.6464127589466,-0.99855141041053,-3.06577837304117));
#76305=CARTESIAN_POINT('Ctrl Pts',(40.6525626071618,-0.902628710776066,
-3.09376453095298));
#76306=CARTESIAN_POINT('Ctrl Pts',(40.6587134155409,-0.806691034915567,
-3.12175505828964));
#76307=CARTESIAN_POINT('Ctrl Pts',(40.66486422392,-0.709469541944053,-3.14527322711302));
#76308=CARTESIAN_POINT('Ctrl Pts',(40.6710150322992,-0.611417644943363,
-3.16421965513646));
#76309=CARTESIAN_POINT('Ctrl Pts',(40.6771724186654,-0.513260886261442,
-3.18318634543281));
#76310=CARTESIAN_POINT('Ctrl Pts',(40.6833298050316,-0.414272377471576,
-3.19757144902812));
#76311=CARTESIAN_POINT('Ctrl Pts',(40.6894871913978,-0.314914233430923,
-3.20732701608093));
#76312=CARTESIAN_POINT('Ctrl Pts',(40.6956480141347,-0.215500638684147,
-3.21708802761026));
#76313=CARTESIAN_POINT('Ctrl Pts',(40.7018088368717,-0.115717431681363,
-3.22221433491865));
#76314=CARTESIAN_POINT('Ctrl Pts',(40.7079696596087,-0.016028235548225,
-3.22271014181623));
#76315=CARTESIAN_POINT('Ctrl Pts',(40.7141407825253,0.0838276293370653,
-3.22320677764534));
#76316=CARTESIAN_POINT('Ctrl Pts',(40.720311905442,0.183588735197978,-3.21905746739879));
#76317=CARTESIAN_POINT('Ctrl Pts',(40.7264830283587,0.282794931016511,-3.21031845608677));
#76318=CARTESIAN_POINT('Ctrl Pts',(40.7311785503043,0.358279551220556,-3.20366906343137));
#76319=CARTESIAN_POINT('Ctrl Pts',(40.7358740722498,0.433442980414044,-3.19436355227302));
#76320=CARTESIAN_POINT('Ctrl Pts',(40.7405695941953,0.508087071587692,-3.18244640020621));
#76321=CARTESIAN_POINT('Ctrl Pts',(40.7467418422881,0.606206482960046,-3.16678134316491));
#76322=CARTESIAN_POINT('Ctrl Pts',(40.7529140903809,0.703773451911838,-3.14654671790471));
#76323=CARTESIAN_POINT('Ctrl Pts',(40.7590863384736,0.800329159595483,-3.12179288211137));
#76324=CARTESIAN_POINT('Ctrl Pts',(40.7652502271263,0.896754096181804,-3.09707257189976));
#76325=CARTESIAN_POINT('Ctrl Pts',(40.7714141157789,0.992170076689239,-3.06784532351005));
#76326=CARTESIAN_POINT('Ctrl Pts',(40.7775780044315,1.08612586599699,-3.03421294007396));
#76327=CARTESIAN_POINT('Ctrl Pts',(40.7837353660901,1.17998216472063,-3.00061617025464));
#76328=CARTESIAN_POINT('Ctrl Pts',(40.7898927277486,1.27238093954544,-2.96262368470892));
#76329=CARTESIAN_POINT('Ctrl Pts',(40.7960500894072,1.36288451772775,-2.92038753487238));
#76330=CARTESIAN_POINT('Ctrl Pts',(40.8022029535535,1.4533219895202,-2.87818223552202));
#76331=CARTESIAN_POINT('Ctrl Pts',(40.8083558176998,1.54186662447143,-2.83173961774241));
#76332=CARTESIAN_POINT('Ctrl Pts',(40.8145086818461,1.62810006422018,-2.78126009991627));
#76333=CARTESIAN_POINT('Ctrl Pts',(40.8206592149826,1.71430083446959,-2.73079970623244));
#76334=CARTESIAN_POINT('Ctrl Pts',(40.8268097481192,1.79819177486622,-2.67630567056568));
#76335=CARTESIAN_POINT('Ctrl Pts',(40.8329602812557,1.87937930638694,-2.61802425222238));
#76336=CARTESIAN_POINT('Ctrl Pts',(40.8391101294709,1.96055779689107,-2.5597493240785));
#76337=CARTESIAN_POINT('Ctrl Pts',(40.8452599776861,2.03903312418386,-2.49768810509254));
#76338=CARTESIAN_POINT('Ctrl Pts',(40.8514098259013,2.11444171555594,-2.43212947723119));
#76339=CARTESIAN_POINT('Ctrl Pts',(40.8575606342805,2.18986208032607,-2.3665606138276));
#76340=CARTESIAN_POINT('Ctrl Pts',(40.8637114426596,2.26221443030482,-2.2974935419846));
#76341=CARTESIAN_POINT('Ctrl Pts',(40.8698622510388,2.33116999913079,-2.2252559398084));
#76342=CARTESIAN_POINT('Ctrl Pts',(40.8760196374049,2.40019931254607,-2.15294108306965));
#76343=CARTESIAN_POINT('Ctrl Pts',(40.8821770237711,2.46582429018738,-2.07744923988472));
#76344=CARTESIAN_POINT('Ctrl Pts',(40.8883344101373,2.52775472598571,-1.99914321842056));
#76345=CARTESIAN_POINT('Ctrl Pts',(40.8944952328743,2.58971972449079,-1.9207934952123));
#76346=CARTESIAN_POINT('Ctrl Pts',(40.9006560556112,2.64798582162219,-1.83962681885158));
#76347=CARTESIAN_POINT('Ctrl Pts',(40.9068168783482,2.70230586789131,-1.75603546628768));
#76348=CARTESIAN_POINT('Ctrl Pts',(40.9129880012649,2.75671673096583,-1.67230435869557));
#76349=CARTESIAN_POINT('Ctrl Pts',(40.9191591241816,2.80716814561218,-1.58614085262557));
#76350=CARTESIAN_POINT('Ctrl Pts',(40.9253302470983,2.8534586172673,-1.49796244346878));
#76351=CARTESIAN_POINT('Ctrl Pts',(40.9300257690439,2.88868039593923,-1.4308687133789));
#76352=CARTESIAN_POINT('Ctrl Pts',(40.9347212909895,2.92149415278127,-1.36260898155911));
#76353=CARTESIAN_POINT('Ctrl Pts',(40.9394168129351,2.95183016262558,-1.29337398053071));
#76354=CARTESIAN_POINT('Ctrl Pts',(40.9455890610278,2.99170674739566,-1.20236480029458));
#76355=CARTESIAN_POINT('Ctrl Pts',(40.9517613091206,3.02744065937287,-1.10934952722247));
#76356=CARTESIAN_POINT('Ctrl Pts',(40.9579335572134,3.05882617184256,-1.01474135273526));
#76357=CARTESIAN_POINT('Ctrl Pts',(40.964097445866,3.09016917705901,-0.920261311686526));
#76358=CARTESIAN_POINT('Ctrl Pts',(40.9702613345186,3.11717535282186,-0.824193065864977));
#76359=CARTESIAN_POINT('Ctrl Pts',(40.9764252231712,3.13968634938288,-0.726971244272297));
#76360=CARTESIAN_POINT('Ctrl Pts',(40.9825825848298,3.16217350885833,-0.629852371692754));
#76361=CARTESIAN_POINT('Ctrl Pts',(40.9887399464883,3.18017485498476,-0.531582772707588));
#76362=CARTESIAN_POINT('Ctrl Pts',(40.9948973081469,3.19358164065124,-0.432612837298341));
#76363=CARTESIAN_POINT('Ctrl Pts',(41.0010501722932,3.20697863361983,-0.333715192347285));
#76364=CARTESIAN_POINT('Ctrl Pts',(41.0072030364395,3.21578768029252,-0.234118657158604));
#76365=CARTESIAN_POINT('Ctrl Pts',(41.0133559005858,3.2199511637498,-0.134283526786764));
#76366=CARTESIAN_POINT('Ctrl Pts',(41.0195064337223,3.22411306987328,-0.0344862189085126));
#76367=CARTESIAN_POINT('Ctrl Pts',(41.0256569668589,3.22363289175207,0.0655490710288874));
#76368=CARTESIAN_POINT('Ctrl Pts',(41.0318074999954,3.21850497270214,0.165358105914306));
#76369=CARTESIAN_POINT('Ctrl Pts',(41.0379573482106,3.21337762469559,0.265156026098697));
#76370=CARTESIAN_POINT('Ctrl Pts',(41.0441071964258,3.20360358705455,0.364727307520266));
#76371=CARTESIAN_POINT('Ctrl Pts',(41.050257044641,3.18922928237789,0.463609908137634));
#76372=CARTESIAN_POINT('Ctrl Pts',(41.0564078530202,3.17485273346878,0.562507947104669));
#76373=CARTESIAN_POINT('Ctrl Pts',(41.0625586613993,3.1558745534252,0.660716661802562));
#76374=CARTESIAN_POINT('Ctrl Pts',(41.0687094697784,3.13239262065319,0.757782312130238));
#76375=CARTESIAN_POINT('Ctrl Pts',(41.0748668561446,3.108885575109,0.854951769396925));
#76376=CARTESIAN_POINT('Ctrl Pts',(41.0810242425108,3.08086526103552,0.950975298165107));
#76377=CARTESIAN_POINT('Ctrl Pts',(41.087181628877,3.04847995850393,1.04541260041185));
#76378=CARTESIAN_POINT('Ctrl Pts',(41.0933424516139,3.01607658208504,1.13990260709622));
#76379=CARTESIAN_POINT('Ctrl Pts',(41.0995032743509,2.97930352571704,1.23280422038544));
#76380=CARTESIAN_POINT('Ctrl Pts',(41.1056640970879,2.93835714000737,1.32369742776349));
#76381=CARTESIAN_POINT('Ctrl Pts',(41.1118352200045,2.8973422966988,1.41474259802242));
#76382=CARTESIAN_POINT('Ctrl Pts',(41.1180063429212,2.85214038380119,1.50377226773134));
#76383=CARTESIAN_POINT('Ctrl Pts',(41.1241774658379,2.80299365198577,1.59039119383486));
#76384=CARTESIAN_POINT('Ctrl Pts',(41.1288729877835,2.76559858452276,1.65629833487081));
#76385=CARTESIAN_POINT('Ctrl Pts',(41.133568509729,2.72592062395105,1.72081029555234));
#76386=CARTESIAN_POINT('Ctrl Pts',(41.1382640316746,2.68408251505558,1.78376529141951));
#76387=CARTESIAN_POINT('Ctrl Pts',(41.1444372077828,2.62907819024535,1.86653186793366));
#76388=CARTESIAN_POINT('Ctrl Pts',(41.1506103838911,2.57014515438866,1.94689758370025));
#76389=CARTESIAN_POINT('Ctrl Pts',(41.1567835599993,2.50751985933295,2.02446578571999));
#76390=CARTESIAN_POINT('Ctrl Pts',(41.1629466708,2.44499667425195,2.10190751349096));
#76391=CARTESIAN_POINT('Ctrl Pts',(41.1691097816006,2.37879347784921,2.17656046723111));
#76392=CARTESIAN_POINT('Ctrl Pts',(41.1752728924013,2.3091901603766,2.2480565752934));
#76393=CARTESIAN_POINT('Ctrl Pts',(41.1814302037015,2.23965233977452,2.31948540536517));
#76394=CARTESIAN_POINT('Ctrl Pts',(41.1875875150018,2.16672105554266,2.38776298181445));
#76395=CARTESIAN_POINT('Ctrl Pts',(41.193744826302,2.09071637201169,2.45255430404757));
#76396=CARTESIAN_POINT('Ctrl Pts',(41.1998973678967,2.01477056482111,2.51729543626917));
#76397=CARTESIAN_POINT('Ctrl Pts',(41.2060499094915,1.93575642291291,2.57855540449767));
#76398=CARTESIAN_POINT('Ctrl Pts',(41.2122024510862,1.85402994020835,2.63603690097674));
#76399=CARTESIAN_POINT('Ctrl Pts',(41.2138096173864,1.83268135656855,2.6510522117391));
#76400=CARTESIAN_POINT('Ctrl Pts',(41.2154167836865,1.8111478745415,2.6658099045286));
#76401=CARTESIAN_POINT('Ctrl Pts',(41.2170239499866,1.789436210378,2.68030513402635));
#76402=CARTESIAN_POINT('Ctrl Pts',(39.9670570335907,1.78943621037801,2.68030513402635));
#76403=CARTESIAN_POINT('Ctrl Pts',(39.9732196010882,1.70662368603128,2.73559276820561));
#76404=CARTESIAN_POINT('Ctrl Pts',(39.9793821685857,1.62113340072966,2.78711433407194));
#76405=CARTESIAN_POINT('Ctrl Pts',(39.9855447360832,1.53334353057214,2.83460317853356));
#76406=CARTESIAN_POINT('Ctrl Pts',(39.9917011085207,1.44564191316245,2.88204428376277));
#76407=CARTESIAN_POINT('Ctrl Pts',(39.9978574809582,1.35564568716505,2.92546052205229));
#76408=CARTESIAN_POINT('Ctrl Pts',(40.0040138533957,1.26376118638599,2.9646290200098));
#76409=CARTESIAN_POINT('Ctrl Pts',(40.0101661718499,1.17193719172973,3.00377172543509));
#76410=CARTESIAN_POINT('Ctrl Pts',(40.0163184903041,1.07822779268038,3.03867208115502));
#76411=CARTESIAN_POINT('Ctrl Pts',(40.0224708087583,0.98306224853093,3.06915398408312));
#76412=CARTESIAN_POINT('Ctrl Pts',(40.0286210952501,0.887928135266615,3.0996258195735));
#76413=CARTESIAN_POINT('Ctrl Pts',(40.0347713817419,0.791339245884843,3.12568196966969));
#76414=CARTESIAN_POINT('Ctrl Pts',(40.0409216682336,0.693742194816822,3.1471954705151));
#76415=CARTESIAN_POINT('Ctrl Pts',(40.0470715685711,0.596151271515395,3.16870762060543));
#76416=CARTESIAN_POINT('Ctrl Pts',(40.0532214689085,0.497552736670877,3.18567759527323));
#76417=CARTESIAN_POINT('Ctrl Pts',(40.059371369246,0.398404664873244,3.19802928152749));
#76418=CARTESIAN_POINT('Ctrl Pts',(40.065522528474,0.299236297370409,3.21038349618375));
#76419=CARTESIAN_POINT('Ctrl Pts',(40.0716736877019,0.199518600493762,3.21811749073813));
#76420=CARTESIAN_POINT('Ctrl Pts',(40.0778248469298,0.0997150502907764,
3.22120698981694));
#76421=CARTESIAN_POINT('Ctrl Pts',(40.083982747012,-0.000197871358417603,
3.22429987457673));
#76422=CARTESIAN_POINT('Ctrl Pts',(40.0901406470941,-0.100196399287679,
3.22273808918772));
#76423=CARTESIAN_POINT('Ctrl Pts',(40.0962985471763,-0.199816923963555,
3.21654951141713));
#76424=CARTESIAN_POINT('Ctrl Pts',(40.1024601521362,-0.299497384959231,
3.21035721031163));
#76425=CARTESIAN_POINT('Ctrl Pts',(40.1086217570962,-0.398798958333763,
3.19953262122687));
#76426=CARTESIAN_POINT('Ctrl Pts',(40.1147833620561,-0.497265089790132,
3.1841553028984));
#76427=CARTESIAN_POINT('Ctrl Pts',(40.1209549333014,-0.595890488445507,
3.16875311203374));
#76428=CARTESIAN_POINT('Ctrl Pts',(40.1271265045467,-0.693677321720815,
3.14878357472114));
#76429=CARTESIAN_POINT('Ctrl Pts',(40.1332980757919,-0.790181112498599,
3.12437695740294));
#76430=CARTESIAN_POINT('Ctrl Pts',(40.1368746965201,-0.846108111430506,
3.11023255074612));
#76431=CARTESIAN_POINT('Ctrl Pts',(40.1404513172483,-0.90160449120352,3.09459884785688));
#76432=CARTESIAN_POINT('Ctrl Pts',(40.1440279379765,-0.956586756639631,
3.07750862541792));
#76433=CARTESIAN_POINT('Ctrl Pts',(40.1502001860692,-1.05147078510283,3.04801567638282));
#76434=CARTESIAN_POINT('Ctrl Pts',(40.156372434162,-1.1451565765698,3.01407858801189));
#76435=CARTESIAN_POINT('Ctrl Pts',(40.1625446822548,-1.23719717747275,2.97581261280906));
#76436=CARTESIAN_POINT('Ctrl Pts',(40.1687085709074,-1.32911312235386,2.93759846347648));
#76437=CARTESIAN_POINT('Ctrl Pts',(40.17487245956,-1.41938790786098,2.89506724569189));
#76438=CARTESIAN_POINT('Ctrl Pts',(40.1810363482126,-1.50758942075117,2.84838405081533));
#76439=CARTESIAN_POINT('Ctrl Pts',(40.1871937098712,-1.59569753630974,2.80175028917059));
#76440=CARTESIAN_POINT('Ctrl Pts',(40.1933510715297,-1.68173636212607,2.75097349329647));
#76441=CARTESIAN_POINT('Ctrl Pts',(40.1995084331883,-1.76529437220314,2.69626655617873));
#76442=CARTESIAN_POINT('Ctrl Pts',(40.2056612973346,-1.84879134913088,2.64159957856528));
#76443=CARTESIAN_POINT('Ctrl Pts',(40.2118141614809,-1.92981075068336,2.5830084043413));
#76444=CARTESIAN_POINT('Ctrl Pts',(40.2179670256272,-2.00796706315876,2.52075104597213));
#76445=CARTESIAN_POINT('Ctrl Pts',(40.2241175587638,-2.0860937661509,2.45851727377472));
#76446=CARTESIAN_POINT('Ctrl Pts',(40.2302680919003,-2.16135919593939,2.39262034757435));
#76447=CARTESIAN_POINT('Ctrl Pts',(40.2364186250368,-2.23340890014565,2.32336012000942));
#76448=CARTESIAN_POINT('Ctrl Pts',(40.242568473252,-2.30545058092077,2.25410760524044));
#76449=CARTESIAN_POINT('Ctrl Pts',(40.2487183214672,-2.37427693492087,2.18149283476765));
#76450=CARTESIAN_POINT('Ctrl Pts',(40.2548681696825,-2.43956928588356,2.10585357085282));
#76451=CARTESIAN_POINT('Ctrl Pts',(40.2610189780616,-2.50487183081491,2.03020249752581));
#76452=CARTESIAN_POINT('Ctrl Pts',(40.2671697864407,-2.56663899291463,1.95152632167501));
#76453=CARTESIAN_POINT('Ctrl Pts',(40.2733205948199,-2.62459207753573,1.87019624345593));
#76454=CARTESIAN_POINT('Ctrl Pts',(40.279477981186,-2.68260714013062,1.78877918671812));
#76455=CARTESIAN_POINT('Ctrl Pts',(40.2856353675522,-2.73679972740451,1.70470291442654));
#76456=CARTESIAN_POINT('Ctrl Pts',(40.2917927539184,-2.78693431929228,1.61836790083432));
#76457=CARTESIAN_POINT('Ctrl Pts',(40.2979535766554,-2.83709689075378,1.53198470460438));
#76458=CARTESIAN_POINT('Ctrl Pts',(40.3041143993923,-2.88319675624035,1.44334064203683));
#76459=CARTESIAN_POINT('Ctrl Pts',(40.3102752221293,-2.9250452135613,1.35285921703707));
#76460=CARTESIAN_POINT('Ctrl Pts',(40.316446345046,-2.96696363664015,1.26222651760853));
#76461=CARTESIAN_POINT('Ctrl Pts',(40.3226174679627,-3.00461628994125,1.16975072230248));
#76462=CARTESIAN_POINT('Ctrl Pts',(40.3287885908793,-3.03786325502638,1.07587378732849));
#76463=CARTESIAN_POINT('Ctrl Pts',(40.3334841128249,-3.06316041022609,1.0044441278805));
#76464=CARTESIAN_POINT('Ctrl Pts',(40.3381796347704,-3.08590791362778,0.932203663353661));
#76465=CARTESIAN_POINT('Ctrl Pts',(40.342875156716,-3.10606394303052,0.859351118173287));
#76466=CARTESIAN_POINT('Ctrl Pts',(40.350710863735,-3.13969955221256,0.737777583592601));
#76467=CARTESIAN_POINT('Ctrl Pts',(40.358546570754,-3.16621377910518,0.614154268083113));
#76468=CARTESIAN_POINT('Ctrl Pts',(40.366382277773,-3.18540180604714,0.489216615142617));
#76469=CARTESIAN_POINT('Ctrl Pts',(40.3740772191688,-3.20424512707252,0.366523421640472));
#76470=CARTESIAN_POINT('Ctrl Pts',(40.3817721605646,-3.21602311411887,0.242562533622061));
#76471=CARTESIAN_POINT('Ctrl Pts',(40.3894671019604,-3.22058710117146,0.118052048978578));
#76472=CARTESIAN_POINT('Ctrl Pts',(40.3918358843862,-3.2219920621407,0.0797231998450655));
#76473=CARTESIAN_POINT('Ctrl Pts',(40.394204666812,-3.22271373114598,0.041342434832041));
#76474=CARTESIAN_POINT('Ctrl Pts',(40.3965734492378,-3.22274866702434,0.00293115895943825));
#76475=CARTESIAN_POINT('Ctrl Pts',(39.7209886430068,1.78943588752252,2.68030534957241));
#76476=CARTESIAN_POINT('Ctrl Pts',(39.7321640893856,1.65207849352263,2.77200842746209));
#76477=CARTESIAN_POINT('Ctrl Pts',(39.7433052749528,1.50777340075562,2.85308531584831));
#76478=CARTESIAN_POINT('Ctrl Pts',(39.7551126764817,1.34071459180183,2.93069196149534));
#76479=CARTESIAN_POINT('Ctrl Pts',(39.7563102948743,1.32359539338073,2.93846324837295));
#76480=CARTESIAN_POINT('Ctrl Pts',(39.7583549276396,1.29404934284328,2.95156511911777));
#76481=CARTESIAN_POINT('Ctrl Pts',(39.7592059182603,1.28165533818344,2.95696803556938));
#76482=CARTESIAN_POINT('Ctrl Pts',(39.7604085383861,1.2639964284272,2.96453419246989));
#76483=CARTESIAN_POINT('Ctrl Pts',(39.7607639649647,1.25875943674085,2.96676164040834));
#76484=CARTESIAN_POINT('Ctrl Pts',(39.761374413209,1.24973325804424,2.97057253921833));
#76485=CARTESIAN_POINT('Ctrl Pts',(39.7616298392038,1.24594690659992,2.97216263580712));
#76486=CARTESIAN_POINT('Ctrl Pts',(39.7621216805988,1.23863729880266,2.97521591792621));
#76487=CARTESIAN_POINT('Ctrl Pts',(39.7623581571592,1.2351144887013,2.97668008298311));
#76488=CARTESIAN_POINT('Ctrl Pts',(39.7629221835489,1.22669241690849,2.98016297448509));
#76489=CARTESIAN_POINT('Ctrl Pts',(39.7632493804315,1.22179074068081,2.98217588802622));
#76490=CARTESIAN_POINT('Ctrl Pts',(39.7644165006735,1.20425030818957,2.98932850500378));
#76491=CARTESIAN_POINT('Ctrl Pts',(39.7652523952585,1.19158368682434,2.99440011491901));
#76492=CARTESIAN_POINT('Ctrl Pts',(39.7698296790476,1.12167643902437,3.02187655862792));
#76493=CARTESIAN_POINT('Ctrl Pts',(39.773484692314,1.06383198131068,3.04272223631978));
#76494=CARTESIAN_POINT('Ctrl Pts',(39.795127554147,0.711980781055297,3.15825797778673));
#76495=CARTESIAN_POINT('Ctrl Pts',(39.8116408571957,0.40619440215225,3.21193950109201));
#76496=CARTESIAN_POINT('Ctrl Pts',(39.8337766245109,0.0220881041297611,
3.22355534523597));
#76497=CARTESIAN_POINT('Ctrl Pts',(39.8381771210486,-0.0532913925965058,
3.223190309908));
#76498=CARTESIAN_POINT('Ctrl Pts',(39.845355665513,-0.173954576437729,3.21837210993128));
#76499=CARTESIAN_POINT('Ctrl Pts',(39.8480824355653,-0.219278834458008,
3.21560192051278));
#76500=CARTESIAN_POINT('Ctrl Pts',(39.8516275874507,-0.277465623360148,
3.21080969746222));
#76501=CARTESIAN_POINT('Ctrl Pts',(39.8524182724492,-0.290396750720803,
3.20966599585087));
#76502=CARTESIAN_POINT('Ctrl Pts',(39.8536980370717,-0.311249635632164,
3.20769460211176));
#76503=CARTESIAN_POINT('Ctrl Pts',(39.8541855793026,-0.319175939296277,
3.20691560756914));
#76504=CARTESIAN_POINT('Ctrl Pts',(39.8551175969417,-0.334293838818497,
3.20537322213585));
#76505=CARTESIAN_POINT('Ctrl Pts',(39.8555619068705,-0.341485921281881,
3.20461498905343));
#76506=CARTESIAN_POINT('Ctrl Pts',(39.8565795919936,-0.357924835355587,
3.20282593050606));
#76507=CARTESIAN_POINT('Ctrl Pts',(39.8571534643796,-0.367169845094468,
3.20177926016639));
#76508=CARTESIAN_POINT('Ctrl Pts',(39.8589214268339,-0.395574015047169,
3.19843885285245));
#76509=CARTESIAN_POINT('Ctrl Pts',(39.8601196768224,-0.414716941435674,
3.19601309903595));
#76510=CARTESIAN_POINT('Ctrl Pts',(39.8771109014239,-0.684604954247868,
3.15934787544266));
#76511=CARTESIAN_POINT('Ctrl Pts',(39.8938857735702,-0.930434109965115,
3.09586880912285));
#76512=CARTESIAN_POINT('Ctrl Pts',(39.9210651089218,-1.30517274953995,2.95039773149168));
#76513=CARTESIAN_POINT('Ctrl Pts',(39.9311970063851,-1.44018412841049,2.88690068275874));
#76514=CARTESIAN_POINT('Ctrl Pts',(39.9448108739191,-1.61990250625762,2.7866211036197));
#76515=CARTESIAN_POINT('Ctrl Pts',(39.9485234945605,-1.66874766446562,2.75764815298731));
#76516=CARTESIAN_POINT('Ctrl Pts',(39.9541595951937,-1.7430138315697,2.71090011792678));
#76517=CARTESIAN_POINT('Ctrl Pts',(39.9561288307718,-1.76898510473167,2.69402459828752));
#76518=CARTESIAN_POINT('Ctrl Pts',(39.9585628124718,-1.80116703696282,2.67244743629182));
#76519=CARTESIAN_POINT('Ctrl Pts',(39.959049661314,-1.80760827127583,2.66809488874902));
#76520=CARTESIAN_POINT('Ctrl Pts',(39.9598192718702,-1.81779825600206,2.66115535185934));
#76521=CARTESIAN_POINT('Ctrl Pts',(39.9601030542853,-1.82155732915326,2.65858368374509));
#76522=CARTESIAN_POINT('Ctrl Pts',(39.9606372087027,-1.82863632131726,2.65371872049736));
#76523=CARTESIAN_POINT('Ctrl Pts',(39.9608876910953,-1.83195734605558,2.65142718655085));
#76524=CARTESIAN_POINT('Ctrl Pts',(39.9614609800611,-1.83956148105148,2.64615916445889));
#76525=CARTESIAN_POINT('Ctrl Pts',(39.9617834979445,-1.84384166729123,2.64317851706781));
#76526=CARTESIAN_POINT('Ctrl Pts',(39.9627790960626,-1.85706067625363,2.63392529387039));
#76527=CARTESIAN_POINT('Ctrl Pts',(39.963449812422,-1.86597498209866,2.62761758693435));
#76528=CARTESIAN_POINT('Ctrl Pts',(39.9690104295967,-1.93993329092643,2.57471897120221));
#76529=CARTESIAN_POINT('Ctrl Pts',(39.9737457158652,-2.00325973037467,2.52576162974706));
#76530=CARTESIAN_POINT('Ctrl Pts',(39.9802377061916,-2.08921353965109,2.4540422427841));
#76531=CARTESIAN_POINT('Ctrl Pts',(39.9820734717929,-2.1134189107674,2.43322772275074));
#76532=CARTESIAN_POINT('Ctrl Pts',(39.984442657204,-2.14444990185094,2.40573131178357));
#76533=CARTESIAN_POINT('Ctrl Pts',(39.9849866120418,-2.15156012702867,2.39937440764058));
#76534=CARTESIAN_POINT('Ctrl Pts',(39.9935368542357,-2.26307276256311,2.29878214887312));
#76535=CARTESIAN_POINT('Ctrl Pts',(40.0013350345454,-2.36122813691671,2.19784031840064));
#76536=CARTESIAN_POINT('Ctrl Pts',(40.0160780481415,-2.53204057285876,1.99748041896476));
#76537=CARTESIAN_POINT('Ctrl Pts',(40.022991553198,-2.6062074553478,1.89969401693332));
#76538=CARTESIAN_POINT('Ctrl Pts',(40.0340514732086,-2.71290453514553,1.7409699015081));
#76539=CARTESIAN_POINT('Ctrl Pts',(40.0380717589711,-2.74935936884235,1.68280995410925));
#76540=CARTESIAN_POINT('Ctrl Pts',(40.0446805891996,-2.80527280392049,1.58693327420948));
#76541=CARTESIAN_POINT('Ctrl Pts',(40.0472276962569,-2.82589265080441,1.54991715612698));
#76542=CARTESIAN_POINT('Ctrl Pts',(40.0505702291102,-2.85171964725375,1.50132374843055));
#76543=CARTESIAN_POINT('Ctrl Pts',(40.0513417524742,-2.85759718966642,1.49010611655001));
#76544=CARTESIAN_POINT('Ctrl Pts',(40.0525979907795,-2.86703072503994,1.47184058141011));
#76545=CARTESIAN_POINT('Ctrl Pts',(40.0530812707732,-2.87062724589319,1.46481367033135));
#76546=CARTESIAN_POINT('Ctrl Pts',(40.0540102312467,-2.87747781722077,1.45130684268854));
#76547=CARTESIAN_POINT('Ctrl Pts',(40.0544557666593,-2.88073588992689,1.44482901111179));
#76548=CARTESIAN_POINT('Ctrl Pts',(40.0554738934587,-2.88811832588831,1.43002671483367));
#76549=CARTESIAN_POINT('Ctrl Pts',(40.0560469742298,-2.89222859688077,1.42169532951318));
#76550=CARTESIAN_POINT('Ctrl Pts',(40.0575625815878,-2.90297961901785,1.39966377663986));
#76551=CARTESIAN_POINT('Ctrl Pts',(40.0585072245931,-2.90955934924733,1.38593424680419));
#76552=CARTESIAN_POINT('Ctrl Pts',(40.0648607561466,-2.95300078443222,1.29361473809033));
#76553=CARTESIAN_POINT('Ctrl Pts',(40.0703755633625,-2.98676846181998,1.21361630870205));
#76554=CARTESIAN_POINT('Ctrl Pts',(40.0791170094146,-3.03423501618327,1.08713768970816));
#76555=CARTESIAN_POINT('Ctrl Pts',(40.0822723159697,-3.05018660176374,1.04154300420082));
#76556=CARTESIAN_POINT('Ctrl Pts',(40.0919197984805,-3.09543302362643,0.902246194701879));
#76557=CARTESIAN_POINT('Ctrl Pts',(40.0984903261723,-3.1214757690063,0.807552294098496));
#76558=CARTESIAN_POINT('Ctrl Pts',(40.1111536476425,-3.16294652745497,0.62443225562779));
#76559=CARTESIAN_POINT('Ctrl Pts',(40.1172324921037,-3.17908434152186,0.536254539451549));
#76560=CARTESIAN_POINT('Ctrl Pts',(40.1334068397218,-3.21233564652255,0.29912008265209));
#76561=CARTESIAN_POINT('Ctrl Pts',(40.1434412181666,-3.22277104870652,0.149431934785481));
#76562=CARTESIAN_POINT('Ctrl Pts',(40.1532596875225,-3.22274939918938,-0.00449845971419938));
#76563=CARTESIAN_POINT('Ctrl Pts',(40.1535173518547,-3.22274121395295,-0.00854367477969973));
#76564=CARTESIAN_POINT('Ctrl Pts',(40.1549633833723,-3.22265240666992,-0.0312781304336692));
#76565=CARTESIAN_POINT('Ctrl Pts',(40.1561442502217,-3.22241682628457,-0.0499669135980986));
#76566=CARTESIAN_POINT('Ctrl Pts',(40.1577369736299,-3.22187581434776,-0.0753576160558248));
#76567=CARTESIAN_POINT('Ctrl Pts',(40.1581564135566,-3.22171203037629,-0.0820617366684774));
#76568=CARTESIAN_POINT('Ctrl Pts',(40.1588170773794,-3.22142028134979,-0.0926500716955674));
#76569=CARTESIAN_POINT('Ctrl Pts',(40.159059073807,-3.22130621576293,-0.0965346028457733));
#76570=CARTESIAN_POINT('Ctrl Pts',(40.1595534136852,-3.22105844474806,-0.104482468912272));
#76571=CARTESIAN_POINT('Ctrl Pts',(40.1598057146607,-3.22092407735302,-0.108545745477598));
#76572=CARTESIAN_POINT('Ctrl Pts',(40.1603948283916,-3.22059180932549,-0.118049115324318));
#76573=CARTESIAN_POINT('Ctrl Pts',(40.1607312979975,-3.22038781238382,-0.123489006818093));
#76574=CARTESIAN_POINT('Ctrl Pts',(40.1618147005343,-3.21968499538193,-0.141042859973687));
#76575=CARTESIAN_POINT('Ctrl Pts',(40.1625586274475,-3.21913159162467,-0.153154707761682));
#76576=CARTESIAN_POINT('Ctrl Pts',(40.1734342361561,-3.20999858588507,-0.331020313197249));
#76577=CARTESIAN_POINT('Ctrl Pts',(40.1828943525046,-3.18869358329005,-0.495898031008083));
#76578=CARTESIAN_POINT('Ctrl Pts',(40.2052022722087,-3.10758913342228,-0.884504162717305));
#76579=CARTESIAN_POINT('Ctrl Pts',(40.2179033156276,-3.03624216669502,-1.10484698250114));
#76580=CARTESIAN_POINT('Ctrl Pts',(40.232463044738,-2.9340152452497,-1.33343571890868));
#76581=CARTESIAN_POINT('Ctrl Pts',(40.2335989802135,-2.92590993950567,-1.35112815118152));
#76582=CARTESIAN_POINT('Ctrl Pts',(40.2389444749062,-2.88717885999298,-1.43368806582139));
#76583=CARTESIAN_POINT('Ctrl Pts',(40.2432129677869,-2.85455491213075,-1.49759083614846));
#76584=CARTESIAN_POINT('Ctrl Pts',(40.2484251808164,-2.81288876547299,-1.57288898835381));
#76585=CARTESIAN_POINT('Ctrl Pts',(40.2492961739722,-2.80586606497999,-1.58538279026992));
#76586=CARTESIAN_POINT('Ctrl Pts',(40.2507262742465,-2.79423896158135,-1.60574884466103));
#76587=CARTESIAN_POINT('Ctrl Pts',(40.2512835952119,-2.78968401802936,-1.61364921944192));
#76588=CARTESIAN_POINT('Ctrl Pts',(40.2522837541382,-2.78146770122346,-1.62776133998531));
#76589=CARTESIAN_POINT('Ctrl Pts',(40.2527261338012,-2.77781888384923,-1.633980354866));
#76590=CARTESIAN_POINT('Ctrl Pts',(40.25366508845,-2.77004343205775,-1.64713145491186));
#76591=CARTESIAN_POINT('Ctrl Pts',(40.2541618517358,-2.76591158317992,-1.65406038504825));
#76592=CARTESIAN_POINT('Ctrl Pts',(40.2554889614952,-2.7548252883459,-1.67249392026445));
#76593=CARTESIAN_POINT('Ctrl Pts',(40.2563209911938,-2.74782485695075,-1.68397055477577));
#76594=CARTESIAN_POINT('Ctrl Pts',(40.2602726473932,-2.71434397937894,-1.73809504149306));
#76595=CARTESIAN_POINT('Ctrl Pts',(40.2634262196891,-2.6869424379776,-1.78016220835584));
#76596=CARTESIAN_POINT('Ctrl Pts',(40.2721129236422,-2.60967459658906,-1.89293414604569));
#76597=CARTESIAN_POINT('Ctrl Pts',(40.2777145263074,-2.5579287623426,-1.96229443688133));
#76598=CARTESIAN_POINT('Ctrl Pts',(40.2942306478675,-2.39978927835302,-2.15736650156583));
#76599=CARTESIAN_POINT('Ctrl Pts',(40.3053632637638,-2.28648053238194,-2.27710719947868));
#76600=CARTESIAN_POINT('Ctrl Pts',(40.3294825645016,-2.02244628362454,-2.51646754733987));
#76601=CARTESIAN_POINT('Ctrl Pts',(40.3424267680697,-1.86912696070829,-2.6323526470295));
#76602=CARTESIAN_POINT('Ctrl Pts',(40.3552784665909,-1.69644741089108,-2.74013160812073));
#76603=CARTESIAN_POINT('Ctrl Pts',(40.3560154855263,-1.68646652163516,-2.74628580616083));
#76604=CARTESIAN_POINT('Ctrl Pts',(40.357081318219,-1.67191536327321,-2.75514877966776));
#76605=CARTESIAN_POINT('Ctrl Pts',(40.3574129033277,-1.66737177568941,-2.75790085801732));
#76606=CARTESIAN_POINT('Ctrl Pts',(40.357996590674,-1.6593438713714,-2.76273631738093));
#76607=CARTESIAN_POINT('Ctrl Pts',(40.3582489983676,-1.6558623978749,-2.76482436383795));
#76608=CARTESIAN_POINT('Ctrl Pts',(40.3587774806738,-1.648552038456,-2.76919005964107));
#76609=CARTESIAN_POINT('Ctrl Pts',(40.3590534659245,-1.64472238179449,-2.77146634424997));
#76610=CARTESIAN_POINT('Ctrl Pts',(40.3597820659308,-1.63458070616443,-2.77746596409681));
#76611=CARTESIAN_POINT('Ctrl Pts',(40.3602338013023,-1.62826064141315,-2.78117575007049));
#76612=CARTESIAN_POINT('Ctrl Pts',(40.3622881471307,-1.59937541813454,-2.79799874389221));
#76613=CARTESIAN_POINT('Ctrl Pts',(40.3638749654213,-1.57666336613366,-2.81085955370472));
#76614=CARTESIAN_POINT('Ctrl Pts',(40.3777767152751,-1.37443104822405,-2.92215199374848));
#76615=CARTESIAN_POINT('Ctrl Pts',(40.3891730298433,-1.18604078291829,-3.0035585449422));
#76616=CARTESIAN_POINT('Ctrl Pts',(40.4151573245859,-0.743570310688917,
-3.14657508117909));
#76617=CARTESIAN_POINT('Ctrl Pts',(40.429741305321,-0.487223245393259,-3.19631363224641));
#76618=CARTESIAN_POINT('Ctrl Pts',(40.4466146206631,-0.208642366108974,
-3.21604586022124));
#76619=CARTESIAN_POINT('Ctrl Pts',(40.4477741550401,-0.189572546063888,
-3.21722626456615));
#76620=CARTESIAN_POINT('Ctrl Pts',(40.4495039975292,-0.161239837601685,
-3.21872725638837));
#76621=CARTESIAN_POINT('Ctrl Pts',(40.4500702290144,-0.151984011269613,
-3.21917758033607));
#76622=CARTESIAN_POINT('Ctrl Pts',(40.4510803128522,-0.135506213327811,
-3.21990805192836));
#76623=CARTESIAN_POINT('Ctrl Pts',(40.4515236708843,-0.128284970629541,
-3.22020383852983));
#76624=CARTESIAN_POINT('Ctrl Pts',(40.4524584301396,-0.11308432075495,-3.22077525537431));
#76625=CARTESIAN_POINT('Ctrl Pts',(40.4529499966037,-0.105104772061585,
-3.22104552813038));
#76626=CARTESIAN_POINT('Ctrl Pts',(40.4542487147636,-0.0840605483293663,
-3.221680028338));
#76627=CARTESIAN_POINT('Ctrl Pts',(40.4550574248883,-0.070994620734794,
-3.22199443458799));
#76628=CARTESIAN_POINT('Ctrl Pts',(40.4587415268159,-0.0116500550169357,
-3.22306129538118));
#76629=CARTESIAN_POINT('Ctrl Pts',(40.46164553474,0.0346376632234874,-3.22289616805717));
#76630=CARTESIAN_POINT('Ctrl Pts',(40.4694858358697,0.158237804464938,-3.21979233221754));
#76631=CARTESIAN_POINT('Ctrl Pts',(40.4744753989489,0.235471089690614,-3.21506666361623));
#76632=CARTESIAN_POINT('Ctrl Pts',(40.5005415847875,0.631841109465753,-3.17645556664471));
#76633=CARTESIAN_POINT('Ctrl Pts',(40.5228919993727,0.944731889723517,-3.09782676973865));
#76634=CARTESIAN_POINT('Ctrl Pts',(40.5472481070167,1.28957260569195,-2.95396507278737));
#76635=CARTESIAN_POINT('Ctrl Pts',(40.5506424418291,1.33781368246407,-2.93243286136286));
#76636=CARTESIAN_POINT('Ctrl Pts',(40.5545227692339,1.39343490157475,-2.90594801100087));
#76637=CARTESIAN_POINT('Ctrl Pts',(40.5550739861872,1.40134760085045,-2.90214051578807));
#76638=CARTESIAN_POINT('Ctrl Pts',(40.5559522194027,1.41397469943223,-2.89600082417691));
#76639=CARTESIAN_POINT('Ctrl Pts',(40.5562804905998,1.41869905510866,-2.89368937798069));
#76640=CARTESIAN_POINT('Ctrl Pts',(40.5568603756229,1.42705297517178,-2.88957674858487));
#76641=CARTESIAN_POINT('Ctrl Pts',(40.5571122818836,1.43068482412014,-2.88778027465099));
#76642=CARTESIAN_POINT('Ctrl Pts',(40.5576418889508,1.43832655203853,-2.88398238142146));
#76643=CARTESIAN_POINT('Ctrl Pts',(40.5579194924392,1.44233563624463,-2.88197945163579));
#76644=CARTESIAN_POINT('Ctrl Pts',(40.5586569867131,1.45299526787946,-2.87662610855585));
#76645=CARTESIAN_POINT('Ctrl Pts',(40.5591159592597,1.45963845143871,-2.87326097154096));
#76646=CARTESIAN_POINT('Ctrl Pts',(40.5612519216748,1.4905937985297,-2.85744532408666));
#76647=CARTESIAN_POINT('Ctrl Pts',(40.5629115443202,1.51475957980463,-2.84470862899866));
#76648=CARTESIAN_POINT('Ctrl Pts',(40.5674200810938,1.58060693933868,-2.8089263768702));
#76649=CARTESIAN_POINT('Ctrl Pts',(40.5702353299041,1.62194553998349,-2.78526100055333));
#76650=CARTESIAN_POINT('Ctrl Pts',(40.5798571320635,1.7632305747261,-2.70016579764916));
#76651=CARTESIAN_POINT('Ctrl Pts',(40.5864726965714,1.86034265937294,-2.63419938371192));
#76652=CARTESIAN_POINT('Ctrl Pts',(40.6086673725955,2.17542565024408,-2.39403485653286));
#76653=CARTESIAN_POINT('Ctrl Pts',(40.624065525291,2.37429938472125,-2.19694446055123));
#76654=CARTESIAN_POINT('Ctrl Pts',(40.6411699478432,2.54955873791154,-1.97127255671639));
#76655=CARTESIAN_POINT('Ctrl Pts',(40.6415839925144,2.5537768843949,-1.9658048922904));
#76656=CARTESIAN_POINT('Ctrl Pts',(40.6436440090588,2.57464216134981,-1.93857831450175));
#76657=CARTESIAN_POINT('Ctrl Pts',(40.6452997806274,2.59102854793722,-1.91662180239494));
#76658=CARTESIAN_POINT('Ctrl Pts',(40.6476387204415,2.61362797561477,-1.88552073956487));
#76659=CARTESIAN_POINT('Ctrl Pts',(40.6483127190886,2.6200772364769,-1.8765486735939));
#76660=CARTESIAN_POINT('Ctrl Pts',(40.6494036999365,2.63041413662276,-1.86201104154659));
#76661=CARTESIAN_POINT('Ctrl Pts',(40.649819570041,2.63433059014064,-1.85646599476481));
#76662=CARTESIAN_POINT('Ctrl Pts',(40.6506854709005,2.64243548212905,-1.84491352570061));
#76663=CARTESIAN_POINT('Ctrl Pts',(40.651135609418,2.64662101863044,-1.83890412389011));
#76664=CARTESIAN_POINT('Ctrl Pts',(40.6521967464161,2.65642227213904,-1.8247291544925));
#76665=CARTESIAN_POINT('Ctrl Pts',(40.6528083925193,2.66202085535789,-1.81655188125583));
#76666=CARTESIAN_POINT('Ctrl Pts',(40.6548154562938,2.68022499985389,-1.78969808206011));
#76667=CARTESIAN_POINT('Ctrl Pts',(40.6562168332792,2.69267219978799,-1.77091548575454));
#76668=CARTESIAN_POINT('Ctrl Pts',(40.6595210634323,2.72140099637895,-1.72656106798935));
#76669=CARTESIAN_POINT('Ctrl Pts',(40.6614297800688,2.73752054144332,-1.7008873239692));
#76670=CARTESIAN_POINT('Ctrl Pts',(40.6682079940824,2.79308561534073,-1.60955193073903));
#76671=CARTESIAN_POINT('Ctrl Pts',(40.6731468101554,2.83054765639472,-1.54271938521902));
#76672=CARTESIAN_POINT('Ctrl Pts',(40.6988518094608,3.0103220083431,-1.19336850452782));
#76673=CARTESIAN_POINT('Ctrl Pts',(40.7208555206752,3.11283674851488,-0.892396047288326));
#76674=CARTESIAN_POINT('Ctrl Pts',(40.7453280723297,3.18035920336323,-0.524219604486452));
#76675=CARTESIAN_POINT('Ctrl Pts',(40.7490690828834,3.18929075771276,-0.466815096782614));
#76676=CARTESIAN_POINT('Ctrl Pts',(40.7533537576054,3.19792481167503,-0.399365365385379));
#76677=CARTESIAN_POINT('Ctrl Pts',(40.7539758882693,3.19913792113715,-0.389528386398443));
#76678=CARTESIAN_POINT('Ctrl Pts',(40.7549131335055,3.2009042221205,-0.374640542904753));
#76679=CARTESIAN_POINT('Ctrl Pts',(40.7552300930692,3.20149086912764,-0.369593819368888));
#76680=CARTESIAN_POINT('Ctrl Pts',(40.7557967234085,3.20252048668558,-0.360549951750163));
#76681=CARTESIAN_POINT('Ctrl Pts',(40.7560466434655,3.20296791047684,-0.356553362634048));
#76682=CARTESIAN_POINT('Ctrl Pts',(40.7565840991829,3.20391564204478,-0.347942044669304));
#76683=CARTESIAN_POINT('Ctrl Pts',(40.7568714922465,3.20441345960861,-0.343327086484151));
#76684=CARTESIAN_POINT('Ctrl Pts',(40.757663008082,3.20575966164574,-0.33058925324667));
#76685=CARTESIAN_POINT('Ctrl Pts',(40.7581659618445,3.20658714953274,-0.322464135140428));
#76686=CARTESIAN_POINT('Ctrl Pts',(40.7608792923255,3.21089886576763,-0.278468745051941));
#76687=CARTESIAN_POINT('Ctrl Pts',(40.7630588437274,3.21381227257893,-0.242543404083277));
#76688=CARTESIAN_POINT('Ctrl Pts',(40.7694300811919,3.22064938085066,-0.136097907349347));
#76689=CARTESIAN_POINT('Ctrl Pts',(40.7735443335696,3.22285867264353,-0.0654860679921393));
#76690=CARTESIAN_POINT('Ctrl Pts',(40.7851490907652,3.22253574423974,0.136756083327457));
#76691=CARTESIAN_POINT('Ctrl Pts',(40.7924801727759,3.21426376028516,0.268236180175631));
#76692=CARTESIAN_POINT('Ctrl Pts',(40.8138452931435,3.16694963893702,0.647602796871585));
#76693=CARTESIAN_POINT('Ctrl Pts',(40.8279412604807,3.10701481029392,0.891849082088748));
#76694=CARTESIAN_POINT('Ctrl Pts',(40.8442509722197,3.01262235035659,1.14481404581125));
#76695=CARTESIAN_POINT('Ctrl Pts',(40.8454261461252,3.00568853246721,1.16289683368949));
#76696=CARTESIAN_POINT('Ctrl Pts',(40.8471748513558,2.99517789057144,1.18958555396114));
#76697=CARTESIAN_POINT('Ctrl Pts',(40.8477441738693,2.99172595483258,1.19824045778308));
#76698=CARTESIAN_POINT('Ctrl Pts',(40.8487577344429,2.98552762102993,1.21358753838897));
#76699=CARTESIAN_POINT('Ctrl Pts',(40.8492014656553,2.98279612303558,1.22028569454622));
#76700=CARTESIAN_POINT('Ctrl Pts',(40.8501349334438,2.97701255840337,1.23433265755208));
#76701=CARTESIAN_POINT('Ctrl Pts',(40.8506248276797,2.97395578238756,1.24167946144719));
#76702=CARTESIAN_POINT('Ctrl Pts',(40.851914411466,2.96585308455963,1.26095231278851));
#76703=CARTESIAN_POINT('Ctrl Pts',(40.8527156201121,2.96076247407987,1.27285930822398));
#76704=CARTESIAN_POINT('Ctrl Pts',(40.8563177057992,2.9376253775773,1.32608740641049));
#76705=CARTESIAN_POINT('Ctrl Pts',(40.8591456624544,2.91878537458856,1.3670560605923));
#76706=CARTESIAN_POINT('Ctrl Pts',(40.8667336472173,2.86648734871734,1.47476796981538));
#76707=CARTESIAN_POINT('Ctrl Pts',(40.8715428282265,2.83156072440399,1.54076368163563));
#76708=CARTESIAN_POINT('Ctrl Pts',(40.8957387757555,2.64712266128551,1.86178189951004));
#76709=CARTESIAN_POINT('Ctrl Pts',(40.9161944280046,2.46533852167192,2.09655829748027));
#76710=CARTESIAN_POINT('Ctrl Pts',(40.9410302121943,2.19677246649203,2.35939607506963));
#76711=CARTESIAN_POINT('Ctrl Pts',(40.9462462240171,2.13732942732533,2.41337615982134));
#76712=CARTESIAN_POINT('Ctrl Pts',(40.9519991343069,2.06756808855726,2.47212442934103));
#76713=CARTESIAN_POINT('Ctrl Pts',(40.9526856144752,2.05917295967253,2.47912156321815));
#76714=CARTESIAN_POINT('Ctrl Pts',(40.9536953277143,2.04671749650712,2.48939596549854));
#76715=CARTESIAN_POINT('Ctrl Pts',(40.9540209049078,2.04268464429904,2.49270620579504));
#76716=CARTESIAN_POINT('Ctrl Pts',(40.9545970136299,2.03551858507123,2.49855917164138));
#76717=CARTESIAN_POINT('Ctrl Pts',(40.9548478291248,2.03238862911907,2.50110581648721));
#76718=CARTESIAN_POINT('Ctrl Pts',(40.9553807672122,2.02571634491355,2.50651383145511));
#76719=CARTESIAN_POINT('Ctrl Pts',(40.9556627716094,2.02217274472622,2.50937356494077));
#76720=CARTESIAN_POINT('Ctrl Pts',(40.9564244830017,2.01256658522939,2.5170923039061));
#76721=CARTESIAN_POINT('Ctrl Pts',(40.9569031625239,2.00649244905026,2.52193695028403));
#76722=CARTESIAN_POINT('Ctrl Pts',(40.9592415913992,1.97663973137351,2.54557093536626));
#76723=CARTESIAN_POINT('Ctrl Pts',(40.9610798153957,1.95261350356946,2.56404693346831));
#76724=CARTESIAN_POINT('Ctrl Pts',(40.966215553248,1.88403615038903,2.61525932339684));
#76725=CARTESIAN_POINT('Ctrl Pts',(40.969466650066,1.83889666155041,2.64719348360908));
#76726=CARTESIAN_POINT('Ctrl Pts',(40.9727542574148,1.7917828152533,2.67873736985021));
#76727=CARTESIAN_POINT('Ctrl Pts',(40.9728360469865,1.79060976431233,2.67952164117767));
#76728=CARTESIAN_POINT('Ctrl Pts',(40.972917806056,1.78943621030417,2.68030513407564));
#76729=CARTESIAN_POINT('Origin',(-1.72497344927317,0.,0.));
#76730=CARTESIAN_POINT('',(42.4668644404635,1.78943621037806,2.68030513402632));
#76731=CARTESIAN_POINT('',(42.2181629331785,1.7894362082953,2.68030513541681));
#76732=CARTESIAN_POINT('',(-1.72497344927317,1.78943621037804,2.68030513402633));
#76733=CARTESIAN_POINT('',(41.6465734493189,-3.22274984877711,-0.000987272568188218));
#76734=CARTESIAN_POINT('Ctrl Pts',(41.6465734493189,-3.22274984877711,-0.000987272568138916));
#76735=CARTESIAN_POINT('Ctrl Pts',(41.6531888554372,-3.22271684721777,-0.108714129160543));
#76736=CARTESIAN_POINT('Ctrl Pts',(41.6598042615555,-3.21727816025484,-0.216286161899388));
#76737=CARTESIAN_POINT('Ctrl Pts',(41.6664196676738,-3.20650535883275,-0.323173244989212));
#76738=CARTESIAN_POINT('Ctrl Pts',(41.6730617404079,-3.19568913238853,-0.4304911885179));
#76739=CARTESIAN_POINT('Ctrl Pts',(41.6797038131421,-3.17949579627129,-0.537118334178048));
#76740=CARTESIAN_POINT('Ctrl Pts',(41.6863458858763,-3.15804844818564,-0.642532148154681));
#76741=CARTESIAN_POINT('Ctrl Pts',(41.6930019474588,-3.13655592990796,-0.748167973831837));
#76742=CARTESIAN_POINT('Ctrl Pts',(41.6996580090414,-3.10978738345449,-0.852585053181288));
#76743=CARTESIAN_POINT('Ctrl Pts',(41.7063140706239,-3.07791567669217,-0.955276216427788));
#76744=CARTESIAN_POINT('Ctrl Pts',(41.7129909883947,-3.04594410271754,-1.05828915347442));
#76745=CARTESIAN_POINT('Ctrl Pts',(41.7196679061655,-3.00883749347042,-1.15956505302346));
#76746=CARTESIAN_POINT('Ctrl Pts',(41.7263448239363,-2.9668173940531,-1.25861515676715));
#76747=CARTESIAN_POINT('Ctrl Pts',(41.729165111922,-2.94906836888673,-1.30045329633503));
#76748=CARTESIAN_POINT('Ctrl Pts',(41.7319853999078,-2.93044325601467,-1.34189462520743));
#76749=CARTESIAN_POINT('Ctrl Pts',(41.7348056878936,-2.91096115150686,-1.38290373378549));
#76750=CARTESIAN_POINT('Ctrl Pts',(41.7409779359863,-2.86832423534858,-1.47265286347875));
#76751=CARTESIAN_POINT('Ctrl Pts',(41.7471501840791,-2.82145774204699,-1.56058627746622));
#76752=CARTESIAN_POINT('Ctrl Pts',(41.7533224321719,-2.77053907784463,-1.64627785644946));
#76753=CARTESIAN_POINT('Ctrl Pts',(41.7594863208245,-2.71968937579647,-1.7318533782663));
#76754=CARTESIAN_POINT('Ctrl Pts',(41.7656502094771,-2.66479863097746,-1.81519272982256));
#76755=CARTESIAN_POINT('Ctrl Pts',(41.7718140981298,-2.60609148357015,-1.89589154272156));
#76756=CARTESIAN_POINT('Ctrl Pts',(41.7779714597883,-2.54744650166023,-1.97650490296165));
#76757=CARTESIAN_POINT('Ctrl Pts',(41.7841288214469,-2.48499340561815,-2.05448293411046));
#76758=CARTESIAN_POINT('Ctrl Pts',(41.7902861831054,-2.41900123876471,-2.12944841904067));
#76759=CARTESIAN_POINT('Ctrl Pts',(41.7964390472517,-2.35305727446859,-2.20435914704658));
#76760=CARTESIAN_POINT('Ctrl Pts',(41.802591911398,-2.28357966500936,-2.27626137864407));
#76761=CARTESIAN_POINT('Ctrl Pts',(41.8087447755444,-2.21087843322919,-2.34481003835748));
#76762=CARTESIAN_POINT('Ctrl Pts',(41.8148953086809,-2.13820474427747,-2.41333272844249));
#76763=CARTESIAN_POINT('Ctrl Pts',(41.8210458418174,-2.06231017534954,-2.47850407345808));
#76764=CARTESIAN_POINT('Ctrl Pts',(41.827196374954,-1.98354176732155,-2.54001567313883));
#76765=CARTESIAN_POINT('Ctrl Pts',(41.8333462231692,-1.90478213091737,-2.60152042290823));
#76766=CARTESIAN_POINT('Ctrl Pts',(41.8394960713844,-1.82314963403302,-2.65936597025777));
#76767=CARTESIAN_POINT('Ctrl Pts',(41.8456459195996,-1.73902377676392,-2.71328470057047));
#76768=CARTESIAN_POINT('Ctrl Pts',(41.8517967279787,-1.6548847850871,-2.76721184911045));
#76769=CARTESIAN_POINT('Ctrl Pts',(41.8579475363579,-1.56825202554976,-2.81721072845098));
#76770=CARTESIAN_POINT('Ctrl Pts',(41.864098344737,-1.47953243507694,-2.86305803923974));
#76771=CARTESIAN_POINT('Ctrl Pts',(41.8702557311032,-1.39071796336552,-2.90895438147252));
#76772=CARTESIAN_POINT('Ctrl Pts',(41.8764131174694,-1.2998125907652,-2.95069008932893));
#76773=CARTESIAN_POINT('Ctrl Pts',(41.8825705038356,-1.20724611690579,-2.98808874963845));
#76774=CARTESIAN_POINT('Ctrl Pts',(41.8887313265725,-1.11462798269791,-3.02550828173604));
#76775=CARTESIAN_POINT('Ctrl Pts',(41.8948921493095,-1.02034731093287,-3.05858580216776));
#76776=CARTESIAN_POINT('Ctrl Pts',(41.9010529720465,-0.924850066360242,
-3.08719450589908));
#76777=CARTESIAN_POINT('Ctrl Pts',(41.9072240949631,-0.829193161491493,
-3.1158510400587));
#76778=CARTESIAN_POINT('Ctrl Pts',(41.9133952178798,-0.732316042675764,
-3.14002372853251));
#76779=CARTESIAN_POINT('Ctrl Pts',(41.9195663407965,-0.634676030107168,
-3.15963667204117));
#76780=CARTESIAN_POINT('Ctrl Pts',(41.9242618627421,-0.560383097043063,
-3.17455988908045));
#76781=CARTESIAN_POINT('Ctrl Pts',(41.9289573846876,-0.485648722800563,
-3.18684430736783));
#76782=CARTESIAN_POINT('Ctrl Pts',(41.9336529066332,-0.410675552293991,
-3.19647667803912));
#76783=CARTESIAN_POINT('Ctrl Pts',(41.9398251547259,-0.312123567225377,
-3.20913839748034));
#76784=CARTESIAN_POINT('Ctrl Pts',(41.9459974028187,-0.212812002725103,
-3.21726038285199));
#76785=CARTESIAN_POINT('Ctrl Pts',(41.9521696509115,-0.113195239517363,
-3.22076146279892));
#76786=CARTESIAN_POINT('Ctrl Pts',(41.9583335395641,-0.0137133931755583,
-3.22425780102649));
#76787=CARTESIAN_POINT('Ctrl Pts',(41.9644974282167,0.0860724000127909,
-3.22314565789634));
#76788=CARTESIAN_POINT('Ctrl Pts',(41.9706613168693,0.185700516500948,-3.21739535660001));
#76789=CARTESIAN_POINT('Ctrl Pts',(41.9768186785279,0.285223135929762,-3.21165114434659));
#76790=CARTESIAN_POINT('Ctrl Pts',(41.9829760401864,0.384587979338632,-3.20127856311584));
#76791=CARTESIAN_POINT('Ctrl Pts',(41.9891334018449,0.48333225383915,-3.18629996938436));
#76792=CARTESIAN_POINT('Ctrl Pts',(41.9952862659912,0.582004402710598,-3.17133231644414));
#76793=CARTESIAN_POINT('Ctrl Pts',(42.0014391301375,0.680056455706556,-3.15176540488068));
#76794=CARTESIAN_POINT('Ctrl Pts',(42.0075919942838,0.777030499735695,-3.12767344282943));
#76795=CARTESIAN_POINT('Ctrl Pts',(42.0137425274204,0.873967805192531,-3.103590608007));
#76796=CARTESIAN_POINT('Ctrl Pts',(42.0198930605569,0.969827492085029,-3.0749862336431));
#76797=CARTESIAN_POINT('Ctrl Pts',(42.0260435936934,1.06416248280563,-3.04198549843502));
#76798=CARTESIAN_POINT('Ctrl Pts',(42.0321934419086,1.15848696841301,-3.00898843817785));
#76799=CARTESIAN_POINT('Ctrl Pts',(42.0383432901238,1.25128668540362,-2.97159613385995));
#76800=CARTESIAN_POINT('Ctrl Pts',(42.044493138339,1.34213131438872,-2.92998312238095));
#76801=CARTESIAN_POINT('Ctrl Pts',(42.0506439467182,1.43299012677032,-2.88836361394282));
#76802=CARTESIAN_POINT('Ctrl Pts',(42.0567947550973,1.5218928499006,-2.84252227037215));
#76803=CARTESIAN_POINT('Ctrl Pts',(42.0629455634764,1.6084316074118,-2.79268067039157));
#76804=CARTESIAN_POINT('Ctrl Pts',(42.0691029498426,1.69506291386803,-2.7427857672711));
#76805=CARTESIAN_POINT('Ctrl Pts',(42.0752603362088,1.77932482911819,-2.68888228207544));
#76806=CARTESIAN_POINT('Ctrl Pts',(42.0814177225749,1.86083655577004,-2.63123637767683));
#76807=CARTESIAN_POINT('Ctrl Pts',(42.0875785453119,1.94239377323541,-2.57355830172212));
#76808=CARTESIAN_POINT('Ctrl Pts',(42.0937393680488,2.02119740286241,-2.51213391418777));
#76809=CARTESIAN_POINT('Ctrl Pts',(42.0999001907858,2.0968996374192,-2.44726979981596));
#76810=CARTESIAN_POINT('Ctrl Pts',(42.1060713137025,2.17272843731557,-2.38229724018212));
#76811=CARTESIAN_POINT('Ctrl Pts',(42.1122424366191,2.24544516842659,-2.31387376442561));
#76812=CARTESIAN_POINT('Ctrl Pts',(42.1184135595358,2.31473870589036,-2.24234303485284));
#76813=CARTESIAN_POINT('Ctrl Pts',(42.1231090814815,2.36746319870094,-2.18791629355583));
#76814=CARTESIAN_POINT('Ctrl Pts',(42.1278046034272,2.41820660224388,-2.13169138250005));
#76815=CARTESIAN_POINT('Ctrl Pts',(42.1325001253728,2.46684819927642,-2.07383160459732));
#76816=CARTESIAN_POINT('Ctrl Pts',(42.1386723734656,2.53078741795934,-1.99777511759932));
#76817=CARTESIAN_POINT('Ctrl Pts',(42.1448446215584,2.59131848425128,-1.91862498491771));
#76818=CARTESIAN_POINT('Ctrl Pts',(42.1510168696512,2.64812742777466,-1.83671954548526));
#76819=CARTESIAN_POINT('Ctrl Pts',(42.1571807583038,2.70485943159059,-1.75492503542689));
#76820=CARTESIAN_POINT('Ctrl Pts',(42.1633446469565,2.75787908697984,-1.67038298951447));
#76821=CARTESIAN_POINT('Ctrl Pts',(42.1695085356091,2.80691182496822,-1.58346568303629));
#76822=CARTESIAN_POINT('Ctrl Pts',(42.1756658972677,2.85589264177358,-1.4966404140327));
#76823=CARTESIAN_POINT('Ctrl Pts',(42.1818232589263,2.90089472222778,-1.40744526112666));
#76824=CARTESIAN_POINT('Ctrl Pts',(42.1879806205848,2.94168663594483,-1.3162816181971));
#76825=CARTESIAN_POINT('Ctrl Pts',(42.1941334847312,2.98244875408687,-1.22518456378751));
#76826=CARTESIAN_POINT('Ctrl Pts',(42.2002863488775,3.01900664268743,-1.13212227332568));
#76827=CARTESIAN_POINT('Ctrl Pts',(42.2064392130238,3.05117512799439,-1.03752007248458));
#76828=CARTESIAN_POINT('Ctrl Pts',(42.2125897461604,3.08333142628539,-0.942953711644042));
#76829=CARTESIAN_POINT('Ctrl Pts',(42.2187402792969,3.11110148581676,-0.846849010418827));
#76830=CARTESIAN_POINT('Ctrl Pts',(42.2248908124335,3.13434886858439,-0.749649739881074));
#76831=CARTESIAN_POINT('Ctrl Pts',(42.2310406606487,3.15759366253118,-0.652461293421855));
#76832=CARTESIAN_POINT('Ctrl Pts',(42.2371905088639,3.17631667999076,-0.554178942447612));
#76833=CARTESIAN_POINT('Ctrl Pts',(42.2433403570792,3.1904320648593,-0.455259049352848));
#76834=CARTESIAN_POINT('Ctrl Pts',(42.2494911654583,3.20454965353562,-0.356323712086136));
#76835=CARTESIAN_POINT('Ctrl Pts',(42.2556419738375,3.21405811937742,-0.256751065050087));
#76836=CARTESIAN_POINT('Ctrl Pts',(42.2617927822167,3.21892331345298,-0.157004027365236));
#76837=CARTESIAN_POINT('Ctrl Pts',(42.2679501685829,3.22379371061431,-0.0571503151293831));
#76838=CARTESIAN_POINT('Ctrl Pts',(42.2741075549491,3.22401089871511,0.0428777254755896));
#76839=CARTESIAN_POINT('Ctrl Pts',(42.2802649413153,3.21959287528708,0.142615847298526));
#76840=CARTESIAN_POINT('Ctrl Pts',(42.2864257640523,3.21517238620793,0.242409631889109));
#76841=CARTESIAN_POINT('Ctrl Pts',(42.2925865867892,3.20611157329408,0.341912742874543));
#76842=CARTESIAN_POINT('Ctrl Pts',(42.2987474095262,3.19248027543204,0.440666828201722));
#76843=CARTESIAN_POINT('Ctrl Pts',(42.3049185324429,3.17882618762393,0.539586018884353));
#76844=CARTESIAN_POINT('Ctrl Pts',(42.3110896553596,3.16058643095412,0.637753255245494));
#76845=CARTESIAN_POINT('Ctrl Pts',(42.3172607782763,3.13788186881971,0.734720994549995));
#76846=CARTESIAN_POINT('Ctrl Pts',(42.3219563002217,3.12060628199354,0.808502404196861));
#76847=CARTESIAN_POINT('Ctrl Pts',(42.3266518221671,3.10074686348569,0.881589592692564));
#76848=CARTESIAN_POINT('Ctrl Pts',(42.3313473441125,3.07837571211205,0.953792712059928));
#76849=CARTESIAN_POINT('Ctrl Pts',(42.3375183118758,3.04897500744927,1.04868378640816));
#76850=CARTESIAN_POINT('Ctrl Pts',(42.343689279639,3.01513092331397,1.14238115422715));
#76851=CARTESIAN_POINT('Ctrl Pts',(42.3498602474023,2.9769582296873,1.23443803457164));
#76852=CARTESIAN_POINT('Ctrl Pts',(42.3560234343757,2.93883366687578,1.32637884313102));
#76853=CARTESIAN_POINT('Ctrl Pts',(42.3621866213491,2.89639150265972,1.41668287634627));
#76854=CARTESIAN_POINT('Ctrl Pts',(42.3683498083224,2.84979636673714,1.5049180145881));
#76855=CARTESIAN_POINT('Ctrl Pts',(42.3745068736213,2.80324751210626,1.59306551200454));
#76856=CARTESIAN_POINT('Ctrl Pts',(42.3806639389202,2.75255408509429,1.67914781649568));
#76857=CARTESIAN_POINT('Ctrl Pts',(42.3868210042191,2.69792855804005,1.76275326072934));
#76858=CARTESIAN_POINT('Ctrl Pts',(42.3929736012668,2.64334267334214,1.84629803155646));
#76859=CARTESIAN_POINT('Ctrl Pts',(42.3991261983146,2.58483059857675,1.92736915323287));
#76860=CARTESIAN_POINT('Ctrl Pts',(42.4052787953623,2.52264994534249,2.00558091728146));
#76861=CARTESIAN_POINT('Ctrl Pts',(42.4114292904071,2.4604905358059,2.08376596068651));
#76862=CARTESIAN_POINT('Ctrl Pts',(42.4175797854519,2.39466530625443,2.15909324642196));
#76863=CARTESIAN_POINT('Ctrl Pts',(42.4237302804968,2.32547376511001,2.23120804280665));
#76864=CARTESIAN_POINT('Ctrl Pts',(42.4298795872027,2.25629559248333,2.3033089058706));
#76865=CARTESIAN_POINT('Ctrl Pts',(42.4360288939086,2.18375270569772,2.37219820377838));
#76866=CARTESIAN_POINT('Ctrl Pts',(42.4421782006145,2.10818247187806,2.43755702041329));
#76867=CARTESIAN_POINT('Ctrl Pts',(42.4483294334061,2.03258856795084,2.50293630873582));
#76868=CARTESIAN_POINT('Ctrl Pts',(42.4544806661978,1.95396575454669,2.56478262620546));
#76869=CARTESIAN_POINT('Ctrl Pts',(42.4606318989895,1.87268504088621,2.62281686362983));
#76870=CARTESIAN_POINT('Ctrl Pts',(42.4627094128142,1.84523333940979,2.64241731359439));
#76871=CARTESIAN_POINT('Ctrl Pts',(42.4647869266388,1.81747871455803,2.66158328337868));
#76872=CARTESIAN_POINT('Ctrl Pts',(42.4668644404635,1.78943621037806,2.68030513402631));
#76873=CARTESIAN_POINT('Ctrl Pts',(41.2170239499866,1.789436210378,2.68030513402635));
#76874=CARTESIAN_POINT('Ctrl Pts',(41.2231741454125,1.70635148068182,2.73577449904767));
#76875=CARTESIAN_POINT('Ctrl Pts',(41.2293243408382,1.62065528784251,2.78739697266643));
#76876=CARTESIAN_POINT('Ctrl Pts',(41.235474536264,1.53274247640791,2.83492822898834));
#76877=CARTESIAN_POINT('Ctrl Pts',(41.2416244765792,1.44483331160414,2.88245751370973));
#76878=CARTESIAN_POINT('Ctrl Pts',(41.2477744168944,1.35470809335699,2.92589571228594));
#76879=CARTESIAN_POINT('Ctrl Pts',(41.2539243572096,1.26278658245949,2.96504428460357));
#76880=CARTESIAN_POINT('Ctrl Pts',(41.260075687455,1.17084429664666,3.00420170477702));
#76881=CARTESIAN_POINT('Ctrl Pts',(41.2662270177005,1.07710531129399,3.03906740251434));
#76882=CARTESIAN_POINT('Ctrl Pts',(41.2723783479459,0.982008744145685,3.0694912263959));
#76883=CARTESIAN_POINT('Ctrl Pts',(41.2785364887349,0.886806889313731,3.09994873450015));
#76884=CARTESIAN_POINT('Ctrl Pts',(41.2846946295239,0.79024486659597,3.12595441911275));
#76885=CARTESIAN_POINT('Ctrl Pts',(41.2908527703129,0.692776155103506,3.14740826100142));
#76886=CARTESIAN_POINT('Ctrl Pts',(41.2970147337812,0.595246939696369,3.16887542040912));
#76887=CARTESIAN_POINT('Ctrl Pts',(41.3031766972494,0.496810342641535,3.18578503802205));
#76888=CARTESIAN_POINT('Ctrl Pts',(41.3093386607177,0.397927170727749,3.19808873067909));
#76889=CARTESIAN_POINT('Ctrl Pts',(41.3155104475573,0.298886359756286,3.21041203782138));
#76890=CARTESIAN_POINT('Ctrl Pts',(41.3216822343969,0.199397985047641,3.21811472722107));
#76891=CARTESIAN_POINT('Ctrl Pts',(41.3278540212365,0.0999250258606228,
3.22120048300424));
#76892=CARTESIAN_POINT('Ctrl Pts',(41.3309397642958,0.0501909696836931,
3.2227432857189));
#76893=CARTESIAN_POINT('Ctrl Pts',(41.334025507355,0.000460725377187637,
3.2231327841228));
#76894=CARTESIAN_POINT('Ctrl Pts',(41.3371112504142,-0.0492083651102425,
3.22237429534546));
#76895=CARTESIAN_POINT('Ctrl Pts',(41.343283498507,-0.148558811063045,3.22085713049426));
#76896=CARTESIAN_POINT('Ctrl Pts',(41.3494557465998,-0.248013894267614,
3.21473831405031));
#76897=CARTESIAN_POINT('Ctrl Pts',(41.3556279946925,-0.347112303184287,
3.2040022801924));
#76898=CARTESIAN_POINT('Ctrl Pts',(41.3617918833451,-0.446076497272524,
3.19328078677927));
#76899=CARTESIAN_POINT('Ctrl Pts',(41.3679557719978,-0.544684549171801,
3.17795455158715));
#76900=CARTESIAN_POINT('Ctrl Pts',(41.3741196606504,-0.64247531955352,3.15806000992138));
#76901=CARTESIAN_POINT('Ctrl Pts',(41.3802770223089,-0.740162538457424,
3.13818653475485));
#76902=CARTESIAN_POINT('Ctrl Pts',(41.3864343839674,-0.837033773084093,
3.11375445647749));
#76903=CARTESIAN_POINT('Ctrl Pts',(41.392591745626,-0.93263414456588,3.08485187892221));
#76904=CARTESIAN_POINT('Ctrl Pts',(41.3987446097723,-1.02816468681501,3.05597041263231));
#76905=CARTESIAN_POINT('Ctrl Pts',(41.4048974739186,-1.12242579695264,3.02262506452357));
#76906=CARTESIAN_POINT('Ctrl Pts',(41.4110503380649,-1.21497481803341,2.98495456482083));
#76907=CARTESIAN_POINT('Ctrl Pts',(41.4172008712015,-1.30748877695991,2.94729833656965));
#76908=CARTESIAN_POINT('Ctrl Pts',(41.423351404338,-1.39829153376462,2.90532037615488));
#76909=CARTESIAN_POINT('Ctrl Pts',(41.4295019374746,-1.48695842267173,2.85920831905365));
#76910=CARTESIAN_POINT('Ctrl Pts',(41.4356517856898,-1.5756154376633,2.81310139697591));
#76911=CARTESIAN_POINT('Ctrl Pts',(41.441801633905,-1.66213667226087,2.76286149391629));
#76912=CARTESIAN_POINT('Ctrl Pts',(41.4479514821202,-1.74612108424166,2.70872271036862));
#76913=CARTESIAN_POINT('Ctrl Pts',(41.4541022904993,-1.83011860854692,2.65457547423696));
#76914=CARTESIAN_POINT('Ctrl Pts',(41.4602530988785,-1.91157815841264,2.59652838390418));
#76915=CARTESIAN_POINT('Ctrl Pts',(41.4664039072576,-1.99012761168494,2.5348589017358));
#76916=CARTESIAN_POINT('Ctrl Pts',(41.4725612936238,-2.06876106973406,2.47312346708945));
#76917=CARTESIAN_POINT('Ctrl Pts',(41.47871867999,-2.14447787411286,2.40775817345017));
#76918=CARTESIAN_POINT('Ctrl Pts',(41.4848760663562,-2.21693906097446,2.33908075158292));
#76919=CARTESIAN_POINT('Ctrl Pts',(41.4910368890932,-2.28944068764113,2.27036500158892));
#76920=CARTESIAN_POINT('Ctrl Pts',(41.4971977118301,-2.35868277737298,2.19833375534159));
#76921=CARTESIAN_POINT('Ctrl Pts',(41.5033585345671,-2.42436478206505,2.1233400495405));
#76922=CARTESIAN_POINT('Ctrl Pts',(41.5095296574838,-2.49015659943671,2.04822096297761));
#76923=CARTESIAN_POINT('Ctrl Pts',(41.5157007804005,-2.55237617192966,1.97012986350473));
#76924=CARTESIAN_POINT('Ctrl Pts',(41.5218719033172,-2.61076454491503,1.88945125724762));
#76925=CARTESIAN_POINT('Ctrl Pts',(41.5265674252627,-2.65519144913029,1.82806402329775));
#76926=CARTESIAN_POINT('Ctrl Pts',(41.5312629472083,-2.69740115169467,1.7651794096343));
#76927=CARTESIAN_POINT('Ctrl Pts',(41.5359584691539,-2.7372974487943,1.70097626065863));
#76928=CARTESIAN_POINT('Ctrl Pts',(41.5423065722644,-2.79123518152077,1.61417691983259));
#76929=CARTESIAN_POINT('Ctrl Pts',(41.5486546753748,-2.84112404934189,1.5246755827609));
#76930=CARTESIAN_POINT('Ctrl Pts',(41.5550027784852,-2.88669177993702,1.4328740803518));
#76931=CARTESIAN_POINT('Ctrl Pts',(41.561340685878,-2.93218632398999,1.3412200207589));
#76932=CARTESIAN_POINT('Ctrl Pts',(41.5676785932707,-2.97337336231237,1.24727350226578));
#76933=CARTESIAN_POINT('Ctrl Pts',(41.5740165006635,-3.01002462655561,1.15146398555436));
#76934=CARTESIAN_POINT('Ctrl Pts',(41.5803429132751,-3.04660941802866,1.05582823430831));
#76935=CARTESIAN_POINT('Ctrl Pts',(41.5866693258867,-3.07867467933153,0.958336587463989));
#76936=CARTESIAN_POINT('Ctrl Pts',(41.5929957384983,-3.10603918615133,0.859440595150354));
#76937=CARTESIAN_POINT('Ctrl Pts',(41.5993154040876,-3.13337450914324,0.760650073899592));
#76938=CARTESIAN_POINT('Ctrl Pts',(41.6056350696769,-3.15601894407938,0.660458570956468));
#76939=CARTESIAN_POINT('Ctrl Pts',(41.6119547352663,-3.17384021541428,0.559335185303994));
#76940=CARTESIAN_POINT('Ctrl Pts',(41.6182677003448,-3.19164259150543,0.458319017087579));
#76941=CARTESIAN_POINT('Ctrl Pts',(41.6245806654233,-3.20463191844682,0.356373327360609));
#76942=CARTESIAN_POINT('Ctrl Pts',(41.6308936305018,-3.21272660233886,0.253979017094328));
#76943=CARTESIAN_POINT('Ctrl Pts',(41.6361202367589,-3.21942832252161,0.169205105615897));
#76944=CARTESIAN_POINT('Ctrl Pts',(41.641346843016,-3.22277592216168,0.0841240354286471));
#76945=CARTESIAN_POINT('Ctrl Pts',(41.6465734492731,-3.22274984877734,-0.000987271822784419));
#76946=CARTESIAN_POINT('',(41.3996307778974,-3.22274865316434,0.00294635832935292));
#76947=CARTESIAN_POINT('Ctrl Pts',(40.972917806056,1.78943621030417,2.68030513407564));
#76948=CARTESIAN_POINT('Ctrl Pts',(40.980957584323,1.67403477442647,2.75734990985707));
#76949=CARTESIAN_POINT('Ctrl Pts',(40.9887073764522,1.55376902517541,2.82686727887822));
#76950=CARTESIAN_POINT('Ctrl Pts',(41.0100377824585,1.2116588987041,2.99616686366643));
#76951=CARTESIAN_POINT('Ctrl Pts',(41.0236188803539,0.982475836522961,3.0789374930667));
#76952=CARTESIAN_POINT('Ctrl Pts',(41.0386060427792,0.73872344541865,3.13695139008336));
#76953=CARTESIAN_POINT('Ctrl Pts',(41.0390654799045,0.731258067519423,3.13870004774921));
#76954=CARTESIAN_POINT('Ctrl Pts',(41.0412107982511,0.696432798931211,3.14672637711884));
#76955=CARTESIAN_POINT('Ctrl Pts',(41.0429068299818,0.668998518026038,3.1526729044838));
#76956=CARTESIAN_POINT('Ctrl Pts',(41.0452933938915,0.630551126726525,3.1604821547801));
#76957=CARTESIAN_POINT('Ctrl Pts',(41.0459742475717,0.619600188803281,3.16264727328437));
#76958=CARTESIAN_POINT('Ctrl Pts',(41.0470733980874,0.60195082073379,3.16604155829027));
#76959=CARTESIAN_POINT('Ctrl Pts',(41.0474905502978,0.59525929253796,3.16730647600172));
#76960=CARTESIAN_POINT('Ctrl Pts',(41.0483568385336,0.581377611438307,3.16988502302879));
#76961=CARTESIAN_POINT('Ctrl Pts',(41.0488060750347,0.57418690443771,3.17119541871411));
#76962=CARTESIAN_POINT('Ctrl Pts',(41.0498489833794,0.557512546622209,3.17417549139952));
#76963=CARTESIAN_POINT('Ctrl Pts',(41.0504432258945,0.548025782576076,3.17582714080104));
#76964=CARTESIAN_POINT('Ctrl Pts',(41.0523301981932,0.517947367657273,3.18092501939036));
#76965=CARTESIAN_POINT('Ctrl Pts',(41.053627922684,0.49732988106972,3.18421362521021));
#76966=CARTESIAN_POINT('Ctrl Pts',(41.0613795447484,0.374600617119166,3.20256860773854));
#76967=CARTESIAN_POINT('Ctrl Pts',(41.0679814821593,0.271854947992482,3.21292115242249));
#76968=CARTESIAN_POINT('Ctrl Pts',(41.0880760314614,-0.0355140691247797,
3.22904238198276));
#76969=CARTESIAN_POINT('Ctrl Pts',(41.1019533968349,-0.240364069228848,
3.2202769762283));
#76970=CARTESIAN_POINT('Ctrl Pts',(41.1237531475644,-0.559764665086802,
3.17595401467161));
#76971=CARTESIAN_POINT('Ctrl Pts',(41.1316822142413,-0.675586645266371,
3.15334851807387));
#76972=CARTESIAN_POINT('Ctrl Pts',(41.1431342486706,-0.845478873139643,
3.11039669788195));
#76973=CARTESIAN_POINT('Ctrl Pts',(41.1468245362911,-0.900661595518483,
3.09486862599111));
#76974=CARTESIAN_POINT('Ctrl Pts',(41.1510580198752,-0.964832172832273,
3.07494941137412));
#76975=CARTESIAN_POINT('Ctrl Pts',(41.1516776150025,-0.974246333396892,
3.07197966987172));
#76976=CARTESIAN_POINT('Ctrl Pts',(41.152611798047,-0.988476838320987,3.06741859354113));
#76977=CARTESIAN_POINT('Ctrl Pts',(41.1529282132672,-0.993303210872229,
3.06585909983028));
#76978=CARTESIAN_POINT('Ctrl Pts',(41.153494254275,-1.00194906352601,3.06304289943937));
#76979=CARTESIAN_POINT('Ctrl Pts',(41.1537441271462,-1.00576987568242,3.06179043820328));
#76980=CARTESIAN_POINT('Ctrl Pts',(41.1542819116748,-1.01400226186873,3.05907479110576));
#76981=CARTESIAN_POINT('Ctrl Pts',(41.1545696790777,-1.01841300119325,3.05760921706868));
#76982=CARTESIAN_POINT('Ctrl Pts',(41.1553632744113,-1.03059170051063,3.05353327537096));
#76983=CARTESIAN_POINT('Ctrl Pts',(41.1558679231591,-1.03835296452589,3.05090279121717));
#76984=CARTESIAN_POINT('Ctrl Pts',(41.1585620612214,-1.07987136539258,3.0366543936234));
#76985=CARTESIAN_POINT('Ctrl Pts',(41.1607213526855,-1.11344530574384,3.02450522801414));
#76986=CARTESIAN_POINT('Ctrl Pts',(41.1670299422431,-1.21212827182131,2.98692942218416));
#76987=CARTESIAN_POINT('Ctrl Pts',(41.1711033394766,-1.27662275848237,2.95993884921536));
#76988=CARTESIAN_POINT('Ctrl Pts',(41.1861593399872,-1.515140261821,2.85087248226606));
#76989=CARTESIAN_POINT('Ctrl Pts',(41.1967320934736,-1.68258141155163,2.75536772896923));
#76990=CARTESIAN_POINT('Ctrl Pts',(41.2182495554033,-1.99648878942316,2.53697753162626));
#76991=CARTESIAN_POINT('Ctrl Pts',(41.2291511645902,-2.14254158688703,2.41489603816608));
#76992=CARTESIAN_POINT('Ctrl Pts',(41.2417044789304,-2.28966783132644,2.26800796843223));
#76993=CARTESIAN_POINT('Ctrl Pts',(41.2427914679644,-2.3022479575006,2.25523684893812));
#76994=CARTESIAN_POINT('Ctrl Pts',(41.2444412126697,-2.3210970356885,2.23577952745254));
#76995=CARTESIAN_POINT('Ctrl Pts',(41.2450005084585,-2.32744522737459,2.22917030648221));
#76996=CARTESIAN_POINT('Ctrl Pts',(41.2459747616216,-2.33842991676013,2.2176358674692));
#76997=CARTESIAN_POINT('Ctrl Pts',(41.2463891588106,-2.34307928020381,2.21272293834061));
#76998=CARTESIAN_POINT('Ctrl Pts',(41.2472547157605,-2.35274243080177,2.20244739152366));
#76999=CARTESIAN_POINT('Ctrl Pts',(41.2477059919976,-2.3577534249839,2.19708221140661));
#77000=CARTESIAN_POINT('Ctrl Pts',(41.2486039153174,-2.3676700267056,2.18639169206184));
#77001=CARTESIAN_POINT('Ctrl Pts',(41.2490505382254,-2.37257610742014,2.18106684895383));
#77002=CARTESIAN_POINT('Ctrl Pts',(41.2500947522579,-2.3839848641791,2.16860024424316));
#77003=CARTESIAN_POINT('Ctrl Pts',(41.2506929374452,-2.39047343498167,2.16144572111962));
#77004=CARTESIAN_POINT('Ctrl Pts',(41.2541623315757,-2.42783340103523,2.1198773308669));
#77005=CARTESIAN_POINT('Ctrl Pts',(41.2570632236582,-2.45799225818394,2.08483299601679));
#77006=CARTESIAN_POINT('Ctrl Pts',(41.267586577498,-2.56350355193783,1.95675704569465));
#77007=CARTESIAN_POINT('Ctrl Pts',(41.275380692213,-2.63440570316206,1.86020148537382));
#77008=CARTESIAN_POINT('Ctrl Pts',(41.2894731125337,-2.75035948935685,1.68232664511113));
#77009=CARTESIAN_POINT('Ctrl Pts',(41.2957036281926,-2.797579231196,1.60257581120209));
#77010=CARTESIAN_POINT('Ctrl Pts',(41.3093819122003,-2.89308880458486,1.42414855275538));
#77011=CARTESIAN_POINT('Ctrl Pts',(41.3168340968007,-2.93990567010013,1.32480834142187));
#77012=CARTESIAN_POINT('Ctrl Pts',(41.3290186368766,-3.00884358159769,1.15678136266766));
#77013=CARTESIAN_POINT('Ctrl Pts',(41.3337979309899,-3.03389326108652,1.08939234692077));
#77014=CARTESIAN_POINT('Ctrl Pts',(41.3421564354891,-3.07444941986071,0.968001298429983));
#77015=CARTESIAN_POINT('Ctrl Pts',(41.3457674415938,-3.09083755589449,0.914324818958046));
#77016=CARTESIAN_POINT('Ctrl Pts',(41.349866403996,-3.108204256811,0.851624248774252));
#77017=CARTESIAN_POINT('Ctrl Pts',(41.3504279715182,-3.1105558867676,0.842994450106333));
#77018=CARTESIAN_POINT('Ctrl Pts',(41.3513195131313,-3.11424563056493,0.829228486384964));
#77019=CARTESIAN_POINT('Ctrl Pts',(41.3516508018782,-3.11560701659807,0.824098689000286));
#77020=CARTESIAN_POINT('Ctrl Pts',(41.3522341480687,-3.11798718013355,0.815039865022391));
#77021=CARTESIAN_POINT('Ctrl Pts',(41.3524865098037,-3.11901121464037,0.811112249157957));
#77022=CARTESIAN_POINT('Ctrl Pts',(41.3530150874122,-3.12114424586065,0.80286737818465));
#77023=CARTESIAN_POINT('Ctrl Pts',(41.3532912132257,-3.12225170423916,0.798549764493275));
#77024=CARTESIAN_POINT('Ctrl Pts',(41.3540205858157,-3.12515876960255,0.787117578492366));
#77025=CARTESIAN_POINT('Ctrl Pts',(41.3544729498594,-3.12694305218309,0.779999082360786));
#77026=CARTESIAN_POINT('Ctrl Pts',(41.3554609261163,-3.13079837503754,0.764392200885226));
#77027=CARTESIAN_POINT('Ctrl Pts',(41.3559959710274,-3.13285925014294,0.755901332660203));
#77028=CARTESIAN_POINT('Ctrl Pts',(41.3575855143787,-3.13889993420492,0.730564430291809));
#77029=CARTESIAN_POINT('Ctrl Pts',(41.3586346240465,-3.14277865087828,0.713694307322203));
#77030=CARTESIAN_POINT('Ctrl Pts',(41.3737299025313,-3.19697086577163,0.468977618165554));
#77031=CARTESIAN_POINT('Ctrl Pts',(41.3865738748205,-3.22253528388174,0.236331266495792));
#77032=CARTESIAN_POINT('Ctrl Pts',(41.3996307778974,-3.22274865316434,0.00294635832935292));
#77033=CARTESIAN_POINT('Ctrl Pts',(41.3996308389411,-3.22274865416171,0.00294526720681157));
#77034=CARTESIAN_POINT('Ctrl Pts',(41.4101609837527,-3.22292066871231,-0.185275231143605));
#77035=CARTESIAN_POINT('Ctrl Pts',(41.4207837320835,-3.2066040436147,-0.37313437457173));
#77036=CARTESIAN_POINT('Ctrl Pts',(41.4346359164017,-3.16606665841715,-0.603514064877092));
#77037=CARTESIAN_POINT('Ctrl Pts',(41.4373704933508,-3.15718789313295,-0.64836070533953));
#77038=CARTESIAN_POINT('Ctrl Pts',(41.4408847759572,-3.14469440171184,-0.705101543230631));
#77039=CARTESIAN_POINT('Ctrl Pts',(41.4416363749525,-3.14196047385066,-0.717185778268995));
#77040=CARTESIAN_POINT('Ctrl Pts',(41.4428973454155,-3.13727085922018,-0.737372763963564));
#77041=CARTESIAN_POINT('Ctrl Pts',(41.4434054936418,-3.13535328037617,-0.745484300528934));
#77042=CARTESIAN_POINT('Ctrl Pts',(41.444407091479,-3.13151926918105,-0.761426039385879));
#77043=CARTESIAN_POINT('Ctrl Pts',(41.4449004720729,-3.12960488149455,-0.769256674046396));
#77044=CARTESIAN_POINT('Ctrl Pts',(41.4458370319191,-3.12592227937388,-0.784078740958211));
#77045=CARTESIAN_POINT('Ctrl Pts',(41.4462800187235,-3.12415993567352,-0.791071592016112));
#77046=CARTESIAN_POINT('Ctrl Pts',(41.4472855542911,-3.1201133342246,-0.806903770923343));
#77047=CARTESIAN_POINT('Ctrl Pts',(41.4478485576607,-3.11781496360198,-0.815739397068185));
#77048=CARTESIAN_POINT('Ctrl Pts',(41.4495140121126,-3.11092007882728,-0.841790548517696));
#77049=CARTESIAN_POINT('Ctrl Pts',(41.4506198717715,-3.10621835348575,-0.858977639021715));
#77050=CARTESIAN_POINT('Ctrl Pts',(41.4585175222862,-3.07176975141496,-0.980921498774192));
#77051=CARTESIAN_POINT('Ctrl Pts',(41.4654770630248,-3.03687573875394,-1.0841391014907));
#77052=CARTESIAN_POINT('Ctrl Pts',(41.4734735641859,-2.99183893609184,-1.19799890577171));
#77053=CARTESIAN_POINT('Ctrl Pts',(41.4743617336352,-2.9867695885259,-1.21058209763802));
#77054=CARTESIAN_POINT('Ctrl Pts',(41.4817031482774,-2.94431356955439,-1.31407679577869));
#77055=CARTESIAN_POINT('Ctrl Pts',(41.4882639431685,-2.90286718693912,-1.40326049987602));
#77056=CARTESIAN_POINT('Ctrl Pts',(41.5020922428597,-2.80789815596172,-1.58533558153205));
#77057=CARTESIAN_POINT('Ctrl Pts',(41.5093625777834,-2.75368371772362,-1.67773850786885));
#77058=CARTESIAN_POINT('Ctrl Pts',(41.5259672062774,-2.61876733667292,-1.88347722767872));
#77059=CARTESIAN_POINT('Ctrl Pts',(41.5352563835041,-2.53511753338876,-1.99464686724353));
#77060=CARTESIAN_POINT('Ctrl Pts',(41.5457700151251,-2.42800741622158,-2.11932570617653));
#77061=CARTESIAN_POINT('Ctrl Pts',(41.5473792802327,-2.41124452241144,-2.13837821976389));
#77062=CARTESIAN_POINT('Ctrl Pts',(41.5494395006869,-2.38928045650573,-2.16275559232747));
#77063=CARTESIAN_POINT('Ctrl Pts',(41.5499049948148,-2.38428402200986,-2.16826256642882));
#77064=CARTESIAN_POINT('Ctrl Pts',(41.5506485994047,-2.3762473801383,-2.17705902833002));
#77065=CARTESIAN_POINT('Ctrl Pts',(41.5509276172846,-2.3732193337418,-2.18035951599411));
#77066=CARTESIAN_POINT('Ctrl Pts',(41.5514580732704,-2.36743847351322,-2.18663418522138));
#77067=CARTESIAN_POINT('Ctrl Pts',(41.5517096001292,-2.36468696367123,-2.18960945144182));
#77068=CARTESIAN_POINT('Ctrl Pts',(41.5522868689135,-2.35834832189242,-2.19643767659625));
#77069=CARTESIAN_POINT('Ctrl Pts',(41.5526123128179,-2.35475735989784,-2.20028703843058));
#77070=CARTESIAN_POINT('Ctrl Pts',(41.5536444961484,-2.34331332438144,-2.21249446392588));
#77071=CARTESIAN_POINT('Ctrl Pts',(41.5543485728151,-2.33542495362664,-2.22081952988898));
#77072=CARTESIAN_POINT('Ctrl Pts',(41.5675857807291,-2.18560464052134,-2.37725271909167));
#77073=CARTESIAN_POINT('Ctrl Pts',(41.579087259001,-2.02987112057745,-2.51154315726582));
#77074=CARTESIAN_POINT('Ctrl Pts',(41.5997845458028,-1.72777895193172,-2.72545559509027));
#77075=CARTESIAN_POINT('Ctrl Pts',(41.6089601979415,-1.58603893305355,-2.81030340594898));
#77076=CARTESIAN_POINT('Ctrl Pts',(41.6229182000108,-1.36892008311917,-2.91859723241247));
#77077=CARTESIAN_POINT('Ctrl Pts',(41.6274491850044,-1.29817890194282,-2.95074265819879));
#77078=CARTESIAN_POINT('Ctrl Pts',(41.6348135389141,-1.18355012062124,-2.99791070208356));
#77079=CARTESIAN_POINT('Ctrl Pts',(41.6375918017885,-1.14037854569827,-3.01459713826682));
#77080=CARTESIAN_POINT('Ctrl Pts',(41.6411924577925,-1.08461166028488,-3.03478251333899));
#77081=CARTESIAN_POINT('Ctrl Pts',(41.6419859981151,-1.07233244007331,-3.03914305143121));
#77082=CARTESIAN_POINT('Ctrl Pts',(41.6432728509826,-1.05243967530325,-3.04607170759743));
#77083=CARTESIAN_POINT('Ctrl Pts',(41.6437646240839,-1.04484229702476,-3.04868605967826));
#77084=CARTESIAN_POINT('Ctrl Pts',(41.6446998965571,-1.03040269125539,-3.05359459247757));
#77085=CARTESIAN_POINT('Ctrl Pts',(41.6451432108069,-1.02356236926262,-3.0558942580258));
#77086=CARTESIAN_POINT('Ctrl Pts',(41.646151913646,-1.00800754856697,-3.06106558788978));
#77087=CARTESIAN_POINT('Ctrl Pts',(41.6467177679957,-0.999288422945987,
-3.06392304020655));
#77088=CARTESIAN_POINT('Ctrl Pts',(41.6484372861928,-0.972814041576651,
-3.07247425876791));
#77089=CARTESIAN_POINT('Ctrl Pts',(41.6495947856717,-0.955021703470315,
-3.07805112897944));
#77090=CARTESIAN_POINT('Ctrl Pts',(41.6585337071672,-0.817858721331375,
-3.11974006437207));
#77091=CARTESIAN_POINT('Ctrl Pts',(41.6665367618616,-0.696545584555774,
-3.14904564045875));
#77092=CARTESIAN_POINT('Ctrl Pts',(41.6862708095288,-0.400982854423891,
-3.20252909398001));
#77093=CARTESIAN_POINT('Ctrl Pts',(41.6981667776634,-0.225858522660113,
-3.21962073225346));
#77094=CARTESIAN_POINT('Ctrl Pts',(41.7223526362528,0.131577845530588,-3.2251926589007));
#77095=CARTESIAN_POINT('Ctrl Pts',(41.734595686057,0.313324992523949,-3.21263508685753));
#77096=CARTESIAN_POINT('Ctrl Pts',(41.7469095899262,0.505780280299551,-3.18283985422686));
#77097=CARTESIAN_POINT('Ctrl Pts',(41.7477195238514,0.518488264655123,-3.18079442311357));
#77098=CARTESIAN_POINT('Ctrl Pts',(41.7488814112151,0.536795331804624,-3.17773515285817));
#77099=CARTESIAN_POINT('Ctrl Pts',(41.7492367301017,0.542404319754735,-3.17678256811051));
#77100=CARTESIAN_POINT('Ctrl Pts',(41.7498470515294,0.552057340823478,-3.17511686665986));
#77101=CARTESIAN_POINT('Ctrl Pts',(41.7501024579607,0.556102574271717,-3.17441086693698));
#77102=CARTESIAN_POINT('Ctrl Pts',(41.7505943059448,0.563903791934002,-3.17303397917033));
#77103=CARTESIAN_POINT('Ctrl Pts',(41.7508308085039,0.567659928901751,-3.1723641539092));
#77104=CARTESIAN_POINT('Ctrl Pts',(41.7513949599317,0.576631360882703,-3.1707478504196));
#77105=CARTESIAN_POINT('Ctrl Pts',(41.7517222554968,0.581845548407632,-3.16979516941375));
#77106=CARTESIAN_POINT('Ctrl Pts',(41.7527125496249,0.59764946688726,-3.16686733532586));
#77107=CARTESIAN_POINT('Ctrl Pts',(41.7533733071196,0.608231796460825,-3.16485192295055));
#77108=CARTESIAN_POINT('Ctrl Pts',(41.7622654608353,0.751112757138264,-3.13689701852716));
#77109=CARTESIAN_POINT('Ctrl Pts',(41.7700539637878,0.881685121248366,-3.10273012347454));
#77110=CARTESIAN_POINT('Ctrl Pts',(41.7918661125119,1.24735908910469,-2.98208278985948));
#77111=CARTESIAN_POINT('Ctrl Pts',(41.8055122053887,1.47502514175452,-2.87628677778942));
#77112=CARTESIAN_POINT('Ctrl Pts',(41.8239015214452,1.74573136360546,-2.70981674816123));
#77113=CARTESIAN_POINT('Ctrl Pts',(41.8278625908618,1.80216791083966,-2.67261570894969));
#77114=CARTESIAN_POINT('Ctrl Pts',(41.8335380702332,1.88003922898702,-2.61769710646741));
#77115=CARTESIAN_POINT('Ctrl Pts',(41.8351991518457,1.90248014290615,-2.60143323546238));
#77116=CARTESIAN_POINT('Ctrl Pts',(41.8381271469185,1.94140359901069,-2.57245076048246));
#77117=CARTESIAN_POINT('Ctrl Pts',(41.8393891926808,1.95797804895761,-2.55985796046748));
#77118=CARTESIAN_POINT('Ctrl Pts',(41.8412404050538,1.98198887004077,-2.54124559484091));
#77119=CARTESIAN_POINT('Ctrl Pts',(41.8418245826476,1.98952249646303,-2.53535190599361));
#77120=CARTESIAN_POINT('Ctrl Pts',(41.8428568653536,2.0027580013335,-2.52490221945136));
#77121=CARTESIAN_POINT('Ctrl Pts',(41.8433044092251,2.00847087481128,-2.52036020706156));
#77122=CARTESIAN_POINT('Ctrl Pts',(41.844172130646,2.01949800274255,-2.51153180223163));
#77123=CARTESIAN_POINT('Ctrl Pts',(41.8445922085786,2.0248141659362,-2.50724784753738));
#77124=CARTESIAN_POINT('Ctrl Pts',(41.8457065766934,2.03885755325565,-2.49585738914383));
#77125=CARTESIAN_POINT('Ctrl Pts',(41.8464020326518,2.04756117427818,-2.48872205395502));
#77126=CARTESIAN_POINT('Ctrl Pts',(41.8488722893242,2.07826061597207,-2.46328422448105));
#77127=CARTESIAN_POINT('Ctrl Pts',(41.8506571533664,2.10004934835103,-2.44473495655003));
#77128=CARTESIAN_POINT('Ctrl Pts',(41.8528744087912,2.12662757904884,-2.42149076634008));
#77129=CARTESIAN_POINT('Ctrl Pts',(41.8532955067176,2.13165373860917,-2.41706738197877));
#77130=CARTESIAN_POINT('Ctrl Pts',(41.8696681866981,2.32623850712508,-2.24473969602674));
#77131=CARTESIAN_POINT('Ctrl Pts',(41.8865940554169,2.49532658028293,-2.05512492662079));
#77132=CARTESIAN_POINT('Ctrl Pts',(41.9175801968807,2.75780891158807,-1.68003038129437));
#77133=CARTESIAN_POINT('Ctrl Pts',(41.9314665902514,2.8589310548206,-1.5015138538914));
#77134=CARTESIAN_POINT('Ctrl Pts',(41.9453847689313,2.94854310027333,-1.30093616725125));
#77135=CARTESIAN_POINT('Ctrl Pts',(41.9463272765626,2.95454989162051,-1.28723590835997));
#77136=CARTESIAN_POINT('Ctrl Pts',(41.9476354298151,2.96280383584513,-1.26804816076304));
#77137=CARTESIAN_POINT('Ctrl Pts',(41.9480058218087,2.96513145525455,-1.26259580314025));
#77138=CARTESIAN_POINT('Ctrl Pts',(41.9486340300147,2.96906344650798,-1.25331442491127));
#77139=CARTESIAN_POINT('Ctrl Pts',(41.9488923120766,2.97067548173606,-1.249488687402));
#77140=CARTESIAN_POINT('Ctrl Pts',(41.9493838139719,2.973734497994,-1.24218954103691));
#77141=CARTESIAN_POINT('Ctrl Pts',(41.9496171152882,2.97518279046933,-1.2387167085592));
#77142=CARTESIAN_POINT('Ctrl Pts',(41.9501655802575,2.97857864925566,-1.2305335317448));
#77143=CARTESIAN_POINT('Ctrl Pts',(41.9504804348797,2.98052113659516,-1.22582107083507));
#77144=CARTESIAN_POINT('Ctrl Pts',(41.9514088365538,2.98622793670706,-1.21188265099598));
#77145=CARTESIAN_POINT('Ctrl Pts',(41.9520205110591,2.98996069258822,-1.20264371806954));
#77146=CARTESIAN_POINT('Ctrl Pts',(41.9577860711542,3.0248788786772,-1.11505033344076));
#77147=CARTESIAN_POINT('Ctrl Pts',(41.9627674763962,3.05302338059868,-1.03550977188465));
#77148=CARTESIAN_POINT('Ctrl Pts',(41.9689647025155,3.0847621278938,-0.933208618793959));
#77149=CARTESIAN_POINT('Ctrl Pts',(41.9702741390275,3.09127670787651,-0.911396765009225));
#77150=CARTESIAN_POINT('Ctrl Pts',(41.9872816734895,3.17327016891815,-0.625871536357382));
#77151=CARTESIAN_POINT('Ctrl Pts',(42.0021201130746,3.21501338363019,-0.353639111426309));
#77152=CARTESIAN_POINT('Ctrl Pts',(42.0220536919655,3.22351668149749,-0.00859460259406048));
#77153=CARTESIAN_POINT('Ctrl Pts',(42.0261982704399,3.22292700887958,0.0622425999063536));
#77154=CARTESIAN_POINT('Ctrl Pts',(42.0329938607677,3.21821452912751,0.176334783075657));
#77155=CARTESIAN_POINT('Ctrl Pts',(42.0356003462993,3.21555004051634,0.219627806610689));
#77156=CARTESIAN_POINT('Ctrl Pts',(42.0390099496316,3.21097114394594,0.275581173165909));
#77157=CARTESIAN_POINT('Ctrl Pts',(42.0397879427736,3.20985384921835,0.288303537209825));
#77158=CARTESIAN_POINT('Ctrl Pts',(42.0410521228458,3.20792142860916,0.308901861826796));
#77159=CARTESIAN_POINT('Ctrl Pts',(42.0415368405485,3.20715283873196,0.316782132723543));
#77160=CARTESIAN_POINT('Ctrl Pts',(42.0424668050541,3.20562544513741,0.33186675951989));
#77161=CARTESIAN_POINT('Ctrl Pts',(42.0429118998262,3.20487137341624,0.339071554511315));
#77162=CARTESIAN_POINT('Ctrl Pts',(42.0439265889121,3.20310001200219,0.355462076680321));
#77163=CARTESIAN_POINT('Ctrl Pts',(42.0444966610165,3.20206749166539,0.364646062388857));
#77164=CARTESIAN_POINT('Ctrl Pts',(42.0462728769578,3.19873470559984,0.393184072532111));
#77165=CARTESIAN_POINT('Ctrl Pts',(42.0474833073904,3.1962983953354,0.412521481607143));
#77166=CARTESIAN_POINT('Ctrl Pts',(42.0639891261544,3.16084995727654,0.674684441067923));
#77167=CARTESIAN_POINT('Ctrl Pts',(42.0802000346239,3.10042847582344,0.912944539942265));
#77168=CARTESIAN_POINT('Ctrl Pts',(42.1072065135864,2.95879320926322,1.28670195239714));
#77169=CARTESIAN_POINT('Ctrl Pts',(42.1177387300236,2.89361241487982,1.42725938533381));
#77170=CARTESIAN_POINT('Ctrl Pts',(42.1318322435664,2.79039191269221,1.6134470581878));
#77171=CARTESIAN_POINT('Ctrl Pts',(42.1356370463925,2.76082646241958,1.66353134312558));
#77172=CARTESIAN_POINT('Ctrl Pts',(42.1413968535095,2.71318252853803,1.73946829539321));
#77173=CARTESIAN_POINT('Ctrl Pts',(42.1433999175532,2.69605396852741,1.76589992967303));
#77174=CARTESIAN_POINT('Ctrl Pts',(42.1458697087813,2.6741928749655,1.79857475317515));
#77175=CARTESIAN_POINT('Ctrl Pts',(42.1463593146701,2.66982212924108,1.80505636380382));
#77176=CARTESIAN_POINT('Ctrl Pts',(42.1471322803188,2.66286220585679,1.8152970190725));
#77177=CARTESIAN_POINT('Ctrl Pts',(42.1474166757966,2.66028858779679,1.81906652574608));
#77178=CARTESIAN_POINT('Ctrl Pts',(42.1479513333705,2.65542577391065,1.82615656165483));
#77179=CARTESIAN_POINT('Ctrl Pts',(42.1482017085895,2.65313837983643,1.82947822235146));
#77180=CARTESIAN_POINT('Ctrl Pts',(42.1487738901179,2.64788776658259,1.83707239168229));
#77181=CARTESIAN_POINT('Ctrl Pts',(42.1490954117769,2.64492044502432,1.84134202067219));
#77182=CARTESIAN_POINT('Ctrl Pts',(42.150084908614,2.63573676987695,1.85448825239833));
#77183=CARTESIAN_POINT('Ctrl Pts',(42.1507505615988,2.62948588847686,1.86334080846466));
#77184=CARTESIAN_POINT('Ctrl Pts',(42.1561584858292,2.57811911551218,1.93531365995502));
#77185=CARTESIAN_POINT('Ctrl Pts',(42.1607554418366,2.53077780660235,1.99682323705733));
#77186=CARTESIAN_POINT('Ctrl Pts',(42.1826618000868,2.29004689214005,2.28726594393112));
#77187=CARTESIAN_POINT('Ctrl Pts',(42.1987330626371,2.06759082090384,2.49018049204545));
#77188=CARTESIAN_POINT('Ctrl Pts',(42.2167267425001,1.81004140527699,2.66646240289804));
#77189=CARTESIAN_POINT('Ctrl Pts',(42.2174439808744,1.79975849288206,2.67341372982728));
#77190=CARTESIAN_POINT('Ctrl Pts',(42.2181629331785,1.7894362082953,2.68030513541681));
#77191=CARTESIAN_POINT('Origin',(-1.72497344927317,0.,0.));
#77192=CARTESIAN_POINT('',(43.716926315029,1.78943621037803,2.68030513402633));
#77193=CARTESIAN_POINT('',(43.4684957936438,1.78943612473158,2.68030519120596));
#77194=CARTESIAN_POINT('',(-1.72497344927317,1.78943621037804,2.68030513402633));
#77195=CARTESIAN_POINT('',(42.8965734492311,-3.22274897654346,-0.00256840185549188));
#77196=CARTESIAN_POINT('Ctrl Pts',(42.8965734492731,-3.22274897654292,-0.00256840253464825));
#77197=CARTESIAN_POINT('Ctrl Pts',(42.9070119662925,-3.22261461734424,-0.171158008007782));
#77198=CARTESIAN_POINT('Ctrl Pts',(42.9174504833119,-3.20924843949099,-0.339234248199928));
#77199=CARTESIAN_POINT('Ctrl Pts',(42.9278890003314,-3.18290631195516,-0.50519795309958));
#77200=CARTESIAN_POINT('Ctrl Pts',(42.9340612484241,-3.16733033060296,-0.603331544212998));
#77201=CARTESIAN_POINT('Ctrl Pts',(42.9402334965167,-3.14718428142756,-0.700916841221411));
#77202=CARTESIAN_POINT('Ctrl Pts',(42.9464057446094,-3.12251810559492,-0.797494979753408));
#77203=CARTESIAN_POINT('Ctrl Pts',(42.9525696332619,-3.09788533662103,-0.893942316808363));
#77204=CARTESIAN_POINT('Ctrl Pts',(42.9587335219145,-3.06874471543247,-0.989384789434819));
#77205=CARTESIAN_POINT('Ctrl Pts',(42.964897410567,-3.03519763550417,-1.08337107028473));
#77206=CARTESIAN_POINT('Ctrl Pts',(42.9710547722254,-3.00168607886396,-1.17725782826295));
#77207=CARTESIAN_POINT('Ctrl Pts',(42.9772121338839,-2.96377748522139,-1.26969105321386));
#77208=CARTESIAN_POINT('Ctrl Pts',(42.9833694955423,-2.92162350864595,-1.36023293454736));
#77209=CARTESIAN_POINT('Ctrl Pts',(42.9895223596885,-2.87950032253498,-1.45070868151334));
#77210=CARTESIAN_POINT('Ctrl Pts',(42.9956752238347,-2.83313810149224,-1.53929543890168));
#77211=CARTESIAN_POINT('Ctrl Pts',(43.0018280879809,-2.78273688404737,-1.62557466659096));
#77212=CARTESIAN_POINT('Ctrl Pts',(43.0079786211174,-2.73235476108069,-1.71182120743428));
#77213=CARTESIAN_POINT('Ctrl Pts',(43.0141291542538,-2.67793690101353,-1.79576158097013));
#77214=CARTESIAN_POINT('Ctrl Pts',(43.0202796873903,-2.61972920577409,-1.87700198479231));
#77215=CARTESIAN_POINT('Ctrl Pts',(43.0264295356054,-2.56152799252431,-1.95823334171003));
#77216=CARTESIAN_POINT('Ctrl Pts',(43.0325793838205,-2.49953803615927,-2.03676497358742));
#77217=CARTESIAN_POINT('Ctrl Pts',(43.0387292320356,-2.43404788848853,-2.11223304562837));
#77218=CARTESIAN_POINT('Ctrl Pts',(43.0448800404146,-2.36854751596743,-2.18771290035377));
#77219=CARTESIAN_POINT('Ctrl Pts',(43.0510308487937,-2.29954615141603,-2.26012791709842));
#77220=CARTESIAN_POINT('Ctrl Pts',(43.0571816571727,-2.22737117436342,-2.32914903218212));
#77221=CARTESIAN_POINT('Ctrl Pts',(43.0633390435388,-2.15511900972256,-2.3982439619538));
#77222=CARTESIAN_POINT('Ctrl Pts',(43.0694964299049,-2.07968676961233,-2.46393744130707));
#77223=CARTESIAN_POINT('Ctrl Pts',(43.075653816271,-2.00143699861166,-2.52593893494842));
#77224=CARTESIAN_POINT('Ctrl Pts',(43.0818146390078,-1.92314355725967,-2.58797503095313));
#77225=CARTESIAN_POINT('Ctrl Pts',(43.0879754617447,-1.84202980618773,-2.64631478423596));
#77226=CARTESIAN_POINT('Ctrl Pts',(43.0941362844816,-1.75848779783016,-2.70071068931539));
#77227=CARTESIAN_POINT('Ctrl Pts',(43.1003074073982,-1.67480611694209,-2.75519753802739));
#77228=CARTESIAN_POINT('Ctrl Pts',(43.1064785303148,-1.58868844433504,-2.80572714798561));
#77229=CARTESIAN_POINT('Ctrl Pts',(43.1126496532314,-1.50055209231866,-2.85209764572289));
#77230=CARTESIAN_POINT('Ctrl Pts',(43.1173451751779,-1.43349036290944,-2.88738031514006));
#77231=CARTESIAN_POINT('Ctrl Pts',(43.1220406971245,-1.36526044633556,-2.92025602217248));
#77232=CARTESIAN_POINT('Ctrl Pts',(43.1267362190711,-1.29605301174589,-2.95065486854095));
#77233=CARTESIAN_POINT('Ctrl Pts',(43.1329084671636,-1.20508006752428,-2.99061405170496));
#77234=CARTESIAN_POINT('Ctrl Pts',(43.1390807152562,-1.11209727072552,-3.02643238484143));
#77235=CARTESIAN_POINT('Ctrl Pts',(43.1452529633488,-1.01751762584899,-3.0579037662403));
#77236=CARTESIAN_POINT('Ctrl Pts',(43.1514168520012,-0.923066075771607,
-3.08933252408858));
#77237=CARTESIAN_POINT('Ctrl Pts',(43.1575807406536,-0.82702238475968,-3.11642589598497));
#77238=CARTESIAN_POINT('Ctrl Pts',(43.163744629306,-0.729821037891639,-3.1390251377061));
#77239=CARTESIAN_POINT('Ctrl Pts',(43.1699019909644,-0.632722618355907,
-3.16160044889809));
#77240=CARTESIAN_POINT('Ctrl Pts',(43.1760593526227,-0.534469400830379,
-3.1796909931772));
#77241=CARTESIAN_POINT('Ctrl Pts',(43.1822167142811,-0.435511676394324,
-3.19318761462965));
#77242=CARTESIAN_POINT('Ctrl Pts',(43.1883695784272,-0.33662623349731,-3.20667437776558));
#77243=CARTESIAN_POINT('Ctrl Pts',(43.1945224425733,-0.237037735879731,
-3.21557383092338));
#77244=CARTESIAN_POINT('Ctrl Pts',(43.2006753067194,-0.137206426103824,
-3.21982793936816));
#77245=CARTESIAN_POINT('Ctrl Pts',(43.2068258398557,-0.0374129373740154,
-3.2240804361459));
#77246=CARTESIAN_POINT('Ctrl Pts',(43.212976372992,0.0626227472322829,-3.22369106662332));
#77247=CARTESIAN_POINT('Ctrl Pts',(43.2191269061283,0.16243639593016,-3.21865375270115));
#77248=CARTESIAN_POINT('Ctrl Pts',(43.2252767543433,0.262238929413218,-3.21361699973259));
#77249=CARTESIAN_POINT('Ctrl Pts',(43.2314266025583,0.361819042322848,-3.20393335330992));
#77250=CARTESIAN_POINT('Ctrl Pts',(43.2375764507733,0.460714650667325,-3.18964881658788));
#77251=CARTESIAN_POINT('Ctrl Pts',(43.2437272591523,0.559625699392309,-3.17536204964869));
#77252=CARTESIAN_POINT('Ctrl Pts',(43.2498780675312,0.657851601325742,-3.15647302772775));
#77253=CARTESIAN_POINT('Ctrl Pts',(43.2560288759101,0.754938527703059,-3.13307921730197));
#77254=CARTESIAN_POINT('Ctrl Pts',(43.2621862622761,0.85212928377311,-3.10966038834652));
#77255=CARTESIAN_POINT('Ctrl Pts',(43.2683436486421,0.948178208798035,-3.08172725248936));
#77256=CARTESIAN_POINT('Ctrl Pts',(43.2745010350081,1.04264487033308,-3.04942769005401));
#77257=CARTESIAN_POINT('Ctrl Pts',(43.2806618577448,1.13716425269073,-3.01711010158202));
#77258=CARTESIAN_POINT('Ctrl Pts',(43.2868226804816,1.23009920894446,-2.98042139307577));
#77259=CARTESIAN_POINT('Ctrl Pts',(43.2929835032183,1.32102954851137,-2.93955753378971));
#77260=CARTESIAN_POINT('Ctrl Pts',(43.2991546261348,1.41211191304002,-2.89862535487926));
#77261=CARTESIAN_POINT('Ctrl Pts',(43.3053257490513,1.50118257871883,-2.85350427850703));
#77262=CARTESIAN_POINT('Ctrl Pts',(43.3114968719678,1.58784608274892,-2.80443619645712));
#77263=CARTESIAN_POINT('Ctrl Pts',(43.3161923939154,1.65378714254311,-2.76710097249347));
#77264=CARTESIAN_POINT('Ctrl Pts',(43.3208879158631,1.71833509488387,-2.72748158986566));
#77265=CARTESIAN_POINT('Ctrl Pts',(43.3255834378107,1.78132804395446,-2.68570064644617));
#77266=CARTESIAN_POINT('Ctrl Pts',(43.3317556859043,1.86413206747814,-2.63077973429977));
#77267=CARTESIAN_POINT('Ctrl Pts',(43.3379279339978,1.94453951891321,-2.57192911623941));
#77268=CARTESIAN_POINT('Ctrl Pts',(43.3441001820914,2.02215370790222,-2.50938477402676));
#77269=CARTESIAN_POINT('Ctrl Pts',(43.3502640707448,2.09966277941113,-2.44692513931068));
#77270=CARTESIAN_POINT('Ctrl Pts',(43.3564279593983,2.17438577251549,-2.38078199387189));
#77271=CARTESIAN_POINT('Ctrl Pts',(43.3625918480517,2.24595421962877,-2.31123499580457));
#77272=CARTESIAN_POINT('Ctrl Pts',(43.3687492097111,2.31744688230509,-2.24176164164463));
#77273=CARTESIAN_POINT('Ctrl Pts',(43.3749065713704,2.38579133017254,-2.16889190173063));
#77274=CARTESIAN_POINT('Ctrl Pts',(43.3810639330298,2.45065226330621,-2.09294554321228));
#77275=CARTESIAN_POINT('Ctrl Pts',(43.3872167971769,2.5154658201679,-2.01705465807619));
#77276=CARTESIAN_POINT('Ctrl Pts',(43.393369661324,2.57680063986894,-1.93809195156581));
#77277=CARTESIAN_POINT('Ctrl Pts',(43.3995225254711,2.63435904520707,-1.8564132038519));
#77278=CARTESIAN_POINT('Ctrl Pts',(43.4056730586084,2.69189564456962,-1.77476540009426));
#77279=CARTESIAN_POINT('Ctrl Pts',(43.4118235917457,2.74565842241112,-1.69040395436823));
#77280=CARTESIAN_POINT('Ctrl Pts',(43.4179741248831,2.79539125090078,-1.60371609609911));
#77281=CARTESIAN_POINT('Ctrl Pts',(43.4241239730991,2.84511854115916,-1.51703789136114));
#77282=CARTESIAN_POINT('Ctrl Pts',(43.4302738213151,2.89081655813809,-1.42803416592069));
#77283=CARTESIAN_POINT('Ctrl Pts',(43.4364236695311,2.9322741465557,-1.3371185033276));
#77284=CARTESIAN_POINT('Ctrl Pts',(43.442574477911,2.97373820766652,-1.24618864624771));
#77285=CARTESIAN_POINT('Ctrl Pts',(43.448725286291,3.01096034497466,-1.15334665436403));
#77286=CARTESIAN_POINT('Ctrl Pts',(43.4548760946709,3.04377715828944,-1.05902699360096));
#77287=CARTESIAN_POINT('Ctrl Pts',(43.4610334810379,3.07662906757199,-0.964606462599733));
#77288=CARTESIAN_POINT('Ctrl Pts',(43.4671908674048,3.10506610190875,-0.86870551808728));
#77289=CARTESIAN_POINT('Ctrl Pts',(43.4733482537718,3.1289745132135,-0.771774616167423));
#77290=CARTESIAN_POINT('Ctrl Pts',(43.4795090765095,3.15289626754413,-0.674789618159069));
#77291=CARTESIAN_POINT('Ctrl Pts',(43.4856698992473,3.1722842813181,-0.57677394415378));
#77292=CARTESIAN_POINT('Ctrl Pts',(43.491830721985,3.18707620426854,-0.478187024798082));
#77293=CARTESIAN_POINT('Ctrl Pts',(43.4980018449024,3.20189285759529,-0.379435279569272));
#77294=CARTESIAN_POINT('Ctrl Pts',(43.5041729678199,3.21209802686905,-0.280110813597029));
#77295=CARTESIAN_POINT('Ctrl Pts',(43.5103440907373,3.21768136283026,-0.180677087077551));
#77296=CARTESIAN_POINT('Ctrl Pts',(43.515039612675,3.22192964581572,-0.105019342050436));
#77297=CARTESIAN_POINT('Ctrl Pts',(43.5197351346127,3.22350320671854,-0.0292984234542198));
#77298=CARTESIAN_POINT('Ctrl Pts',(43.5244306565504,3.22241763723597,0.046283190583255));
#77299=CARTESIAN_POINT('Ctrl Pts',(43.5306030380365,3.22099062889376,0.145637120000158));
#77300=CARTESIAN_POINT('Ctrl Pts',(43.5367754195226,3.21496186675561,0.24509986855709));
#77301=CARTESIAN_POINT('Ctrl Pts',(43.5429478010087,3.20431536576978,0.34421010907832));
#77302=CARTESIAN_POINT('Ctrl Pts',(43.5491117885684,3.19368334314145,0.4431855679002));
#77303=CARTESIAN_POINT('Ctrl Pts',(43.555275776128,3.17844610962596,0.541809043401481));
#77304=CARTESIAN_POINT('Ctrl Pts',(43.5614397636877,3.15863968518723,0.639619341218158));
#77305=CARTESIAN_POINT('Ctrl Pts',(43.5679183699936,3.13782231250054,0.742422016609864));
#77306=CARTESIAN_POINT('Ctrl Pts',(43.5743969762995,3.11195693817601,0.844325818887086));
#77307=CARTESIAN_POINT('Ctrl Pts',(43.5808755826054,3.08114727120735,0.944801066696865));
#77308=CARTESIAN_POINT('Ctrl Pts',(43.5870281944349,3.05188790391388,1.04022053950578));
#77309=CARTESIAN_POINT('Ctrl Pts',(43.5931808062643,3.01816985646978,1.13435124988518));
#77310=CARTESIAN_POINT('Ctrl Pts',(43.5993334180938,2.98013405524829,1.2267512279388));
#77311=CARTESIAN_POINT('Ctrl Pts',(43.6054837360839,2.94211243467417,1.31911675709262));
#77312=CARTESIAN_POINT('Ctrl Pts',(43.611634054074,2.89977642460012,1.40975243503371));
#77313=CARTESIAN_POINT('Ctrl Pts',(43.6177843720641,2.85331575527376,1.49823454879619));
#77314=CARTESIAN_POINT('Ctrl Pts',(43.6239340422079,2.80685997990089,1.58670734225926));
#77315=CARTESIAN_POINT('Ctrl Pts',(43.6300837123518,2.75628061150776,1.67302663827981));
#77316=CARTESIAN_POINT('Ctrl Pts',(43.6362333824957,2.70181371112788,1.75679259813484));
#77317=CARTESIAN_POINT('Ctrl Pts',(43.6423840497997,2.64733797901842,1.84057214051983));
#77318=CARTESIAN_POINT('Ctrl Pts',(43.6485347171037,2.58897370006314,1.92179716055282));
#77319=CARTESIAN_POINT('Ctrl Pts',(43.6546853844077,2.52700013232355,2.00009697108334));
#77320=CARTESIAN_POINT('Ctrl Pts',(43.6608420666493,2.46496595861666,2.07847335354493));
#77321=CARTESIAN_POINT('Ctrl Pts',(43.6669987488909,2.39931572077314,2.15391847552512));
#77322=CARTESIAN_POINT('Ctrl Pts',(43.6731554311325,2.33036866048638,2.2260951167286));
#77323=CARTESIAN_POINT('Ctrl Pts',(43.6793156067755,2.26138247851965,2.29831271212862));
#77324=CARTESIAN_POINT('Ctrl Pts',(43.6854757824184,2.18909606308223,2.36725783414701));
#77325=CARTESIAN_POINT('Ctrl Pts',(43.6916359580614,2.11386373381855,2.43263184171931));
#77326=CARTESIAN_POINT('Ctrl Pts',(43.6978049516411,2.0385237138061,2.49809942842036));
#77327=CARTESIAN_POINT('Ctrl Pts',(43.7039739452209,1.96022970289234,2.55998542821244));
#77328=CARTESIAN_POINT('Ctrl Pts',(43.7101429388007,1.87936695546459,2.61803311843219));
#77329=CARTESIAN_POINT('Ctrl Pts',(43.7124040642101,1.84972827769303,2.63930937777946));
#77330=CARTESIAN_POINT('Ctrl Pts',(43.7146651896196,1.81974476091569,2.66007041629675));
#77331=CARTESIAN_POINT('Ctrl Pts',(43.716926315029,1.78943621037803,2.68030513402633));
#77332=CARTESIAN_POINT('Ctrl Pts',(42.4668644404635,1.78943621037806,2.68030513402631));
#77333=CARTESIAN_POINT('Ctrl Pts',(42.4730228196522,1.7063097483104,2.73580236058314));
#77334=CARTESIAN_POINT('Ctrl Pts',(42.4791811988409,1.62065192585895,2.78739362741565));
#77335=CARTESIAN_POINT('Ctrl Pts',(42.4853395780296,1.53287140170373,2.83485851998629));
#77336=CARTESIAN_POINT('Ctrl Pts',(42.4915018923073,1.44503478743852,2.88235374173382));
#77337=CARTESIAN_POINT('Ctrl Pts',(42.4976642065849,1.35507316197229,2.92571715166353));
#77338=CARTESIAN_POINT('Ctrl Pts',(42.5038265208625,1.26341635432497,2.96477599122163));
#77339=CARTESIAN_POINT('Ctrl Pts',(42.5099985241704,1.17161543432828,3.00389624314262));
#77340=CARTESIAN_POINT('Ctrl Pts',(42.5161705274784,1.07811441805955,3.03869826355687));
#77341=CARTESIAN_POINT('Ctrl Pts',(42.5223425307863,0.983359410082434,3.069058786192));
#77342=CARTESIAN_POINT('Ctrl Pts',(42.5249598748083,0.943176921300858,3.08193368733162));
#77343=CARTESIAN_POINT('Ctrl Pts',(42.5275772188302,0.902769061359369,3.09401048815375));
#77344=CARTESIAN_POINT('Ctrl Pts',(42.5301945628522,0.862170336031154,3.10528257557471));
#77345=CARTESIAN_POINT('Ctrl Pts',(42.5363668109449,0.766429996637244,3.13186453022073));
#77346=CARTESIAN_POINT('Ctrl Pts',(42.5425390590377,0.669290652049423,3.15406140438831));
#77347=CARTESIAN_POINT('Ctrl Pts',(42.5487113071304,0.571190470249088,3.17172807932783));
#77348=CARTESIAN_POINT('Ctrl Pts',(42.554875195783,0.473223151318917,3.18937082724607));
#77349=CARTESIAN_POINT('Ctrl Pts',(42.5610390844356,0.374298005424443,3.20249549464088));
#77350=CARTESIAN_POINT('Ctrl Pts',(42.5672029730882,0.274867710449411,3.2110068988173));
#77351=CARTESIAN_POINT('Ctrl Pts',(42.5733603347467,0.175542703058871,3.21950929019549));
#77352=CARTESIAN_POINT('Ctrl Pts',(42.5795176964052,0.0757140404387358,
3.22340809340008));
#77353=CARTESIAN_POINT('Ctrl Pts',(42.5856750580637,-0.0241570242698424,
3.22265946086124));
#77354=CARTESIAN_POINT('Ctrl Pts',(42.59182792221,-0.123955140309737,3.22191137514491));
#77355=CARTESIAN_POINT('Ctrl Pts',(42.5979807863562,-0.223795163807456,
3.21652260601525));
#77356=CARTESIAN_POINT('Ctrl Pts',(42.6041336505025,-0.323213279610985,
3.20650132362098));
#77357=CARTESIAN_POINT('Ctrl Pts',(42.610284183639,-0.422593730906763,3.19648383778497));
#77358=CARTESIAN_POINT('Ctrl Pts',(42.6164347167755,-0.521552160403222,
3.18183736942622));
#77359=CARTESIAN_POINT('Ctrl Pts',(42.622585249912,-0.619628211402932,3.1626220833564));
#77360=CARTESIAN_POINT('Ctrl Pts',(42.6287350981272,-0.717693340686126,
3.14340893709447));
#77361=CARTESIAN_POINT('Ctrl Pts',(42.6348849463424,-0.81487586055913,3.11962806817058));
#77362=CARTESIAN_POINT('Ctrl Pts',(42.6410347945575,-0.910724964878155,
3.09139088451261));
#77363=CARTESIAN_POINT('Ctrl Pts',(42.6471856029366,-1.00658903393289,3.06314929223765));
#77364=CARTESIAN_POINT('Ctrl Pts',(42.6533364113157,-1.10111885721787,3.03045012604058));
#77365=CARTESIAN_POINT('Ctrl Pts',(42.6594872196948,-1.19387913610439,2.99345455467001));
#77366=CARTESIAN_POINT('Ctrl Pts',(42.665644606061,-1.28673861754694,2.95641941835542));
#77367=CARTESIAN_POINT('Ctrl Pts',(42.6718019924271,-1.37782437132591,2.91507886276786));
#77368=CARTESIAN_POINT('Ctrl Pts',(42.6779593787933,-1.46672154529698,2.8696420458067));
#77369=CARTESIAN_POINT('Ctrl Pts',(42.6841202015302,-1.55566833181994,2.82417987104912));
#77370=CARTESIAN_POINT('Ctrl Pts',(42.6902810242672,-1.64242372891095,2.77461709770201));
#77371=CARTESIAN_POINT('Ctrl Pts',(42.6964418470041,-1.72659977509332,2.72120759574636));
#77372=CARTESIAN_POINT('Ctrl Pts',(42.7026129699207,-1.81091655384361,2.66770879930966));
#77373=CARTESIAN_POINT('Ctrl Pts',(42.7087840928374,-1.89264501213276,2.61035067762098));
#77374=CARTESIAN_POINT('Ctrl Pts',(42.714955215754,-1.97142821041354,2.54942902895642));
#77375=CARTESIAN_POINT('Ctrl Pts',(42.7196507377,-2.03137325469363,2.5030745903641));
#77376=CARTESIAN_POINT('Ctrl Pts',(42.7243462596459,-2.08961379107395,2.45465792433793));
#77377=CARTESIAN_POINT('Ctrl Pts',(42.7290417815918,-2.14600705485164,2.4043234564066));
#77378=CARTESIAN_POINT('Ctrl Pts',(42.7351222412986,-2.21903343447167,2.33914290616189));
#77379=CARTESIAN_POINT('Ctrl Pts',(42.7412027010054,-2.28923440967352,2.27050086199092));
#77380=CARTESIAN_POINT('Ctrl Pts',(42.7472831607122,-2.35625617205213,2.19867560457796));
#77381=CARTESIAN_POINT('Ctrl Pts',(42.7535035894005,-2.42482074011787,2.12519696755092));
#77382=CARTESIAN_POINT('Ctrl Pts',(42.7597240180888,-2.49005751577951,2.04838699778255));
#77383=CARTESIAN_POINT('Ctrl Pts',(42.7659444467771,-2.55162278540211,1.96858800248217));
#77384=CARTESIAN_POINT('Ctrl Pts',(42.7720094906818,-2.61165016968376,1.89078236651974));
#77385=CARTESIAN_POINT('Ctrl Pts',(42.7780745345866,-2.66818700987442,1.81013564901337));
#77386=CARTESIAN_POINT('Ctrl Pts',(42.7841395784913,-2.72095245481611,1.72700182429845));
#77387=CARTESIAN_POINT('Ctrl Pts',(42.7902008683294,-2.77368523964853,1.64391945674082));
#77388=CARTESIAN_POINT('Ctrl Pts',(42.7962621581675,-2.82265102483982,1.55835341620575));
#77389=CARTESIAN_POINT('Ctrl Pts',(42.8023234480056,-2.86761118870067,1.47068814945205));
#77390=CARTESIAN_POINT('Ctrl Pts',(42.8083827193884,-2.91255638048725,1.38305207589457));
#77391=CARTESIAN_POINT('Ctrl Pts',(42.8144419907712,-2.95349839674967,1.29331856370545));
#77392=CARTESIAN_POINT('Ctrl Pts',(42.8205012621539,-2.99024425283826,1.2018971964639));
#77393=CARTESIAN_POINT('Ctrl Pts',(42.826840611077,-3.02868861165756,1.10625006179073));
#77394=CARTESIAN_POINT('Ctrl Pts',(42.8331799600001,-3.0625393141137,1.00875575114826));
#77395=CARTESIAN_POINT('Ctrl Pts',(42.8395193089232,-3.09163202552679,0.909906028794799));
#77396=CARTESIAN_POINT('Ctrl Pts',(42.8455824738989,-3.11945726610376,0.815362853825724));
#77397=CARTESIAN_POINT('Ctrl Pts',(42.8516456388745,-3.14293034275207,0.719580363387587));
#77398=CARTESIAN_POINT('Ctrl Pts',(42.8577088038502,-3.16195921200763,0.623002009707894));
#77399=CARTESIAN_POINT('Ctrl Pts',(42.8637745881198,-3.18099630175592,0.526381934071794));
#77400=CARTESIAN_POINT('Ctrl Pts',(42.8698403723895,-3.19558529637308,0.428965753991759));
#77401=CARTESIAN_POINT('Ctrl Pts',(42.8759061566592,-3.205685835828,0.331203690305177));
#77402=CARTESIAN_POINT('Ctrl Pts',(42.8819788888794,-3.21579794477583,0.233329646708139));
#77403=CARTESIAN_POINT('Ctrl Pts',(42.8880516210995,-3.22141131975012,0.13510937576864));
#77404=CARTESIAN_POINT('Ctrl Pts',(42.8941243533197,-3.22253766425402,0.0369941206709852));
#77405=CARTESIAN_POINT('Ctrl Pts',(42.8949407186235,-3.22268908021306,0.0238043591057623));
#77406=CARTESIAN_POINT('Ctrl Pts',(42.8957570839273,-3.22275948437315,0.0106164887023605));
#77407=CARTESIAN_POINT('Ctrl Pts',(42.8965734492311,-3.22274897654346,-0.00256840185549149));
#77408=CARTESIAN_POINT('Ctrl Pts',(42.2181629331785,1.7894362082953,2.68030513541681));
#77409=CARTESIAN_POINT('Ctrl Pts',(42.2217196605947,1.73837085614481,2.71439759336871));
#77410=CARTESIAN_POINT('Ctrl Pts',(42.2253186739974,1.68634193990611,2.7470235475656));
#77411=CARTESIAN_POINT('Ctrl Pts',(42.2316293281462,1.59486245394465,2.80080902053283));
#77412=CARTESIAN_POINT('Ctrl Pts',(42.2343155408901,1.55584615997304,2.82266892187229));
#77413=CARTESIAN_POINT('Ctrl Pts',(42.2378150347013,1.50499593401331,2.84978446799692));
#77414=CARTESIAN_POINT('Ctrl Pts',(42.2386015006529,1.49356652458364,2.85579118712937));
#77415=CARTESIAN_POINT('Ctrl Pts',(42.239876084008,1.47504297060026,2.86538461347792));
#77416=CARTESIAN_POINT('Ctrl Pts',(42.2403626868135,1.46797103474877,2.8690140793695));
#77417=CARTESIAN_POINT('Ctrl Pts',(42.2412940102413,1.45443607947318,2.87589735746737));
#77418=CARTESIAN_POINT('Ctrl Pts',(42.2417385698248,1.4479753795481,2.87915564338288));
#77419=CARTESIAN_POINT('Ctrl Pts',(42.2427583876119,1.4331551821444,2.88656732437899));
#77420=CARTESIAN_POINT('Ctrl Pts',(42.2433341504346,1.42478853231344,2.89070619910277));
#77421=CARTESIAN_POINT('Ctrl Pts',(42.2451136447508,1.39893238610334,2.90335738122805));
#77422=CARTESIAN_POINT('Ctrl Pts',(42.2463216153317,1.38138396410044,2.91174762316685));
#77423=CARTESIAN_POINT('Ctrl Pts',(42.2629444337684,1.13998320979188,3.02449261211886));
#77424=CARTESIAN_POINT('Ctrl Pts',(42.2792904611879,0.904980560503523,3.1029146491541));
#77425=CARTESIAN_POINT('Ctrl Pts',(42.3063450856634,0.513217508158918,3.18532149947807));
#77426=CARTESIAN_POINT('Ctrl Pts',(42.3167876425959,0.360982577635473,3.2061440865308));
#77427=CARTESIAN_POINT('Ctrl Pts',(42.3307667904361,0.150215664862116,3.2197650826473));
#77428=CARTESIAN_POINT('Ctrl Pts',(42.3345445296417,0.0924984469676575,
3.22193991328354));
#77429=CARTESIAN_POINT('Ctrl Pts',(42.3402680615161,0.00341235853275508,
3.22290057495599));
#77430=CARTESIAN_POINT('Ctrl Pts',(42.3422612323528,-0.027930546787336,
3.22278137969128));
#77431=CARTESIAN_POINT('Ctrl Pts',(42.3447205573488,-0.067071557395471,
3.22206143381895));
#77432=CARTESIAN_POINT('Ctrl Pts',(42.3452093619568,-0.0748745683871715,
3.22188955104423));
#77433=CARTESIAN_POINT('Ctrl Pts',(42.3459813525845,-0.0872368952137637,
3.2215723014069));
#77434=CARTESIAN_POINT('Ctrl Pts',(42.3462655699483,-0.0917965970982968,
3.2214456001082));
#77435=CARTESIAN_POINT('Ctrl Pts',(42.3468000807563,-0.100387869615858,
3.22118861730599));
#77436=CARTESIAN_POINT('Ctrl Pts',(42.3470504865306,-0.104419417348497,
3.22106044930886));
#77437=CARTESIAN_POINT('Ctrl Pts',(42.3476229871091,-0.113651970450272,
3.22074958280677));
#77438=CARTESIAN_POINT('Ctrl Pts',(42.3479447960978,-0.118852771066763,
3.22056185552321));
#77439=CARTESIAN_POINT('Ctrl Pts',(42.3489360504688,-0.134905837682814,
3.21994346741317));
#77440=CARTESIAN_POINT('Ctrl Pts',(42.3496031616894,-0.145756536208583,
3.21947054007426));
#77441=CARTESIAN_POINT('Ctrl Pts',(42.3550547446546,-0.234790786360319,
3.21513893386138));
#77442=CARTESIAN_POINT('Ctrl Pts',(42.359691272036,-0.312819599756684,3.2084873756921));
#77443=CARTESIAN_POINT('Ctrl Pts',(42.3756697738247,-0.586054586034389,
3.17513070920855));
#77444=CARTESIAN_POINT('Ctrl Pts',(42.3865082030507,-0.778987479177579,
3.1333855714471));
#77445=CARTESIAN_POINT('Ctrl Pts',(42.4089683434236,-1.16096633016335,3.01324690163493));
#77446=CARTESIAN_POINT('Ctrl Pts',(42.420564748736,-1.34877744233324,2.93398744304411));
#77447=CARTESIAN_POINT('Ctrl Pts',(42.4342155460878,-1.54829430158038,2.82655997206818));
#77448=CARTESIAN_POINT('Ctrl Pts',(42.4356216765461,-1.56861509404701,2.81533357940513));
#77449=CARTESIAN_POINT('Ctrl Pts',(42.4376466466783,-1.59753977939494,2.79894352188412));
#77450=CARTESIAN_POINT('Ctrl Pts',(42.4382590881115,-1.60624391988547,2.79395752503463));
#77451=CARTESIAN_POINT('Ctrl Pts',(42.4393224896502,-1.62128032860834,2.785250724596));
#77452=CARTESIAN_POINT('Ctrl Pts',(42.4397727649262,-1.62762345191738,2.78154874128539));
#77453=CARTESIAN_POINT('Ctrl Pts',(42.4406390223109,-1.63978076027161,2.77439765022244));
#77454=CARTESIAN_POINT('Ctrl Pts',(42.4410548816434,-1.6455968617693,2.77095186366352));
#77455=CARTESIAN_POINT('Ctrl Pts',(42.4420351073943,-1.65925830404118,2.76279987344018));
#77456=CARTESIAN_POINT('Ctrl Pts',(42.4426000262205,-1.66709450135167,2.75807853060882));
#77457=CARTESIAN_POINT('Ctrl Pts',(42.4442717860968,-1.69017392681571,2.74403878397038));
#77458=CARTESIAN_POINT('Ctrl Pts',(42.4453820551361,-1.70535970015946,2.73462703547898));
#77459=CARTESIAN_POINT('Ctrl Pts',(42.4579106220937,-1.87511046551275,2.62745608363986));
#77460=CARTESIAN_POINT('Ctrl Pts',(42.4698207573752,-2.02113623095133,2.51685371930569));
#77461=CARTESIAN_POINT('Ctrl Pts',(42.4889853753387,-2.23408158038254,2.32503035665892));
#77462=CARTESIAN_POINT('Ctrl Pts',(42.4960085769168,-2.30778320620272,2.25189298094657));
#77463=CARTESIAN_POINT('Ctrl Pts',(42.5159684578198,-2.50683552729827,2.03431145885023));
#77464=CARTESIAN_POINT('Ctrl Pts',(42.5288838874211,-2.62306039654953,1.88207829401876));
#77465=CARTESIAN_POINT('Ctrl Pts',(42.5419386110903,-2.73306808475678,1.70782854072295));
#77466=CARTESIAN_POINT('Ctrl Pts',(42.5428771848956,-2.74093336154571,1.69517663037139));
#77467=CARTESIAN_POINT('Ctrl Pts',(42.5441808258271,-2.7518006091536,1.67742242694465));
#77468=CARTESIAN_POINT('Ctrl Pts',(42.5445505964582,-2.75487653368268,1.6723659517125));
#77469=CARTESIAN_POINT('Ctrl Pts',(42.5451780624932,-2.76008530663172,1.66374994548331));
#77470=CARTESIAN_POINT('Ctrl Pts',(42.5454362211682,-2.76222523229623,1.66019473186239));
#77471=CARTESIAN_POINT('Ctrl Pts',(42.5459277162155,-2.76629348073228,1.65340621543178));
#77472=CARTESIAN_POINT('Ctrl Pts',(42.5461611332657,-2.76822300702437,1.65017366313347));
#77473=CARTESIAN_POINT('Ctrl Pts',(42.5467101788511,-2.77275552353652,1.64254997686655));
#77474=CARTESIAN_POINT('Ctrl Pts',(42.5470254967309,-2.77535376322781,1.63815600892932));
#77475=CARTESIAN_POINT('Ctrl Pts',(42.547956174419,-2.78300793308283,1.62514131236917));
#77476=CARTESIAN_POINT('Ctrl Pts',(42.5485696487335,-2.78803427190687,1.61650312265316));
#77477=CARTESIAN_POINT('Ctrl Pts',(42.5544040706871,-2.83564307919883,1.53380071315588));
#77478=CARTESIAN_POINT('Ctrl Pts',(42.5594479812322,-2.87530902560953,1.45808682188049));
#77479=CARTESIAN_POINT('Ctrl Pts',(42.5665251897491,-2.92775120725039,1.34749959431129));
#77480=CARTESIAN_POINT('Ctrl Pts',(42.5686415274892,-2.9430054581154,1.31384980308687));
#77481=CARTESIAN_POINT('Ctrl Pts',(42.5807315369125,-3.02737965235529,1.11887904927416));
#77482=CARTESIAN_POINT('Ctrl Pts',(42.5904003789349,-3.08380983833858,0.952385771762098));
#77483=CARTESIAN_POINT('Ctrl Pts',(42.6106707814109,-3.17115166698426,0.603250921046015));
#77484=CARTESIAN_POINT('Ctrl Pts',(42.6212639353053,-3.20046041095039,0.420896165356633));
#77485=CARTESIAN_POINT('Ctrl Pts',(42.6336276446777,-3.21552799154996,0.216604768133396));
#77486=CARTESIAN_POINT('Ctrl Pts',(42.6348710084127,-3.21684084956794,0.196144866243502));
#77487=CARTESIAN_POINT('Ctrl Pts',(42.6367017223952,-3.2184782250612,0.166151807952567));
#77488=CARTESIAN_POINT('Ctrl Pts',(42.6372842637606,-3.21895579505952,0.156627248115719));
#77489=CARTESIAN_POINT('Ctrl Pts',(42.6383128620846,-3.2197226315505,0.139844560690493));
#77490=CARTESIAN_POINT('Ctrl Pts',(42.6387583583515,-3.22002964847593,0.132587280073419));
#77491=CARTESIAN_POINT('Ctrl Pts',(42.6396281597261,-3.22058021168594,0.118440638948911));
#77492=CARTESIAN_POINT('Ctrl Pts',(42.6400523858353,-3.22082619323022,0.111551408241236));
#77493=CARTESIAN_POINT('Ctrl Pts',(42.6410727838833,-3.22136379854938,0.0950061273349007));
#77494=CARTESIAN_POINT('Ctrl Pts',(42.6416696220326,-3.22163411133951,0.085349494596543));
#77495=CARTESIAN_POINT('Ctrl Pts',(42.6438489790326,-3.22246069900972,0.0501653940528284));
#77496=CARTESIAN_POINT('Ctrl Pts',(42.6454396267255,-3.22275699725731,0.0246333012112815));
#77497=CARTESIAN_POINT('Ctrl Pts',(42.6545039466654,-3.22271665035957,-0.119996792985065));
#77498=CARTESIAN_POINT('Ctrl Pts',(42.6621734231361,-3.21608164533105,-0.238987172216434));
#77499=CARTESIAN_POINT('Ctrl Pts',(42.6809218207046,-3.18449910205122,-0.522075959496533));
#77500=CARTESIAN_POINT('Ctrl Pts',(42.6921395575668,-3.15343606146854,-0.685149989314532));
#77501=CARTESIAN_POINT('Ctrl Pts',(42.716099656827,-3.06058909433109,-1.02682877364644));
#77502=CARTESIAN_POINT('Ctrl Pts',(42.7287972074266,-2.99536474041529,-1.2039064197207));
#77503=CARTESIAN_POINT('Ctrl Pts',(42.741434267157,-2.9100165621998,-1.38494036336811));
#77504=CARTESIAN_POINT('Ctrl Pts',(42.7421744035054,-2.90493707545927,-1.39556325549378));
#77505=CARTESIAN_POINT('Ctrl Pts',(42.7432438988451,-2.89747767967071,-1.41094612664779));
#77506=CARTESIAN_POINT('Ctrl Pts',(42.7435760556443,-2.89514409452615,-1.4157282752676));
#77507=CARTESIAN_POINT('Ctrl Pts',(42.7441604016862,-2.89100868095609,-1.42414987297785));
#77508=CARTESIAN_POINT('Ctrl Pts',(42.7444128986318,-2.88921180460668,-1.42779172252958));
#77509=CARTESIAN_POINT('Ctrl Pts',(42.744941199931,-2.88543120662733,-1.43541775191868));
#77510=CARTESIAN_POINT('Ctrl Pts',(42.7452169162615,-2.88344611896537,-1.43940121241359));
#77511=CARTESIAN_POINT('Ctrl Pts',(42.7459440381348,-2.87817943924847,-1.44991520235635));
#77512=CARTESIAN_POINT('Ctrl Pts',(42.746394570686,-2.8748838499502,-1.45643874923965));
#77513=CARTESIAN_POINT('Ctrl Pts',(42.7484356644581,-2.85980815460908,-1.48603020650837));
#77514=CARTESIAN_POINT('Ctrl Pts',(42.7500106817074,-2.84777200580747,-1.50896758028767));
#77515=CARTESIAN_POINT('Ctrl Pts',(42.7637103489831,-2.73967162466017,-1.70907379045854));
#77516=CARTESIAN_POINT('Ctrl Pts',(42.7749436684661,-2.62744734433604,-1.87703945943681));
#77517=CARTESIAN_POINT('Ctrl Pts',(42.7997413760648,-2.34745020904844,-2.2213152346494));
#77518=CARTESIAN_POINT('Ctrl Pts',(42.8132833097584,-2.17398290814975,-2.39134771558752));
#77519=CARTESIAN_POINT('Ctrl Pts',(42.8282270159554,-1.97704674604733,-2.54508607217044));
#77520=CARTESIAN_POINT('Ctrl Pts',(42.8286887813643,-1.97095521375683,-2.5498063641481));
#77521=CARTESIAN_POINT('Ctrl Pts',(42.8308362774878,-1.94259868566993,-2.57161733758292));
#77522=CARTESIAN_POINT('Ctrl Pts',(42.8325321482607,-1.92012847228508,-2.58843813106864));
#77523=CARTESIAN_POINT('Ctrl Pts',(42.834918521569,-1.88841924799229,-2.61153497156755));
#77524=CARTESIAN_POINT('Ctrl Pts',(42.8355993476656,-1.87936255676633,-2.61806007173481));
#77525=CARTESIAN_POINT('Ctrl Pts',(42.8366984652818,-1.86472634305043,-2.62848998547855));
#77526=CARTESIAN_POINT('Ctrl Pts',(42.837115612308,-1.85916796995023,-2.63242443321941));
#77527=CARTESIAN_POINT('Ctrl Pts',(42.8379818988246,-1.84761796599909,-2.64054517833469));
#77528=CARTESIAN_POINT('Ctrl Pts',(42.8384311388199,-1.84162448528395,-2.64472876509274));
#77529=CARTESIAN_POINT('Ctrl Pts',(42.8394861546221,-1.82754045376776,-2.65448865214723));
#77530=CARTESIAN_POINT('Ctrl Pts',(42.8400925568614,-1.81943856258134,-2.66004838830055));
#77531=CARTESIAN_POINT('Ctrl Pts',(42.842065277114,-1.79306142615782,-2.67797220656704));
#77532=CARTESIAN_POINT('Ctrl Pts',(42.8434372753487,-1.77468490897253,-2.69018546794621));
#77533=CARTESIAN_POINT('Ctrl Pts',(42.8466619423443,-1.73142804882892,-2.71829840987218));
#77534=CARTESIAN_POINT('Ctrl Pts',(42.8485201017628,-1.70645205698459,-2.73404656458143));
#77535=CARTESIAN_POINT('Ctrl Pts',(42.8550680211417,-1.6182841110775,-2.7879604890752));
#77536=CARTESIAN_POINT('Ctrl Pts',(42.8598220203931,-1.55400410220819,-2.82429407492053));
#77537=CARTESIAN_POINT('Ctrl Pts',(42.8842274045853,-1.22263479200983,-2.99685840271323));
#77538=CARTESIAN_POINT('Ctrl Pts',(42.9049902663269,-0.938762874228008,
-3.09752787809967));
#77539=CARTESIAN_POINT('Ctrl Pts',(42.9298908095668,-0.56917769571837,-3.17303627705564));
#77540=CARTESIAN_POINT('Ctrl Pts',(42.9349214925085,-0.492712588071752,
-3.18580586511337));
#77541=CARTESIAN_POINT('Ctrl Pts',(42.940493130576,-0.405111871963003,-3.19720491967623));
#77542=CARTESIAN_POINT('Ctrl Pts',(42.9411735877429,-0.394361781473908,
-3.19854868970525));
#77543=CARTESIAN_POINT('Ctrl Pts',(42.9421761538398,-0.378443101331638,
-3.20045706252447));
#77544=CARTESIAN_POINT('Ctrl Pts',(42.9425005599095,-0.373279729674426,
-3.20106339117617));
#77545=CARTESIAN_POINT('Ctrl Pts',(42.9430753654353,-0.364108272558035,
-3.20211789186341));
#77546=CARTESIAN_POINT('Ctrl Pts',(42.9433260441527,-0.360100798837707,
-3.20257103635188));
#77547=CARTESIAN_POINT('Ctrl Pts',(42.9438595260158,-0.351555734270683,
-3.20352102600854));
#77548=CARTESIAN_POINT('Ctrl Pts',(42.9441422078362,-0.347017950873448,
-3.20401575226539));
#77549=CARTESIAN_POINT('Ctrl Pts',(42.9449076545637,-0.334704164156703,
-3.20533178080819));
#77550=CARTESIAN_POINT('Ctrl Pts',(42.9453893746934,-0.326926136581007,
-3.20613443367199));
#77551=CARTESIAN_POINT('Ctrl Pts',(42.9478048923463,-0.28778572483437,-3.21002960943406));
#77552=CARTESIAN_POINT('Ctrl Pts',(42.9497153166246,-0.256380799457424,
-3.21269042673705));
#77553=CARTESIAN_POINT('Ctrl Pts',(42.9550937780551,-0.166881663234144,
-3.21895253256684));
#77554=CARTESIAN_POINT('Ctrl Pts',(42.9585101707497,-0.108719765296343,
-3.22144156265614));
#77555=CARTESIAN_POINT('Ctrl Pts',(42.9708375407736,0.104314046705968,-3.22478143352988));
#77556=CARTESIAN_POINT('Ctrl Pts',(42.979444100391,0.259130744852789,-3.21604635687948));
#77557=CARTESIAN_POINT('Ctrl Pts',(42.9916223030091,0.475209588365181,-3.18814405554449));
#77558=CARTESIAN_POINT('Ctrl Pts',(42.9951481626782,0.537440841841549,-3.17824539833281));
#77559=CARTESIAN_POINT('Ctrl Pts',(43.0089115203352,0.777321840479593,-3.13284220569045));
#77560=CARTESIAN_POINT('Ctrl Pts',(43.0193336093857,0.952120201069912,-3.08421512959863));
#77561=CARTESIAN_POINT('Ctrl Pts',(43.0313476415777,1.13863229861123,-3.01495485959217));
#77562=CARTESIAN_POINT('Ctrl Pts',(43.0324302602187,1.15531705586102,-3.00860080393486));
#77563=CARTESIAN_POINT('Ctrl Pts',(43.0340744758414,1.18046729977594,-2.99878277931221));
#77564=CARTESIAN_POINT('Ctrl Pts',(43.0346326458818,1.18897243355327,-2.99542079729703));
#77565=CARTESIAN_POINT('Ctrl Pts',(43.0356054873813,1.20373859651637,-2.98951110450956));
#77566=CARTESIAN_POINT('Ctrl Pts',(43.0360196027049,1.21000616407742,-2.9869798014919));
#77567=CARTESIAN_POINT('Ctrl Pts',(43.0368851072826,1.22306754248793,-2.98165680425003));
#77568=CARTESIAN_POINT('Ctrl Pts',(43.037336614726,1.22985985904333,-2.97886156736226));
#77569=CARTESIAN_POINT('Ctrl Pts',(43.03840683849,1.24590892381344,-2.9721926600866));
#77570=CARTESIAN_POINT('Ctrl Pts',(43.0390262339669,1.25515721206088,-2.96829894459281));
#77571=CARTESIAN_POINT('Ctrl Pts',(43.0410847805439,1.28575945236797,-2.95524619477804));
#77572=CARTESIAN_POINT('Ctrl Pts',(43.0425303224932,1.3070321456878,-2.94589958512677));
#77573=CARTESIAN_POINT('Ctrl Pts',(43.0570334638071,1.51826965226037,-2.85034951259255));
#77574=CARTESIAN_POINT('Ctrl Pts',(43.0707352894934,1.69950509787366,-2.7461405804526));
#77575=CARTESIAN_POINT('Ctrl Pts',(43.0942041431959,1.98360901088827,-2.54383160767006));
#77576=CARTESIAN_POINT('Ctrl Pts',(43.1037523944928,2.09240987631214,-2.45511801006155));
#77577=CARTESIAN_POINT('Ctrl Pts',(43.1182881902953,2.25092515153934,-2.30765463485599));
#77578=CARTESIAN_POINT('Ctrl Pts',(43.123363085877,2.30490626242056,-2.25373966361566));
#77579=CARTESIAN_POINT('Ctrl Pts',(43.1319348510027,2.39447514355486,-2.15769263017475));
#77580=CARTESIAN_POINT('Ctrl Pts',(43.1354764983054,2.43098872175777,-2.11646956249706));
#77581=CARTESIAN_POINT('Ctrl Pts',(43.1395055754905,2.47215445009682,-2.06752243513258));
#77582=CARTESIAN_POINT('Ctrl Pts',(43.1400638809961,2.47785021912557,-2.06069283030513));
#77583=CARTESIAN_POINT('Ctrl Pts',(43.1409512307291,2.4868904535251,-2.0497613136018));
#77584=CARTESIAN_POINT('Ctrl Pts',(43.1412815706574,2.4902531609399,-2.04567464811875));
#77585=CARTESIAN_POINT('Ctrl Pts',(43.1418638260637,2.49617564900892,-2.03844086204139));
#77586=CARTESIAN_POINT('Ctrl Pts',(43.1421160421045,2.49873957186375,-2.03529717031141));
#77587=CARTESIAN_POINT('Ctrl Pts',(43.1426449316822,2.50411293160897,-2.02868329777976));
#77588=CARTESIAN_POINT('Ctrl Pts',(43.1429215129071,2.50692108792429,-2.025212126282));
#77589=CARTESIAN_POINT('Ctrl Pts',(43.1436533885243,2.51434669713987,-2.01599419507258));
#77590=CARTESIAN_POINT('Ctrl Pts',(43.1441077893007,2.51895169414898,-2.01023736733903));
#77591=CARTESIAN_POINT('Ctrl Pts',(43.146191814602,2.54004427037647,-1.98368269920788));
#77592=CARTESIAN_POINT('Ctrl Pts',(43.1478050834613,2.55629486997702,-1.96269676496711));
#77593=CARTESIAN_POINT('Ctrl Pts',(43.1621705348721,2.700051774668,-1.77223500856972));
#77594=CARTESIAN_POINT('Ctrl Pts',(43.1739400141392,2.81081599430541,-1.59073431099035));
#77595=CARTESIAN_POINT('Ctrl Pts',(43.1998773356525,3.01238978044801,-1.172657197809));
#77596=CARTESIAN_POINT('Ctrl Pts',(43.2140405920445,3.09481465354932,-0.933657143999897));
#77597=CARTESIAN_POINT('Ctrl Pts',(43.2304272438378,3.15268440221548,-0.668634434885807));
#77598=CARTESIAN_POINT('Ctrl Pts',(43.2315998120293,3.15663669289056,-0.649719717576928));
#77599=CARTESIAN_POINT('Ctrl Pts',(43.2333453759244,3.16224066718501,-0.62164152931996));
#77600=CARTESIAN_POINT('Ctrl Pts',(43.2339141849805,3.16402317065066,-0.612504368060808));
#77601=CARTESIAN_POINT('Ctrl Pts',(43.2349271669012,3.16712013233677,-0.596254929518021));
#77602=CARTESIAN_POINT('Ctrl Pts',(43.2353708350004,3.16845028985694,-0.589145680607206));
#77603=CARTESIAN_POINT('Ctrl Pts',(43.2363045118478,3.17119439774743,-0.57420122237302));
#77604=CARTESIAN_POINT('Ctrl Pts',(43.2367946795013,3.17260326522033,-0.566365139971526));
#77605=CARTESIAN_POINT('Ctrl Pts',(43.2380857569203,3.17623072560392,-0.545750988381942));
#77606=CARTESIAN_POINT('Ctrl Pts',(43.2388881921863,3.17840122997594,-0.532964705187144));
#77607=CARTESIAN_POINT('Ctrl Pts',(43.2425035604747,3.18780338988673,-0.475476272433506));
#77608=CARTESIAN_POINT('Ctrl Pts',(43.2453438188681,3.19416927150867,-0.430639601260777));
#77609=CARTESIAN_POINT('Ctrl Pts',(43.2529724429511,3.20857414346446,-0.311138966819544));
#77610=CARTESIAN_POINT('Ctrl Pts',(43.2578106119749,3.21495152298744,-0.236306464384234));
#77611=CARTESIAN_POINT('Ctrl Pts',(43.2828154348829,3.23409932160388,0.145726984973295));
#77612=CARTESIAN_POINT('Ctrl Pts',(43.3041512721203,3.2054753472886,0.453343125383568));
#77613=CARTESIAN_POINT('Ctrl Pts',(43.3288565824333,3.11774957536298,0.818806655019639));
#77614=CARTESIAN_POINT('Ctrl Pts',(43.3332862104494,3.09964661718638,0.884872421551637));
#77615=CARTESIAN_POINT('Ctrl Pts',(43.3382658838135,3.07635558039444,0.960345809590095));
#77616=CARTESIAN_POINT('Ctrl Pts',(43.3389249598881,3.0732114819375,0.970360203999077));
#77617=CARTESIAN_POINT('Ctrl Pts',(43.3399021040513,3.06845728015622,0.985248101136925));
#77618=CARTESIAN_POINT('Ctrl Pts',(43.3402223060454,3.06688440909329,0.990133285507645));
#77619=CARTESIAN_POINT('Ctrl Pts',(43.3407924711809,3.06405680793869,0.998844156965081));
#77620=CARTESIAN_POINT('Ctrl Pts',(43.3410426966749,3.06280657591428,1.00267125786436));
#77621=CARTESIAN_POINT('Ctrl Pts',(43.3415783065097,3.06011044801472,1.01087231132271));
#77622=CARTESIAN_POINT('Ctrl Pts',(43.3418635578245,3.05866235007608,1.01524549381287));
#77623=CARTESIAN_POINT('Ctrl Pts',(43.3426432005881,3.05467112354348,1.02721274629916));
#77624=CARTESIAN_POINT('Ctrl Pts',(43.3431364803648,3.05210903634055,1.03480052796213));
#77625=CARTESIAN_POINT('Ctrl Pts',(43.3457092260153,3.03855482337168,1.07445389231433));
#77626=CARTESIAN_POINT('Ctrl Pts',(43.3477615208502,3.02708509764862,1.10635555288692));
#77627=CARTESIAN_POINT('Ctrl Pts',(43.353655367817,2.99229927086567,1.19851425675956));
#77628=CARTESIAN_POINT('Ctrl Pts',(43.3574325985022,2.96767104873109,1.25826109755009));
#77629=CARTESIAN_POINT('Ctrl Pts',(43.3783652969155,2.81913672199175,1.58992531565403));
#77630=CARTESIAN_POINT('Ctrl Pts',(43.3944258541196,2.65968341526877,1.84431575048016));
#77631=CARTESIAN_POINT('Ctrl Pts',(43.4129284517434,2.45445088831277,2.08858732932336));
#77632=CARTESIAN_POINT('Ctrl Pts',(43.4141054212306,2.44130217861829,2.1039415023352));
#77633=CARTESIAN_POINT('Ctrl Pts',(43.4197820489023,2.37746668483341,2.17708012124055));
#77634=CARTESIAN_POINT('Ctrl Pts',(43.4243485183919,2.32487120431583,2.23315878004042));
#77635=CARTESIAN_POINT('Ctrl Pts',(43.4298892953644,2.25992421593957,2.29762373585778));
#77636=CARTESIAN_POINT('Ctrl Pts',(43.4307796305721,2.24945381316668,2.30787560860098));
#77637=CARTESIAN_POINT('Ctrl Pts',(43.432235130183,2.23228381667067,2.3244593978631));
#77638=CARTESIAN_POINT('Ctrl Pts',(43.4327983989897,2.22562625427951,2.33083467967221));
#77639=CARTESIAN_POINT('Ctrl Pts',(43.4338051662157,2.21370439969849,2.34215339858362));
#77640=CARTESIAN_POINT('Ctrl Pts',(43.4342481823049,2.2084506497448,2.34710788802611));
#77641=CARTESIAN_POINT('Ctrl Pts',(43.4351842559037,2.19733384195525,2.35752109691249));
#77642=CARTESIAN_POINT('Ctrl Pts',(43.4356774861151,2.19146700204927,2.36297569019799));
#77643=CARTESIAN_POINT('Ctrl Pts',(43.4369852917782,2.17588708490755,2.37735292151821));
#77644=CARTESIAN_POINT('Ctrl Pts',(43.4378014651827,2.16613954165151,2.38623783338958));
#77645=CARTESIAN_POINT('Ctrl Pts',(43.4415690716463,2.12103424815053,2.42684731614712));
#77646=CARTESIAN_POINT('Ctrl Pts',(43.4445507319769,2.08503382315228,2.45784615978638));
#77647=CARTESIAN_POINT('Ctrl Pts',(43.4526513374431,1.98647656436327,2.5389868563962));
#77648=CARTESIAN_POINT('Ctrl Pts',(43.457827997611,1.92271544037624,2.58760641990464));
#77649=CARTESIAN_POINT('Ctrl Pts',(43.4648790302444,1.834809030872,2.64959333917145));
#77650=CARTESIAN_POINT('Ctrl Pts',(43.4666839122602,1.81221492822833,2.66509751486038));
#77651=CARTESIAN_POINT('Ctrl Pts',(43.4684957936438,1.78943612473158,2.68030519120596));
#77652=CARTESIAN_POINT('Origin',(-1.72497344927317,0.,0.));
#77653=CARTESIAN_POINT('',(44.9670777766272,1.78943621037802,2.68030513402634));
#77654=CARTESIAN_POINT('',(44.7203641905528,1.78943621037803,2.68030513402633));
#77655=CARTESIAN_POINT('',(-1.72497344927317,1.78943621037804,2.68030513402633));
#77656=CARTESIAN_POINT('',(44.1465734493244,-3.22274921673691,0.00224689155001823));
#77657=CARTESIAN_POINT('Ctrl Pts',(44.1465734493244,-3.22274921673691,0.0022468915499753));
#77658=CARTESIAN_POINT('Ctrl Pts',(44.1526529568098,-3.22281760930423,-0.095849562091568));
#77659=CARTESIAN_POINT('Ctrl Pts',(44.1587324642952,-3.21840290922743,-0.194120808494868));
#77660=CARTESIAN_POINT('Ctrl Pts',(44.1648119717806,-3.20948372755331,-0.292116013033343));
#77661=CARTESIAN_POINT('Ctrl Pts',(44.1708844563096,-3.20057484918487,-0.389998014972797));
#77662=CARTESIAN_POINT('Ctrl Pts',(44.1769569408386,-3.18717186664683,-0.487604165813532));
#77663=CARTESIAN_POINT('Ctrl Pts',(44.1830294253676,-3.16930542664221,-0.584483254812545));
#77664=CARTESIAN_POINT('Ctrl Pts',(44.1890968615674,-3.15145383981163,-0.681281803873583));
#77665=CARTESIAN_POINT('Ctrl Pts',(44.1951642977673,-3.12914624990319,-0.777354053550099));
#77666=CARTESIAN_POINT('Ctrl Pts',(44.2012317339671,-3.10246504238519,-0.872254677991387));
#77667=CARTESIAN_POINT('Ctrl Pts',(44.2072965624384,-3.07579530220618,-0.967114515012184));
#77668=CARTESIAN_POINT('Ctrl Pts',(44.2133613909097,-3.0447557976732,-1.06080329618506));
#77669=CARTESIAN_POINT('Ctrl Pts',(44.2194262193809,-3.00947962439654,-1.15288765837877));
#77670=CARTESIAN_POINT('Ctrl Pts',(44.2254901704919,-2.97420855430017,-1.24495869931171));
#77671=CARTESIAN_POINT('Ctrl Pts',(44.2315541216029,-2.93470219353686,-1.33542536435833));
#77672=CARTESIAN_POINT('Ctrl Pts',(44.2376180727139,-2.89114254196026,-1.42387231329482));
#77673=CARTESIAN_POINT('Ctrl Pts',(44.2436828756468,-2.84757677142465,-1.51233168664784));
#77674=CARTESIAN_POINT('Ctrl Pts',(44.2497476785798,-2.79995677867317,-1.59877037946745));
#77675=CARTESIAN_POINT('Ctrl Pts',(44.2558124815128,-2.74851092068858,-1.68279686277209));
#77676=CARTESIAN_POINT('Ctrl Pts',(44.2618835398218,-2.69701200027315,-1.76691001290734));
#77677=CARTESIAN_POINT('Ctrl Pts',(44.2679545981307,-2.64167957332646,-1.84860560559265));
#77678=CARTESIAN_POINT('Ctrl Pts',(44.2740256564397,-2.58278561195192,-1.92752069903131));
#77679=CARTESIAN_POINT('Ctrl Pts',(44.2801002125747,-2.52385771896009,-2.0064812592154));
#77680=CARTESIAN_POINT('Ctrl Pts',(44.2861747687096,-2.46136449333861,-2.08265778770013));
#77681=CARTESIAN_POINT('Ctrl Pts',(44.2922493248445,-2.39561708433311,-2.15572176955918));
#77682=CARTESIAN_POINT('Ctrl Pts',(44.29833346357,-2.3297659590251,-2.22890100958823));
#77683=CARTESIAN_POINT('Ctrl Pts',(44.3044176022955,-2.26065071977042,-2.29895758658903));
#77684=CARTESIAN_POINT('Ctrl Pts',(44.310501741021,-2.18861791905681,-2.36560122735922));
#77685=CARTESIAN_POINT('Ctrl Pts',(44.3136076711837,-2.1518454425353,-2.39962255779829));
#77686=CARTESIAN_POINT('Ctrl Pts',(44.3167136013464,-2.11431314330431,-2.43275512131571));
#77687=CARTESIAN_POINT('Ctrl Pts',(44.319819531509,-2.0760700651483,-2.46496463404552));
#77688=CARTESIAN_POINT('Ctrl Pts',(44.3259917795973,-2.00007165125118,-2.52897286763693));
#77689=CARTESIAN_POINT('Ctrl Pts',(44.3321640276855,-1.92097649915154,-2.58957575854878));
#77690=CARTESIAN_POINT('Ctrl Pts',(44.3383362757738,-1.83912266263081,-2.64645902940094));
#77691=CARTESIAN_POINT('Ctrl Pts',(44.3445001644218,-1.7573796855965,-2.70326525987893));
#77692=CARTESIAN_POINT('Ctrl Pts',(44.3506640530699,-1.67288580390756,-2.75636163758103));
#77693=CARTESIAN_POINT('Ctrl Pts',(44.3568279417179,-1.58601304345421,-2.80547325570805));
#77694=CARTESIAN_POINT('Ctrl Pts',(44.3629853033718,-1.49923227330649,-2.85453286912452));
#77695=CARTESIAN_POINT('Ctrl Pts',(44.3691426650256,-1.41007800848197,-2.89961589913159));
#77696=CARTESIAN_POINT('Ctrl Pts',(44.3753000266795,-1.31895143260922,-2.94049055106764));
#77697=CARTESIAN_POINT('Ctrl Pts',(44.381452890821,-1.22789141818314,-2.98133534699364));
#77698=CARTESIAN_POINT('Ctrl Pts',(44.3876057549626,-1.1348623520684,-3.01797769908814));
#77699=CARTESIAN_POINT('Ctrl Pts',(44.3937586191041,-1.04028939166791,-3.05023204757986));
#77700=CARTESIAN_POINT('Ctrl Pts',(44.3999091522358,-0.945752260191214,
-3.08247417652606));
#77701=CARTESIAN_POINT('Ctrl Pts',(44.4060596853675,-0.849672807295397,
-3.11033146497705));
#77702=CARTESIAN_POINT('Ctrl Pts',(44.4122102184992,-0.752494680015537,
-3.1336670721454));
#77703=CARTESIAN_POINT('Ctrl Pts',(44.4183600667095,-0.655327374460668,
-3.15700008066804));
#77704=CARTESIAN_POINT('Ctrl Pts',(44.4245099149198,-0.557062060136261,
-3.1758123075808));
#77705=CARTESIAN_POINT('Ctrl Pts',(44.4306597631301,-0.45815502131104,-3.19001748254574));
#77706=CARTESIAN_POINT('Ctrl Pts',(44.4368105715043,-0.359232540321682,
-3.2042248753371));
#77707=CARTESIAN_POINT('Ctrl Pts',(44.4429613798785,-0.259668565829818,
-3.21382372572693));
#77708=CARTESIAN_POINT('Ctrl Pts',(44.4491121882527,-0.159925985765453,
-3.21877946457612));
#77709=CARTESIAN_POINT('Ctrl Pts',(44.4552695746139,-0.0600767359176954,
-3.22374050334426));
#77710=CARTESIAN_POINT('Ctrl Pts',(44.4614269609751,0.0399510662436259,
-3.22404849322508));
#77711=CARTESIAN_POINT('Ctrl Pts',(44.4675843473363,0.139693157421742,-3.21972101031589));
#77712=CARTESIAN_POINT('Ctrl Pts',(44.4737451700682,0.239490913582315,-3.21539111228528));
#77713=CARTESIAN_POINT('Ctrl Pts',(44.4799059928002,0.339002208577645,-3.20642062847573));
#77714=CARTESIAN_POINT('Ctrl Pts',(44.4860668155321,0.437768627146858,-3.19287898166936));
#77715=CARTESIAN_POINT('Ctrl Pts',(44.4922379384438,0.536700171691406,-3.17931469480305));
#77716=CARTESIAN_POINT('Ctrl Pts',(44.4984090613555,0.634883924931221,-3.16116405837411));
#77717=CARTESIAN_POINT('Ctrl Pts',(44.5045801842671,0.731872234600702,-3.13854752946655));
#77718=CARTESIAN_POINT('Ctrl Pts',(44.5092757062609,0.805669296774438,-3.12133892571179));
#77719=CARTESIAN_POINT('Ctrl Pts',(44.5139712282547,0.878774483578418,-3.10154586109726));
#77720=CARTESIAN_POINT('Ctrl Pts',(44.5186667502485,0.950997881658948,-3.07924026207443));
#77721=CARTESIAN_POINT('Ctrl Pts',(44.5248389983783,1.04593529954678,-3.04991962593781));
#77722=CARTESIAN_POINT('Ctrl Pts',(44.531011246508,1.13968255083815,-3.01615268230944));
#77723=CARTESIAN_POINT('Ctrl Pts',(44.5371834946378,1.23179247345417,-2.97805387205162));
#77724=CARTESIAN_POINT('Ctrl Pts',(44.5433473833275,1.32377764616418,-2.94000666126174));
#77725=CARTESIAN_POINT('Ctrl Pts',(44.5495112720172,1.41412949992564,-2.89763940952146));
#77726=CARTESIAN_POINT('Ctrl Pts',(44.5556751607069,1.5024156224767,-2.85111642340995));
#77727=CARTESIAN_POINT('Ctrl Pts',(44.5618325224026,1.59060825810347,-2.80464270088319));
#77728=CARTESIAN_POINT('Ctrl Pts',(44.5679898840983,1.67673912915199,-2.75402219406405));
#77729=CARTESIAN_POINT('Ctrl Pts',(44.574147245794,1.76039632378757,-2.69946704845516));
#77730=CARTESIAN_POINT('Ctrl Pts',(44.5803001099774,1.84399241282648,-2.6449517514778));
#77731=CARTESIAN_POINT('Ctrl Pts',(44.5864529741608,1.92511805501856,-2.58650776621703));
#77732=CARTESIAN_POINT('Ctrl Pts',(44.5926058383442,2.00338726886607,-2.52439240480662));
#77733=CARTESIAN_POINT('Ctrl Pts',(44.5987563715178,2.08162683045724,-2.46230057577285));
#77734=CARTESIAN_POINT('Ctrl Pts',(44.6049069046914,2.15701177407305,-2.39654040402348));
#77735=CARTESIAN_POINT('Ctrl Pts',(44.611057437865,2.22918710352607,-2.32741109818894));
#77736=CARTESIAN_POINT('Ctrl Pts',(44.6172072861172,2.30135439555739,-2.25828949057188));
#77737=CARTESIAN_POINT('Ctrl Pts',(44.6233571343693,2.37031247033412,-2.18579979525279));
#77738=CARTESIAN_POINT('Ctrl Pts',(44.6295069826215,2.43574203890022,-2.11027919537539));
#77739=CARTESIAN_POINT('Ctrl Pts',(44.6356577910375,2.50118182285714,-2.03474680461415));
#77740=CARTESIAN_POINT('Ctrl Pts',(44.6418085994534,2.5630917219174,-1.95618289770892));
#77741=CARTESIAN_POINT('Ctrl Pts',(44.6479594078694,2.62119236796707,-1.87495816822967));
#77742=CARTESIAN_POINT('Ctrl Pts',(44.654116794272,2.67935514979558,-1.79364657290349));
#77743=CARTESIAN_POINT('Ctrl Pts',(44.6602741806746,2.73370029043168,-1.70966882658044));
#77744=CARTESIAN_POINT('Ctrl Pts',(44.6664315670772,2.78399154312429,-1.62342497526448));
#77745=CARTESIAN_POINT('Ctrl Pts',(44.6725923898503,2.83431086281969,-1.53713299219027));
#77746=CARTESIAN_POINT('Ctrl Pts',(44.6787532126235,2.8805715878488,-1.4485727705376));
#77747=CARTESIAN_POINT('Ctrl Pts',(44.6849140353966,2.92258424744677,-1.35816747092397));
#77748=CARTESIAN_POINT('Ctrl Pts',(44.6910851583489,2.96466714732472,-1.26761102416523));
#77749=CARTESIAN_POINT('Ctrl Pts',(44.6972562813011,3.00248763059313,-1.17520373993617));
#77750=CARTESIAN_POINT('Ctrl Pts',(44.7034274042533,3.03590497665852,-1.08138731969633));
#77751=CARTESIAN_POINT('Ctrl Pts',(44.7081229258316,3.06133177025094,-1.01000371106538));
#77752=CARTESIAN_POINT('Ctrl Pts',(44.7128184474099,3.08421038868229,-0.937804669863619));
#77753=CARTESIAN_POINT('Ctrl Pts',(44.7175139689882,3.10449864903982,-0.864988844211257));
#77754=CARTESIAN_POINT('Ctrl Pts',(44.7236862170209,3.13116750211432,-0.769272675274183));
#77755=CARTESIAN_POINT('Ctrl Pts',(44.7298584650537,3.15345254656793,-0.672153521110634));
#77756=CARTESIAN_POINT('Ctrl Pts',(44.7360307130864,3.17120826595635,-0.574069417779857));
#77757=CARTESIAN_POINT('Ctrl Pts',(44.7421946016792,3.18893993772539,-0.476118155542837));
#77758=CARTESIAN_POINT('Ctrl Pts',(44.7483584902719,3.20215440039602,-0.37720496538648));
#77759=CARTESIAN_POINT('Ctrl Pts',(44.7545223788646,3.21075606038626,-0.277782438597017));
#77760=CARTESIAN_POINT('Ctrl Pts',(44.7606797404634,3.21934861200581,-0.178465191164078));
#77761=CARTESIAN_POINT('Ctrl Pts',(44.7668371020623,3.22333803462936,-0.0786401097310378));
#77762=CARTESIAN_POINT('Ctrl Pts',(44.7729944636611,3.22268006199457,0.0212315925614776));
#77763=CARTESIAN_POINT('Ctrl Pts',(44.7791473277481,3.22202256996167,0.121030345726199));
#77764=CARTESIAN_POINT('Ctrl Pts',(44.7853001918352,3.21672443454802,0.220875218990439));
#77765=CARTESIAN_POINT('Ctrl Pts',(44.7914530559222,3.20679340486268,0.320302389983657));
#77766=CARTESIAN_POINT('Ctrl Pts',(44.7976035889998,3.19686613754291,0.419691893043447));
#77767=CARTESIAN_POINT('Ctrl Pts',(44.8037541220774,3.18230950658779,0.518663576521987));
#77768=CARTESIAN_POINT('Ctrl Pts',(44.809904655155,3.16318325888739,0.616757029302923));
#77769=CARTESIAN_POINT('Ctrl Pts',(44.8160545033117,3.14405914107842,0.714839558435483));
#77770=CARTESIAN_POINT('Ctrl Pts',(44.8222043514683,3.12036650136265,0.812043624962921));
#77771=CARTESIAN_POINT('Ctrl Pts',(44.828354199625,3.0922163383949,0.907918321801928));
#77772=CARTESIAN_POINT('Ctrl Pts',(44.834505007946,3.06406178039452,1.0038079873792));
#77773=CARTESIAN_POINT('Ctrl Pts',(44.840655816267,3.03144843920041,1.09836745419547));
#77774=CARTESIAN_POINT('Ctrl Pts',(44.846806624588,2.99453708834475,1.19116127750516));
#77775=CARTESIAN_POINT('Ctrl Pts',(44.8529640108972,2.95758626260795,1.28405433926215));
#77776=CARTESIAN_POINT('Ctrl Pts',(44.8591213972063,2.91632840931499,1.37517758243127));
#77777=CARTESIAN_POINT('Ctrl Pts',(44.8652787835154,2.87097230968958,1.46411596518024));
#77778=CARTESIAN_POINT('Ctrl Pts',(44.8714396061959,2.82559089731133,1.55310398348692));
#77779=CARTESIAN_POINT('Ctrl Pts',(44.8776004288763,2.77610689883539,1.63990433568739));
#77780=CARTESIAN_POINT('Ctrl Pts',(44.8837612515567,2.72277383195886,1.72412883001823));
#77781=CARTESIAN_POINT('Ctrl Pts',(44.8899323744182,2.66935159837899,1.80849413793698));
#77782=CARTESIAN_POINT('Ctrl Pts',(44.8961034972797,2.6120676916164,1.89027462987103));
#77783=CARTESIAN_POINT('Ctrl Pts',(44.9022746201413,2.55121758580642,1.96911309791288));
#77784=CARTESIAN_POINT('Ctrl Pts',(44.9069701426701,2.50491757701946,2.02910020417178));
#77785=CARTESIAN_POINT('Ctrl Pts',(44.911665665199,2.45655379384332,2.087384674831));
#77786=CARTESIAN_POINT('Ctrl Pts',(44.9163611877278,2.40627053220781,2.14382361408964));
#77787=CARTESIAN_POINT('Ctrl Pts',(44.9225333531327,2.34017424452021,2.21801141028038));
#77788=CARTESIAN_POINT('Ctrl Pts',(44.9287055185376,2.27052747811876,2.28927019455793));
#77789=CARTESIAN_POINT('Ctrl Pts',(44.9348776839424,2.19762001868556,2.35724072083707));
#77790=CARTESIAN_POINT('Ctrl Pts',(44.9410406362659,2.12482138691904,2.42510978872175));
#77791=CARTESIAN_POINT('Ctrl Pts',(44.9472035885894,2.04877205618219,2.4897000661279));
#77792=CARTESIAN_POINT('Ctrl Pts',(44.9533665409128,1.96980090855367,2.55068656309652));
#77793=CARTESIAN_POINT('Ctrl Pts',(44.9579369528176,1.91123633522698,2.59591381736485));
#77794=CARTESIAN_POINT('Ctrl Pts',(44.9625073647224,1.85106573411159,2.63915978083607));
#77795=CARTESIAN_POINT('Ctrl Pts',(44.9670777766272,1.78943621037802,2.68030513402634));
#77796=CARTESIAN_POINT('Ctrl Pts',(43.716926315029,1.78943621037803,2.68030513402633));
#77797=CARTESIAN_POINT('Ctrl Pts',(43.7190435017826,1.76105704067242,2.6992517506809));
#77798=CARTESIAN_POINT('Ctrl Pts',(43.7211606885363,1.73239290766513,2.71773692959355));
#77799=CARTESIAN_POINT('Ctrl Pts',(43.7232778752899,1.70346037892409,2.73575223657695));
#77800=CARTESIAN_POINT('Ctrl Pts',(43.7294501233816,1.61911319273265,2.78827237631396));
#77801=CARTESIAN_POINT('Ctrl Pts',(43.7356223714733,1.53218636313262,2.83698048428247));
#77802=CARTESIAN_POINT('Ctrl Pts',(43.741794619565,1.44305929443266,2.88161368598421));
#77803=CARTESIAN_POINT('Ctrl Pts',(43.7479585082166,1.35405293578609,2.92618643830464));
#77804=CARTESIAN_POINT('Ctrl Pts',(43.7541223968682,1.26285264592198,2.96669506096335));
#77805=CARTESIAN_POINT('Ctrl Pts',(43.7602862855197,1.16986584160716,3.00292049097887));
#77806=CARTESIAN_POINT('Ctrl Pts',(43.7664436471772,1.07697750180988,3.0391075615786));
#77807=CARTESIAN_POINT('Ctrl Pts',(43.7726010088347,0.98230681106408,3.07102029974576));
#77808=CARTESIAN_POINT('Ctrl Pts',(43.7787583704922,0.886283900001522,3.09848647102066));
#77809=CARTESIAN_POINT('Ctrl Pts',(43.7849112346374,0.790331126806957,3.12593258022211));
#77810=CARTESIAN_POINT('Ctrl Pts',(43.7910640987826,0.693028513380123,3.14893846081337));
#77811=CARTESIAN_POINT('Ctrl Pts',(43.7972169629278,0.594823328022513,3.16738105868874));
#77812=CARTESIAN_POINT('Ctrl Pts',(43.8033674960633,0.496655347654633,3.18581666959432));
#77813=CARTESIAN_POINT('Ctrl Pts',(43.8095180291987,0.397585901225343,3.19969235281176));
#77814=CARTESIAN_POINT('Ctrl Pts',(43.8156685623342,0.298073612445653,3.2089359114921));
#77815=CARTESIAN_POINT('Ctrl Pts',(43.8218184105483,0.198572405321534,3.21817844081279));
#77816=CARTESIAN_POINT('Ctrl Pts',(43.8279682587624,0.0986288864057926,
3.22278983096988));
#77817=CARTESIAN_POINT('Ctrl Pts',(43.8341181069765,-0.00129302174893185,
3.2227497406089));
#77818=CARTESIAN_POINT('Ctrl Pts',(43.8402689153546,-0.101230530518191,
3.2227096439887));
#77819=CARTESIAN_POINT('Ctrl Pts',(43.8464197237326,-0.201145987408588,
3.21801662455096));
#77820=CARTESIAN_POINT('Ctrl Pts',(43.8525705321106,-0.300576304171876,
3.20870245549044));
#77821=CARTESIAN_POINT('Ctrl Pts',(43.8587279184757,-0.400112956768798,
3.19937832538419));
#77822=CARTESIAN_POINT('Ctrl Pts',(43.8648853048408,-0.499162999856632,
3.1854232173993));
#77823=CARTESIAN_POINT('Ctrl Pts',(43.8710426912059,-0.597269417687098,
3.16692071343691));
#77824=CARTESIAN_POINT('Ctrl Pts',(43.8772035139418,-0.69543058764883,3.14840788342706));
#77825=CARTESIAN_POINT('Ctrl Pts',(43.8833643366776,-0.792646660926259,
3.12534270361975));
#77826=CARTESIAN_POINT('Ctrl Pts',(43.8895251594135,-0.888473801333701,
3.09785923935282));
#77827=CARTESIAN_POINT('Ctrl Pts',(43.8956962823291,-0.984461153585005,
3.07032982592715));
#77828=CARTESIAN_POINT('Ctrl Pts',(43.9018674052447,-1.07905452286466,3.03836751213368));
#77829=CARTESIAN_POINT('Ctrl Pts',(43.9080385281603,-1.17182800149522,3.00215534198544));
#77830=CARTESIAN_POINT('Ctrl Pts',(43.9127340501167,-1.24241805647297,2.97460200325804));
#77831=CARTESIAN_POINT('Ctrl Pts',(43.9174295720732,-1.31195486234312,2.94458923460663));
#77832=CARTESIAN_POINT('Ctrl Pts',(43.9221250940296,-1.38026069932417,2.91221530186234));
#77833=CARTESIAN_POINT('Ctrl Pts',(43.9282973421279,-1.4700484963608,2.86965987422987));
#77834=CARTESIAN_POINT('Ctrl Pts',(43.9344695902262,-1.55802441789106,2.82287322294944));
#77835=CARTESIAN_POINT('Ctrl Pts',(43.9406418383245,-1.64376218374863,2.77203236737559));
#77836=CARTESIAN_POINT('Ctrl Pts',(43.9468057269826,-1.72938382988641,2.721260368575));
#77837=CARTESIAN_POINT('Ctrl Pts',(43.9529696156408,-1.81277297499114,2.66644529874857));
#77838=CARTESIAN_POINT('Ctrl Pts',(43.9591335042989,-1.89352504691214,2.60781143091605));
#77839=CARTESIAN_POINT('Ctrl Pts',(43.965290865963,-1.97419160977797,2.54923965098443));
#77840=CARTESIAN_POINT('Ctrl Pts',(43.971448227627,-2.05222630149996,2.48685736622848));
#77841=CARTESIAN_POINT('Ctrl Pts',(43.9776055892911,-2.1272516608781,2.42093327743483));
#77842=CARTESIAN_POINT('Ctrl Pts',(43.9837584534429,-2.20222221959785,2.35505734147243));
#77843=CARTESIAN_POINT('Ctrl Pts',(43.9899113175947,-2.27418749085708,2.28564503079462));
#77844=CARTESIAN_POINT('Ctrl Pts',(43.9960641817466,-2.34280211789449,2.2130060548695));
#77845=CARTESIAN_POINT('Ctrl Pts',(44.0022147148886,-2.41139075031172,2.14039459818732));
#77846=CARTESIAN_POINT('Ctrl Pts',(44.0083652480306,-2.47663096283152,2.06455922062285));
#77847=CARTESIAN_POINT('Ctrl Pts',(44.0145157811727,-2.5382140402841,1.98584668295533));
#77848=CARTESIAN_POINT('Ctrl Pts',(44.0206656293934,-2.59979025986543,1.90714291069011));
#77849=CARTESIAN_POINT('Ctrl Pts',(44.0268154776141,-2.65770988640599,1.82556295743417));
#77850=CARTESIAN_POINT('Ctrl Pts',(44.0329653258347,-2.71170496090233,1.74148608019637));
#77851=CARTESIAN_POINT('Ctrl Pts',(44.0391161342193,-2.76570846554522,1.65739607619832));
#77852=CARTESIAN_POINT('Ctrl Pts',(44.0452669426039,-2.81578596635182,1.57080873942461));
#77853=CARTESIAN_POINT('Ctrl Pts',(44.0514177509885,-2.86171379465896,1.48213080393015));
#77854=CARTESIAN_POINT('Ctrl Pts',(44.0575751373601,-2.90769074051907,1.39335803174616));
#77855=CARTESIAN_POINT('Ctrl Pts',(44.0637325237317,-2.94950895175349,1.30249058266012));
#77856=CARTESIAN_POINT('Ctrl Pts',(44.0698899101033,-2.98699162510762,1.20995809598388));
#77857=CARTESIAN_POINT('Ctrl Pts',(44.0760507328456,-3.02449521713638,1.11737396792755));
#77858=CARTESIAN_POINT('Ctrl Pts',(44.0822115555879,-3.05765830847178,1.02312336147732));
#77859=CARTESIAN_POINT('Ctrl Pts',(44.0883723783302,-3.08635368930061,0.927652126090644));
#77860=CARTESIAN_POINT('Ctrl Pts',(44.0945435012522,-3.11509704547126,0.83202127389392));
#77861=CARTESIAN_POINT('Ctrl Pts',(44.1007146241741,-3.13935766546156,0.735166137980126));
#77862=CARTESIAN_POINT('Ctrl Pts',(44.1068857470961,-3.1590592348845,0.637543969456977));
#77863=CARTESIAN_POINT('Ctrl Pts',(44.1115812689871,-3.17404988596756,0.563264614605248));
#77864=CARTESIAN_POINT('Ctrl Pts',(44.1162767908782,-3.18640214017127,0.488541423362433));
#77865=CARTESIAN_POINT('Ctrl Pts',(44.1209723127692,-3.19610256468347,0.413577028525253));
#77866=CARTESIAN_POINT('Ctrl Pts',(44.1295060249372,-3.21373226221536,0.277335608886467));
#77867=CARTESIAN_POINT('Ctrl Pts',(44.1380397371051,-3.22265321509459,0.139943391985787));
#77868=CARTESIAN_POINT('Ctrl Pts',(44.146573449273,-3.22274921673633,0.00224689238003723));
#77869=CARTESIAN_POINT('',(43.9000265507268,-3.22274886258475,-0.00270762048436531));
#77870=CARTESIAN_POINT('Ctrl Pts',(43.4684957936438,1.78943612473158,2.68030519120596));
#77871=CARTESIAN_POINT('Ctrl Pts',(43.4877157978139,1.54780402775395,2.84162458298458));
#77872=CARTESIAN_POINT('Ctrl Pts',(43.5078864493151,1.28539961238176,2.96957769162189));
#77873=CARTESIAN_POINT('Ctrl Pts',(43.5301679120223,0.960501825768391,3.07671790198192));
#77874=CARTESIAN_POINT('Ctrl Pts',(43.5334674418493,0.911331458664287,3.0916391281324));
#77875=CARTESIAN_POINT('Ctrl Pts',(43.5372517817597,0.853432532566815,3.10770756046767));
#77876=CARTESIAN_POINT('Ctrl Pts',(43.5377982946381,0.845033415565883,3.11000191313858));
#77877=CARTESIAN_POINT('Ctrl Pts',(43.5386704724684,0.831566970626343,3.11362190513594));
#77878=CARTESIAN_POINT('Ctrl Pts',(43.538997365623,0.826505601174957,3.11496925938776));
#77879=CARTESIAN_POINT('Ctrl Pts',(43.5395756779191,0.8175259030862,3.11733625916046));
#77880=CARTESIAN_POINT('Ctrl Pts',(43.5398273840808,0.81360891454056,3.11836086586996));
#77881=CARTESIAN_POINT('Ctrl Pts',(43.5403124180941,0.806044098609917,3.12032444808976));
#77882=CARTESIAN_POINT('Ctrl Pts',(43.5405458039166,0.802396575251329,3.12126440511255));
#77883=CARTESIAN_POINT('Ctrl Pts',(43.5411886306378,0.792329537570116,3.12383984079869));
#77884=CARTESIAN_POINT('Ctrl Pts',(43.5415972985089,0.785906570775604,3.12546193560499));
#77885=CARTESIAN_POINT('Ctrl Pts',(43.5432213124402,0.760292952470528,3.13184660357921));
#77886=CARTESIAN_POINT('Ctrl Pts',(43.5444278781981,0.741063160271112,3.13645244820113));
#77887=CARTESIAN_POINT('Ctrl Pts',(43.5529605414526,0.603761799507086,3.16800505074666));
#77888=CARTESIAN_POINT('Ctrl Pts',(43.5599549918109,0.484282687136266,3.18845751385116));
#77889=CARTESIAN_POINT('Ctrl Pts',(43.5763624822714,0.196750469310036,3.22113560177844));
#77890=CARTESIAN_POINT('Ctrl Pts',(43.5856419666568,0.0283441807176981,
3.22701479711338));
#77891=CARTESIAN_POINT('Ctrl Pts',(43.6053741388683,-0.321396223821876,
3.2118340535394));
#77892=CARTESIAN_POINT('Ctrl Pts',(43.6158326678356,-0.502019122454991,
3.18859475684349));
#77893=CARTESIAN_POINT('Ctrl Pts',(43.6278876224103,-0.697163904403001,
3.14648995652153));
#77894=CARTESIAN_POINT('Ctrl Pts',(43.6289706431008,-0.714590646619772,
3.14257804103835));
#77895=CARTESIAN_POINT('Ctrl Pts',(43.6306153674344,-0.740891888532359,
3.13644391695774));
#77896=CARTESIAN_POINT('Ctrl Pts',(43.6311736411122,-0.749791112451979,
3.13432840010267));
#77897=CARTESIAN_POINT('Ctrl Pts',(43.6321466125339,-0.765251038963044,
3.13058366857307));
#77898=CARTESIAN_POINT('Ctrl Pts',(43.6325607537696,-0.771815876804614,
3.12897163773967));
#77899=CARTESIAN_POINT('Ctrl Pts',(43.6334262629721,-0.785502792908852,
3.12556504798225));
#77900=CARTESIAN_POINT('Ctrl Pts',(43.63387774897,-0.792623898416815,3.12376677443606));
#77901=CARTESIAN_POINT('Ctrl Pts',(43.6349478323443,-0.809457586498474,
3.11945454083183));
#77902=CARTESIAN_POINT('Ctrl Pts',(43.635567108389,-0.819164657128837,3.11691954941381));
#77903=CARTESIAN_POINT('Ctrl Pts',(43.637624854785,-0.851302745727447,3.1083662216641));
#77904=CARTESIAN_POINT('Ctrl Pts',(43.6390697091569,-0.873680134157912,
3.10215085231447));
#77905=CARTESIAN_POINT('Ctrl Pts',(43.6533941161485,-1.0936397264507,3.03848786729265));
#77906=CARTESIAN_POINT('Ctrl Pts',(43.6668993394536,-1.28532129224465,2.96249510637663));
#77907=CARTESIAN_POINT('Ctrl Pts',(43.6912165112321,-1.60716973328735,2.79775218404842));
#77908=CARTESIAN_POINT('Ctrl Pts',(43.7018439395147,-1.74057921387812,2.71676195556411));
#77909=CARTESIAN_POINT('Ctrl Pts',(43.7148563692884,-1.8990374942846,2.60408559597139));
#77910=CARTESIAN_POINT('Ctrl Pts',(43.7174238771067,-1.93006783092945,2.58117096241183));
#77911=CARTESIAN_POINT('Ctrl Pts',(43.7251496374181,-2.02291568918314,2.50999582096536));
#77912=CARTESIAN_POINT('Ctrl Pts',(43.7302423114258,-2.08339523886887,2.46002713359831));
#77913=CARTESIAN_POINT('Ctrl Pts',(43.7358746360664,-2.15011481775636,2.40067529942196));
#77914=CARTESIAN_POINT('Ctrl Pts',(43.7365571251502,-2.15819664580325,2.39341239003989));
#77915=CARTESIAN_POINT('Ctrl Pts',(43.7375621030969,-2.17009553626384,2.38260991746821));
#77916=CARTESIAN_POINT('Ctrl Pts',(43.7378869049005,-2.17394090111141,2.37910185042888));
#77917=CARTESIAN_POINT('Ctrl Pts',(43.7384621502992,-2.18075113466646,2.37285868138165));
#77918=CARTESIAN_POINT('Ctrl Pts',(43.7387128747457,-2.18371937848494,2.37012731933458));
#77919=CARTESIAN_POINT('Ctrl Pts',(43.7391974865555,-2.18945653070508,2.36482809582943));
#77920=CARTESIAN_POINT('Ctrl Pts',(43.7394314265268,-2.19222603677146,2.36226095652493));
#77921=CARTESIAN_POINT('Ctrl Pts',(43.739943215619,-2.19828460475079,2.35662525504995));
#77922=CARTESIAN_POINT('Ctrl Pts',(43.7402209091242,-2.20157177392333,2.35355465648566));
#77923=CARTESIAN_POINT('Ctrl Pts',(43.7413444792351,-2.21487059820334,2.34107976552734));
#77924=CARTESIAN_POINT('Ctrl Pts',(43.7421860612179,-2.22482869539563,2.33161822071004));
#77925=CARTESIAN_POINT('Ctrl Pts',(43.7495215986104,-2.31156148875756,2.24814867953351));
#77926=CARTESIAN_POINT('Ctrl Pts',(43.7557454985783,-2.38468822838401,2.17042763984898));
#77927=CARTESIAN_POINT('Ctrl Pts',(43.7668528465909,-2.51065228014839,2.02247983370302));
#77928=CARTESIAN_POINT('Ctrl Pts',(43.7717727701243,-2.56472727665808,1.95345198314072));
#77929=CARTESIAN_POINT('Ctrl Pts',(43.782435155217,-2.67604197552961,1.79875288049955));
#77930=CARTESIAN_POINT('Ctrl Pts',(43.7881660857676,-2.7321235398809,1.71237063152408));
#77931=CARTESIAN_POINT('Ctrl Pts',(43.8042176906825,-2.87557815923005,1.46636800151938));
#77932=CARTESIAN_POINT('Ctrl Pts',(43.8146779103869,-2.95370962208854,1.3018335267992));
#77933=CARTESIAN_POINT('Ctrl Pts',(43.8267347640332,-3.02381862247912,1.11488004083615));
#77934=CARTESIAN_POINT('Ctrl Pts',(43.8278178032251,-3.0299508139322,1.09810500974019));
#77935=CARTESIAN_POINT('Ctrl Pts',(43.8294625509683,-3.03901221997626,1.07266302397029));
#77936=CARTESIAN_POINT('Ctrl Pts',(43.8300208294152,-3.04204455743757,1.06403296190034));
#77937=CARTESIAN_POINT('Ctrl Pts',(43.8309938068158,-3.04725383077033,1.04900302654227));
#77938=CARTESIAN_POINT('Ctrl Pts',(43.8314079492444,-3.04944745833011,1.04260896630515));
#77939=CARTESIAN_POINT('Ctrl Pts',(43.8322734586615,-3.05398246321459,1.02925342893996));
#77940=CARTESIAN_POINT('Ctrl Pts',(43.8327249436739,-3.05632019000713,1.0222907616417));
#77941=CARTESIAN_POINT('Ctrl Pts',(43.8337950205934,-3.06179481757895,1.0057985434146));
#77942=CARTESIAN_POINT('Ctrl Pts',(43.8344142911464,-3.06491104690823,0.996262257530085));
#77943=CARTESIAN_POINT('Ctrl Pts',(43.8364720007518,-3.07509313055501,0.964603103829358));
#77944=CARTESIAN_POINT('Ctrl Pts',(43.8379168235111,-3.08196425050239,0.942418814861096));
#77945=CARTESIAN_POINT('Ctrl Pts',(43.8522329707281,-3.1473072543721,0.723090129842494));
#77946=CARTESIAN_POINT('Ctrl Pts',(43.8657291158139,-3.18701264822889,0.520888115878363));
#77947=CARTESIAN_POINT('Ctrl Pts',(43.8867175598491,-3.21764322098082,0.21031966200839));
#77948=CARTESIAN_POINT('Ctrl Pts',(43.8939471317267,-3.22283591521967,0.103872347831675));
#77949=CARTESIAN_POINT('Ctrl Pts',(43.901142110102,-3.22274892502026,-0.00263225773335575));
#77950=CARTESIAN_POINT('Ctrl Pts',(43.9000265507268,-3.22274886258475,-0.00270762048436531));
#77951=CARTESIAN_POINT('Ctrl Pts',(43.9096069044335,-3.22261879382433,-0.157522134600772));
#77952=CARTESIAN_POINT('Ctrl Pts',(43.9191872581401,-3.21133027161691,-0.311883592365834));
#77953=CARTESIAN_POINT('Ctrl Pts',(43.9287676118467,-3.18909511021841,-0.464531958514156));
#77954=CARTESIAN_POINT('Ctrl Pts',(43.9306763029786,-3.18466520536568,-0.494944048889516));
#77955=CARTESIAN_POINT('Ctrl Pts',(43.9325849941104,-3.17980092626336,-0.525288252370513));
#77956=CARTESIAN_POINT('Ctrl Pts',(43.9344936852422,-3.17450413358386,-0.555554739300273));
#77957=CARTESIAN_POINT('Ctrl Pts',(43.940665933334,-3.15737557990436,-0.653429279127569));
#77958=CARTESIAN_POINT('Ctrl Pts',(43.9468381814259,-3.13568621731844,-0.750683199551832));
#77959=CARTESIAN_POINT('Ctrl Pts',(43.9530104295177,-3.10949324956114,-0.846858484892082));
#77960=CARTESIAN_POINT('Ctrl Pts',(43.9591743181695,-3.08333575648705,-0.942903514363202));
#77961=CARTESIAN_POINT('Ctrl Pts',(43.9653382068212,-3.05268689480415,-1.03787239694889));
#77962=CARTESIAN_POINT('Ctrl Pts',(43.9715020954729,-3.01765519470704,-1.13131546809791));
#77963=CARTESIAN_POINT('Ctrl Pts',(43.9776594571306,-2.98266058997488,-1.22465959158478));
#77964=CARTESIAN_POINT('Ctrl Pts',(43.9838168187882,-2.94329252526662,-1.31648071129962));
#77965=CARTESIAN_POINT('Ctrl Pts',(43.9899741804459,-2.89970957094703,-1.40634347392739));
#77966=CARTESIAN_POINT('Ctrl Pts',(43.9961270445913,-2.85615845085793,-1.49614059823527));
#77967=CARTESIAN_POINT('Ctrl Pts',(44.0022799087367,-2.80839875107193,-1.58398181975867));
#77968=CARTESIAN_POINT('Ctrl Pts',(44.0084327728821,-2.75663711508082,-1.66945181968779));
#77969=CARTESIAN_POINT('Ctrl Pts',(44.0145833060178,-2.70489508896184,-1.75488943934654));
#77970=CARTESIAN_POINT('Ctrl Pts',(44.0207338391534,-2.6491543639489,-1.83795725126199));
#77971=CARTESIAN_POINT('Ctrl Pts',(44.0268843722891,-2.58966704930943,-1.91826539775417));
#77972=CARTESIAN_POINT('Ctrl Pts',(44.0330342205034,-2.53018635915748,-1.99856460115795));
#77973=CARTESIAN_POINT('Ctrl Pts',(44.0391840687177,-2.46696016742312,-2.07610440108029));
#77974=CARTESIAN_POINT('Ctrl Pts',(44.0453339169321,-2.40028275318897,-2.15052557930464));
#77975=CARTESIAN_POINT('Ctrl Pts',(44.0514847253103,-2.33359492873871,-2.22495837676405));
#77976=CARTESIAN_POINT('Ctrl Pts',(44.0576355336886,-2.26345510141153,-2.29627126185731));
#77977=CARTESIAN_POINT('Ctrl Pts',(44.0637863420669,-2.19019582233104,-2.36414039818782));
#77978=CARTESIAN_POINT('Ctrl Pts',(44.0699437284322,-2.11685819605443,-2.43208211722186));
#77979=CARTESIAN_POINT('Ctrl Pts',(44.0761011147976,-2.04039477544658,-2.49657243730347));
#77980=CARTESIAN_POINT('Ctrl Pts',(44.0822585011629,-1.9611726619434,-2.55732660263523));
#77981=CARTESIAN_POINT('Ctrl Pts',(44.088419323899,-1.88190633543491,-2.61811467421003));
#77982=CARTESIAN_POINT('Ctrl Pts',(44.0945801466351,-1.79987860656931,-2.67516219055248));
#77983=CARTESIAN_POINT('Ctrl Pts',(44.1007409693713,-1.71548539930341,-2.72822788770968));
#77984=CARTESIAN_POINT('Ctrl Pts',(44.1069120922871,-1.63095109640112,-2.7813823045465));
#77985=CARTESIAN_POINT('Ctrl Pts',(44.113083215203,-1.54404379375434,-2.83054139080731));
#77986=CARTESIAN_POINT('Ctrl Pts',(44.1192543381189,-1.45518394917245,-2.87550990896761));
#77987=CARTESIAN_POINT('Ctrl Pts',(44.1239498600732,-1.38757172417166,-2.90972583160524));
#77988=CARTESIAN_POINT('Ctrl Pts',(44.1286453820276,-1.3188295870886,-2.94151658870071));
#77989=CARTESIAN_POINT('Ctrl Pts',(44.1333409039819,-1.24914929040216,-2.97081531112046));
#77990=CARTESIAN_POINT('Ctrl Pts',(44.1395131520737,-1.1575547706802,-3.00932838491779));
#77991=CARTESIAN_POINT('Ctrl Pts',(44.1456854001654,-1.06401624545754,-3.04366929034211));
#77992=CARTESIAN_POINT('Ctrl Pts',(44.1518576482571,-0.968949932253002,
-3.07363849391676));
#77993=CARTESIAN_POINT('Ctrl Pts',(44.1580215369087,-0.874012372971452,
-3.10356710842891));
#77994=CARTESIAN_POINT('Ctrl Pts',(44.1641854255603,-0.777551549047892,
-3.12913565999139));
#77995=CARTESIAN_POINT('Ctrl Pts',(44.1703493142118,-0.680004405698589,
-3.15019230694421));
#77996=CARTESIAN_POINT('Ctrl Pts',(44.1765066758693,-0.582560555848621,
-3.17122665683458));
#77997=CARTESIAN_POINT('Ctrl Pts',(44.1826640375268,-0.484033095757913,
-3.18775850947409));
#77998=CARTESIAN_POINT('Ctrl Pts',(44.1888213991842,-0.3848739891357,-3.19968585567189));
#77999=CARTESIAN_POINT('Ctrl Pts',(44.1949742633295,-0.285787311148003,
-3.21160448979647));
#78000=CARTESIAN_POINT('Ctrl Pts',(44.2011271274747,-0.18607033388292,-3.21892525250218));
#78001=CARTESIAN_POINT('Ctrl Pts',(44.2072799916199,-0.0861841614773,-3.22159740700331));
#78002=CARTESIAN_POINT('Ctrl Pts',(44.2134305247554,0.0136641690974123,
-3.22426854915993));
#78003=CARTESIAN_POINT('Ctrl Pts',(44.2195810578908,0.113681133709421,-3.22229457085069));
#78004=CARTESIAN_POINT('Ctrl Pts',(44.2257315910263,0.213402462540845,-3.2156767485992));
#78005=CARTESIAN_POINT('Ctrl Pts',(44.2318814392404,0.313112686438066,-3.20905966330621));
#78006=CARTESIAN_POINT('Ctrl Pts',(44.2380312874545,0.412526906585908,-3.19779979097804));
#78007=CARTESIAN_POINT('Ctrl Pts',(44.2441811356686,0.511183825705347,-3.18195044883437));
#78008=CARTESIAN_POINT('Ctrl Pts',(44.2503319440466,0.609856147939027,-3.16609863216352));
#78009=CARTESIAN_POINT('Ctrl Pts',(44.2564827524247,0.707770505380661,-3.14565599133951));
#78010=CARTESIAN_POINT('Ctrl Pts',(44.2626335608027,0.804474670169112,-3.12072716967637));
#78011=CARTESIAN_POINT('Ctrl Pts',(44.2687909471678,0.901282255305708,-3.09577168786451));
#78012=CARTESIAN_POINT('Ctrl Pts',(44.2749483335329,0.996876641878205,-3.06632055324456));
#78013=CARTESIAN_POINT('Ctrl Pts',(44.2811057198979,1.09081979526626,-3.0325286044414));
#78014=CARTESIAN_POINT('Ctrl Pts',(44.2872665426338,1.1848153773127,-2.99871779671689));
#78015=CARTESIAN_POINT('Ctrl Pts',(44.2934273653697,1.27715748948332,-2.96056151619983));
#78016=CARTESIAN_POINT('Ctrl Pts',(44.2995881881055,1.36742909825289,-2.91826236376226));
#78017=CARTESIAN_POINT('Ctrl Pts',(44.3057593110211,1.45785163066296,-2.87589249205688));
#78018=CARTESIAN_POINT('Ctrl Pts',(44.3119304339367,1.54619636063744,-2.82936611566188));
#78019=CARTESIAN_POINT('Ctrl Pts',(44.3181015568523,1.63207170678766,-2.77893136050591));
#78020=CARTESIAN_POINT('Ctrl Pts',(44.3227970788087,1.69741306829971,-2.74055625382915));
#78021=CARTESIAN_POINT('Ctrl Pts',(44.3274926007651,1.76132531397057,-2.69991934319405));
#78022=CARTESIAN_POINT('Ctrl Pts',(44.3321881227215,1.82364851036005,-2.65714577567012));
#78023=CARTESIAN_POINT('Ctrl Pts',(44.3383603708198,1.90557214610582,-2.60092006247854));
#78024=CARTESIAN_POINT('Ctrl Pts',(44.3445326189181,1.98503726029677,-2.54080310036477));
#78025=CARTESIAN_POINT('Ctrl Pts',(44.3507048670164,2.06165095051911,-2.47703712542296));
#78026=CARTESIAN_POINT('Ctrl Pts',(44.3568687556746,2.13816087829606,-2.41335751250696));
#78027=CARTESIAN_POINT('Ctrl Pts',(44.3630326443327,2.21182672703464,-2.34603898510911));
#78028=CARTESIAN_POINT('Ctrl Pts',(44.3691965329909,2.28228450542419,-2.27536700310096));
#78029=CARTESIAN_POINT('Ctrl Pts',(44.3753538946549,2.3526676754735,-2.20476985625509));
#78030=CARTESIAN_POINT('Ctrl Pts',(44.381511256319,2.41984922384378,-2.1308266204447));
#78031=CARTESIAN_POINT('Ctrl Pts',(44.3876686179831,2.48349895808877,-2.05386233415777));
#78032=CARTESIAN_POINT('Ctrl Pts',(44.3938214821349,2.54710220075582,-1.97695426477664));
#78033=CARTESIAN_POINT('Ctrl Pts',(44.3999743462868,2.60717848226385,-1.89702986586594));
#78034=CARTESIAN_POINT('Ctrl Pts',(44.4061272104386,2.66343579864805,-1.81444958843722));
#78035=CARTESIAN_POINT('Ctrl Pts',(44.4122777435806,2.7196718019736,-1.73190059650896));
#78036=CARTESIAN_POINT('Ctrl Pts',(44.4184282767227,2.77209147069796,-1.64669808392377));
#78037=CARTESIAN_POINT('Ctrl Pts',(44.4245788098647,2.82044484319969,-1.55923328882123));
#78038=CARTESIAN_POINT('Ctrl Pts',(44.4307286580854,2.86879283108576,-1.4717782337695));
#78039=CARTESIAN_POINT('Ctrl Pts',(44.4368785063061,2.91307521286436,-1.38206177721953));
#78040=CARTESIAN_POINT('Ctrl Pts',(44.4430283545268,2.95308741129367,-1.2905007957219));
#78041=CARTESIAN_POINT('Ctrl Pts',(44.4491791629114,2.99310585675014,-1.1989255189853));
#78042=CARTESIAN_POINT('Ctrl Pts',(44.4553299712961,3.02885262067261,-1.10550554336071));
#78043=CARTESIAN_POINT('Ctrl Pts',(44.4614807796807,3.0601712057145,-1.01067786866827));
#78044=CARTESIAN_POINT('Ctrl Pts',(44.4676381660523,3.09152328444239,-0.915748780442773));
#78045=CARTESIAN_POINT('Ctrl Pts',(44.4737955524239,3.11843759105824,-0.819409400157921));
#78046=CARTESIAN_POINT('Ctrl Pts',(44.4799529387955,3.14080752738901,-0.722111929271725));
#78047=CARTESIAN_POINT('Ctrl Pts',(44.4861137615378,3.16318994813931,-0.624760157719311));
#78048=CARTESIAN_POINT('Ctrl Pts',(44.4922745842801,3.18102287033894,-0.526449658132515));
#78049=CARTESIAN_POINT('Ctrl Pts',(44.4984354070225,3.19425122935006,-0.427640791197048));
#78050=CARTESIAN_POINT('Ctrl Pts',(44.5046065299444,3.20750170464007,-0.328666727319451));
#78051=CARTESIAN_POINT('Ctrl Pts',(44.5107776528664,3.21613220207214,-0.229193064728275));
#78052=CARTESIAN_POINT('Ctrl Pts',(44.5169487757883,3.22013971532271,-0.129683369409323));
#78053=CARTESIAN_POINT('Ctrl Pts',(44.5216442976793,3.22318897660537,-0.0539678215838685));
#78054=CARTESIAN_POINT('Ctrl Pts',(44.5263398195703,3.22356285074246,0.0217685218144568));
#78055=CARTESIAN_POINT('Ctrl Pts',(44.5310353414613,3.22128013491466,0.0973234550568934));
#78056=CARTESIAN_POINT('Ctrl Pts',(44.5372077907022,3.21827941467403,0.196643403119909));
#78057=CARTESIAN_POINT('Ctrl Pts',(44.5433802399431,3.21067569309872,0.295999261434805));
#78058=CARTESIAN_POINT('Ctrl Pts',(44.549552689184,3.1984602949907,0.394929492274231));
#78059=CARTESIAN_POINT('Ctrl Pts',(44.5557167273029,3.18626154265824,0.493724912082246));
#78060=CARTESIAN_POINT('Ctrl Pts',(44.5618807654217,3.16946365769102,0.592095429893225));
#78061=CARTESIAN_POINT('Ctrl Pts',(44.5680448035406,3.14810996312968,0.689580468505031));
#78062=CARTESIAN_POINT('Ctrl Pts',(44.5743914446661,3.12612368830928,0.789953396648254));
#78063=CARTESIAN_POINT('Ctrl Pts',(44.5807380857916,3.09930744334619,0.889387094077229));
#78064=CARTESIAN_POINT('Ctrl Pts',(44.5870847269171,3.06776600361313,0.987385086769861));
#78065=CARTESIAN_POINT('Ctrl Pts',(44.5932373666891,3.03718870883173,1.08238751962989));
#78066=CARTESIAN_POINT('Ctrl Pts',(44.599390006461,3.00217104426191,1.17604029840144));
#78067=CARTESIAN_POINT('Ctrl Pts',(44.605542646233,2.96285985464771,1.26790340492364));
#78068=CARTESIAN_POINT('Ctrl Pts',(44.6116929325193,2.92356370220853,1.35973137230035));
#78069=CARTESIAN_POINT('Ctrl Pts',(44.6178432188056,2.87997745949126,1.44977062912724));
#78070=CARTESIAN_POINT('Ctrl Pts',(44.6239935050919,2.83229652355686,1.53760006671038));
#78071=CARTESIAN_POINT('Ctrl Pts',(44.6301430839192,2.78462107229512,1.62541940139375));
#78072=CARTESIAN_POINT('Ctrl Pts',(44.6362926627465,2.7328520721566,1.71102904090691));
#78073=CARTESIAN_POINT('Ctrl Pts',(44.6424422415738,2.67723092407883,1.79403236917732));
#78074=CARTESIAN_POINT('Ctrl Pts',(44.6485927579275,2.62160129634751,1.87704835161782));
#78075=CARTESIAN_POINT('Ctrl Pts',(44.6547432742813,2.56211859665406,1.95745687328124));
#78076=CARTESIAN_POINT('Ctrl Pts',(44.660893790635,2.49906702543883,2.03489104496145));
#78077=CARTESIAN_POINT('Ctrl Pts',(44.6670500122561,2.43595696709016,2.11239704518845));
#78078=CARTESIAN_POINT('Ctrl Pts',(44.6732062338773,2.36927170495756,2.1869228520603));
#78079=CARTESIAN_POINT('Ctrl Pts',(44.6793624554984,2.29933492787142,2.25813561416726));
#78080=CARTESIAN_POINT('Ctrl Pts',(44.6855221287894,2.22935893863781,2.32938830384087));
#78081=CARTESIAN_POINT('Ctrl Pts',(44.6916818020804,2.15612812223851,2.39732395465477));
#78082=CARTESIAN_POINT('Ctrl Pts',(44.6978414753715,2.08000072026934,2.46164874955364));
#78083=CARTESIAN_POINT('Ctrl Pts',(44.7040093662931,2.00377175660436,2.52605936027026));
#78084=CARTESIAN_POINT('Ctrl Pts',(44.7101772572147,1.92463883962987,2.5868492382469));
#78085=CARTESIAN_POINT('Ctrl Pts',(44.7163451481363,1.84299047136763,2.64376694981765));
#78086=CARTESIAN_POINT('Ctrl Pts',(44.7176848289418,1.82525624857537,2.65612961424445));
#78087=CARTESIAN_POINT('Ctrl Pts',(44.7190245097473,1.80740345041526,2.66830977218673));
#78088=CARTESIAN_POINT('Ctrl Pts',(44.7203641905528,1.78943621037803,2.68030513402633));
#78089=CARTESIAN_POINT('Origin',(-1.72497344927317,0.,0.));
#78090=CARTESIAN_POINT('',(46.216937227185,1.78943621037807,2.68030513402631));
#78091=CARTESIAN_POINT('',(45.9705987712989,1.78932308991453,2.68012452748162));
#78092=CARTESIAN_POINT('',(-1.72497344927317,1.78943621037804,2.68030513402633));
#78093=CARTESIAN_POINT('',(45.3965734492404,-3.22274967111447,0.00145596415035607));
#78094=CARTESIAN_POINT('Ctrl Pts',(45.396573449273,-3.22274967111471,0.00145596361978267));
#78095=CARTESIAN_POINT('Ctrl Pts',(45.4028312200437,-3.22279569093976,-0.100408103620474));
#78096=CARTESIAN_POINT('Ctrl Pts',(45.4090889908143,-3.21800781208672,-0.202255132764274));
#78097=CARTESIAN_POINT('Ctrl Pts',(45.415346761585,-3.2084172616612,-0.303605397801885));
#78098=CARTESIAN_POINT('Ctrl Pts',(45.4216072500032,-3.19882254621644,-0.40499967760246));
#78099=CARTESIAN_POINT('Ctrl Pts',(45.4278677384214,-3.1844210469915,-0.505896352872799));
#78100=CARTESIAN_POINT('Ctrl Pts',(45.4341282268395,-3.16529571634117,-0.605822243411565));
#78101=CARTESIAN_POINT('Ctrl Pts',(45.4406927782651,-3.14524149561597,-0.710601392157561));
#78102=CARTESIAN_POINT('Ctrl Pts',(45.4472573296907,-3.11999311937981,-0.814312578103785));
#78103=CARTESIAN_POINT('Ctrl Pts',(45.4538218811163,-3.08970564774613,-0.916425977799434));
#78104=CARTESIAN_POINT('Ctrl Pts',(45.4600966167591,-3.06075532571062,-1.01403121342577));
#78105=CARTESIAN_POINT('Ctrl Pts',(45.4663713524019,-3.02720158720057,-1.11017637426488));
#78106=CARTESIAN_POINT('Ctrl Pts',(45.4726460880447,-2.98922957059347,-1.20441858869314));
#78107=CARTESIAN_POINT('Ctrl Pts',(45.4789267294548,-2.95122181480891,-1.29874950368374));
#78108=CARTESIAN_POINT('Ctrl Pts',(45.4852073708648,-2.90878766842503,-1.39117353019518));
#78109=CARTESIAN_POINT('Ctrl Pts',(45.4914880122748,-2.86215862993982,-1.48127159547499));
#78110=CARTESIAN_POINT('Ctrl Pts',(45.4977796281942,-2.8154481139765,-1.57152709404916));
#78111=CARTESIAN_POINT('Ctrl Pts',(45.5040712441137,-2.7645282803184,-1.65944816268342));
#78112=CARTESIAN_POINT('Ctrl Pts',(45.5103628600331,-2.70967440190764,-1.74464385997443));
#78113=CARTESIAN_POINT('Ctrl Pts',(45.5112095213377,-2.70229272812937,-1.75610862532804));
#78114=CARTESIAN_POINT('Ctrl Pts',(45.5120561826423,-2.69483987223226,-1.76752408602211));
#78115=CARTESIAN_POINT('Ctrl Pts',(45.5129028439468,-2.68731655974303,-1.77888933613952));
#78116=CARTESIAN_POINT('Ctrl Pts',(45.5190750921054,-2.63247083642038,-1.8617431806827));
#78117=CARTESIAN_POINT('Ctrl Pts',(45.525247340264,-2.57369323324841,-1.942204021402));
#78118=CARTESIAN_POINT('Ctrl Pts',(45.5314195884226,-2.51121937177829,-2.01987495387845));
#78119=CARTESIAN_POINT('Ctrl Pts',(45.537583477137,-2.4488301223878,-2.0974406919749));
#78120=CARTESIAN_POINT('Ctrl Pts',(45.5437473658515,-2.38275483465068,-2.17222369659909));
#78121=CARTESIAN_POINT('Ctrl Pts',(45.549911254566,-2.31327283205333,-2.24385524644171));
#78122=CARTESIAN_POINT('Ctrl Pts',(45.5560686162824,-2.24386440458309,-2.315410944982));
#78123=CARTESIAN_POINT('Ctrl Pts',(45.5622259779988,-2.17105673487563,-2.38382151314611));
#78124=CARTESIAN_POINT('Ctrl Pts',(45.5683833397153,-2.09516928556608,-2.44875136086139));
#78125=CARTESIAN_POINT('Ctrl Pts',(45.5745362039133,-2.01933726668512,-2.5136337819031));
#78126=CARTESIAN_POINT('Ctrl Pts',(45.5806890681113,-1.94043026977323,-2.57504025571928));
#78127=CARTESIAN_POINT('Ctrl Pts',(45.5868419323094,-1.85880380462553,-2.63267278225184));
#78128=CARTESIAN_POINT('Ctrl Pts',(45.5929924654938,-1.77720826367673,-2.69028347469285));
#78129=CARTESIAN_POINT('Ctrl Pts',(45.5991429986783,-1.69289565608329,-2.74412281051767));
#78130=CARTESIAN_POINT('Ctrl Pts',(45.6052935318628,-1.60625297860078,-2.79393431047262));
#78131=CARTESIAN_POINT('Ctrl Pts',(45.6114433801222,-1.5196199496716,-2.84374026340469));
#78132=CARTESIAN_POINT('Ctrl Pts',(45.6175932283815,-1.43065774331018,-2.88951905573437));
#78133=CARTESIAN_POINT('Ctrl Pts',(45.6237430766409,-1.33977975121226,-2.93105915681373));
#78134=CARTESIAN_POINT('Ctrl Pts',(45.6298938850603,-1.24888757056588,-2.97260574344282));
#78135=CARTESIAN_POINT('Ctrl Pts',(45.6360446934797,-1.15607940517697,-3.00991214376555));
#78136=CARTESIAN_POINT('Ctrl Pts',(45.6421955018992,-1.06178957245985,-3.04281456324823));
#78137=CARTESIAN_POINT('Ctrl Pts',(45.6483528882995,-0.967398901498728,
-3.07575217021729));
#78138=CARTESIAN_POINT('Ctrl Pts',(45.6545102746998,-0.871523809911516,
-3.10427624789803));
#78139=CARTESIAN_POINT('Ctrl Pts',(45.6606676611002,-0.774614650359711,
-3.12827263932479));
#78140=CARTESIAN_POINT('Ctrl Pts',(45.6668284838679,-0.677651406906714,
-3.15228242286505));
#78141=CARTESIAN_POINT('Ctrl Pts',(45.6729893066357,-0.579653372255442,
-3.171759403286));
#78142=CARTESIAN_POINT('Ctrl Pts',(45.6791501294034,-0.481079920266214,
-3.18664081327291));
#78143=CARTESIAN_POINT('Ctrl Pts',(45.6853212523452,-0.382341665012466,
-3.20154710323407));
#78144=CARTESIAN_POINT('Ctrl Pts',(45.6914923752869,-0.283026503055811,
-3.21184243088581));
#78145=CARTESIAN_POINT('Ctrl Pts',(45.6976634982286,-0.183597885011521,
-3.21751602624125));
#78146=CARTESIAN_POINT('Ctrl Pts',(45.7023590197146,-0.107944034528595,
-3.22183298591709));
#78147=CARTESIAN_POINT('Ctrl Pts',(45.7070545412005,-0.0322245824695204,
-3.22347528245398));
#78148=CARTESIAN_POINT('Ctrl Pts',(45.7117500626865,0.0433579790249112,
-3.2224583237266));
#78149=CARTESIAN_POINT('Ctrl Pts',(45.7179223123319,0.142711041252509,-3.22112153437035));
#78150=CARTESIAN_POINT('Ctrl Pts',(45.7240945619773,0.242177094397714,-3.21518328861998));
#78151=CARTESIAN_POINT('Ctrl Pts',(45.7302668116227,0.341294855735243,-3.20462718330053));
#78152=CARTESIAN_POINT('Ctrl Pts',(45.7364307018349,0.440278376179301,-3.19408537472255));
#78153=CARTESIAN_POINT('Ctrl Pts',(45.7425945920472,0.538914114265246,-3.17893818314863));
#78154=CARTESIAN_POINT('Ctrl Pts',(45.7487584822594,0.636740865088272,-3.15922120675755));
#78155=CARTESIAN_POINT('Ctrl Pts',(45.7549158454823,0.734464026436455,-3.13952510881958));
#78156=CARTESIAN_POINT('Ctrl Pts',(45.7610732087053,0.831379480143805,-3.11526893176137));
#78157=CARTESIAN_POINT('Ctrl Pts',(45.7672305719282,0.927032187966362,-3.08653995356845));
#78158=CARTESIAN_POINT('Ctrl Pts',(45.7733834376398,1.02261502835973,-3.05783195982955));
#78159=CARTESIAN_POINT('Ctrl Pts',(45.7795363033514,1.11693654188626,-3.02465778500215));
#78160=CARTESIAN_POINT('Ctrl Pts',(45.7856891690631,1.20955382030329,-2.98715535556652));
#78161=CARTESIAN_POINT('Ctrl Pts',(45.791839703765,1.30213601071674,-2.94966713390508));
#78162=CARTESIAN_POINT('Ctrl Pts',(45.7979902384669,1.39301484674711,-2.90785407867085));
#78163=CARTESIAN_POINT('Ctrl Pts',(45.8041407731688,1.48176532251175,-2.86190305417595));
#78164=CARTESIAN_POINT('Ctrl Pts',(45.8102906229476,1.57050591503006,-2.8159571467837));
#78165=CARTESIAN_POINT('Ctrl Pts',(45.8164404727265,1.65711823276217,-2.76587438599479));
#78166=CARTESIAN_POINT('Ctrl Pts',(45.8225903225053,1.74120080898654,-2.7118881439478));
#78167=CARTESIAN_POINT('Ctrl Pts',(45.8287411324445,1.8252965128092,-2.65789347316645));
#78168=CARTESIAN_POINT('Ctrl Pts',(45.8348919423837,1.90686132507393,-2.59999434532863));
#78169=CARTESIAN_POINT('Ctrl Pts',(45.8410427523229,1.98552262035817,-2.53846754687667));
#78170=CARTESIAN_POINT('Ctrl Pts',(45.847200140234,2.06426803981365,-2.4768749487082));
#78171=CARTESIAN_POINT('Ctrl Pts',(45.8533575281451,2.14010339879176,-2.41164720089274));
#78172=CARTESIAN_POINT('Ctrl Pts',(45.8595149160562,2.21268915701501,-2.3431014184043));
#78173=CARTESIAN_POINT('Ctrl Pts',(45.865675740332,2.28531542448442,-2.27451738133197));
#78174=CARTESIAN_POINT('Ctrl Pts',(45.8718365646079,2.35468817790787,-2.20261193445683));
#78175=CARTESIAN_POINT('Ctrl Pts',(45.8779973888838,2.4205062285847,-2.12773756837695));
#78176=CARTESIAN_POINT('Ctrl Pts',(45.8841685133135,2.4864343190907,-2.05273802140265));
#78177=CARTESIAN_POINT('Ctrl Pts',(45.8903396377433,2.5487955644018,-1.97475997983011));
#78178=CARTESIAN_POINT('Ctrl Pts',(45.896510762173,2.6073303120889,-1.89418747914835));
#78179=CARTESIAN_POINT('Ctrl Pts',(45.9012062685907,2.65186843258084,-1.83288119723041));
#78180=CARTESIAN_POINT('Ctrl Pts',(45.9059017750084,2.69419208812412,-1.77007352280184));
#78181=CARTESIAN_POINT('Ctrl Pts',(45.9105972814261,2.73420475130028,-1.70594312345604));
#78182=CARTESIAN_POINT('Ctrl Pts',(45.9167695260658,2.78680140943208,-1.62164369366314));
#78183=CARTESIAN_POINT('Ctrl Pts',(45.9229417707054,2.83558838376867,-1.53476116288655));
#78184=CARTESIAN_POINT('Ctrl Pts',(45.9291140153451,2.88030245554016,-1.44567469615724));
#78185=CARTESIAN_POINT('Ctrl Pts',(45.9352779005448,2.92495596837081,-1.35670888455627));
#78186=CARTESIAN_POINT('Ctrl Pts',(45.9414417857445,2.9655473495035,-1.26554545466496));
#78187=CARTESIAN_POINT('Ctrl Pts',(45.9476056709442,3.00185716622106,-1.17259162375794));
#78188=CARTESIAN_POINT('Ctrl Pts',(45.9537630291543,3.03812853417031,-1.07973622243914));
#78189=CARTESIAN_POINT('Ctrl Pts',(45.9599203873645,3.07012719412026,-0.985094591646198));
#78190=CARTESIAN_POINT('Ctrl Pts',(45.9660777455747,3.0976805212264,-0.889096705040859));
#78191=CARTESIAN_POINT('Ctrl Pts',(45.9722306062933,3.12521372267929,-0.793168937741693));
#78192=CARTESIAN_POINT('Ctrl Pts',(45.9783834670119,3.14830792737386,-0.695887300459184));
#78193=CARTESIAN_POINT('Ctrl Pts',(45.9845363277305,3.16683967523579,-0.597698949181347));
#78194=CARTESIAN_POINT('Ctrl Pts',(45.990686857453,3.18536440239079,-0.499547796317951));
#78195=CARTESIAN_POINT('Ctrl Pts',(45.9968373871755,3.19933002671357,-0.400491038370601));
#78196=CARTESIAN_POINT('Ctrl Pts',(46.002987916898,3.20866393505546,-0.300987232909302));
#78197=CARTESIAN_POINT('Ctrl Pts',(46.0091377617167,3.21799680400246,-0.201494507881113));
#78198=CARTESIAN_POINT('Ctrl Pts',(46.0152876065354,3.22269894183314,-0.101555266790161));
#78199=CARTESIAN_POINT('Ctrl Pts',(46.0214374513541,3.22274958606181,-0.00163341312231848));
#78200=CARTESIAN_POINT('Ctrl Pts',(46.0275882563582,3.22280023819765,0.0983040415088446));
#78201=CARTESIAN_POINT('Ctrl Pts',(46.0337390613623,3.21819795400046,0.198223668908126));
#78202=CARTESIAN_POINT('Ctrl Pts',(46.0398898663665,3.20897408626979,0.297662352589265));
#78203=CARTESIAN_POINT('Ctrl Pts',(46.0460472494114,3.19974035398008,0.397207381980745));
#78204=CARTESIAN_POINT('Ctrl Pts',(46.0522046324564,3.1858752084948,0.49627000718771));
#78205=CARTESIAN_POINT('Ctrl Pts',(46.0583620155014,3.16746181681086,0.594393137195634));
#78206=CARTESIAN_POINT('Ctrl Pts',(46.0645228349418,3.14903814873278,0.692571029084221));
#78207=CARTESIAN_POINT('Ctrl Pts',(46.0706836543823,3.12606127926863,0.789807958837698));
#78208=CARTESIAN_POINT('Ctrl Pts',(46.0768444738227,3.09866487079108,0.885659969189805));
#78209=CARTESIAN_POINT('Ctrl Pts',(46.0830155935174,3.07122265834579,0.981672234211558));
#78210=CARTESIAN_POINT('Ctrl Pts',(46.0891867132122,3.03934628630086,1.07629454297083));
#78211=CARTESIAN_POINT('Ctrl Pts',(46.0953578329069,3.00321841195402,1.1691008222563));
#78212=CARTESIAN_POINT('Ctrl Pts',(46.1000533886598,2.97572900053088,1.23971637991233));
#78213=CARTESIAN_POINT('Ctrl Pts',(46.1047489444128,2.94577916859904,1.30928090671977));
#78214=CARTESIAN_POINT('Ctrl Pts',(46.1094445001657,2.91346702293576,1.37761658989933));
#78215=CARTESIAN_POINT('Ctrl Pts',(46.1156164258726,2.87099533844129,1.46743828128314));
#78216=CARTESIAN_POINT('Ctrl Pts',(46.1217883515795,2.82429123049196,1.55545212808397));
#78217=CARTESIAN_POINT('Ctrl Pts',(46.1279602772864,2.77353130235211,1.64123175614324));
#78218=CARTESIAN_POINT('Ctrl Pts',(46.1341242044575,2.72283715677691,1.72690021769508));
#78219=CARTESIAN_POINT('Ctrl Pts',(46.1402881316286,2.66809785467939,1.81033984354182));
#78220=CARTESIAN_POINT('Ctrl Pts',(46.1464520587997,2.60953730348872,1.89114584953166));
#78221=CARTESIAN_POINT('Ctrl Pts',(46.1526088291193,2.55104474615357,1.97185803277248));
#78222=CARTESIAN_POINT('Ctrl Pts',(46.1587655994388,2.48874001847481,2.04994232885636));
#78223=CARTESIAN_POINT('Ctrl Pts',(46.1649223697583,2.42289139691823,2.12502113901007));
#78224=CARTESIAN_POINT('Ctrl Pts',(46.1710749117893,2.35708799825572,2.200048387248));
#78225=CARTESIAN_POINT('Ctrl Pts',(46.1772274538203,2.28774582815966,2.27207392623162));
#78226=CARTESIAN_POINT('Ctrl Pts',(46.1833799958513,2.21517422701285,2.34075216682118));
#78227=CARTESIAN_POINT('Ctrl Pts',(46.1895307545825,2.14262366057298,2.40941050118514));
#78228=CARTESIAN_POINT('Ctrl Pts',(46.1956815133137,2.06684583405016,2.47472316248043));
#78229=CARTESIAN_POINT('Ctrl Pts',(46.201832272045,1.98818725954731,2.53638108009695));
#78230=CARTESIAN_POINT('Ctrl Pts',(46.2068672570917,1.92379768360679,2.58685399031425));
#78231=CARTESIAN_POINT('Ctrl Pts',(46.2119022421384,1.85747849723844,2.63487846584619));
#78232=CARTESIAN_POINT('Ctrl Pts',(46.216937227185,1.78943621037807,2.68030513402631));
#78233=CARTESIAN_POINT('Ctrl Pts',(44.9670777766272,1.78943621037802,2.68030513402634));
#78234=CARTESIAN_POINT('Ctrl Pts',(44.9732498862039,1.70620866293451,2.73586984761275));
#78235=CARTESIAN_POINT('Ctrl Pts',(44.9794219957806,1.62031946228957,2.78760190383352));
#78236=CARTESIAN_POINT('Ctrl Pts',(44.9855941053572,1.53215912380563,2.83524354894587));
#78237=CARTESIAN_POINT('Ctrl Pts',(44.9917450764698,1.44430072003734,2.88272202922903));
#78238=CARTESIAN_POINT('Ctrl Pts',(44.9978960475824,1.35418709224094,2.92613786024936));
#78239=CARTESIAN_POINT('Ctrl Pts',(45.004047018695,1.26223192229211,2.96528044826232));
#78240=CARTESIAN_POINT('Ctrl Pts',(45.010196885273,1.17029326480371,3.00441600741071));
#78241=CARTESIAN_POINT('Ctrl Pts',(45.0163467518509,1.07651412203582,3.03927967864055));
#78242=CARTESIAN_POINT('Ctrl Pts',(45.0224966184289,0.981329333323888,3.06970850441179));
#78243=CARTESIAN_POINT('Ctrl Pts',(45.028647025688,0.886136176199941,3.1001400054104));
#78244=CARTESIAN_POINT('Ctrl Pts',(45.0347974329471,0.789537541579017,3.12613575451336));
#78245=CARTESIAN_POINT('Ctrl Pts',(45.0409478402062,0.691983679373301,3.14758258827008));
#78246=CARTESIAN_POINT('Ctrl Pts',(45.047136220728,0.593827509339862,3.16916183703898));
#78247=CARTESIAN_POINT('Ctrl Pts',(45.0533246012498,0.494704708546602,3.1861357026898));
#78248=CARTESIAN_POINT('Ctrl Pts',(45.0595129817715,0.395083056032114,3.19844132998189));
#78249=CARTESIAN_POINT('Ctrl Pts',(45.0656728078821,0.295921077517692,3.21069017667682));
#78250=CARTESIAN_POINT('Ctrl Pts',(45.0718326339927,0.196265281299825,3.21831379667311));
#78251=CARTESIAN_POINT('Ctrl Pts',(45.0779924601033,0.0965794774239169,
3.22130252646977));
#78252=CARTESIAN_POINT('Ctrl Pts',(45.0841951178307,-0.00379947980933119,
3.22431203804289));
#78253=CARTESIAN_POINT('Ctrl Pts',(45.0903977755581,-0.104208416453509,
3.22262196846568));
#78254=CARTESIAN_POINT('Ctrl Pts',(45.0966004332855,-0.20417794773934,3.2162756300039));
#78255=CARTESIAN_POINT('Ctrl Pts',(45.1028030910128,-0.304147479025172,
3.20992929154211));
#78256=CARTESIAN_POINT('Ctrl Pts',(45.1090057487402,-0.403677171599521,
3.19892679497133));
#78257=CARTESIAN_POINT('Ctrl Pts',(45.1152084064676,-0.502308418893908,
3.18336360078586));
#78258=CARTESIAN_POINT('Ctrl Pts',(45.1213806548032,-0.600456112787606,
3.16787670732334));
#78259=CARTESIAN_POINT('Ctrl Pts',(45.1275529031388,-0.69805966120469,3.14781924985067));
#78260=CARTESIAN_POINT('Ctrl Pts',(45.1337251514744,-0.794660154599542,
3.12324075299869));
#78261=CARTESIAN_POINT('Ctrl Pts',(45.1398890403708,-0.891129816259442,
3.09869554425191));
#78262=CARTESIAN_POINT('Ctrl Pts',(45.1460529292671,-0.986598705801894,
3.06964157264494));
#78263=CARTESIAN_POINT('Ctrl Pts',(45.1522168181635,-1.08061540399782,3.03617982193786));
#78264=CARTESIAN_POINT('Ctrl Pts',(45.1583741800664,-1.17453254712581,3.00275350415844));
#78265=CARTESIAN_POINT('Ctrl Pts',(45.1645315419692,-1.26700014910275,2.96492883142535));
#78266=CARTESIAN_POINT('Ctrl Pts',(45.1706889038721,-1.35758026182949,2.92285706034198));
#78267=CARTESIAN_POINT('Ctrl Pts',(45.1768417682625,-1.44809421226379,2.88081601967767));
#78268=CARTESIAN_POINT('Ctrl Pts',(45.182994632653,-1.53672302172453,2.83453423079885));
#78269=CARTESIAN_POINT('Ctrl Pts',(45.1891474970435,-1.62304796865347,2.7842113522414));
#78270=CARTESIAN_POINT('Ctrl Pts',(45.195298030424,-1.70934021141462,2.73390753848412));
#78271=CARTESIAN_POINT('Ctrl Pts',(45.2014485638045,-1.79332995107658,2.67956589558555));
#78272=CARTESIAN_POINT('Ctrl Pts',(45.207599097185,-1.87462316215416,2.62143196791661));
#78273=CARTESIAN_POINT('Ctrl Pts',(45.2137489456438,-1.95590732044119,2.56330451402652));
#78274=CARTESIAN_POINT('Ctrl Pts',(45.2198987941025,-2.03449519382623,2.50138586764527));
#78275=CARTESIAN_POINT('Ctrl Pts',(45.2260486425613,-2.11002268570649,2.43596425021057));
#78276=CARTESIAN_POINT('Ctrl Pts',(45.2321994511833,-2.18556196953902,2.37053241863305));
#78277=CARTESIAN_POINT('Ctrl Pts',(45.2383502598052,-2.25803959445055,2.30159681411835));
#78278=CARTESIAN_POINT('Ctrl Pts',(45.2445010684272,-2.32712619969376,2.22948451737142));
#78279=CARTESIAN_POINT('Ctrl Pts',(45.2506584550336,-2.39628668963083,2.15729510010381));
#78280=CARTESIAN_POINT('Ctrl Pts',(45.2568158416399,-2.46204861701465,2.0819225207886));
#78281=CARTESIAN_POINT('Ctrl Pts',(45.2629732282463,-2.52412111754724,2.00372906014064));
#78282=CARTESIAN_POINT('Ctrl Pts',(45.2691340512224,-2.58622826005899,1.92549196058316));
#78283=CARTESIAN_POINT('Ctrl Pts',(45.2752948741984,-2.64464162123501,1.84443119691035));
#78284=CARTESIAN_POINT('Ctrl Pts',(45.2814556971745,-2.69911333978492,1.76093859674183));
#78285=CARTESIAN_POINT('Ctrl Pts',(45.287626820326,-2.75367612867754,1.67730640671066));
#78286=CARTESIAN_POINT('Ctrl Pts',(45.2937979434775,-2.8042838914251,1.59123463360137));
#78287=CARTESIAN_POINT('Ctrl Pts',(45.2999690666291,-2.85073437580245,1.50314040632212));
#78288=CARTESIAN_POINT('Ctrl Pts',(45.3046645861551,-2.88607788638083,1.43611076614776));
#78289=CARTESIAN_POINT('Ctrl Pts',(45.3093601056811,-2.9190154984685,1.36791075557459));
#78290=CARTESIAN_POINT('Ctrl Pts',(45.3140556252071,-2.94947714083506,1.29873097991518));
#78291=CARTESIAN_POINT('Ctrl Pts',(45.3209321105432,-2.99408754781707,1.19741871611951));
#78292=CARTESIAN_POINT('Ctrl Pts',(45.3278085958793,-3.03352293723517,1.09369460885342));
#78293=CARTESIAN_POINT('Ctrl Pts',(45.3346850812154,-3.06754223427876,0.98808005921386));
#78294=CARTESIAN_POINT('Ctrl Pts',(45.3414563185369,-3.10104084912839,0.88408199257659));
#78295=CARTESIAN_POINT('Ctrl Pts',(45.3482275558585,-3.12928783886883,0.778251211611842));
#78296=CARTESIAN_POINT('Ctrl Pts',(45.35499879318,-3.15209929248381,0.671109240603247));
#78297=CARTESIAN_POINT('Ctrl Pts',(45.3619279025234,-3.1754425972411,0.561469244671201));
#78298=CARTESIAN_POINT('Ctrl Pts',(45.3688570118668,-3.19309357957785,0.450456397961443));
#78299=CARTESIAN_POINT('Ctrl Pts',(45.3757861212102,-3.20490764928325,0.338651032872615));
#78300=CARTESIAN_POINT('Ctrl Pts',(45.3827152305536,-3.21672171898867,0.226845667783756));
#78301=CARTESIAN_POINT('Ctrl Pts',(45.389644339897,-3.22269871422779,0.11424808868431));
#78302=CARTESIAN_POINT('Ctrl Pts',(45.3965734492404,-3.22274967111447,0.00145596415041658));
#78303=CARTESIAN_POINT('',(45.1500265507268,-3.22274935820264,0.00203388900681504));
#78304=CARTESIAN_POINT('Ctrl Pts',(44.7203641905528,1.78943621037803,2.68030513402633));
#78305=CARTESIAN_POINT('Ctrl Pts',(44.7235369804355,1.74688407618643,2.70871396285133));
#78306=CARTESIAN_POINT('Ctrl Pts',(44.7267097703181,1.70368994908445,2.73608605417297));
#78307=CARTESIAN_POINT('Ctrl Pts',(44.7298825602008,1.65990979412347,2.76239335321257));
#78308=CARTESIAN_POINT('Ctrl Pts',(44.7360548082891,1.57474122395254,2.81357076558717));
#78309=CARTESIAN_POINT('Ctrl Pts',(44.7422270563773,1.48705372016049,2.86089576058143));
#78310=CARTESIAN_POINT('Ctrl Pts',(44.7483993044656,1.39723080362417,2.9041115067958));
#78311=CARTESIAN_POINT('Ctrl Pts',(44.7545631931136,1.30752953957013,2.94726872337204));
#78312=CARTESIAN_POINT('Ctrl Pts',(44.7607270817616,1.21569899915141,2.986327566344));
#78313=CARTESIAN_POINT('Ctrl Pts',(44.7668909704096,1.12215001817333,3.02107545407486));
#78314=CARTESIAN_POINT('Ctrl Pts',(44.7730483320635,1.02870009700774,3.05578654697153));
#78315=CARTESIAN_POINT('Ctrl Pts',(44.7792056937173,0.933535757908711,3.08619560967981));
#78316=CARTESIAN_POINT('Ctrl Pts',(44.7853630553712,0.837089805889483,3.11213724301739));
#78317=CARTESIAN_POINT('Ctrl Pts',(44.7915159195127,0.740714300740688,3.13805992784709));
#78318=CARTESIAN_POINT('Ctrl Pts',(44.7976687836542,0.643059462053335,3.15952155849571));
#78319=CARTESIAN_POINT('Ctrl Pts',(44.8038216477957,0.544574451297885,3.17640618144053));
#78320=CARTESIAN_POINT('Ctrl Pts',(44.8099721809274,0.446126751544787,3.19328440765349));
#78321=CARTESIAN_POINT('Ctrl Pts',(44.8161227140591,0.346849932307474,3.20558899828749));
#78322=CARTESIAN_POINT('Ctrl Pts',(44.8222732471908,0.247203703415233,3.21325503057535));
#78323=CARTESIAN_POINT('Ctrl Pts',(44.8284230954011,0.14756857109483,3.22092020917633));
#78324=CARTESIAN_POINT('Ctrl Pts',(44.8345729436113,0.047564544002484,3.22394782308566));
#78325=CARTESIAN_POINT('Ctrl Pts',(44.8407227918216,-0.0523441912946446,
3.22232488246262));
#78326=CARTESIAN_POINT('Ctrl Pts',(44.8468736001958,-0.15226852514893,3.220701688453));
#78327=CARTESIAN_POINT('Ctrl Pts',(44.85302440857,-0.252097103298146,3.2144265047803));
#78328=CARTESIAN_POINT('Ctrl Pts',(44.8591752169442,-0.351367398917399,
3.20353843639779));
#78329=CARTESIAN_POINT('Ctrl Pts',(44.8653326033054,-0.450743859234878,
3.19263872376172));
#78330=CARTESIAN_POINT('Ctrl Pts',(44.8714899896666,-0.549560412136144,
3.1771163226696));
#78331=CARTESIAN_POINT('Ctrl Pts',(44.8776473760278,-0.647361423232053,
3.1570620440864));
#78332=CARTESIAN_POINT('Ctrl Pts',(44.8838081987597,-0.745217016014586,
3.13699657342719));
#78333=CARTESIAN_POINT('Ctrl Pts',(44.8899690214916,-0.84205551727638,3.11239429538733));
#78334=CARTESIAN_POINT('Ctrl Pts',(44.8961298442235,-0.937435270241421,
3.08339628925758));
#78335=CARTESIAN_POINT('Ctrl Pts',(44.9023009671352,-1.03297448707043,3.0543498018311));
#78336=CARTESIAN_POINT('Ctrl Pts',(44.9084720900469,-1.12704967460522,3.02089305223879));
#78337=CARTESIAN_POINT('Ctrl Pts',(44.9146432129585,-1.21923787819585,2.98321580829689));
#78338=CARTESIAN_POINT('Ctrl Pts',(44.9193387349525,-1.28938260610739,2.95454771496364));
#78339=CARTESIAN_POINT('Ctrl Pts',(44.9240342569465,-1.35843525740968,2.92343718470311));
#78340=CARTESIAN_POINT('Ctrl Pts',(44.9287297789405,-1.42621969123783,2.88998528626453));
#78341=CARTESIAN_POINT('Ctrl Pts',(44.9349020270704,-1.51532210529602,2.84601287641504));
#78342=CARTESIAN_POINT('Ctrl Pts',(44.9410742752002,-1.60254584467215,2.79783847557569));
#78343=CARTESIAN_POINT('Ctrl Pts',(44.94724652333,-1.68746748683512,2.74564583356528));
#78344=CARTESIAN_POINT('Ctrl Pts',(44.9534104120199,-1.77227411460465,2.6935238791312));
#78345=CARTESIAN_POINT('Ctrl Pts',(44.9595743007097,-1.85478447545235,2.63739472582188));
#78346=CARTESIAN_POINT('Ctrl Pts',(44.9657381893995,-1.93459760068094,2.577489027317));
#78347=CARTESIAN_POINT('Ctrl Pts',(44.9718955510953,-2.01432621111425,2.5176467634644));
#78348=CARTESIAN_POINT('Ctrl Pts',(44.9780529127911,-2.09136291868725,2.45403616415223));
#78349=CARTESIAN_POINT('Ctrl Pts',(44.9842102744869,-2.1653345660287,2.38693187578978));
#78350=CARTESIAN_POINT('Ctrl Pts',(44.9903631386704,-2.23925218237269,2.31987660231025));
#78351=CARTESIAN_POINT('Ctrl Pts',(44.9965160028539,-2.31010886886649,2.24933300434687));
#78352=CARTESIAN_POINT('Ctrl Pts',(45.0026688670374,-2.37756421816483,2.17561622328072));
#78353=CARTESIAN_POINT('Ctrl Pts',(45.0088194002111,-2.44499401203456,2.10192736978378));
#78354=CARTESIAN_POINT('Ctrl Pts',(45.0149699333847,-2.50902473622744,2.02506804196943));
#78355=CARTESIAN_POINT('Ctrl Pts',(45.0211204665584,-2.5693532073192,1.94538984744409));
#78356=CARTESIAN_POINT('Ctrl Pts',(45.0272703148107,-2.62967496025157,1.8657205258572));
#78357=CARTESIAN_POINT('Ctrl Pts',(45.0334201630629,-2.68629501755139,1.78323330796266));
#78358=CARTESIAN_POINT('Ctrl Pts',(45.0395700113152,-2.73895146161718,1.69831164790362));
#78359=CARTESIAN_POINT('Ctrl Pts',(45.0457208197312,-2.79161612683074,1.61337672919166));
#78360=CARTESIAN_POINT('Ctrl Pts',(45.0518716281473,-2.84031572072484,1.52600698257051));
#78361=CARTESIAN_POINT('Ctrl Pts',(45.0580224365633,-2.88483304574274,1.43661263418177));
#78362=CARTESIAN_POINT('Ctrl Pts',(45.064179822966,-2.92939797984685,1.34712268294094));
#78363=CARTESIAN_POINT('Ctrl Pts',(45.0703372093687,-2.9697715194839,1.25560419581561));
#78364=CARTESIAN_POINT('Ctrl Pts',(45.0764945957713,-3.0057836894657,1.16248955893889));
#78365=CARTESIAN_POINT('Ctrl Pts',(45.0826554185446,-3.04181595744911,1.06932295579293));
#78366=CARTESIAN_POINT('Ctrl Pts',(45.0888162413179,-3.07348187076344,0.974558840888284));
#78367=CARTESIAN_POINT('Ctrl Pts',(45.0949770640911,-3.10066129822277,0.878645022863892));
#78368=CARTESIAN_POINT('Ctrl Pts',(45.1011481870434,-3.1278861665233,0.782570848092476));
#78369=CARTESIAN_POINT('Ctrl Pts',(45.1073193099957,-3.15060946728607,0.685343553900044));
#78370=CARTESIAN_POINT('Ctrl Pts',(45.113490432948,-3.16876213897789,0.587421542914688));
#78371=CARTESIAN_POINT('Ctrl Pts',(45.1181859545254,-3.18257425425655,0.512914047433577));
#78372=CARTESIAN_POINT('Ctrl Pts',(45.1228814761028,-3.19374127328364,0.43800456595355));
#78373=CARTESIAN_POINT('Ctrl Pts',(45.1275769976802,-3.202252974824,0.362895918592192));
#78374=CARTESIAN_POINT('Ctrl Pts',(45.135060182029,-3.2158179495982,0.243196361229775));
#78375=CARTESIAN_POINT('Ctrl Pts',(45.1425433663779,-3.22267319133973,0.122722239128668));
#78376=CARTESIAN_POINT('Ctrl Pts',(45.1500265507268,-3.22274935820264,0.00203388900681504));
#78377=CARTESIAN_POINT('Ctrl Pts',(45.1500283205554,-3.22644826576858,0.00200764693452582));
#78378=CARTESIAN_POINT('Ctrl Pts',(45.2088269525103,-3.21944509740503,-0.947386556412211));
#78379=CARTESIAN_POINT('Ctrl Pts',(45.3339079907115,-2.27377397144541,-2.97911589626085));
#78380=CARTESIAN_POINT('Ctrl Pts',(45.5252714351595,1.18232080972543,-3.62362621122949));
#78381=CARTESIAN_POINT('Ctrl Pts',(45.724118653899,3.68751965146775,-0.964753018247734));
#78382=CARTESIAN_POINT('Ctrl Pts',(45.8725610992789,3.02903273905734,1.68169936845078));
#78383=CARTESIAN_POINT('Ctrl Pts',(45.9547211384122,2.00465334780378,2.53949398247757));
#78384=CARTESIAN_POINT('Ctrl Pts',(45.9705987712989,1.78932308991422,2.68012452748182));
#78385=CARTESIAN_POINT('Origin',(-1.72497344927317,0.,0.));
#78386=CARTESIAN_POINT('',(47.4668462457454,1.78943621037804,2.68030513402633));
#78387=CARTESIAN_POINT('',(47.2204000228944,1.78943621037803,2.68030513402633));
#78388=CARTESIAN_POINT('',(-1.72497344927317,1.78943621037804,2.68030513402633));
#78389=CARTESIAN_POINT('',(46.64657344933,-3.22274878923343,-0.00279356304438793));
#78390=CARTESIAN_POINT('Ctrl Pts',(46.64657344933,-3.22274878923343,-0.00279356304438944));
#78391=CARTESIAN_POINT('Ctrl Pts',(46.6539949073187,-3.22264437215106,-0.123252640009857));
#78392=CARTESIAN_POINT('Ctrl Pts',(46.6614163653074,-3.21578244460685,-0.243415722663157));
#78393=CARTESIAN_POINT('Ctrl Pts',(46.668837823296,-3.20228492487645,-0.362613875091683));
#78394=CARTESIAN_POINT('Ctrl Pts',(46.6763621523232,-3.18860031200701,-0.483464268594949));
#78395=CARTESIAN_POINT('Ctrl Pts',(46.6838864813503,-3.16809494364444,-0.603322798527606));
#78396=CARTESIAN_POINT('Ctrl Pts',(46.6914108103774,-3.14094482293906,-0.721514505573045));
#78397=CARTESIAN_POINT('Ctrl Pts',(46.6962692590465,-3.123414028189,-0.797830724563636));
#78398=CARTESIAN_POINT('Ctrl Pts',(46.7011277077156,-3.10311384349577,-0.873452451264103));
#78399=CARTESIAN_POINT('Ctrl Pts',(46.7059861563847,-3.08010212327673,-0.948202759269441));
#78400=CARTESIAN_POINT('Ctrl Pts',(46.7121584215066,-3.05086759847718,-1.04316696500268));
#78401=CARTESIAN_POINT('Ctrl Pts',(46.7183306866286,-3.01718566831026,-1.13694503262286));
#78402=CARTESIAN_POINT('Ctrl Pts',(46.7245029517505,-2.97917036856004,-1.22908969469027));
#78403=CARTESIAN_POINT('Ctrl Pts',(46.7306668572702,-2.94120655603203,-1.32110955772356));
#78404=CARTESIAN_POINT('Ctrl Pts',(46.7368307627898,-2.89892120347925,-1.41150001429682));
#78405=CARTESIAN_POINT('Ctrl Pts',(46.7429946683095,-2.85247822575668,-1.49982850155744));
#78406=CARTESIAN_POINT('Ctrl Pts',(46.7491520466541,-2.80608442812754,-1.58806345469366));
#78407=CARTESIAN_POINT('Ctrl Pts',(46.7553094249986,-2.75554195926,-1.67424039715845));
#78408=CARTESIAN_POINT('Ctrl Pts',(46.7614668033431,-2.70106259151513,-1.75794722310358));
#78409=CARTESIAN_POINT('Ctrl Pts',(46.7676196838393,-2.64662301991724,-1.84159290279672));
#78410=CARTESIAN_POINT('Ctrl Pts',(46.7737725643356,-2.58825250331351,-1.92277169041361));
#78411=CARTESIAN_POINT('Ctrl Pts',(46.7799254448318,-2.5262080042061,-2.00109736944134));
#78412=CARTESIAN_POINT('Ctrl Pts',(46.7860759941076,-2.46418701269018,-2.07939337221908));
#78413=CARTESIAN_POINT('Ctrl Pts',(46.7922265433834,-2.3984950739998,-2.15483807422403));
#78414=CARTESIAN_POINT('Ctrl Pts',(46.7983770926592,-2.32943107527019,-2.22707620616483));
#78415=CARTESIAN_POINT('Ctrl Pts',(46.8045269567858,-2.26037477002374,-2.29930629103537));
#78416=CARTESIAN_POINT('Ctrl Pts',(46.8106768209123,-2.18794745172932,-2.36833020203992));
#78417=CARTESIAN_POINT('Ctrl Pts',(46.8168266850389,-2.11248601448805,-2.43382834256905));
#78418=CARTESIAN_POINT('Ctrl Pts',(46.822977509084,-2.0370127986402,-2.4993367065561));
#78419=CARTESIAN_POINT('Ctrl Pts',(46.829128333129,-1.95850485124619,-2.56131792221652));
#78420=CARTESIAN_POINT('Ctrl Pts',(46.8352791571741,-1.87733261314578,-2.61949228327156));
#78421=CARTESIAN_POINT('Ctrl Pts',(46.8414365587323,-1.7960735718044,-2.67772885430379));
#78422=CARTESIAN_POINT('Ctrl Pts',(46.8475939602905,-1.71214490411932,-2.73215018795683));
#78423=CARTESIAN_POINT('Ctrl Pts',(46.8537513618487,-1.62594644257923,-2.78251967259244));
#78424=CARTESIAN_POINT('Ctrl Pts',(46.8599121995386,-1.53969987807459,-2.83291726586816));
#78425=CARTESIAN_POINT('Ctrl Pts',(46.8660730372286,-1.45118138202589,-2.87925830564476));
#78426=CARTESIAN_POINT('Ctrl Pts',(46.8722338749185,-1.36081394415636,-2.92135293518082));
#78427=CARTESIAN_POINT('Ctrl Pts',(46.8784050122434,-1.27029543078865,-2.96351793815314));
#78428=CARTESIAN_POINT('Ctrl Pts',(46.8845761495683,-1.1779222033766,-3.00142218565318));
#78429=CARTESIAN_POINT('Ctrl Pts',(46.8907472868932,-1.08413583688106,-3.03492455420068));
#78430=CARTESIAN_POINT('Ctrl Pts',(46.8954426496369,-1.01277767582838,-3.06041511855229));
#78431=CARTESIAN_POINT('Ctrl Pts',(46.9001380123805,-0.940601824703771,
-3.08335842016347));
#78432=CARTESIAN_POINT('Ctrl Pts',(46.9048333751242,-0.86780687241381,-3.10371209919531));
#78433=CARTESIAN_POINT('Ctrl Pts',(46.911005680367,-0.772114017528194,-3.130468097966));
#78434=CARTESIAN_POINT('Ctrl Pts',(46.9171779856098,-0.675014195943398,
-3.15284147084316));
#78435=CARTESIAN_POINT('Ctrl Pts',(46.9233502908525,-0.57694532063497,-3.17068630733118));
#78436=CARTESIAN_POINT('Ctrl Pts',(46.9295142370435,-0.479009258395676,
-3.18850697684986));
#78437=CARTESIAN_POINT('Ctrl Pts',(46.9356781832346,-0.38010717450795,-3.20181122276752));
#78438=CARTESIAN_POINT('Ctrl Pts',(46.9418421294256,-0.280691581725667,
-3.21050304445399));
#78439=CARTESIAN_POINT('Ctrl Pts',(46.9479995489326,-0.181381254976336,
-3.21918566281971));
#78440=CARTESIAN_POINT('Ctrl Pts',(46.9541569684395,-0.0815589306455282,
-3.22326552890595));
#78441=CARTESIAN_POINT('Ctrl Pts',(46.9603143879465,0.0183142107331389,
-3.22269796167516));
#78442=CARTESIAN_POINT('Ctrl Pts',(46.9664673101688,0.118114406301845,-3.22213080898676));
#78443=CARTESIAN_POINT('Ctrl Pts',(46.9726202323911,0.217964912075569,-3.21692297412134));
#78444=CARTESIAN_POINT('Ctrl Pts',(46.9787731546133,0.31740189162692,-3.20708178905554));
#78445=CARTESIAN_POINT('Ctrl Pts',(46.9849237459473,0.416801201843157,-3.19724433208867));
#78446=CARTESIAN_POINT('Ctrl Pts',(46.9910743372813,0.515786865334471,-3.18277705529739));
#78447=CARTESIAN_POINT('Ctrl Pts',(46.9972249286153,0.613898410160742,-3.16373929148755));
#78448=CARTESIAN_POINT('Ctrl Pts',(47.003374835081,0.711999030267057,-3.14470364753259));
#78449=CARTESIAN_POINT('Ctrl Pts',(47.0095247415466,0.809225298807935,-3.12109861111653));
#78450=CARTESIAN_POINT('Ctrl Pts',(47.0156746480123,0.905126201654985,-3.0930347753586));
#78451=CARTESIAN_POINT('Ctrl Pts',(47.0218255146265,1.00104207694248,-3.06496655816007));
#78452=CARTESIAN_POINT('Ctrl Pts',(47.0279763812407,1.09563175861427,-3.03243828093851));
#78453=CARTESIAN_POINT('Ctrl Pts',(47.0341272478549,1.18845964986827,-2.99561032564901));
#78454=CARTESIAN_POINT('Ctrl Pts',(47.0402846920712,1.28138680923835,-2.95874298734984));
#78455=CARTESIAN_POINT('Ctrl Pts',(47.0464421362876,1.37254801145771,-2.91756694978181));
#78456=CARTESIAN_POINT('Ctrl Pts',(47.052599580504,1.46152801916254,-2.87229062103799));
#78457=CARTESIAN_POINT('Ctrl Pts',(47.0587604609681,1.55055768340403,-2.82698902520625));
#78458=CARTESIAN_POINT('Ctrl Pts',(47.0649213414323,1.63740335144169,-2.77758279601963));
#78459=CARTESIAN_POINT('Ctrl Pts',(47.0710822218965,1.72167659529636,-2.72432510242605));
#78460=CARTESIAN_POINT('Ctrl Pts',(47.0772534017357,1.80609072189543,-2.67097837594742));
#78461=CARTESIAN_POINT('Ctrl Pts',(47.0834245815749,1.88792347819824,-2.61376757307797));
#78462=CARTESIAN_POINT('Ctrl Pts',(47.0895957614142,1.96681738192434,-2.55298784733894));
#78463=CARTESIAN_POINT('Ctrl Pts',(47.0942907055641,2.02683872004956,-2.506747513201));
#78464=CARTESIAN_POINT('Ctrl Pts',(47.098985649714,2.08515970847106,-2.45844237546095));
#78465=CARTESIAN_POINT('Ctrl Pts',(47.1036805938639,2.14163737351416,-2.40821654401496));
#78466=CARTESIAN_POINT('Ctrl Pts',(47.1098526614097,2.2158840423445,-2.34218866075789));
#78467=CARTESIAN_POINT('Ctrl Pts',(47.1160247289555,2.28720506002567,-2.272607706105));
#78468=CARTESIAN_POINT('Ctrl Pts',(47.1221967965013,2.35524091165208,-2.19976312601614));
#78469=CARTESIAN_POINT('Ctrl Pts',(47.1283605043972,2.42318461329789,-2.12701720900684));
#78470=CARTESIAN_POINT('Ctrl Pts',(47.134524212293,2.48785169891878,-2.05101676717502));
#78471=CARTESIAN_POINT('Ctrl Pts',(47.1406879201888,2.54891674199184,-1.97209051640479));
#78472=CARTESIAN_POINT('Ctrl Pts',(47.1468451011119,2.60991712108668,-1.89324784349029));
#78473=CARTESIAN_POINT('Ctrl Pts',(47.153002282035,2.66732277651969,-1.81148586291148));
#78474=CARTESIAN_POINT('Ctrl Pts',(47.1591594629581,2.72084676406627,-1.7271683325519));
#78475=CARTESIAN_POINT('Ctrl Pts',(47.1653121471282,2.77433166162168,-1.64291238152653));
#78476=CARTESIAN_POINT('Ctrl Pts',(47.1714648312984,2.82394029540775,-1.55610495705118));
#78477=CARTESIAN_POINT('Ctrl Pts',(47.1776175154685,2.86942803792344,-1.4671401765608));
#78478=CARTESIAN_POINT('Ctrl Pts',(47.1837678691481,2.91489855076353,-1.37820909381452));
#78479=CARTESIAN_POINT('Ctrl Pts',(47.1899182228278,2.95625107627835,-1.28712266508161));
#78480=CARTESIAN_POINT('Ctrl Pts',(47.1960685765074,2.9932865491922,-1.19430029595786));
#78481=CARTESIAN_POINT('Ctrl Pts',(47.2022182459899,3.03031790208839,-1.1014882528748));
#78482=CARTESIAN_POINT('Ctrl Pts',(47.2083679154724,3.06303299620828,-1.00694105681462));
#78483=CARTESIAN_POINT('Ctrl Pts',(47.2145175849548,3.09128100061009,-0.911097874965736));
#78484=CARTESIAN_POINT('Ctrl Pts',(47.2206682155309,3.11953341971699,-0.815239714381489));
#78485=CARTESIAN_POINT('Ctrl Pts',(47.226818846107,3.14331723961166,-0.718085582430075));
#78486=CARTESIAN_POINT('Ctrl Pts',(47.2329694766831,3.16253184843985,-0.620088598591862));
#78487=CARTESIAN_POINT('Ctrl Pts',(47.239126687776,3.18176701484419,-0.521986768463238));
#78488=CARTESIAN_POINT('Ctrl Pts',(47.2452838988689,3.19642312447634,-0.423040712841666));
#78489=CARTESIAN_POINT('Ctrl Pts',(47.2514411099618,3.20645097407994,-0.323712392907326));
#78490=CARTESIAN_POINT('Ctrl Pts',(47.2576017585541,3.21648442211546,-0.224328619126176));
#78491=CARTESIAN_POINT('Ctrl Pts',(47.2637624071464,3.22188444084847,-0.124562589804339));
#78492=CARTESIAN_POINT('Ctrl Pts',(47.2699230557388,3.22265397643253,-0.0248779155799095));
#78493=CARTESIAN_POINT('Ctrl Pts',(47.2760940081682,3.22342479908389,0.0749734837283165));
#78494=CARTESIAN_POINT('Ctrl Pts',(47.2822649605977,3.21954968586724,0.174742821869841));
#78495=CARTESIAN_POINT('Ctrl Pts',(47.2884359130272,3.21108363338839,0.273969819296283));
#78496=CARTESIAN_POINT('Ctrl Pts',(47.293133212886,3.20463931420627,0.349500941327117));
#78497=CARTESIAN_POINT('Ctrl Pts',(47.2978305127448,3.19553599947028,0.424717890956712));
#78498=CARTESIAN_POINT('Ctrl Pts',(47.3025278126036,3.18381768600742,0.499422170879856));
#78499=CARTESIAN_POINT('Ctrl Pts',(47.3087009908281,3.16841751150901,0.597598324832455));
#78500=CARTESIAN_POINT('Ctrl Pts',(47.3148741690525,3.14844493899141,0.695234285421411));
#78501=CARTESIAN_POINT('Ctrl Pts',(47.321047347277,3.12394910720187,0.791870910005332));
#78502=CARTESIAN_POINT('Ctrl Pts',(47.3272102069154,3.09949422066611,0.888346004613346));
#78503=CARTESIAN_POINT('Ctrl Pts',(47.3333730665538,3.07053122456943,0.983824669490771));
#78504=CARTESIAN_POINT('Ctrl Pts',(47.3395359261922,3.03716064498571,1.07785563924396));
#78505=CARTESIAN_POINT('Ctrl Pts',(47.3456928862413,3.0038220104287,1.17179659492251));
#78506=CARTESIAN_POINT('Ctrl Pts',(47.3518498462903,2.96608431985286,1.2642922021938));
#78507=CARTESIAN_POINT('Ctrl Pts',(47.3580068063394,2.92409839401049,1.35490447805196));
#78508=CARTESIAN_POINT('Ctrl Pts',(47.3641595193605,2.88214142976529,1.44545425019778));
#78509=CARTESIAN_POINT('Ctrl Pts',(47.3703122323817,2.83594223626957,1.53412288007275));
#78510=CARTESIAN_POINT('Ctrl Pts',(47.3764649454029,2.78570006155276,1.6204915086371));
#78511=CARTESIAN_POINT('Ctrl Pts',(47.3826150599722,2.73547910542274,1.70682366146664));
#78512=CARTESIAN_POINT('Ctrl Pts',(47.3887651745415,2.68121878132588,1.79085736956817));
#78513=CARTESIAN_POINT('Ctrl Pts',(47.3949152891108,2.62316420412631,1.87219847256919));
#78514=CARTESIAN_POINT('Ctrl Pts',(47.4010666547556,2.56509781728333,1.95355612223142));
#78515=CARTESIAN_POINT('Ctrl Pts',(47.4072180204003,2.50323587876763,2.03221971234551));
#78516=CARTESIAN_POINT('Ctrl Pts',(47.4133693860451,2.43786647152331,2.10782462020029));
#78517=CARTESIAN_POINT('Ctrl Pts',(47.4195211257958,2.3724930887261,2.18343412609752));
#78518=CARTESIAN_POINT('Ctrl Pts',(47.4256728655465,2.30361210310448,2.25598425601033));
#78519=CARTESIAN_POINT('Ctrl Pts',(47.4318246052971,2.2315504287417,2.32514520976276));
#78520=CARTESIAN_POINT('Ctrl Pts',(47.4379822105324,2.15942004590611,2.39437210624486));
#78521=CARTESIAN_POINT('Ctrl Pts',(47.4441398157677,2.08410323496244,2.46020307499644));
#78522=CARTESIAN_POINT('Ctrl Pts',(47.450297421003,2.00596203592081,2.52234689782045));
#78523=CARTESIAN_POINT('Ctrl Pts',(47.4558136959171,1.93595944245132,2.57801828268711));
#78524=CARTESIAN_POINT('Ctrl Pts',(47.4613299708313,1.86369079257126,2.63073098797996));
#78525=CARTESIAN_POINT('Ctrl Pts',(47.4668462457454,1.78943621037804,2.68030513402633));
#78526=CARTESIAN_POINT('Ctrl Pts',(46.216937227185,1.78943621037807,2.68030513402631));
#78527=CARTESIAN_POINT('Ctrl Pts',(46.2230877404723,1.70631878588743,2.73579632687922));
#78528=CARTESIAN_POINT('Ctrl Pts',(46.2292382537596,1.62062966051722,2.78740969530876));
#78529=CARTESIAN_POINT('Ctrl Pts',(46.2353887670468,1.53277076357632,2.8349129349639));
#78530=CARTESIAN_POINT('Ctrl Pts',(46.2415456899858,1.4448203059963,2.88246567930366));
#78531=CARTESIAN_POINT('Ctrl Pts',(46.2477026129248,1.35469594328053,2.92589953232438));
#78532=CARTESIAN_POINT('Ctrl Pts',(46.2538595358637,1.26282357950996,2.96502852760874));
#78533=CARTESIAN_POINT('Ctrl Pts',(46.2600196269283,1.17090394160692,3.00417765723199));
#78534=CARTESIAN_POINT('Ctrl Pts',(46.2661797179928,1.07723491838889,3.03901736522023));
#78535=CARTESIAN_POINT('Ctrl Pts',(46.2723398090574,0.982259737026324,3.06941091604187));
#78536=CARTESIAN_POINT('Ctrl Pts',(46.2785105450889,0.887120433469441,3.09985698854531));
#78537=CARTESIAN_POINT('Ctrl Pts',(46.2846812811204,0.79067088188869,3.12584143853654));
#78538=CARTESIAN_POINT('Ctrl Pts',(46.2908520171519,0.693366991542634,3.14727815382421));
#78539=CARTESIAN_POINT('Ctrl Pts',(46.2966652510697,0.601700410310481,3.16747293119929));
#78540=CARTESIAN_POINT('Ctrl Pts',(46.3024784849875,0.50927600227785,3.18363207842856));
#78541=CARTESIAN_POINT('Ctrl Pts',(46.3082917189053,0.416478177357678,3.19572581588046));
#78542=CARTESIAN_POINT('Ctrl Pts',(46.3144639766131,0.317949183302638,3.20856645936026));
#78543=CARTESIAN_POINT('Ctrl Pts',(46.3206362343209,0.218652370678122,3.21686874010675));
#78544=CARTESIAN_POINT('Ctrl Pts',(46.3268084920286,0.119041973504201,3.22055066270416));
#78545=CARTESIAN_POINT('Ctrl Pts',(46.3329723903487,0.0195664835174384,
3.22422759869541));
#78546=CARTESIAN_POINT('Ctrl Pts',(46.3391362886688,-0.0802213166197347,
3.2232965982539));
#78547=CARTESIAN_POINT('Ctrl Pts',(46.3453001869889,-0.179859856710437,
3.21772714729576));
#78548=CARTESIAN_POINT('Ctrl Pts',(46.3514575583544,-0.279392889507493,
3.21216359383167));
#78549=CARTESIAN_POINT('Ctrl Pts',(46.3576149297198,-0.3787765451741,3.20197137879874));
#78550=CARTESIAN_POINT('Ctrl Pts',(46.3637723010853,-0.477547989810642,
3.18717201919316));
#78551=CARTESIAN_POINT('Ctrl Pts',(46.3699251749581,-0.576247289400351,
3.172383469397));
#78552=CARTESIAN_POINT('Ctrl Pts',(46.376078048831,-0.674334838734504,3.15299452973312));
#78553=CARTESIAN_POINT('Ctrl Pts',(46.3822309227038,-0.771352589650201,
3.12907857762312));
#78554=CARTESIAN_POINT('Ctrl Pts',(46.3883814655759,-0.868333585635746,
3.10517168601124));
#78555=CARTESIAN_POINT('Ctrl Pts',(46.394532008448,-0.964245167232633,3.07674129359341));
#78556=CARTESIAN_POINT('Ctrl Pts',(46.4006825513201,-1.05864002926922,3.04391176792772));
#78557=CARTESIAN_POINT('Ctrl Pts',(46.4068324092684,-1.15302437950546,3.01108589815402));
#78558=CARTESIAN_POINT('Ctrl Pts',(46.4129822672168,-1.245891935713,2.97386201178683));
#78559=CARTESIAN_POINT('Ctrl Pts',(46.4191321251652,-1.33681206134223,2.93241386491572));
#78560=CARTESIAN_POINT('Ctrl Pts',(46.4252829432638,-1.42774638192961,2.89095924692827));
#78561=CARTESIAN_POINT('Ctrl Pts',(46.4314337613623,-1.51673227275081,2.84527923866662));
#78562=CARTESIAN_POINT('Ctrl Pts',(46.4375845794609,-1.60336145485579,2.79559467870125));
#78563=CARTESIAN_POINT('Ctrl Pts',(46.4437419754652,-1.69008328131795,2.74585698428386));
#78564=CARTESIAN_POINT('Ctrl Pts',(46.4498993714694,-1.77444298865255,2.69210640275822));
#78565=CARTESIAN_POINT('Ctrl Pts',(46.4560567674737,-1.85605929590869,2.63460840592505));
#78566=CARTESIAN_POINT('Ctrl Pts',(46.4622175998187,-1.93772115187402,2.57707832041226));
#78567=CARTESIAN_POINT('Ctrl Pts',(46.4683784321636,-2.01663621561404,2.5157969210819));
#78568=CARTESIAN_POINT('Ctrl Pts',(46.4745392645086,-2.09245612288099,2.45107016144334));
#78569=CARTESIAN_POINT('Ctrl Pts',(46.4807103968838,-2.168402790185,2.3862351879234));
#78570=CARTESIAN_POINT('Ctrl Pts',(46.486881529259,-2.24124364776206,2.31794364560584));
#78571=CARTESIAN_POINT('Ctrl Pts',(46.4930526616342,-2.31066694634494,2.2465386321114));
#78572=CARTESIAN_POINT('Ctrl Pts',(46.4977480869711,-2.36348900481347,2.19220874755187));
#78573=CARTESIAN_POINT('Ctrl Pts',(46.502443512308,-2.41433332229022,2.13607717478546));
#78574=CARTESIAN_POINT('Ctrl Pts',(46.507138937645,-2.4630788926605,2.07830698671547));
#78575=CARTESIAN_POINT('Ctrl Pts',(46.5132722927928,-2.52675233510899,2.0028452223465));
#78576=CARTESIAN_POINT('Ctrl Pts',(46.5194056479406,-2.58707524734235,1.9243115331488));
#78577=CARTESIAN_POINT('Ctrl Pts',(46.5255390030883,-2.64373401534343,1.84303771491961));
#78578=CARTESIAN_POINT('Ctrl Pts',(46.5316645122836,-2.70032030392768,1.76186786434022));
#78579=CARTESIAN_POINT('Ctrl Pts',(46.5377900214788,-2.75325150827311,1.67796520329826));
#78580=CARTESIAN_POINT('Ctrl Pts',(46.5439155306741,-2.80225295442358,1.59169593262165));
#78581=CARTESIAN_POINT('Ctrl Pts',(46.550034892833,-2.85120522692009,1.50551323439539));
#78582=CARTESIAN_POINT('Ctrl Pts',(46.556154254992,-2.89623535952982,1.41696902467224));
#78583=CARTESIAN_POINT('Ctrl Pts',(46.5622736171509,-2.93711149370048,1.32645905932771));
#78584=CARTESIAN_POINT('Ctrl Pts',(46.5683885251004,-2.97795787462922,1.23601497508836));
#78585=CARTESIAN_POINT('Ctrl Pts',(46.5745034330499,-3.01465608571694,1.14360837851562));
#78586=CARTESIAN_POINT('Ctrl Pts',(46.5806183409994,-3.04702033759801,1.04965928984794));
#78587=CARTESIAN_POINT('Ctrl Pts',(46.5867314730216,-3.07937519006426,0.955737486422634));
#78588=CARTESIAN_POINT('Ctrl Pts',(46.5928446050439,-3.10739843466665,0.86027449432106));
#78589=CARTESIAN_POINT('Ctrl Pts',(46.5989577370661,-3.13095287065684,0.76370916206741));
#78590=CARTESIAN_POINT('Ctrl Pts',(46.6050697410841,-3.15450296034705,0.667161648194215));
#78591=CARTESIAN_POINT('Ctrl Pts',(46.611181745102,-3.17358578126501,0.569512627248587));
#78592=CARTESIAN_POINT('Ctrl Pts',(46.6172937491199,-3.18811468945743,0.47121363452872));
#78593=CARTESIAN_POINT('Ctrl Pts',(46.623408458521,-3.20265002864429,0.372871131294042));
#78594=CARTESIAN_POINT('Ctrl Pts',(46.6295231679221,-3.21262736756129,0.273878517798201));
#78595=CARTESIAN_POINT('Ctrl Pts',(46.6356378773232,-3.21801172049166,0.17469438822795));
#78596=CARTESIAN_POINT('Ctrl Pts',(46.6392830679732,-3.22122152028264,0.115567283730771));
#78597=CARTESIAN_POINT('Ctrl Pts',(46.6429282586231,-3.22280007565892,0.0563722112005146));
#78598=CARTESIAN_POINT('Ctrl Pts',(46.646573449273,-3.22274878923423,-0.00279356211900748));
#78599=CARTESIAN_POINT('',(46.4000265227372,-3.22266022380361,0.00169756151001587));
#78600=CARTESIAN_POINT('Ctrl Pts',(45.9705987712989,1.78932308991422,2.68012452748182));
#78601=CARTESIAN_POINT('Ctrl Pts',(46.0210035446588,1.10574053552164,3.12656706705717));
#78602=CARTESIAN_POINT('Ctrl Pts',(46.1376907242651,-0.881920472688252,
3.57354541826147));
#78603=CARTESIAN_POINT('Ctrl Pts',(46.2808328527696,-2.93975493458649,1.93617029787196));
#78604=CARTESIAN_POINT('Ctrl Pts',(46.3735702079145,-3.22033984576282,0.431640650872118));
#78605=CARTESIAN_POINT('Ctrl Pts',(46.4000251568126,-3.21830085460638,0.00171746357588361));
#78606=CARTESIAN_POINT('Ctrl Pts',(46.4000265507268,-3.22274955312531,0.00169715368999332));
#78607=CARTESIAN_POINT('Ctrl Pts',(46.4062581732079,-3.22280295769783,-0.0997135572294896));
#78608=CARTESIAN_POINT('Ctrl Pts',(46.4124897956889,-3.21806535961105,-0.201121896896725));
#78609=CARTESIAN_POINT('Ctrl Pts',(46.41872141817,-3.20856390007265,-0.302051753265169));
#78610=CARTESIAN_POINT('Ctrl Pts',(46.4249548901296,-3.19905962060328,-0.403011564529283));
#78611=CARTESIAN_POINT('Ctrl Pts',(46.4311883620892,-3.18478870581297,-0.503492193516223));
#78612=CARTESIAN_POINT('Ctrl Pts',(46.4374218340487,-3.16583008376198,-0.603023584321204));
#78613=CARTESIAN_POINT('Ctrl Pts',(46.4436586485661,-3.14686129558034,-0.70260834657482));
#78614=CARTESIAN_POINT('Ctrl Pts',(46.4498954630835,-3.12319987712051,-0.801242447405722));
#78615=CARTESIAN_POINT('Ctrl Pts',(46.4561322776009,-3.09497549546286,-0.89846772061352));
#78616=CARTESIAN_POINT('Ctrl Pts',(46.4623782356076,-3.0667097354172,-0.995835531047709));
#78617=CARTESIAN_POINT('Ctrl Pts',(46.4686241936143,-3.03386777351972,-1.09178998832456));
#78618=CARTESIAN_POINT('Ctrl Pts',(46.474870151621,-2.99662868287034,-1.18588958149517));
#78619=CARTESIAN_POINT('Ctrl Pts',(46.4811213541571,-2.95935832375774,-1.28006818705883));
#78620=CARTESIAN_POINT('Ctrl Pts',(46.4873725566932,-2.91768365327421,-1.37238844584609));
#78621=CARTESIAN_POINT('Ctrl Pts',(46.4936237592294,-2.87183040081695,-1.46243212199527));
#78622=CARTESIAN_POINT('Ctrl Pts',(46.4998860894401,-2.82589552565277,-1.552636083581));
#78623=CARTESIAN_POINT('Ctrl Pts',(46.5061484196508,-2.77576742312358,-1.64055500839909));
#78624=CARTESIAN_POINT('Ctrl Pts',(46.5124107498616,-2.72171601364334,-1.72579822215037));
#78625=CARTESIAN_POINT('Ctrl Pts',(46.5147763428602,-2.70129811303246,-1.75799881567537));
#78626=CARTESIAN_POINT('Ctrl Pts',(46.5171419358589,-2.68032079515301,-1.78981792885236));
#78627=CARTESIAN_POINT('Ctrl Pts',(46.5195075288576,-2.65880008360341,-1.82123575572481));
#78628=CARTESIAN_POINT('Ctrl Pts',(46.5256797784124,-2.60264874972824,-1.90321040987512));
#78629=CARTESIAN_POINT('Ctrl Pts',(46.5318520279673,-2.54260393550251,-1.98273007495402));
#78630=CARTESIAN_POINT('Ctrl Pts',(46.5380242775221,-2.47890752031201,-2.05940162868746));
#78631=CARTESIAN_POINT('Ctrl Pts',(46.544188167611,-2.41529737318388,-2.13596934131211));
#78632=CARTESIAN_POINT('Ctrl Pts',(46.5503520577,-2.3480457301317,-2.20969627837632));
#78633=CARTESIAN_POINT('Ctrl Pts',(46.5565159477889,-2.27743772054739,-2.28021818945642));
#78634=CARTESIAN_POINT('Ctrl Pts',(46.5626733108566,-2.20690447867853,-2.35066542399187));
#78635=CARTESIAN_POINT('Ctrl Pts',(46.5688306739243,-2.13302224180427,-2.41791407455335));
#78636=CARTESIAN_POINT('Ctrl Pts',(46.574988036992,-2.05611574860215,-2.48163365363428));
#78637=CARTESIAN_POINT('Ctrl Pts',(46.5811409025014,-1.97926543065437,-2.54530668965477));
#78638=CARTESIAN_POINT('Ctrl Pts',(46.5872937680108,-1.89939558177457,-2.60545550292683));
#78639=CARTESIAN_POINT('Ctrl Pts',(46.5934466335201,-1.81686638781891,-2.66178776225939));
#78640=CARTESIAN_POINT('Ctrl Pts',(46.5995971679912,-1.73436846038723,-2.71809867988421));
#78641=CARTESIAN_POINT('Ctrl Pts',(46.6057477024622,-1.64921354815239,-2.77059567198646));
#78642=CARTESIAN_POINT('Ctrl Pts',(46.6118982369332,-1.56179266225975,-2.81902842174598));
#78643=CARTESIAN_POINT('Ctrl Pts',(46.618048086453,-1.4743815119514,-2.86745577781595));
#78644=CARTESIAN_POINT('Ctrl Pts',(46.6241979359727,-1.38470526965231,-2.91181958089788));
#78645=CARTESIAN_POINT('Ctrl Pts',(46.6303477854925,-1.29318062611911,-2.95191487525135));
#78646=CARTESIAN_POINT('Ctrl Pts',(46.6364985951448,-1.20164169348925,-2.99201642940016));
#78647=CARTESIAN_POINT('Ctrl Pts',(46.6426494047972,-1.10825418434345,-3.02784797683744));
#78648=CARTESIAN_POINT('Ctrl Pts',(46.6488002144496,-1.01345495636064,-3.05925262342423));
#78649=CARTESIAN_POINT('Ctrl Pts',(46.654957602033,-0.918554346149848,-3.09069085544318));
#78650=CARTESIAN_POINT('Ctrl Pts',(46.6611149896164,-0.822239415427962,
-3.11769259581678));
#78651=CARTESIAN_POINT('Ctrl Pts',(46.6672723771998,-0.724962268816142,
-3.14015083575502));
#78652=CARTESIAN_POINT('Ctrl Pts',(46.6734332011249,-0.627630833351503,
-3.16262160928543));
#78653=CARTESIAN_POINT('Ctrl Pts',(46.6795940250499,-0.529336539917454,
-3.18054375473742));
#78654=CARTESIAN_POINT('Ctrl Pts',(46.685754848975,-0.430539699163005,-3.19386178942431));
#78655=CARTESIAN_POINT('Ctrl Pts',(46.69192597302,-0.331577682561036,-3.20720209018418));
#78656=CARTESIAN_POINT('Ctrl Pts',(46.698097097065,-0.232111873290175,-3.21592286671934));
#78657=CARTESIAN_POINT('Ctrl Pts',(46.70426822111,-0.13260583457467,-3.22002069172494));
#78658=CARTESIAN_POINT('Ctrl Pts',(46.7089637299391,-0.0568932934027771,
-3.2231386607292));
#78659=CARTESIAN_POINT('Ctrl Pts',(46.7136592387682,0.0188424719052745,
-3.22358127729843));
#78660=CARTESIAN_POINT('Ctrl Pts',(46.7183547475973,0.0943992403508688,
-3.221367154784));
#78661=CARTESIAN_POINT('Ctrl Pts',(46.7245270053207,0.193718795391608,-3.21845668537852));
#78662=CARTESIAN_POINT('Ctrl Pts',(46.7306992630441,0.293078432466108,-3.21094353465639));
#78663=CARTESIAN_POINT('Ctrl Pts',(46.7368715207675,0.392016665811267,-3.19881860945978));
#78664=CARTESIAN_POINT('Ctrl Pts',(46.7430354191033,0.490820902314827,-3.18671010563665));
#78665=CARTESIAN_POINT('Ctrl Pts',(46.7491993174392,0.58920444212071,-3.17000229422451));
#78666=CARTESIAN_POINT('Ctrl Pts',(46.755363215775,0.686706701132125,-3.14873807566146));
#78667=CARTESIAN_POINT('Ctrl Pts',(46.7615205871563,0.784105714960766,-3.12749637378833));
#78668=CARTESIAN_POINT('Ctrl Pts',(46.7676779585376,0.880624881204119,-3.10170794893263));
#78669=CARTESIAN_POINT('Ctrl Pts',(46.7738353299189,0.975810600396833,-3.07146727715813));
#78670=CARTESIAN_POINT('Ctrl Pts',(46.7799882038075,1.070926793643,-3.04124869390014));
#78671=CARTESIAN_POINT('Ctrl Pts',(46.7861410776961,1.16471106354602,-3.0065844604398));
#78672=CARTESIAN_POINT('Ctrl Pts',(46.7922939515848,1.25672274150975,-2.96761950281235));
#78673=CARTESIAN_POINT('Ctrl Pts',(46.7984444944727,1.3486995610814,-2.9286693069608));
#78674=CARTESIAN_POINT('Ctrl Pts',(46.8045950373605,1.43890472352187,-2.88542179358704));
#78675=CARTESIAN_POINT('Ctrl Pts',(46.8107455802484,1.52691623562123,-2.83807053680776));
#78676=CARTESIAN_POINT('Ctrl Pts',(46.8168954382126,1.61491794676929,-2.79072455305869));
#78677=CARTESIAN_POINT('Ctrl Pts',(46.8230452961768,1.7007261107242,-2.73927594027524));
#78678=CARTESIAN_POINT('Ctrl Pts',(46.829195154141,1.78394300724425,-2.68396440166489));
#78679=CARTESIAN_POINT('Ctrl Pts',(46.8353459722553,1.86717289605075,-2.62864422750834));
#78680=CARTESIAN_POINT('Ctrl Pts',(46.8414967903696,1.94781035206711,-2.56946017007818));
#78681=CARTESIAN_POINT('Ctrl Pts',(46.8476476084839,2.02548718047142,-2.50669488455335));
#78682=CARTESIAN_POINT('Ctrl Pts',(46.8538050045038,2.10324707926237,-2.44386247558073));
#78683=CARTESIAN_POINT('Ctrl Pts',(46.8599624005237,2.17803968934412,-2.37744146414566));
#78684=CARTESIAN_POINT('Ctrl Pts',(46.8661197965435,2.24953053573908,-2.30775430479015));
#78685=CARTESIAN_POINT('Ctrl Pts',(46.8722806289041,2.32106127999047,-2.23802825418604));
#78686=CARTESIAN_POINT('Ctrl Pts',(46.8784414612646,2.38928629431012,-2.16503274296757));
#78687=CARTESIAN_POINT('Ctrl Pts',(46.8846022936251,2.4539100108565,-2.089124989348));
#78688=CARTESIAN_POINT('Ctrl Pts',(46.8907734260156,2.51864176900815,-2.01309032882811));
#78689=CARTESIAN_POINT('Ctrl Pts',(46.8969445584061,2.57975993690463,-1.93413404417319));
#78690=CARTESIAN_POINT('Ctrl Pts',(46.9031156907966,2.63701097745493,-1.85264423656627));
#78691=CARTESIAN_POINT('Ctrl Pts',(46.9078111159767,2.68057153658342,-1.79064114372271));
#78692=CARTESIAN_POINT('Ctrl Pts',(46.9125065411568,2.72189420194264,-1.72717197777526));
#78693=CARTESIAN_POINT('Ctrl Pts',(46.9172019663369,2.76088529323415,-1.66241690321753));
#78694=CARTESIAN_POINT('Ctrl Pts',(46.9233741891572,2.81213980038256,-1.57729516586987));
#78695=CARTESIAN_POINT('Ctrl Pts',(46.9295464119775,2.85954421333119,-1.48965101133111));
#78696=CARTESIAN_POINT('Ctrl Pts',(46.9357186347978,2.90284135274562,-1.39986772349746));
#78697=CARTESIAN_POINT('Ctrl Pts',(46.9418824981635,2.94607985194526,-1.31020603518182));
#78698=CARTESIAN_POINT('Ctrl Pts',(46.9480463615292,2.98522194717725,-1.21841135983221));
#78699=CARTESIAN_POINT('Ctrl Pts',(46.9542102248949,3.02005468392615,-1.124894336636));
#78700=CARTESIAN_POINT('Ctrl Pts',(46.9603675612842,3.05485053594266,-1.03147633954845));
#78701=CARTESIAN_POINT('Ctrl Pts',(46.9665248976735,3.08534595080881,-0.936340025336802));
#78702=CARTESIAN_POINT('Ctrl Pts',(46.9726822340628,3.11137513641882,-0.839918045391802));
#78703=CARTESIAN_POINT('Ctrl Pts',(46.9788350730678,3.13738531003366,-0.74356649309076));
#78704=CARTESIAN_POINT('Ctrl Pts',(46.9849879120728,3.15893562729801,-0.645931560178757));
#78705=CARTESIAN_POINT('Ctrl Pts',(46.9911407510778,3.17590972684832,-0.547462299533217));
#78706=CARTESIAN_POINT('Ctrl Pts',(46.9972912591591,3.19287739597967,-0.449030342698692));
#78707=CARTESIAN_POINT('Ctrl Pts',(47.0034417672403,3.20527221842371,-0.349765113758991));
#78708=CARTESIAN_POINT('Ctrl Pts',(47.0095922753215,3.21302885395988,-0.250126260359202));
#78709=CARTESIAN_POINT('Ctrl Pts',(47.0157420985959,3.22078462586054,-0.150498500899773));
#78710=CARTESIAN_POINT('Ctrl Pts',(47.0218919218703,3.22390320386356,-0.0504976327562812));
#78711=CARTESIAN_POINT('Ctrl Pts',(47.0280417451446,3.22237117658844,0.0494121725088487));
#78712=CARTESIAN_POINT('Ctrl Pts',(47.0341925287261,3.22083891008423,0.149337578887788));
#78713=CARTESIAN_POINT('Ctrl Pts',(47.0403433123075,3.21465460253941,0.249171459775504));
#78714=CARTESIAN_POINT('Ctrl Pts',(47.0464940958889,3.20385693885345,0.348451256075473));
#78715=CARTESIAN_POINT('Ctrl Pts',(47.0526514578309,3.19304772689509,0.447837233690782));
#78716=CARTESIAN_POINT('Ctrl Pts',(47.0588088197729,3.17761535305071,0.546667510678373));
#78717=CARTESIAN_POINT('Ctrl Pts',(47.0649661817148,3.15765021446684,0.644486373461454));
#78718=CARTESIAN_POINT('Ctrl Pts',(47.0711269801964,3.13767393296305,0.742359830794476));
#78719=CARTESIAN_POINT('Ctrl Pts',(47.0772877786781,3.11315995519581,0.839220328634971));
#78720=CARTESIAN_POINT('Ctrl Pts',(47.0834485771597,3.08424895927587,0.934626085504626));
#78721=CARTESIAN_POINT('Ctrl Pts',(47.0896196763495,3.05528962486019,1.03019135852465));
#78722=CARTESIAN_POINT('Ctrl Pts',(47.0957907755393,3.02191873272581,1.12429662255493));
#78723=CARTESIAN_POINT('Ctrl Pts',(47.1019618747291,2.98432566643191,1.21651875414057));
#78724=CARTESIAN_POINT('Ctrl Pts',(47.1066576448449,2.95572000124364,1.28669327511375));
#78725=CARTESIAN_POINT('Ctrl Pts',(47.1113534149608,2.92467064979647,1.35577782472826));
#78726=CARTESIAN_POINT('Ctrl Pts',(47.1160491850767,2.89127853832094,1.42359614229062));
#78727=CARTESIAN_POINT('Ctrl Pts',(47.1222212498799,2.84738834121644,1.51273573824845));
#78728=CARTESIAN_POINT('Ctrl Pts',(47.128393314683,2.79929470480908,1.60000058535238));
#78729=CARTESIAN_POINT('Ctrl Pts',(47.1345653794862,2.74718097696689,1.68496713389052));
#78730=CARTESIAN_POINT('Ctrl Pts',(47.1407294212012,2.69513499193866,1.76982323412015));
#78731=CARTESIAN_POINT('Ctrl Pts',(47.1468934629161,2.63907952473299,1.85238660546671));
#78732=CARTESIAN_POINT('Ctrl Pts',(47.1530575046311,2.57924488033207,1.93225604146572));
#78733=CARTESIAN_POINT('Ctrl Pts',(47.1592142957543,2.5194806177684,2.01203152925628));
#78734=CARTESIAN_POINT('Ctrl Pts',(47.1653710868774,2.45594627986877,2.08911903954387));
#78735=CARTESIAN_POINT('Ctrl Pts',(47.1715278780006,2.38891609433598,2.16314526944506));
#78736=CARTESIAN_POINT('Ctrl Pts',(47.177680431001,2.32193205007221,2.23712054224145));
#78737=CARTESIAN_POINT('Ctrl Pts',(47.1838329840014,2.25145723131628,2.30803840181296));
#78738=CARTESIAN_POINT('Ctrl Pts',(47.1899855370018,2.17780641596424,2.37555820326192));
#78739=CARTESIAN_POINT('Ctrl Pts',(47.1961360151527,2.10418043816494,2.44305523474394));
#78740=CARTESIAN_POINT('Ctrl Pts',(47.2022864933035,2.02738090985673,2.50715618991461));
#78741=CARTESIAN_POINT('Ctrl Pts',(47.2084369714544,1.94775914652902,2.56755756889939));
#78742=CARTESIAN_POINT('Ctrl Pts',(47.2124246552677,1.89613610047936,2.60671901218419));
#78743=CARTESIAN_POINT('Ctrl Pts',(47.216412339081,1.8433274341045,2.64432605614692));
#78744=CARTESIAN_POINT('Ctrl Pts',(47.2204000228943,1.78943621037803,2.68030513402633));
#78745=CARTESIAN_POINT('Origin',(-1.72497344927317,0.,0.));
#78746=CARTESIAN_POINT('',(48.7170675950372,1.78943621037805,2.68030513402632));
#78747=CARTESIAN_POINT('',(48.4702430335869,1.79020435040141,2.68143717906909));
#78748=CARTESIAN_POINT('',(-1.72497344927317,1.78943621037804,2.68030513402633));
#78749=CARTESIAN_POINT('',(47.8965734492249,-3.22274998787281,-0.000279581503351442));
#78750=CARTESIAN_POINT('Ctrl Pts',(47.896573449273,-3.22274998787274,-0.000279582277973307));
#78751=CARTESIAN_POINT('Ctrl Pts',(47.8974054557895,-3.22274882591617,-0.0136734766987837));
#78752=CARTESIAN_POINT('Ctrl Pts',(47.8982374623059,-3.22266416599954,-0.0270669804709197));
#78753=CARTESIAN_POINT('Ctrl Pts',(47.8990694688224,-3.22249601981345,-0.0404594214793921));
#78754=CARTESIAN_POINT('Ctrl Pts',(47.9052431614043,-3.22124833383841,-0.139834621161703));
#78755=CARTESIAN_POINT('Ctrl Pts',(47.9114168539863,-3.2153973580358,-0.239326650631789));
#78756=CARTESIAN_POINT('Ctrl Pts',(47.9175905465683,-3.2049263431869,-0.338474071749408));
#78757=CARTESIAN_POINT('Ctrl Pts',(47.9237558739739,-3.19446951626273,-0.437487150955776));
#78758=CARTESIAN_POINT('Ctrl Pts',(47.9299212013795,-3.17940513810442,-0.536156121936185));
#78759=CARTESIAN_POINT('Ctrl Pts',(47.9360865287852,-3.15976846088399,-0.634019586529329));
#78760=CARTESIAN_POINT('Ctrl Pts',(47.9422453217225,-3.14015259606112,-0.731779328211086));
#78761=CARTESIAN_POINT('Ctrl Pts',(47.9484041146598,-3.11597415164381,-0.828734837495918));
#78762=CARTESIAN_POINT('Ctrl Pts',(47.9545629075971,-3.08732006438016,-0.924430842505624));
#78763=CARTESIAN_POINT('Ctrl Pts',(47.9607171861463,-3.05868698052973,-1.02005670245306));
#78764=CARTESIAN_POINT('Ctrl Pts',(47.9668714646954,-3.02558490060815,-1.11442447901149));
#78765=CARTESIAN_POINT('Ctrl Pts',(47.9730257432445,-2.98815141939414,-1.20709098964113));
#78766=CARTESIAN_POINT('Ctrl Pts',(47.9791776800203,-2.95073218204796,-1.29972223960337));
#78767=CARTESIAN_POINT('Ctrl Pts',(47.985329616796,-2.9089849807545,-1.39065310783238));
#78768=CARTESIAN_POINT('Ctrl Pts',(47.9914815535718,-2.8630963637999,-1.47945827048139));
#78769=CARTESIAN_POINT('Ctrl Pts',(47.9976327930992,-2.81721294776975,-1.56825336813013));
#78770=CARTESIAN_POINT('Ctrl Pts',(48.0037840326267,-2.76718924859587,-1.65492285348826));
#78771=CARTESIAN_POINT('Ctrl Pts',(48.0099352721542,-2.71325834445333,-1.73906489779834));
#78772=CARTESIAN_POINT('Ctrl Pts',(48.0160874579449,-2.65931914396168,-1.82321988592582));
#78773=CARTESIAN_POINT('Ctrl Pts',(48.0222396437356,-2.60147177895841,-1.90484629518602));
#78774=CARTESIAN_POINT('Ctrl Pts',(48.0283918295263,-2.5399927706897,-1.98357109460287));
#78775=CARTESIAN_POINT('Ctrl Pts',(48.0345505634188,-2.47844832701058,-2.06237968505191));
#78776=CARTESIAN_POINT('Ctrl Pts',(48.0407092973112,-2.41326478906135,-2.13828015568584));
#78777=CARTESIAN_POINT('Ctrl Pts',(48.0468680312037,-2.34475903942898,-2.21093252034433));
#78778=CARTESIAN_POINT('Ctrl Pts',(48.0530301869928,-2.27621522684409,-2.28362525188473));
#78779=CARTESIAN_POINT('Ctrl Pts',(48.0591923427819,-2.20434583869357,-2.35306598162725));
#78780=CARTESIAN_POINT('Ctrl Pts',(48.065354498571,-2.12950317605368,-2.41895303502926));
#78781=CARTESIAN_POINT('Ctrl Pts',(48.0715269170853,-2.05453586715217,-2.48494981962745));
#78782=CARTESIAN_POINT('Ctrl Pts',(48.0776993355997,-1.97658573163578,-2.54738083436659));
#78783=CARTESIAN_POINT('Ctrl Pts',(48.083871754114,-1.89603666061632,-2.60598590635079));
#78784=CARTESIAN_POINT('Ctrl Pts',(48.0885533985967,-1.83494195146005,-2.65043657204613));
#78785=CARTESIAN_POINT('Ctrl Pts',(48.0932350430794,-1.77235275676703,-2.69268707810716));
#78786=CARTESIAN_POINT('Ctrl Pts',(48.0979166875621,-1.7084460037503,-2.73264154523963));
#78787=CARTESIAN_POINT('Ctrl Pts',(48.1040905820961,-1.62416930256219,-2.78533129285944));
#78788=CARTESIAN_POINT('Ctrl Pts',(48.1102644766302,-1.53730524013941,-2.83421092951381));
#78789=CARTESIAN_POINT('Ctrl Pts',(48.1164383711642,-1.44823306185246,-2.87901694351691));
#78790=CARTESIAN_POINT('Ctrl Pts',(48.1226039262358,-1.35928119888294,-2.92376243525704));
#78791=CARTESIAN_POINT('Ctrl Pts',(48.1287694813075,-1.26812753288073,-2.96444504796746));
#78792=CARTESIAN_POINT('Ctrl Pts',(48.1349350363791,-1.1751793770992,-3.00084504667281));
#78793=CARTESIAN_POINT('Ctrl Pts',(48.141094082028,-1.08232935341321,-3.03720661526494));
#78794=CARTESIAN_POINT('Ctrl Pts',(48.1472531276769,-0.98768900859587,-3.06929440166731));
#78795=CARTESIAN_POINT('Ctrl Pts',(48.1534121733258,-0.891688432166575,
-3.09693546953118));
#78796=CARTESIAN_POINT('Ctrl Pts',(48.1595667407557,-0.795757657395764,
-3.12455643967844));
#78797=CARTESIAN_POINT('Ctrl Pts',(48.1657213081857,-0.698469033277891,
-3.1477369997403));
#78798=CARTESIAN_POINT('Ctrl Pts',(48.1718758756156,-0.600269856836845,
-3.16635336964671));
#78799=CARTESIAN_POINT('Ctrl Pts',(48.1780281233123,-0.502107692890165,
-3.18496272281112));
#78800=CARTESIAN_POINT('Ctrl Pts',(48.184180371009,-0.403036084600878,-3.19901122333952));
#78801=CARTESIAN_POINT('Ctrl Pts',(48.1903326187057,-0.30351375894017,-3.20842593192269));
#78802=CARTESIAN_POINT('Ctrl Pts',(48.1964841906779,-0.204002364191394,
-3.21783960645296));
#78803=CARTESIAN_POINT('Ctrl Pts',(48.2026357626501,-0.104040782666354,
-3.22262046003778));
#78804=CARTESIAN_POINT('Ctrl Pts',(48.2087873346222,-0.00409311987213795,
-3.22274740072344));
#78805=CARTESIAN_POINT('Ctrl Pts',(48.2149398738825,0.0958702589352058,
-3.22287436136957));
#78806=CARTESIAN_POINT('Ctrl Pts',(48.2210924131428,0.195819280525088,-3.21834595500233));
#78807=CARTESIAN_POINT('Ctrl Pts',(48.2272449524031,0.295290589862111,-3.20919320547064));
#78808=CARTESIAN_POINT('Ctrl Pts',(48.2334040698349,0.394868251927418,-3.20003067000277));
#78809=CARTESIAN_POINT('Ctrl Pts',(48.2395631872667,0.493966748688855,-3.18623395804791));
#78810=CARTESIAN_POINT('Ctrl Pts',(48.2457223046985,0.592128711458684,-3.16788591201866));
#78811=CARTESIAN_POINT('Ctrl Pts',(48.2518848613001,0.690345486570182,-3.14952762068318));
#78812=CARTESIAN_POINT('Ctrl Pts',(48.2580474179016,0.787624263677323,-3.12661303354869));
#78813=CARTESIAN_POINT('Ctrl Pts',(48.2642099745031,0.883520765206578,-3.09927549920119));
#78814=CARTESIAN_POINT('Ctrl Pts',(48.2703828176556,0.979577337354357,-3.07189233299057));
#78815=CARTESIAN_POINT('Ctrl Pts',(48.2765556608081,1.07424661348701,-3.04007161099999));
#78816=CARTESIAN_POINT('Ctrl Pts',(48.2827285039605,1.16710215795649,-3.00399569164027));
#78817=CARTESIAN_POINT('Ctrl Pts',(48.2874069714076,1.23747842240244,-2.97665334546702));
#78818=CARTESIAN_POINT('Ctrl Pts',(48.2920854388547,1.30681319972372,-2.94686770528887));
#78819=CARTESIAN_POINT('Ctrl Pts',(48.2967639063017,1.3749305652862,-2.91473558031287));
#78820=CARTESIAN_POINT('Ctrl Pts',(48.3029274850561,1.46467079580665,-2.87240358055557));
#78821=CARTESIAN_POINT('Ctrl Pts',(48.3090910638104,1.55261480753019,-2.82584747331742));
#78822=CARTESIAN_POINT('Ctrl Pts',(48.3152546425648,1.63833672151117,-2.77524239471943));
#78823=CARTESIAN_POINT('Ctrl Pts',(48.3214098424018,1.72394210305904,-2.7247061098833));
#78824=CARTESIAN_POINT('Ctrl Pts',(48.3275650422389,1.8073310187133,-2.67013201273159));
#78825=CARTESIAN_POINT('Ctrl Pts',(48.3337202420759,1.88809912584259,-2.61174257029525));
#78826=CARTESIAN_POINT('Ctrl Pts',(48.3398689064705,1.96878147534777,-2.55341512435771));
#78827=CARTESIAN_POINT('Ctrl Pts',(48.3460175708651,2.04684819710807,-2.49128064024699));
#78828=CARTESIAN_POINT('Ctrl Pts',(48.3521662352597,2.12192191323499,-2.42560610088142));
#78829=CARTESIAN_POINT('Ctrl Pts',(48.3583104241631,2.19694098468834,-2.3599793647145));
#78830=CARTESIAN_POINT('Ctrl Pts',(48.3644546130665,2.26897105447251,-2.2908179817846));
#78831=CARTESIAN_POINT('Ctrl Pts',(48.3705988019699,2.33766672511419,-2.21843004054531));
#78832=CARTESIAN_POINT('Ctrl Pts',(48.3767406757194,2.40633651096445,-2.14606937535913));
#78833=CARTESIAN_POINT('Ctrl Pts',(48.3828825494689,2.47167409433348,-2.07048488309211));
#78834=CARTESIAN_POINT('Ctrl Pts',(48.3890244232184,2.53337062315425,-1.99202179913752));
#78835=CARTESIAN_POINT('Ctrl Pts',(48.3951656376339,2.59506052881372,-1.91356713824448));
#78836=CARTESIAN_POINT('Ctrl Pts',(48.4013068520493,2.65310988762784,-1.83223484249483));
#78837=CARTESIAN_POINT('Ctrl Pts',(48.4074480664648,2.7072505307929,-1.74840273564805));
#78838=CARTESIAN_POINT('Ctrl Pts',(48.4135902763867,2.76139995029351,-1.66455703940415));
#78839=CARTESIAN_POINT('Ctrl Pts',(48.4197324863086,2.81163915926097,-1.57821109326239));
#78840=CARTESIAN_POINT('Ctrl Pts',(48.4258746962306,2.85774422714311,-1.48977028253695));
#78841=CARTESIAN_POINT('Ctrl Pts',(48.4320235914747,2.90389947683881,-1.40123321080424));
#78842=CARTESIAN_POINT('Ctrl Pts',(48.4381724867187,2.94591139838106,-1.31059710858022));
#78843=CARTESIAN_POINT('Ctrl Pts',(48.4443213819628,2.98360288606393,-1.21829035158743));
#78844=CARTESIAN_POINT('Ctrl Pts',(48.4504737595226,3.02131571963959,-1.1259313183312));
#78845=CARTESIAN_POINT('Ctrl Pts',(48.4566261370824,3.05470310140924,-1.03190015688265));
#78846=CARTESIAN_POINT('Ctrl Pts',(48.4627785146422,3.0836375016226,-0.936641511511598));
#78847=CARTESIAN_POINT('Ctrl Pts',(48.4689413557902,3.11262111169791,-0.841220856050377));
#78848=CARTESIAN_POINT('Ctrl Pts',(48.4751041969382,3.13713650586268,-0.744568969294602));
#78849=CARTESIAN_POINT('Ctrl Pts',(48.4812670380863,3.15710703715677,-0.64714196157814));
#78850=CARTESIAN_POINT('Ctrl Pts',(48.4860484004047,3.1726009211487,-0.571554450509453));
#78851=CARTESIAN_POINT('Ctrl Pts',(48.4908297627231,3.18536018203299,-0.495500621829391));
#78852=CARTESIAN_POINT('Ctrl Pts',(48.4956111250415,3.195370606819,-0.419194760913312));
#78853=CARTESIAN_POINT('Ctrl Pts',(48.5017953688468,3.20831815259115,-0.320500285102992));
#78854=CARTESIAN_POINT('Ctrl Pts',(48.5079796126521,3.21671131869511,-0.221034556122838));
#78855=CARTESIAN_POINT('Ctrl Pts',(48.5141638564573,3.22046816606932,-0.121253263189552));
#78856=CARTESIAN_POINT('Ctrl Pts',(48.5203397087429,3.2242199157049,-0.0216073654164394));
#78857=CARTESIAN_POINT('Ctrl Pts',(48.5265155610285,3.22334783589932,0.0783528166081075));
#78858=CARTESIAN_POINT('Ctrl Pts',(48.5326914133142,3.21782147504578,0.178164298427564));
#78859=CARTESIAN_POINT('Ctrl Pts',(48.5388606914528,3.21230099696058,0.277869531697386));
#78860=CARTESIAN_POINT('Ctrl Pts',(48.5450299695915,3.20213611239049,0.377425949919311));
#78861=CARTESIAN_POINT('Ctrl Pts',(48.5511992477301,3.18734840121872,0.476369322845732));
#78862=CARTESIAN_POINT('Ctrl Pts',(48.5573639095059,3.17257175543246,0.575238658177498));
#78863=CARTESIAN_POINT('Ctrl Pts',(48.5635285712817,3.15317922536676,0.673495433867807));
#78864=CARTESIAN_POINT('Ctrl Pts',(48.5696932330575,3.12924424947995,0.770680212277874));
#78865=CARTESIAN_POINT('Ctrl Pts',(48.5758554869797,3.10531862234906,0.867827031310971));
#78866=CARTESIAN_POINT('Ctrl Pts',(48.5820177409018,3.07685417855164,0.96390226561091));
#78867=CARTESIAN_POINT('Ctrl Pts',(48.588179994824,3.04397535096775,1.05845719100998));
#78868=CARTESIAN_POINT('Ctrl Pts',(48.5943414734557,3.01110065996157,1.15300022018815));
#78869=CARTESIAN_POINT('Ctrl Pts',(48.6005029520874,2.97381283155318,1.24602291223366));
#78870=CARTESIAN_POINT('Ctrl Pts',(48.6066644307191,2.93228570302068,1.33709315994082));
#78871=CARTESIAN_POINT('Ctrl Pts',(48.612826765544,2.89075280391723,1.42817606268444));
#78872=CARTESIAN_POINT('Ctrl Pts',(48.618989100369,2.84497961414036,1.51730558859858));
#78873=CARTESIAN_POINT('Ctrl Pts',(48.625151435194,2.795187086339,1.60407191698617));
#78874=CARTESIAN_POINT('Ctrl Pts',(48.6313201165647,2.74534327756,1.69092760541116));
#78875=CARTESIAN_POINT('Ctrl Pts',(48.6374887979355,2.69147208003589,1.77541486009589));
#78876=CARTESIAN_POINT('Ctrl Pts',(48.6436574793062,2.63383911875181,1.85715079060174));
#78877=CARTESIAN_POINT('Ctrl Pts',(48.6498294857358,2.57617509199692,1.93893077862445));
#78878=CARTESIAN_POINT('Ctrl Pts',(48.6560014921654,2.51474552811655,2.01795614685807));
#78879=CARTESIAN_POINT('Ctrl Pts',(48.662173498595,2.44985661502894,2.09387681784267));
#78880=CARTESIAN_POINT('Ctrl Pts',(48.6683555081248,2.38486253512,2.16992053504982));
#78881=CARTESIAN_POINT('Ctrl Pts',(48.6745375176546,2.31639820269218,2.24284918805124));
#78882=CARTESIAN_POINT('Ctrl Pts',(48.6807195271844,2.24480703191651,2.31234922794075));
#78883=CARTESIAN_POINT('Ctrl Pts',(48.6852991327166,2.19177260675709,2.36383455251585));
#78884=CARTESIAN_POINT('Ctrl Pts',(48.6898787382488,2.1370230110744,2.41343910677724));
#78885=CARTESIAN_POINT('Ctrl Pts',(48.694458343781,2.08070882147903,2.46105025603285));
#78886=CARTESIAN_POINT('Ctrl Pts',(48.7006391968184,2.0047045177545,2.52530852334874));
#78887=CARTESIAN_POINT('Ctrl Pts',(48.7068200498558,1.92559082778242,2.58615246483035));
#78888=CARTESIAN_POINT('Ctrl Pts',(48.7130009028932,1.84370708895466,2.64326724578472));
#78889=CARTESIAN_POINT('Ctrl Pts',(48.7143564669412,1.82574862079535,2.65579346881604));
#78890=CARTESIAN_POINT('Ctrl Pts',(48.7157120309892,1.80765705640678,2.66814045872364));
#78891=CARTESIAN_POINT('Ctrl Pts',(48.7170675950372,1.78943621037805,2.68030513402632));
#78892=CARTESIAN_POINT('Ctrl Pts',(47.4668462457454,1.78943621037804,2.68030513402633));
#78893=CARTESIAN_POINT('Ctrl Pts',(47.4730172821142,1.70636788358127,2.73576354807726));
#78894=CARTESIAN_POINT('Ctrl Pts',(47.479188318483,1.62081413773693,2.78729317563132));
#78895=CARTESIAN_POINT('Ctrl Pts',(47.4853593548518,1.53318972188769,2.83468637404527));
#78896=CARTESIAN_POINT('Ctrl Pts',(47.4906979136823,1.45738590693071,2.87568619365003));
#78897=CARTESIAN_POINT('Ctrl Pts',(47.4960364725128,1.38003294650229,2.913591009904));
#78898=CARTESIAN_POINT('Ctrl Pts',(47.5013750313432,1.30141033699827,2.94829589716739));
#78899=CARTESIAN_POINT('Ctrl Pts',(47.507547600212,1.21050500332719,2.98842251439108));
#78900=CARTESIAN_POINT('Ctrl Pts',(47.5137201690807,1.11758221817913,3.02441140884019));
#78901=CARTESIAN_POINT('Ctrl Pts',(47.5198927379495,1.02305466733697,3.05605574395168));
#78902=CARTESIAN_POINT('Ctrl Pts',(47.5260569501904,0.928655091019067,3.08765723791585));
#78903=CARTESIAN_POINT('Ctrl Pts',(47.5322211624313,0.832655475507946,3.1149257266562));
#78904=CARTESIAN_POINT('Ctrl Pts',(47.5383853746722,0.735490068682984,3.13770169413357));
#78905=CARTESIAN_POINT('Ctrl Pts',(47.5445430622812,0.638427508497301,3.16045355393943));
#78906=CARTESIAN_POINT('Ctrl Pts',(47.5507007498902,0.540202030756116,3.17872224771765));
#78907=CARTESIAN_POINT('Ctrl Pts',(47.5568584374992,0.441263775350576,3.19239782030112));
#78908=CARTESIAN_POINT('Ctrl Pts',(47.563011629791,0.342397748169423,3.20606340926076));
#78909=CARTESIAN_POINT('Ctrl Pts',(47.5691648220828,0.242820406811316,3.21514248435243));
#78910=CARTESIAN_POINT('Ctrl Pts',(47.5753180143746,0.142991932068644,3.21957619413849));
#78911=CARTESIAN_POINT('Ctrl Pts',(47.5814688768994,0.0432012551194085,
3.22400822520065));
#78912=CARTESIAN_POINT('Ctrl Pts',(47.5876197394241,-0.056839932864205,
3.22379836656984));
#78913=CARTESIAN_POINT('Ctrl Pts',(47.5937706019489,-0.156667370397694,
3.21893971635889));
#78914=CARTESIAN_POINT('Ctrl Pts',(47.5999207804033,-0.25648370558835,3.2140816065044));
#78915=CARTESIAN_POINT('Ctrl Pts',(47.6060709588578,-0.356085903782014,
3.20457575409293));
#78916=CARTESIAN_POINT('Ctrl Pts',(47.6122211373122,-0.455011758880625,
3.19046734222126));
#78917=CARTESIAN_POINT('Ctrl Pts',(47.6183722763906,-0.553953065651398,
3.17635672669357));
#78918=CARTESIAN_POINT('Ctrl Pts',(47.6245234154689,-0.652217389483371,
3.15764218511765));
#78919=CARTESIAN_POINT('Ctrl Pts',(47.6306745545473,-0.749350687482992,
3.13442037858178));
#78920=CARTESIAN_POINT('Ctrl Pts',(47.6368322702674,-0.846587837938679,
3.11117374387996));
#78921=CARTESIAN_POINT('Ctrl Pts',(47.6429899859875,-0.942691124543513,
3.08341032224836));
#78922=CARTESIAN_POINT('Ctrl Pts',(47.6491477017075,-1.03721981015267,3.05127721256638));
#78923=CARTESIAN_POINT('Ctrl Pts',(47.6553088535669,-1.13180124482361,3.01912617191057));
#78924=CARTESIAN_POINT('Ctrl Pts',(47.6614700054262,-1.22480592437142,2.98260074595528));
#78925=CARTESIAN_POINT('Ctrl Pts',(47.6676311572856,-1.31581326616096,2.94189615912847));
#78926=CARTESIAN_POINT('Ctrl Pts',(47.6738026054996,-1.40697269702269,2.90112354786843));
#78927=CARTESIAN_POINT('Ctrl Pts',(47.6799740537136,-1.49612773479907,2.85615802087152));
#78928=CARTESIAN_POINT('Ctrl Pts',(47.6861455019276,-1.58288244116645,2.80724076985693));
#78929=CARTESIAN_POINT('Ctrl Pts',(47.6908377513127,-1.64884341231761,2.77004821261049));
#78930=CARTESIAN_POINT('Ctrl Pts',(47.6955300006978,-1.71341731197272,2.73057219493661));
#78931=CARTESIAN_POINT('Ctrl Pts',(47.7002222500829,-1.77644236525286,2.6889347491962));
#78932=CARTESIAN_POINT('Ctrl Pts',(47.7063797254309,-1.85914794631434,2.63429538017306));
#78933=CARTESIAN_POINT('Ctrl Pts',(47.7125372007789,-1.93947937218019,2.57573816524997));
#78934=CARTESIAN_POINT('Ctrl Pts',(47.7186946761269,-2.01704061049959,2.51349651642796));
#78935=CARTESIAN_POINT('Ctrl Pts',(47.7248437993372,-2.09449664301502,2.45133929357497));
#78936=CARTESIAN_POINT('Ctrl Pts',(47.7309929225474,-2.1691896181193,2.38550783992295));
#78937=CARTESIAN_POINT('Ctrl Pts',(47.7371420457577,-2.24075154303061,2.31627936244874));
#78938=CARTESIAN_POINT('Ctrl Pts',(47.7432846684349,-2.31223781639796,2.24712406971926));
#78939=CARTESIAN_POINT('Ctrl Pts',(47.749427291112,-2.38059930729441,2.17457919390108));
#78940=CARTESIAN_POINT('Ctrl Pts',(47.7555699137891,-2.44550104646649,2.09896217074803));
#78941=CARTESIAN_POINT('Ctrl Pts',(47.7617080978264,-2.51035588784531,2.02339978821887));
#78942=CARTESIAN_POINT('Ctrl Pts',(47.7678462818636,-2.57175566375418,1.94477000179743));
#78943=CARTESIAN_POINT('Ctrl Pts',(47.7739844659008,-2.62940291799779,1.86342637561152));
#78944=CARTESIAN_POINT('Ctrl Pts',(47.7801203781277,-2.68702883634914,1.78211285560963));
#78945=CARTESIAN_POINT('Ctrl Pts',(47.7862562903545,-2.74090474014038,1.6980878473495));
#78946=CARTESIAN_POINT('Ctrl Pts',(47.7923922025813,-2.79077464818404,1.61173646281061));
#78947=CARTESIAN_POINT('Ctrl Pts',(47.7985275060852,-2.84063960880401,1.52539364489841));
#78948=CARTESIAN_POINT('Ctrl Pts',(47.804662809589,-2.8864991454356,1.43672528776936));
#78949=CARTESIAN_POINT('Ctrl Pts',(47.8107981130929,-2.92814220246344,1.34614293618938));
#78950=CARTESIAN_POINT('Ctrl Pts',(47.8169344700213,-2.96979240955621,1.25554503172396));
#78951=CARTESIAN_POINT('Ctrl Pts',(47.8230708269497,-3.00722451686743,1.16303287698175));
#78952=CARTESIAN_POINT('Ctrl Pts',(47.8292071838781,-3.04027519801814,1.06903895289917));
#78953=CARTESIAN_POINT('Ctrl Pts',(47.8353501327987,-3.07336138392101,0.974944055678911));
#78954=CARTESIAN_POINT('Ctrl Pts',(47.8414930817193,-3.10205660135938,0.879364623766396));
#78955=CARTESIAN_POINT('Ctrl Pts',(47.8476360306399,-3.12624716888796,0.782749130641511));
#78956=CARTESIAN_POINT('Ctrl Pts',(47.8537825320079,-3.15045172574311,0.686077765090956));
#78957=CARTESIAN_POINT('Ctrl Pts',(47.8599290333759,-3.17014635990226,0.588369573355306));
#78958=CARTESIAN_POINT('Ctrl Pts',(47.8660755347439,-3.1852687799006,0.490081995476812));
#78959=CARTESIAN_POINT('Ctrl Pts',(47.8722321041398,-3.20041597056705,0.391633421608901));
#78960=CARTESIAN_POINT('Ctrl Pts',(47.8783886735356,-3.21097594526943,0.29260400048704));
#78961=CARTESIAN_POINT('Ctrl Pts',(47.8845452429314,-3.21693840401225,0.19345507822518));
#78962=CARTESIAN_POINT('Ctrl Pts',(47.8885546450292,-3.22082139355637,0.128885368804992));
#78963=CARTESIAN_POINT('Ctrl Pts',(47.8925640471271,-3.22275558727389,0.0642649951616726));
#78964=CARTESIAN_POINT('Ctrl Pts',(47.8965734492249,-3.22274998787281,-0.000279581503348901));
#78965=CARTESIAN_POINT('',(47.6500265507268,-3.22274888240162,-0.00268392978501451));
#78966=CARTESIAN_POINT('Ctrl Pts',(47.2204000228943,1.78943621037803,2.68030513402633));
#78967=CARTESIAN_POINT('Ctrl Pts',(47.2265503217517,1.70631850415497,2.73579651497059));
#78968=CARTESIAN_POINT('Ctrl Pts',(47.232700620609,1.62062450475473,2.7874130976737));
#78969=CARTESIAN_POINT('Ctrl Pts',(47.2388509194664,1.5327554146123,2.83492123373414));
#78970=CARTESIAN_POINT('Ctrl Pts',(47.2451880431622,1.44221716497809,2.88387250289288));
#78971=CARTESIAN_POINT('Ctrl Pts',(47.251525166858,1.34936998556573,2.92846147270142));
#78972=CARTESIAN_POINT('Ctrl Pts',(47.2578622905538,1.25467812721937,2.96848452237455));
#78973=CARTESIAN_POINT('Ctrl Pts',(47.2640218596828,1.16263936082786,3.00738619970428));
#78974=CARTESIAN_POINT('Ctrl Pts',(47.2701814288117,1.06885835291513,3.04197433513195));
#78975=CARTESIAN_POINT('Ctrl Pts',(47.2763409979407,0.973778471150405,3.07211214828235));
#78976=CARTESIAN_POINT('Ctrl Pts',(47.2827668989199,0.874587457534403,3.10355308172772));
#78977=CARTESIAN_POINT('Ctrl Pts',(47.2891927998991,0.773983233015376,3.13015002880449));
#78978=CARTESIAN_POINT('Ctrl Pts',(47.2956187008784,0.672481183617758,3.15180688180289));
#78979=CARTESIAN_POINT('Ctrl Pts',(47.3020446018576,0.570979134220111,3.17346373480129));
#78980=CARTESIAN_POINT('Ctrl Pts',(47.3084705028369,0.468579793637156,3.19018048042091));
#78981=CARTESIAN_POINT('Ctrl Pts',(47.3148964038161,0.365802898924829,3.2019222041827));
#78982=CARTESIAN_POINT('Ctrl Pts',(47.3210687091399,0.267082053951235,3.21320054543299));
#78983=CARTESIAN_POINT('Ctrl Pts',(47.3272410144636,0.167665388864387,3.21992885365931));
#78984=CARTESIAN_POINT('Ctrl Pts',(47.3334133197873,0.06800838669313,3.22203234338816));
#78985=CARTESIAN_POINT('Ctrl Pts',(47.3395772660597,-0.0315136516439381,
3.22413298439557));
#78986=CARTESIAN_POINT('Ctrl Pts',(47.3457412123321,-0.131274949682221,
3.2216212468552));
#78987=CARTESIAN_POINT('Ctrl Pts',(47.3519051586046,-0.230813505313807,
3.21447393647308));
#78988=CARTESIAN_POINT('Ctrl Pts',(47.3580625781933,-0.330246664720032,
3.20733419400805));
#78989=CARTESIAN_POINT('Ctrl Pts',(47.364219997782,-0.429457119750578,3.19556866794352));
#78990=CARTESIAN_POINT('Ctrl Pts',(47.3703774173707,-0.527982429544278,
3.17920620856725));
#78991=CARTESIAN_POINT('Ctrl Pts',(47.3765303396749,-0.626435777967615,
3.16285570007955));
#78992=CARTESIAN_POINT('Ctrl Pts',(47.3826832619791,-0.724204548868616,
3.14191500457379));
#78993=CARTESIAN_POINT('Ctrl Pts',(47.3888361842832,-0.820831908505135,
3.11646475039905));
#78994=CARTESIAN_POINT('Ctrl Pts',(47.3949867756992,-0.917422663166053,
3.09102413744743));
#78995=CARTESIAN_POINT('Ctrl Pts',(47.4011373671152,-1.0128724461579,3.0610774707991));
#78996=CARTESIAN_POINT('Ctrl Pts',(47.4072879585312,-1.10673597347601,3.02675619228145));
#78997=CARTESIAN_POINT('Ctrl Pts',(47.4134378650789,-1.20058904909106,2.99243873543791));
#78998=CARTESIAN_POINT('Ctrl Pts',(47.4195877716266,-1.29285581224778,2.95374778434491));
#78999=CARTESIAN_POINT('Ctrl Pts',(47.4257376781743,-1.38310842808469,2.91086389902742));
#79000=CARTESIAN_POINT('Ctrl Pts',(47.4318885448703,-1.47337513452599,2.86797331850384));
#79001=CARTESIAN_POINT('Ctrl Pts',(47.4380394115664,-1.56162667668805,2.82088868994946));
#79002=CARTESIAN_POINT('Ctrl Pts',(47.4441902782624,-1.64745832048031,2.76983729572338));
#79003=CARTESIAN_POINT('Ctrl Pts',(47.45034772256,-1.73338175074464,2.71873130825915));
#79004=CARTESIAN_POINT('Ctrl Pts',(47.4565051668576,-1.81687974104749,2.66365030682196));
#79005=CARTESIAN_POINT('Ctrl Pts',(47.4626626111552,-1.89757525903276,2.60486577366412));
#79006=CARTESIAN_POINT('Ctrl Pts',(47.4688234917003,-1.97831581027566,2.54604843497887));
#79007=CARTESIAN_POINT('Ctrl Pts',(47.4749843722455,-2.05625043577832,2.48352372037595));
#79008=CARTESIAN_POINT('Ctrl Pts',(47.4811452527906,-2.13103565698307,2.41760306733068));
#79009=CARTESIAN_POINT('Ctrl Pts',(47.4873164327096,-2.20594589943208,2.35157221227046));
#79010=CARTESIAN_POINT('Ctrl Pts',(47.4934876126286,-2.2776959086766,2.28213438111367));
#79011=CARTESIAN_POINT('Ctrl Pts',(47.4996587925476,-2.34597940490285,2.20963757079564));
#79012=CARTESIAN_POINT('Ctrl Pts',(47.5043537358837,-2.39792848915891,2.15448305886163));
#79013=CARTESIAN_POINT('Ctrl Pts',(47.5090486792197,-2.44787194695625,2.09755878406992));
#79014=CARTESIAN_POINT('Ctrl Pts',(47.5137436225558,-2.49569140684989,2.03902966243152));
#79015=CARTESIAN_POINT('Ctrl Pts',(47.5198916750508,-2.55831123602816,1.96238547600402));
#79016=CARTESIAN_POINT('Ctrl Pts',(47.5260397275457,-2.61751393702052,1.88271087171108));
#79017=CARTESIAN_POINT('Ctrl Pts',(47.5321877800407,-2.67299039278759,1.8003443899891));
#79018=CARTESIAN_POINT('Ctrl Pts',(47.5383278548084,-2.72839486217701,1.71808478720483));
#79019=CARTESIAN_POINT('Ctrl Pts',(47.5444679295762,-2.78008244862477,1.63314060436496));
#79020=CARTESIAN_POINT('Ctrl Pts',(47.550608004344,-2.8277835636169,1.54588410944616));
#79021=CARTESIAN_POINT('Ctrl Pts',(47.5567417847098,-2.87543577855413,1.45871706416376));
#79022=CARTESIAN_POINT('Ctrl Pts',(47.5628755650755,-2.91910943321578,1.36924279815371));
#79023=CARTESIAN_POINT('Ctrl Pts',(47.5690093454413,-2.95857824073278,1.27786241667971));
#79024=CARTESIAN_POINT('Ctrl Pts',(47.5751385086787,-2.99801733858624,1.18655082067351));
#79025=CARTESIAN_POINT('Ctrl Pts',(47.5812676719161,-3.03325770759927,1.09333636151927));
#79026=CARTESIAN_POINT('Ctrl Pts',(47.5873968351535,-3.06411951315494,0.998643665980567));
#79027=CARTESIAN_POINT('Ctrl Pts',(47.5935237873491,-3.09497018558514,0.903985130000682));
#79028=CARTESIAN_POINT('Ctrl Pts',(47.5996507395447,-3.1214452944217,0.807849831755124));
#79029=CARTESIAN_POINT('Ctrl Pts',(47.6057776917403,-3.14341389342911,0.710680418399755));
#79030=CARTESIAN_POINT('Ctrl Pts',(47.6119033629361,-3.16537789932581,0.613531320853912));
#79031=CARTESIAN_POINT('Ctrl Pts',(47.6180290341319,-3.18283717672938,0.515348965925687));
#79032=CARTESIAN_POINT('Ctrl Pts',(47.6241547053277,-3.19571150870808,0.416587944629584));
#79033=CARTESIAN_POINT('Ctrl Pts',(47.6302823669541,-3.20859002397757,0.317794832653253));
#79034=CARTESIAN_POINT('Ctrl Pts',(47.6364100285805,-3.21688056513942,0.218423113421889));
#79035=CARTESIAN_POINT('Ctrl Pts',(47.6425376902069,-3.22055466709273,0.118933589734913));
#79036=CARTESIAN_POINT('Ctrl Pts',(47.6450339770468,-3.22205142277443,0.0784035468182273));
#79037=CARTESIAN_POINT('Ctrl Pts',(47.6475302638868,-3.22278264268373,0.0378539829513926));
#79038=CARTESIAN_POINT('Ctrl Pts',(47.6500265507268,-3.22274888240162,-0.00268392978501451));
#79039=CARTESIAN_POINT('Ctrl Pts',(47.6500278454515,-3.22023055859585,-0.00270284149074349));
#79040=CARTESIAN_POINT('Ctrl Pts',(47.6708821773994,-3.22287022505361,-0.341100026664383));
#79041=CARTESIAN_POINT('Ctrl Pts',(47.7580189155941,-3.01777852171772,-1.75191763288685));
#79042=CARTESIAN_POINT('Ctrl Pts',(47.9114380600351,-0.968103398024024,
-3.68661448347931));
#79043=CARTESIAN_POINT('Ctrl Pts',(48.1102852787748,2.57778134821769,-2.80783294777081));
#79044=CARTESIAN_POINT('Ctrl Pts',(48.296553603292,3.68122906515452,0.43159223718354));
#79045=CARTESIAN_POINT('Ctrl Pts',(48.4165395215627,2.50785121046015,2.19182082035424));
#79046=CARTESIAN_POINT('Ctrl Pts',(48.4702430335869,1.79020435040156,2.68143717906899));
#79047=CARTESIAN_POINT('Origin',(24.9384,0.,0.));
#79048=CARTESIAN_POINT('',(0.989963935465355,-3.93416568820139,0.00240681427912712));
#79049=CARTESIAN_POINT('',(0.585831332880558,1.74924991682375,3.52258622726146));
#79050=CARTESIAN_POINT('Ctrl Pts',(0.989963522034966,-3.93299925901829,
0.00241424140712914));
#79051=CARTESIAN_POINT('Ctrl Pts',(0.983684296778858,-3.93292343624727,
0.125935816900034));
#79052=CARTESIAN_POINT('Ctrl Pts',(0.977405071522742,-3.92702906700058,
0.249289462579013));
#79053=CARTESIAN_POINT('Ctrl Pts',(0.971125846266634,-3.91536025446055,
0.372079397159524));
#79054=CARTESIAN_POINT('Ctrl Pts',(0.965241985179104,-3.9044261552299,0.487138005276138));
#79055=CARTESIAN_POINT('Ctrl Pts',(0.959358124091569,-3.88839801893483,
0.601903673559196));
#79056=CARTESIAN_POINT('Ctrl Pts',(0.95347426300404,-3.86729751325782,0.715890315586026));
#79057=CARTESIAN_POINT('Ctrl Pts',(0.947598037826548,-3.84622439122579,
0.829729028943051));
#79058=CARTESIAN_POINT('Ctrl Pts',(0.941721812649061,-3.82009206596904,
0.942790325620221));
#79059=CARTESIAN_POINT('Ctrl Pts',(0.935845587471569,-3.7889740420547,1.05459220015874));
#79060=CARTESIAN_POINT('Ctrl Pts',(0.929975432826291,-3.75788816513285,
1.16627857591011));
#79061=CARTESIAN_POINT('Ctrl Pts',(0.924105278181015,-3.72182694485705,
1.27670772340426));
#79062=CARTESIAN_POINT('Ctrl Pts',(0.918235123535737,-3.68091499425547,
1.38540745092021));
#79063=CARTESIAN_POINT('Ctrl Pts',(0.912153602868706,-3.63852993148507,
1.49802111773744));
#79064=CARTESIAN_POINT('Ctrl Pts',(0.90607208220167,-3.59093831837406,1.60877803345252));
#79065=CARTESIAN_POINT('Ctrl Pts',(0.89999056153464,-3.53833547547697,1.71716949162893));
#79066=CARTESIAN_POINT('Ctrl Pts',(0.894127361297117,-3.48762102133713,
1.82166980629048));
#79067=CARTESIAN_POINT('Ctrl Pts',(0.888264161059598,-3.43224914112038,
1.92397117538651));
#79068=CARTESIAN_POINT('Ctrl Pts',(0.882400960822075,-3.37244370385505,
2.02363842232956));
#79069=CARTESIAN_POINT('Ctrl Pts',(0.876538733713052,-3.31264819263234,
2.12328912727597));
#79070=CARTESIAN_POINT('Ctrl Pts',(0.870676506604024,-3.24842079940996,
2.22030622661834));
#79071=CARTESIAN_POINT('Ctrl Pts',(0.864814279495,-3.18003049757982,2.31428067322489));
#79072=CARTESIAN_POINT('Ctrl Pts',(0.85895162032655,-3.1116351552294,2.40826204596119));
#79073=CARTESIAN_POINT('Ctrl Pts',(0.853088961158097,-3.03907653664482,
2.49919998737317));
#79074=CARTESIAN_POINT('Ctrl Pts',(0.847226301989647,-2.96266552858476,
2.58671644478779));
#79075=CARTESIAN_POINT('Ctrl Pts',(0.841361805614357,-2.8862305752769,2.67426032761286));
#79076=CARTESIAN_POINT('Ctrl Pts',(0.835497309239071,-2.80594110245673,
2.75838028438628));
#79077=CARTESIAN_POINT('Ctrl Pts',(0.829632812863782,-2.72214618334568,
2.83873372412711));
#79078=CARTESIAN_POINT('Ctrl Pts',(0.823761874740816,-2.63825922125414,
2.919175426619));
#79079=CARTESIAN_POINT('Ctrl Pts',(0.817890936617861,-2.55085942448793,
2.99584206890481));
#79080=CARTESIAN_POINT('Ctrl Pts',(0.812019998494897,-2.46033047483642,
3.06843004720512));
#79081=CARTESIAN_POINT('Ctrl Pts',(0.806145224363962,-2.36974237454065,
3.14106545371153));
#79082=CARTESIAN_POINT('Ctrl Pts',(0.800270450233023,-2.27602138115173,
3.20961664647278));
#79083=CARTESIAN_POINT('Ctrl Pts',(0.794395676102088,-2.17958039394005,
3.27382319411909));
#79084=CARTESIAN_POINT('Ctrl Pts',(0.788512509971539,-2.08300164266983,
3.33812145955931));
#79085=CARTESIAN_POINT('Ctrl Pts',(0.782629343840982,-1.98369549383543,
3.39806248092037));
#79086=CARTESIAN_POINT('Ctrl Pts',(0.776746177710432,-1.88209972512649,
3.45343157231743));
#79087=CARTESIAN_POINT('Ctrl Pts',(0.77525699431595,-1.85638317584779,3.46744693915331));
#79088=CARTESIAN_POINT('Ctrl Pts',(0.77376781092148,-1.83052002340702,3.48116961036836));
#79089=CARTESIAN_POINT('Ctrl Pts',(0.772278627526997,-1.80451755736747,
3.4945965983433));
#79090=CARTESIAN_POINT('Ctrl Pts',(0.766455262790914,-1.70283643176066,
3.5471020510463));
#79091=CARTESIAN_POINT('Ctrl Pts',(0.760631898054829,-1.59868024946819,
3.59525952156886));
#79092=CARTESIAN_POINT('Ctrl Pts',(0.754808533318744,-1.49246073302146,
3.6388253544776));
#79093=CARTESIAN_POINT('Ctrl Pts',(0.748992614587671,-1.38637703342419,
3.68233548223566));
#79094=CARTESIAN_POINT('Ctrl Pts',(0.7431766958566,-1.27823563018259,3.7212654856502));
#79095=CARTESIAN_POINT('Ctrl Pts',(0.737360777125527,-1.16847319636026,
3.75541733891024));
#79096=CARTESIAN_POINT('Ctrl Pts',(0.731550674180361,-1.05882052246498,
3.78953504109698));
#79097=CARTESIAN_POINT('Ctrl Pts',(0.725740571235197,-0.947550440725385,
3.81888396960525));
#79098=CARTESIAN_POINT('Ctrl Pts',(0.71993046829003,-0.835119262116037,
3.84331430123048));
#79099=CARTESIAN_POINT('Ctrl Pts',(0.714124405676074,-0.722766267870076,
3.86772764406356));
#79100=CARTESIAN_POINT('Ctrl Pts',(0.70831834306211,-0.609254192345964,
3.8872291026441));
#79101=CARTESIAN_POINT('Ctrl Pts',(0.702512280448154,-0.495053445997505,
3.90171899111225));
#79102=CARTESIAN_POINT('Ctrl Pts',(0.696708301752118,-0.380893688697493,
3.91620367885484));
#79103=CARTESIAN_POINT('Ctrl Pts',(0.690904323056092,-0.266046168834459,
3.92568031837934));
#79104=CARTESIAN_POINT('Ctrl Pts',(0.685100344360055,-0.150989718573033,
3.93010064818768));
#79105=CARTESIAN_POINT('Ctrl Pts',(0.679296985641433,-0.0359455585704462,
3.93452050581913));
#79106=CARTESIAN_POINT('Ctrl Pts',(0.673493626922802,0.0793070669081008,
3.93388511163517));
#79107=CARTESIAN_POINT('Ctrl Pts',(0.667690268204179,0.194286813897208,
3.92819826815624));
#79108=CARTESIAN_POINT('Ctrl Pts',(0.661886066318469,0.309283266236282,
3.92251059843866));
#79109=CARTESIAN_POINT('Ctrl Pts',(0.656081864432768,0.424006340962809,
3.91177004230581));
#79110=CARTESIAN_POINT('Ctrl Pts',(0.650277662547058,0.537978126806255,
3.8960324093978));
#79111=CARTESIAN_POINT('Ctrl Pts',(0.644467730218229,0.652062436102339,
3.88027923884792));
#79112=CARTESIAN_POINT('Ctrl Pts',(0.638657797889396,0.765393557871783,
3.85951919809204));
#79113=CARTESIAN_POINT('Ctrl Pts',(0.632847865560567,0.877502083968805,
3.83385955567368));
#79114=CARTESIAN_POINT('Ctrl Pts',(0.627034879167403,0.989669541329025,
3.80818642494008));
#79115=CARTESIAN_POINT('Ctrl Pts',(0.621221892774245,1.10061271792731,3.77760867621448));
#79116=CARTESIAN_POINT('Ctrl Pts',(0.615408906381081,1.20987750582488,3.74228345010088));
#79117=CARTESIAN_POINT('Ctrl Pts',(0.609587021543605,1.31930955484514,3.70690414858849));
#79118=CARTESIAN_POINT('Ctrl Pts',(0.603765136706121,1.42705769026697,3.66676300351413));
#79119=CARTESIAN_POINT('Ctrl Pts',(0.597943251868646,1.53268768508301,3.62206535832733));
#79120=CARTESIAN_POINT('Ctrl Pts',(0.593905945539284,1.60593898746127,3.59106885275259));
#79121=CARTESIAN_POINT('Ctrl Pts',(0.589868639209918,1.67817213107512,3.55788211578977));
#79122=CARTESIAN_POINT('Ctrl Pts',(0.585831332880556,1.74924991682375,3.52258622726146));
#79123=CARTESIAN_POINT('',(0.585799999999996,-1.74869447533084,3.52286199445102));
#79124=CARTESIAN_POINT('Origin',(0.585799999999996,0.,0.));
#79125=CARTESIAN_POINT('',(0.806636477965097,-3.93492227854593,0.00403485423253799));
#79126=CARTESIAN_POINT('Ctrl Pts',(0.585799999999983,-1.74869447533085,
3.52286199445101));
#79127=CARTESIAN_POINT('Ctrl Pts',(0.65208240624653,-2.92241244012897,2.94024646086725));
#79128=CARTESIAN_POINT('Ctrl Pts',(0.725694565568235,-3.86568596277398,
1.59600203772709));
#79129=CARTESIAN_POINT('Ctrl Pts',(0.79930672488994,-3.93806320532033,0.148344931151628));
#79130=CARTESIAN_POINT('Ctrl Pts',(0.806636477965097,-3.93698214742112,
0.00403696641419293));
#79131=CARTESIAN_POINT('',(2.05663644556805,-3.93145140809557,0.00214295819816745));
#79132=CARTESIAN_POINT('Ctrl Pts',(0.806636477965096,-3.93299793235017,
0.00403288101531948));
#79133=CARTESIAN_POINT('Ctrl Pts',(0.812372634790166,-3.93311361551045,
-0.108785133810083));
#79134=CARTESIAN_POINT('Ctrl Pts',(0.818108791615234,-3.92837095544938,
-0.221831062669951));
#79135=CARTESIAN_POINT('Ctrl Pts',(0.823844948440303,-3.91873779066641,
-0.334638802297222));
#79136=CARTESIAN_POINT('Ctrl Pts',(0.829573999063958,-3.90911655986839,
-0.447306790773436));
#79137=CARTESIAN_POINT('Ctrl Pts',(0.835303049687616,-3.89461689714465,
-0.559736749150826));
#79138=CARTESIAN_POINT('Ctrl Pts',(0.841032100311271,-3.87525862470365,
-0.671460789368933));
#79139=CARTESIAN_POINT('Ctrl Pts',(0.846968031026604,-3.85520131128005,
-0.78721926412103));
#79140=CARTESIAN_POINT('Ctrl Pts',(0.852903961741931,-3.82992782729007,
-0.902219406262141));
#79141=CARTESIAN_POINT('Ctrl Pts',(0.858839892457265,-3.7995192218675,-1.01594423206166));
#79142=CARTESIAN_POINT('Ctrl Pts',(0.864560073793223,-3.77021585807632,
-1.1255355762283));
#79143=CARTESIAN_POINT('Ctrl Pts',(0.870280255129183,-3.73614427695648,
-1.23394223546885));
#79144=CARTESIAN_POINT('Ctrl Pts',(0.876000436465141,-3.69742913017487,
-1.34071131394282));
#79145=CARTESIAN_POINT('Ctrl Pts',(0.88171906679873,-3.65872448083746,-1.44745144244409));
#79146=CARTESIAN_POINT('Ctrl Pts',(0.887437697132324,-3.61537891402056,
-1.5525544652223));
#79147=CARTESIAN_POINT('Ctrl Pts',(0.893156327465913,-3.56756658433904,
-1.65558378414006));
#79148=CARTESIAN_POINT('Ctrl Pts',(0.898874923668654,-3.51975454001874,
-1.75861248814167));
#79149=CARTESIAN_POINT('Ctrl Pts',(0.904593519871397,-3.46747596893911,
-1.85956712037717));
#79150=CARTESIAN_POINT('Ctrl Pts',(0.910312116074138,-3.4109522850809,-1.95803307145241));
#79151=CARTESIAN_POINT('Ctrl Pts',(0.916032194932967,-3.35441394637017,
-2.0565245517199));
#79152=CARTESIAN_POINT('Ctrl Pts',(0.921752273791793,-3.29362852544886,
-2.1525256944756));
#79153=CARTESIAN_POINT('Ctrl Pts',(0.927472352650621,-3.22886178257336,
-2.24564925779544));
#79154=CARTESIAN_POINT('Ctrl Pts',(0.933198659375992,-3.16402452342685,
-2.3388742115224));
#79155=CARTESIAN_POINT('Ctrl Pts',(0.938924966101368,-3.09519754230098,
-2.42921498008899));
#79156=CARTESIAN_POINT('Ctrl Pts',(0.944651272826739,-3.02268793654951,
-2.51631608472347));
#79157=CARTESIAN_POINT('Ctrl Pts',(0.950381294483434,-2.95013129032003,
-2.60347369604497));
#79158=CARTESIAN_POINT('Ctrl Pts',(0.956111316140125,-2.87388755933752,
-2.68738714521717));
#79159=CARTESIAN_POINT('Ctrl Pts',(0.96184133779682,-2.79430046944768,-2.76773804512719));
#79160=CARTESIAN_POINT('Ctrl Pts',(0.967579836774316,-2.71459563387847,
-2.84820782074067));
#79161=CARTESIAN_POINT('Ctrl Pts',(0.973318335751806,-2.63153789155595,
-2.92510424442966));
#79162=CARTESIAN_POINT('Ctrl Pts',(0.979056834729302,-2.54550357690634,
-2.99814951927969));
#79163=CARTESIAN_POINT('Ctrl Pts',(0.980536035645958,-2.5233266910007,-3.01697824747834));
#79164=CARTESIAN_POINT('Ctrl Pts',(0.982015236562617,-2.50095217360799,
-3.03555131633519));
#79165=CARTESIAN_POINT('Ctrl Pts',(0.983494437479273,-2.47838675880302,
-3.05386444915125));
#79166=CARTESIAN_POINT('Ctrl Pts',(0.989375340371957,-2.38867277086066,
-3.12667251365377));
#79167=CARTESIAN_POINT('Ctrl Pts',(0.995256243264646,-2.29559995768826,
-3.19564383824247));
#79168=CARTESIAN_POINT('Ctrl Pts',(1.00113714615733,-2.19953006256088,-3.26045341998485));
#79169=CARTESIAN_POINT('Ctrl Pts',(1.00701044555888,-2.10358437737356,-3.32517920862792));
#79170=CARTESIAN_POINT('Ctrl Pts',(1.01288374496043,-2.00464965514114,-3.38575372729037));
#79171=CARTESIAN_POINT('Ctrl Pts',(1.01875704436198,-1.90312105332842,-3.44189181357842));
#79172=CARTESIAN_POINT('Ctrl Pts',(1.02462430792401,-1.80169678986217,-3.49797220819148));
#79173=CARTESIAN_POINT('Ctrl Pts',(1.03049157148602,-1.69768430773464,-3.54962504138893));
#79174=CARTESIAN_POINT('Ctrl Pts',(1.03635883504804,-1.59150757477639,-3.59660849126359));
#79175=CARTESIAN_POINT('Ctrl Pts',(1.04244145259683,-1.48143369581434,-3.64531643725734));
#79176=CARTESIAN_POINT('Ctrl Pts',(1.04852407014562,-1.36903401549716,-3.68900539503127));
#79177=CARTESIAN_POINT('Ctrl Pts',(1.0546066876944,-1.25480907559537,-3.72745800563916));
#79178=CARTESIAN_POINT('Ctrl Pts',(1.06046709673469,-1.14475696972857,-3.7645058760702));
#79179=CARTESIAN_POINT('Ctrl Pts',(1.06632750577497,-1.03301105334662,-3.79669314223012));
#79180=CARTESIAN_POINT('Ctrl Pts',(1.07218791481525,-0.920038438947165,
-3.82387477185899));
#79181=CARTESIAN_POINT('Ctrl Pts',(1.07804739144925,-0.807083798783841,
-3.85105207682005));
#79182=CARTESIAN_POINT('Ctrl Pts',(1.08390686808325,-0.692903249131352,
-3.87322523260343));
#79183=CARTESIAN_POINT('Ctrl Pts',(1.08976634471724,-0.57797684805735,-3.89029970093689));
#79184=CARTESIAN_POINT('Ctrl Pts',(1.0956262962771,-0.463041131898891,-3.90737555320053));
#79185=CARTESIAN_POINT('Ctrl Pts',(1.10148624783695,-0.347359851667637,
-3.91935183596716));
#79186=CARTESIAN_POINT('Ctrl Pts',(1.10734619939681,-0.231420299174159,
-3.92618563559215));
#79187=CARTESIAN_POINT('Ctrl Pts',(1.11320803320733,-0.11544350621927,-3.9330216302735));
#79188=CARTESIAN_POINT('Ctrl Pts',(1.11906986701784,0.000791312908998643,
-3.93471183292274));
#79189=CARTESIAN_POINT('Ctrl Pts',(1.12493170082837,0.116795436012624,-3.93126542300652));
#79190=CARTESIAN_POINT('Ctrl Pts',(1.13080005434631,0.232928582382179,-3.92781517988979));
#79191=CARTESIAN_POINT('Ctrl Pts',(1.13666840786426,0.348830108527222,-3.91921693303263));
#79192=CARTESIAN_POINT('Ctrl Pts',(1.14253676138221,0.464014881146512,-3.90553187031864));
#79193=CARTESIAN_POINT('Ctrl Pts',(1.14840899313578,0.579275776256942,-3.89183776351798));
#79194=CARTESIAN_POINT('Ctrl Pts',(1.15428122488935,0.693818568909999,-3.87305021272871));
#79195=CARTESIAN_POINT('Ctrl Pts',(1.16015345664292,0.807168491414923,-3.84928149483341));
#79196=CARTESIAN_POINT('Ctrl Pts',(1.16603415994399,0.920681937652066,-3.82547848710911));
#79197=CARTESIAN_POINT('Ctrl Pts',(1.17191486324507,1.03299868141443,-3.7966800717954));
#79198=CARTESIAN_POINT('Ctrl Pts',(1.17779556654614,1.1436591919416,-3.76304831920711));
#79199=CARTESIAN_POINT('Ctrl Pts',(1.1793109297704,1.17217463634432,-3.75438195424523));
#79200=CARTESIAN_POINT('Ctrl Pts',(1.18082629299465,1.20058021115646,-3.74539489838777));
#79201=CARTESIAN_POINT('Ctrl Pts',(1.18234165621891,1.22886828704132,-3.73609043427807));
#79202=CARTESIAN_POINT('Ctrl Pts',(1.1882243843005,1.33868424120848,-3.69996996400009));
#79203=CARTESIAN_POINT('Ctrl Pts',(1.19410711238208,1.44708284648009,-3.65894555660818));
#79204=CARTESIAN_POINT('Ctrl Pts',(1.19998984046366,1.55359503319098,-3.61314703172239));
#79205=CARTESIAN_POINT('Ctrl Pts',(1.20586514879311,1.65997287848507,-3.56740627148223));
#79206=CARTESIAN_POINT('Ctrl Pts',(1.21174045712255,1.76446866236883,-3.51690353076491));
#79207=CARTESIAN_POINT('Ctrl Pts',(1.217615765452,1.86662890811831,-3.46181823892836));
#79208=CARTESIAN_POINT('Ctrl Pts',(1.22348521851548,1.96868734212001,-3.40678784447188));
#79209=CARTESIAN_POINT('Ctrl Pts',(1.22935467157896,2.0684145078154,-3.34718417793659));
#79210=CARTESIAN_POINT('Ctrl Pts',(1.23522412464244,2.16537794472313,-3.28323428291473));
#79211=CARTESIAN_POINT('Ctrl Pts',(1.24130598923895,2.26585042277286,-3.21697008448311));
#79212=CARTESIAN_POINT('Ctrl Pts',(1.24738785383545,2.36335493625515,-3.14603930720408));
#79213=CARTESIAN_POINT('Ctrl Pts',(1.25346971843196,2.45743907257205,-3.07074619670793));
#79214=CARTESIAN_POINT('Ctrl Pts',(1.2593327570952,2.54813805477908,-2.99816213783748));
#79215=CARTESIAN_POINT('Ctrl Pts',(1.26519579575845,2.63565820070237,-2.92152452934664));
#79216=CARTESIAN_POINT('Ctrl Pts',(1.27105883442169,2.71962534769648,-2.84114888173196));
#79217=CARTESIAN_POINT('Ctrl Pts',(1.27692109967458,2.80358141834184,-2.76078383670098));
#79218=CARTESIAN_POINT('Ctrl Pts',(1.28278336492747,2.88398512471447,-2.67668201764516));
#79219=CARTESIAN_POINT('Ctrl Pts',(1.28864563018036,2.96049787944984,-2.58919703880817));
#79220=CARTESIAN_POINT('Ctrl Pts',(1.29450852716744,3.03701887941485,-2.50170263234381));
#79221=CARTESIAN_POINT('Ctrl Pts',(1.30037142415452,3.10964782302408,-2.41082465108394));
#79222=CARTESIAN_POINT('Ctrl Pts',(1.3062343211416,3.178085723247,-2.31695061140578));
#79223=CARTESIAN_POINT('Ctrl Pts',(1.31209925511507,3.24654740131754,-2.22304395642814));
#79224=CARTESIAN_POINT('Ctrl Pts',(1.31796418908855,3.31081489785301,-2.12613950537412));
#79225=CARTESIAN_POINT('Ctrl Pts',(1.32382912306202,3.37063234323854,-2.02665404218734));
#79226=CARTESIAN_POINT('Ctrl Pts',(1.32970079216489,3.4305184813386,-1.92705433262179));
#79227=CARTESIAN_POINT('Ctrl Pts',(1.33557246126776,3.48594415583052,-1.8248680478289));
#79228=CARTESIAN_POINT('Ctrl Pts',(1.34144413037063,3.53669923705489,-1.72053698205396));
#79229=CARTESIAN_POINT('Ctrl Pts',(1.34731980744516,3.58748896344122,-1.61613470042075));
#79230=CARTESIAN_POINT('Ctrl Pts',(1.35319548451969,3.63360158470154,-1.50958509926003));
#79231=CARTESIAN_POINT('Ctrl Pts',(1.35907116159422,3.67487559543297,-1.40134876390253));
#79232=CARTESIAN_POINT('Ctrl Pts',(1.36495547492183,3.7162102719903,-1.29295333940975));
#79233=CARTESIAN_POINT('Ctrl Pts',(1.37083978824944,3.75269201467683,-1.18286662188127));
#79234=CARTESIAN_POINT('Ctrl Pts',(1.37672410157706,3.78420947000849,-1.07156319790203));
#79235=CARTESIAN_POINT('Ctrl Pts',(1.37821235937089,3.79218085017261,-1.04341238760437));
#79236=CARTESIAN_POINT('Ctrl Pts',(1.37970061716473,3.7998349301741,-1.01518378915294));
#79237=CARTESIAN_POINT('Ctrl Pts',(1.38118887495856,3.80717043128948,-0.986885153964277));
#79238=CARTESIAN_POINT('Ctrl Pts',(1.38705348940439,3.83607663691244,-0.875371822462174));
#79239=CARTESIAN_POINT('Ctrl Pts',(1.3929181038502,3.86012892210552,-0.762395905546755));
#79240=CARTESIAN_POINT('Ctrl Pts',(1.39878271829603,3.87918063792592,-0.648418520972878));
#79241=CARTESIAN_POINT('Ctrl Pts',(1.40463962831864,3.8982073252499,-0.534590870028694));
#79242=CARTESIAN_POINT('Ctrl Pts',(1.41049653834125,3.9122464385708,-0.419764772610415));
#79243=CARTESIAN_POINT('Ctrl Pts',(1.41635344836386,3.9212013774418,-0.304415435792203));
#79244=CARTESIAN_POINT('Ctrl Pts',(1.42220424217116,3.93014696490839,-0.189186555217397));
#79245=CARTESIAN_POINT('Ctrl Pts',(1.42805503597846,3.93401890569487,-0.0734359327945867));
#79246=CARTESIAN_POINT('Ctrl Pts',(1.43390582978577,3.93277195371724,0.0423528045715599));
#79247=CARTESIAN_POINT('Ctrl Pts',(1.43999459078212,3.93147428491951,0.162850974753455));
#79248=CARTESIAN_POINT('Ctrl Pts',(1.44608335177847,3.92463242110289,0.283389975391991));
#79249=CARTESIAN_POINT('Ctrl Pts',(1.45217211277483,3.91225522049489,0.403420487469947));
#79250=CARTESIAN_POINT('Ctrl Pts',(1.45801595739492,3.90037588457939,0.518622851739805));
#79251=CARTESIAN_POINT('Ctrl Pts',(1.463859802015,3.88339795179009,0.633356390142418));
#79252=CARTESIAN_POINT('Ctrl Pts',(1.4697036466351,3.86138234699156,0.747138119989815));
#79253=CARTESIAN_POINT('Ctrl Pts',(1.47554655267681,3.83937027811365,0.860901575382912));
#79254=CARTESIAN_POINT('Ctrl Pts',(1.48138945871854,3.81232222460642,0.973713119198366));
#79255=CARTESIAN_POINT('Ctrl Pts',(1.48723236476025,3.78035043649894,1.08509887902544));
#79256=CARTESIAN_POINT('Ctrl Pts',(1.4930757575243,3.7483759850963,1.19649391744383));
#79257=CARTESIAN_POINT('Ctrl Pts',(1.49891915028835,3.71147709824281,1.30646253723765));
#79258=CARTESIAN_POINT('Ctrl Pts',(1.5047625430524,3.66981600672843,1.41454567856955));
#79259=CARTESIAN_POINT('Ctrl Pts',(1.51060784785759,3.62814128311296,1.522664186241));
#79260=CARTESIAN_POINT('Ctrl Pts',(1.51645315266278,3.58170140563401,1.62889560209278));
#79261=CARTESIAN_POINT('Ctrl Pts',(1.52229845746796,3.53070659277404,1.73280118759825));
#79262=CARTESIAN_POINT('Ctrl Pts',(1.52815041052508,3.47965378013918,1.83682495180135));
#79263=CARTESIAN_POINT('Ctrl Pts',(1.5340023635822,3.42403587471379,1.9385172333325));
#79264=CARTESIAN_POINT('Ctrl Pts',(1.53985431663932,3.36410891449219,2.03746416199995));
#79265=CARTESIAN_POINT('Ctrl Pts',(1.54571020270278,3.30414167829566,2.13647759135431));
#79266=CARTESIAN_POINT('Ctrl Pts',(1.55156608876624,3.23985985082548,2.23274165019659));
#79267=CARTESIAN_POINT('Ctrl Pts',(1.5574219748297,3.17156160540978,2.32587316573594));
#79268=CARTESIAN_POINT('Ctrl Pts',(1.56328654009602,3.10316213290043,2.41914271458182));
#79269=CARTESIAN_POINT('Ctrl Pts',(1.56915110536234,3.03073462069176,2.50927013216155));
#79270=CARTESIAN_POINT('Ctrl Pts',(1.57501567062866,2.95461616807978,2.59590683563983));
#79271=CARTESIAN_POINT('Ctrl Pts',(1.57668914498518,2.93289549950179,2.62062892415276));
#79272=CARTESIAN_POINT('Ctrl Pts',(1.57836261934168,2.91087450860319,2.64506701647413));
#79273=CARTESIAN_POINT('Ctrl Pts',(1.5800360936982,2.88856153455991,2.6692136034909));
#79274=CARTESIAN_POINT('Ctrl Pts',(1.58591017028305,2.81024057442334,2.75397074413504));
#79275=CARTESIAN_POINT('Ctrl Pts',(1.59178424686792,2.72805535120082,2.83541916327497));
#79276=CARTESIAN_POINT('Ctrl Pts',(1.59765832345277,2.64231648922465,2.91318598286678));
#79277=CARTESIAN_POINT('Ctrl Pts',(1.60352479877662,2.55668857634133,2.99085216946804));
#79278=CARTESIAN_POINT('Ctrl Pts',(1.60939127410046,2.46751647285204,3.0648459558061));
#79279=CARTESIAN_POINT('Ctrl Pts',(1.61525774942431,2.37514960216785,3.13482908103806));
#79280=CARTESIAN_POINT('Ctrl Pts',(1.62111819982907,2.28287759303025,3.20474033301669));
#79281=CARTESIAN_POINT('Ctrl Pts',(1.62697865023383,2.18741767027199,3.27064886890375));
#79282=CARTESIAN_POINT('Ctrl Pts',(1.63283910063859,2.08915399344872,3.33225518105341));
#79283=CARTESIAN_POINT('Ctrl Pts',(1.63892427613023,1.98712229338737,3.39622385153625));
#79284=CARTESIAN_POINT('Ctrl Pts',(1.64500945162186,1.88206784372643,3.45555343979431));
#79285=CARTESIAN_POINT('Ctrl Pts',(1.6510946271135,1.77445623100745,3.50995642198572));
#79286=CARTESIAN_POINT('Ctrl Pts',(1.6569482966211,1.67093862220514,3.56228968310762));
#79287=CARTESIAN_POINT('Ctrl Pts',(1.6628019661287,1.56505526984246,3.61006414650832));
#79288=CARTESIAN_POINT('Ctrl Pts',(1.66865563563629,1.45724693615371,3.65306999208482));
#79289=CARTESIAN_POINT('Ctrl Pts',(1.67450841228232,1.34945504649512,3.69606927796973));
#79290=CARTESIAN_POINT('Ctrl Pts',(1.68036118892835,1.23973914291635,3.73430123926779));
#79291=CARTESIAN_POINT('Ctrl Pts',(1.68621396557439,1.12856000089635,3.76760418892123));
#79292=CARTESIAN_POINT('Ctrl Pts',(1.69206726446448,1.01737093834614,3.80091011020148));
#79293=CARTESIAN_POINT('Ctrl Pts',(1.69792056335458,0.904718773547644,3.82928602697692));
#79294=CARTESIAN_POINT('Ctrl Pts',(1.70377386224468,0.79107878826895,3.85262032268311));
#79295=CARTESIAN_POINT('Ctrl Pts',(1.70962909851816,0.677401189291951,3.87596234180775));
#79296=CARTESIAN_POINT('Ctrl Pts',(1.71548433479164,0.562735524128474,3.89425933861837));
#79297=CARTESIAN_POINT('Ctrl Pts',(1.72133957106511,0.447565888134444,3.90745105865428));
#79298=CARTESIAN_POINT('Ctrl Pts',(1.72720144344763,0.332265723118647,3.9206577296996));
#79299=CARTESIAN_POINT('Ctrl Pts',(1.73306331583015,0.216460857861962,3.9287475279576));
#79300=CARTESIAN_POINT('Ctrl Pts',(1.73892518821268,0.100639218276715,3.93171219034973));
#79301=CARTESIAN_POINT('Ctrl Pts',(1.7447909989767,-0.0152602377079235,
3.93467884459202));
#79302=CARTESIAN_POINT('Ctrl Pts',(1.75065680974071,-0.131176078438516,
3.93251351403517));
#79303=CARTESIAN_POINT('Ctrl Pts',(1.75652262050473,-0.246623416349175,
3.92525997744204));
#79304=CARTESIAN_POINT('Ctrl Pts',(1.76239704144614,-0.362240214561096,
3.91799579368701));
#79305=CARTESIAN_POINT('Ctrl Pts',(1.76827146238757,-0.47738672824052,3.9056285415912));
#79306=CARTESIAN_POINT('Ctrl Pts',(1.77414588332898,-0.591586112199691,
3.88825344748159));
#79307=CARTESIAN_POINT('Ctrl Pts',(1.77572502636527,-0.622284825098546,
3.88358273029232));
#79308=CARTESIAN_POINT('Ctrl Pts',(1.77730416940156,-0.652915171796896,
3.87855041553838));
#79309=CARTESIAN_POINT('Ctrl Pts',(1.77888331243784,-0.68346807235756,3.87315896834455));
#79310=CARTESIAN_POINT('Ctrl Pts',(1.78475698171083,-0.79711049049179,3.85310532089681));
#79311=CARTESIAN_POINT('Ctrl Pts',(1.79063065098381,-0.910058892662766,
3.82801245027434));
#79312=CARTESIAN_POINT('Ctrl Pts',(1.79650432025679,-1.02183170271352,3.79794009580583));
#79313=CARTESIAN_POINT('Ctrl Pts',(1.80237040603293,-1.13346020284273,3.76790656776668));
#79314=CARTESIAN_POINT('Ctrl Pts',(1.80823649180907,-1.2439157339494,3.73290644742008));
#79315=CARTESIAN_POINT('Ctrl Pts',(1.81410257758521,-1.35272486981782,3.69305082913522));
#79316=CARTESIAN_POINT('Ctrl Pts',(1.81996265661022,-1.46142258736996,3.65323602218342));
#79317=CARTESIAN_POINT('Ctrl Pts',(1.82582273563522,-1.56847687738249,3.60857574810993));
#79318=CARTESIAN_POINT('Ctrl Pts',(1.83168281466022,-1.67342814022944,3.55923127367248));
#79319=CARTESIAN_POINT('Ctrl Pts',(1.83776813618178,-1.7824133903927,3.50799015713077));
#79320=CARTESIAN_POINT('Ctrl Pts',(1.84385345770332,-1.8891302631675,3.45169764004533));
#79321=CARTESIAN_POINT('Ctrl Pts',(1.84993877922487,-1.99308510711857,3.39059003062626));
#79322=CARTESIAN_POINT('Ctrl Pts',(1.85579212552627,-2.09307714520534,3.33181187103131));
#79323=CARTESIAN_POINT('Ctrl Pts',(1.86164547182768,-2.19051349141098,3.26857923608651));
#79324=CARTESIAN_POINT('Ctrl Pts',(1.86749881812908,-2.28497940652602,3.20114949850081));
#79325=CARTESIAN_POINT('Ctrl Pts',(1.87335129001247,-2.37943120959433,3.1337298340892));
#79326=CARTESIAN_POINT('Ctrl Pts',(1.87920376189587,-2.47091312770396,3.06211455368878));
#79327=CARTESIAN_POINT('Ctrl Pts',(1.88505623377926,-2.55904010084445,2.98660388439278));
#79328=CARTESIAN_POINT('Ctrl Pts',(1.89090924677398,-2.64717522208095,2.91108623348647));
#79329=CARTESIAN_POINT('Ctrl Pts',(1.8967622597687,-2.73195446793767,2.83167274653416));
#79330=CARTESIAN_POINT('Ctrl Pts',(1.90261527276342,-2.81302706473549,2.74870291829903));
#79331=CARTESIAN_POINT('Ctrl Pts',(1.90847024244689,-2.89412676446951,2.66570535287465));
#79332=CARTESIAN_POINT('Ctrl Pts',(1.91432521213035,-2.97151706253956,2.57914937741913));
#79333=CARTESIAN_POINT('Ctrl Pts',(1.92018018181382,-3.04488563559911,2.48940966217338));
#79334=CARTESIAN_POINT('Ctrl Pts',(1.92604181781465,-3.1183377442224,2.39956777160393));
#79335=CARTESIAN_POINT('Ctrl Pts',(1.93190345381548,-3.18775872655857,2.30653522604996));
#79336=CARTESIAN_POINT('Ctrl Pts',(1.93776508981632,-3.25287793121025,2.21071802015664));
#79337=CARTESIAN_POINT('Ctrl Pts',(1.94363068151742,-3.3180410812818,2.11483615242715));
#79338=CARTESIAN_POINT('Ctrl Pts',(1.94949627321853,-3.3788964567285,2.01616623321353));
#79339=CARTESIAN_POINT('Ctrl Pts',(1.95536186491963,-3.43521883526877,1.91513982617841));
#79340=CARTESIAN_POINT('Ctrl Pts',(1.96123609408465,-3.49162415216157,1.81396465121162));
#79341=CARTESIAN_POINT('Ctrl Pts',(1.96711032324967,-3.54348296555399,1.71042643083464));
#79342=CARTESIAN_POINT('Ctrl Pts',(1.97298455241469,-3.59061768585969,1.60497776744466));
#79343=CARTESIAN_POINT('Ctrl Pts',(1.97456654533562,-3.6033115716035,1.57657931135477));
#79344=CARTESIAN_POINT('Ctrl Pts',(1.97614853825655,-3.61566310577279,1.548042382819));
#79345=CARTESIAN_POINT('Ctrl Pts',(1.97773053117749,-3.62766943983772,1.51937600193879));
#79346=CARTESIAN_POINT('Ctrl Pts',(1.98430602295599,-3.6775732983755,1.40022530960424));
#79347=CARTESIAN_POINT('Ctrl Pts',(1.9908815147345,-3.72165215810053,1.2784965980874));
#79348=CARTESIAN_POINT('Ctrl Pts',(1.99745700651301,-3.75966149616237,1.15474431554094));
#79349=CARTESIAN_POINT('Ctrl Pts',(2.00397687500376,-3.79734930628078,1.03203887618966));
#79350=CARTESIAN_POINT('Ctrl Pts',(2.0104967434945,-3.82906975507951,0.907344193337815));
#79351=CARTESIAN_POINT('Ctrl Pts',(2.01701661198525,-3.854630735699,0.781223970065293));
#79352=CARTESIAN_POINT('Ctrl Pts',(2.02361991540764,-3.88051882087186,0.65348978291872));
#79353=CARTESIAN_POINT('Ctrl Pts',(2.03022321883004,-3.90008851960739,0.524293517975706));
#79354=CARTESIAN_POINT('Ctrl Pts',(2.03682652225243,-3.91319083428004,0.394241670180517));
#79355=CARTESIAN_POINT('Ctrl Pts',(2.04342982567482,-3.92629314895268,0.26418982238533));
#79356=CARTESIAN_POINT('Ctrl Pts',(2.05003312909721,-3.93292792584975,0.133282638315857));
#79357=CARTESIAN_POINT('Ctrl Pts',(2.0566364325196,-3.9329994155864,0.00214406087016673));
#79358=CARTESIAN_POINT('',(3.30663650988561,-3.93223110072523,-0.00324727255823224));
#79359=CARTESIAN_POINT('Ctrl Pts',(2.0566364779651,-3.92760797316549,0.00214022045425887));
#79360=CARTESIAN_POINT('Ctrl Pts',(2.09661690194911,-3.92376833228284,-0.790766574382641));
#79361=CARTESIAN_POINT('Ctrl Pts',(2.20287973217967,-3.30533753684168,-2.90375943243531));
#79362=CARTESIAN_POINT('Ctrl Pts',(2.37542496865678,0.147023520660857,-4.64930955531007));
#79363=CARTESIAN_POINT('Ctrl Pts',(2.57427218739642,3.9905524730503,-2.3902958242871));
#79364=CARTESIAN_POINT('Ctrl Pts',(2.77311940613606,4.16846304929326,2.06445390521175));
#79365=CARTESIAN_POINT('Ctrl Pts',(2.97196662487571,0.517297643089777,4.62280760769746));
#79366=CARTESIAN_POINT('Ctrl Pts',(3.14980564881872,-3.17309355288368,3.11310308288762));
#79367=CARTESIAN_POINT('Ctrl Pts',(3.26136226651518,-3.9229062319681,0.893358099881881));
#79368=CARTESIAN_POINT('Ctrl Pts',(3.30663647796509,-3.92984741018714,-0.00324467181678128));
#79369=CARTESIAN_POINT('',(4.55663647792001,-3.93299992902536,-0.000747185703456276));
#79370=CARTESIAN_POINT('Ctrl Pts',(3.30663652016415,-3.93299865875662,-0.00324811000753884));
#79371=CARTESIAN_POINT('Ctrl Pts',(3.31356358509945,-3.93288527511355,-0.140539554911472));
#79372=CARTESIAN_POINT('Ctrl Pts',(3.32049065003477,-3.92557928781996,-0.27752307573409));
#79373=CARTESIAN_POINT('Ctrl Pts',(3.32741771497007,-3.91120026655955,-0.413523245857523));
#79374=CARTESIAN_POINT('Ctrl Pts',(3.33445827286756,-3.89658565955951,-0.55175164139948));
#79375=CARTESIAN_POINT('Ctrl Pts',(3.34149883076505,-3.87466438934153,-0.688964114611102));
#79376=CARTESIAN_POINT('Ctrl Pts',(3.34853938866253,-3.84561221477454,-0.824472979288515));
#79377=CARTESIAN_POINT('Ctrl Pts',(3.35557994656002,-3.81656004020754,-0.95998184396593));
#79378=CARTESIAN_POINT('Ctrl Pts',(3.36262050445751,-3.7803770898771,-1.09378708058283));
#79379=CARTESIAN_POINT('Ctrl Pts',(3.369661062355,-3.73728746254593,-1.22522300920975));
#79380=CARTESIAN_POINT('Ctrl Pts',(3.37553351744045,-3.70134685885581,-1.33485233102118));
#79381=CARTESIAN_POINT('Ctrl Pts',(3.3814059725259,-3.66051820663356,-1.44308243253663));
#79382=CARTESIAN_POINT('Ctrl Pts',(3.38727842761135,-3.61492857934629,-1.54944518012914));
#79383=CARTESIAN_POINT('Ctrl Pts',(3.39314327559298,-3.56939800828382,-1.65567014676781));
#79384=CARTESIAN_POINT('Ctrl Pts',(3.39900812357461,-3.51911888808148,-1.76003219348437));
#79385=CARTESIAN_POINT('Ctrl Pts',(3.40487297155624,-3.46426798301453,-1.862078500456));
#79386=CARTESIAN_POINT('Ctrl Pts',(3.41073179078696,-3.40947346175243,-1.96401990926685));
#79387=CARTESIAN_POINT('Ctrl Pts',(3.41659061001768,-3.35011669781919,-2.06364995128611));
#79388=CARTESIAN_POINT('Ctrl Pts',(3.4224494292484,-3.28642217370034,-2.16053657599466));
#79389=CARTESIAN_POINT('Ctrl Pts',(3.42853521474199,-3.2202601714881,-2.26117651587933));
#79390=CARTESIAN_POINT('Ctrl Pts',(3.43462100023558,-3.14941770805553,-2.35885576629735));
#79391=CARTESIAN_POINT('Ctrl Pts',(3.44070678572918,-3.0741986320021,-2.45311878452642));
#79392=CARTESIAN_POINT('Ctrl Pts',(3.44655882504513,-3.00186861136011,-2.54376129719758));
#79393=CARTESIAN_POINT('Ctrl Pts',(3.45241086436109,-2.92549225713851,-2.63124480923989));
#79394=CARTESIAN_POINT('Ctrl Pts',(3.45826290367704,-2.84538287023236,-2.71519526402582));
#79395=CARTESIAN_POINT('Ctrl Pts',(3.46411405332442,-2.76528566212415,-2.79913295606739));
#79396=CARTESIAN_POINT('Ctrl Pts',(3.46996520297179,-2.68145683503781,-2.87953835985712));
#79397=CARTESIAN_POINT('Ctrl Pts',(3.47581635261917,-2.59424791964966,-2.95607285623907));
#79398=CARTESIAN_POINT('Ctrl Pts',(3.4816680294769,-2.50703114641373,-3.03261424866392));
#79399=CARTESIAN_POINT('Ctrl Pts',(3.48751970633462,-2.41643399014157,-3.10528376766225));
#79400=CARTESIAN_POINT('Ctrl Pts',(3.49337138319235,-2.32284200753851,-3.17378228743159));
#79401=CARTESIAN_POINT('Ctrl Pts',(3.49922500417839,-2.22921893045997,-3.24230356476502));
#79402=CARTESIAN_POINT('Ctrl Pts',(3.50507862516442,-2.13259938197047,-3.30665084339127));
#79403=CARTESIAN_POINT('Ctrl Pts',(3.51093224615046,-2.03339830286724,-3.36656803613066));
#79404=CARTESIAN_POINT('Ctrl Pts',(3.5167925215223,-1.93408445215563,-3.42655334262703));
#79405=CARTESIAN_POINT('Ctrl Pts',(3.52265279689415,-1.83218356734116,-3.48209829748689));
#79406=CARTESIAN_POINT('Ctrl Pts',(3.52851307226599,-1.72813570276538,-3.53299249826936));
#79407=CARTESIAN_POINT('Ctrl Pts',(3.53437729470334,-1.62401775893387,-3.58392097777276));
#79408=CARTESIAN_POINT('Ctrl Pts',(3.54024151714069,-1.51775033401841,-3.63019230130826));
#79409=CARTESIAN_POINT('Ctrl Pts',(3.54610573957803,-1.4097923649181,-3.67164465707381));
#79410=CARTESIAN_POINT('Ctrl Pts',(3.55197859733777,-1.30167542301653,-3.7131580532347));
#79411=CARTESIAN_POINT('Ctrl Pts',(3.55785145509751,-1.19186335917039,-3.74983818867805));
#79412=CARTESIAN_POINT('Ctrl Pts',(3.56372431285725,-1.08082919488469,-3.78157338306225));
#79413=CARTESIAN_POINT('Ctrl Pts',(3.56531896893638,-1.05068010694269,-3.79019043505252));
#79414=CARTESIAN_POINT('Ctrl Pts',(3.56691362501551,-1.02044096452048,-3.79844319705715));
#79415=CARTESIAN_POINT('Ctrl Pts',(3.56850828109464,-0.990121329568143,
-3.80633008982855));
#79416=CARTESIAN_POINT('Ctrl Pts',(3.57438072828865,-0.878466874711392,
-3.83537419653658));
#79417=CARTESIAN_POINT('Ctrl Pts',(3.58025317548266,-0.765346438429972,
-3.85954987543601));
#79418=CARTESIAN_POINT('Ctrl Pts',(3.58612562267666,-0.651222527430752,
-3.87871089664681));
#79419=CARTESIAN_POINT('Ctrl Pts',(3.59199046272136,-0.537246452180766,
-3.89784709673202));
#79420=CARTESIAN_POINT('Ctrl Pts',(3.59785530276606,-0.422269891140721,
-3.91198148949371));
#79421=CARTESIAN_POINT('Ctrl Pts',(3.60372014281076,-0.306769337349473,
-3.92101792570018));
#79422=CARTESIAN_POINT('Ctrl Pts',(3.60957895406889,-0.191387512829826,
-3.93004507286471));
#79423=CARTESIAN_POINT('Ctrl Pts',(3.61543776532703,-0.0754831765679285,
-3.93398465499945));
#79424=CARTESIAN_POINT('Ctrl Pts',(3.62129657658517,0.040458847897597,-3.93279189401458));
#79425=CARTESIAN_POINT('Ctrl Pts',(3.62738236505388,0.160892602194006,-3.93155292407208));
#79426=CARTESIAN_POINT('Ctrl Pts',(3.63346815352259,0.281366575838322,-3.9247758271046));
#79427=CARTESIAN_POINT('Ctrl Pts',(3.63955394199131,0.401333266375885,-3.91246988605664));
#79428=CARTESIAN_POINT('Ctrl Pts',(3.64540597329665,0.516691996347188,-3.90063662030567));
#79429=CARTESIAN_POINT('Ctrl Pts',(3.651258004602,0.631581244978,-3.88369145141041));
#79430=CARTESIAN_POINT('Ctrl Pts',(3.65711003590734,0.745516948544496,-3.8616956741091));
#79431=CARTESIAN_POINT('Ctrl Pts',(3.66296117754383,0.859435330766979,-3.83970324076769));
#79432=CARTESIAN_POINT('Ctrl Pts',(3.66881231918033,0.972400050410675,-3.81266180405009));
#79433=CARTESIAN_POINT('Ctrl Pts',(3.67466346081681,1.08393618279765,-3.78068397933788));
#79434=CARTESIAN_POINT('Ctrl Pts',(3.68051512967199,1.19548236517773,-3.74870327325519));
#79435=CARTESIAN_POINT('Ctrl Pts',(3.68636679852716,1.30559930703886,-3.71178540889549));
#79436=CARTESIAN_POINT('Ctrl Pts',(3.69221846738233,1.41382690762245,-3.67009297910594));
#79437=CARTESIAN_POINT('Ctrl Pts',(3.69807208038277,1.52209046549996,-3.62838669751755));
#79438=CARTESIAN_POINT('Ctrl Pts',(3.7039256933832,1.62846304841473,-3.58190284477065));
#79439=CARTESIAN_POINT('Ctrl Pts',(3.70977930638364,1.73250487179925,-3.53085200329777));
#79440=CARTESIAN_POINT('Ctrl Pts',(3.7156395738357,1.83666497107257,-3.47974312666698));
#79441=CARTESIAN_POINT('Ctrl Pts',(3.72149984128775,1.93848865092629,-3.42405708083812));
#79442=CARTESIAN_POINT('Ctrl Pts',(3.72736010873981,2.03756097805657,-3.36405027618512));
#79443=CARTESIAN_POINT('Ctrl Pts',(3.73322432328592,2.13670003384666,-3.30400305486108));
#79444=CARTESIAN_POINT('Ctrl Pts',(3.73908853783204,2.2330837040564,-3.23962950897484));
#79445=CARTESIAN_POINT('Ctrl Pts',(3.74495275237815,2.32632772029525,-3.17122820651336));
#79446=CARTESIAN_POINT('Ctrl Pts',(3.75082560235005,2.41970904422912,-3.10272617881978));
#79447=CARTESIAN_POINT('Ctrl Pts',(3.75669845232195,2.50994116598464,-3.03018481522649));
#79448=CARTESIAN_POINT('Ctrl Pts',(3.76257130229385,2.59667437253834,-2.95394163838804));
#79449=CARTESIAN_POINT('Ctrl Pts',(3.76416603480732,2.62022618556797,-2.93323832166502));
#79450=CARTESIAN_POINT('Ctrl Pts',(3.7657607673208,2.64352022341602,-2.91226224876372));
#79451=CARTESIAN_POINT('Ctrl Pts',(3.76735549983428,2.66654998642768,-2.89102061042161));
#79452=CARTESIAN_POINT('Ctrl Pts',(3.77322794292317,2.75135478691542,-2.81280040030813));
#79453=CARTESIAN_POINT('Ctrl Pts',(3.77910038601206,2.83285690181505,-2.73071458870866));
#79454=CARTESIAN_POINT('Ctrl Pts',(3.78497282910096,2.91068323909851,-2.6450731713189));
#79455=CARTESIAN_POINT('Ctrl Pts',(3.79083766495501,2.98840875918961,-2.55954269487216));
#79456=CARTESIAN_POINT('Ctrl Pts',(3.79670250080907,3.06246769545385,-2.47046607537385));
#79457=CARTESIAN_POINT('Ctrl Pts',(3.80256733666312,3.13252152151712,-2.37819215313482));
#79458=CARTESIAN_POINT('Ctrl Pts',(3.80842614365053,3.20250333445235,-2.28601308558327));
#79459=CARTESIAN_POINT('Ctrl Pts',(3.81428495063794,3.26848797793113,-2.19064358002084));
#79460=CARTESIAN_POINT('Ctrl Pts',(3.82014375762535,3.33017563498916,-2.0924672614224));
#79461=CARTESIAN_POINT('Ctrl Pts',(3.82622954766487,3.39425320738438,-1.9904873765879));
#79462=CARTESIAN_POINT('Ctrl Pts',(3.8323153377044,3.45369380440183,-1.88547913208565));
#79463=CARTESIAN_POINT('Ctrl Pts',(3.83840112774392,3.50820919364773,-1.77790811168787));
#79464=CARTESIAN_POINT('Ctrl Pts',(3.84425315460459,3.56063057527853,-1.67446903529696));
#79465=CARTESIAN_POINT('Ctrl Pts',(3.85010518146526,3.60849793277353,-1.5686608332186));
#79466=CARTESIAN_POINT('Ctrl Pts',(3.85595720832593,3.65160108937571,-1.46092384608854));
#79467=CARTESIAN_POINT('Ctrl Pts',(3.86180834546086,3.69469769269496,-1.35320323898755));
#79468=CARTESIAN_POINT('Ctrl Pts',(3.86765948259579,3.73303138183604,-1.24355481358343));
#79469=CARTESIAN_POINT('Ctrl Pts',(3.87351061973073,3.76644009297464,-1.13243897232177));
#79470=CARTESIAN_POINT('Ctrl Pts',(3.87936228403202,3.79985181411765,-1.02131311992348));
#79471=CARTESIAN_POINT('Ctrl Pts',(3.88521394833331,3.82833755615214,-0.908719984724476));
#79472=CARTESIAN_POINT('Ctrl Pts',(3.89106561263461,3.85178531217261,-0.795134522537734));
#79473=CARTESIAN_POINT('Ctrl Pts',(3.89691922103335,3.87524085823717,-0.681511323871822));
#79474=CARTESIAN_POINT('Ctrl Pts',(3.9027728294321,3.89365500657552,-0.566895547275909));
#79475=CARTESIAN_POINT('Ctrl Pts',(3.90862643783084,3.90696710471404,-0.451771006907689));
#79476=CARTESIAN_POINT('Ctrl Pts',(3.91448670063306,3.9202943360945,-0.336515592540206));
#79477=CARTESIAN_POINT('Ctrl Pts',(3.92034696343528,3.92850789310142,-0.220750670868103));
#79478=CARTESIAN_POINT('Ctrl Pts',(3.9262072262375,3.93159911146462,-0.104963930617245));
#79479=CARTESIAN_POINT('Ctrl Pts',(3.93207143609996,3.93469241185476,0.0109007954259721));
#79480=CARTESIAN_POINT('Ctrl Pts',(3.93793564596241,3.9326565111082,0.126786957026716));
#79481=CARTESIAN_POINT('Ctrl Pts',(3.94379985582487,3.92553478914966,0.242209865975237));
#79482=CARTESIAN_POINT('Ctrl Pts',(3.94967270109944,3.91840258001458,0.357802742303846));
#79483=CARTESIAN_POINT('Ctrl Pts',(3.95554554637401,3.906169646254,0.472930595011592));
#79484=CARTESIAN_POINT('Ctrl Pts',(3.96141839164858,3.88893082125202,0.587116740960479));
#79485=CARTESIAN_POINT('Ctrl Pts',(3.96301316729036,3.88424960509175,0.618124076532006));
#79486=CARTESIAN_POINT('Ctrl Pts',(3.96460794293215,3.87919954224919,0.649062047781664));
#79487=CARTESIAN_POINT('Ctrl Pts',(3.96620271857393,3.87378316741701,0.679921298266663));
#79488=CARTESIAN_POINT('Ctrl Pts',(3.97207516613946,3.85383843264438,0.793554417331757));
#79489=CARTESIAN_POINT('Ctrl Pts',(3.977947613705,3.82885611548635,0.906499453759549));
#79490=CARTESIAN_POINT('Ctrl Pts',(3.98382006127053,3.79889525322836,1.01827494076947));
#79491=CARTESIAN_POINT('Ctrl Pts',(3.989684901662,3.76897320229934,1.12990563370905));
#79492=CARTESIAN_POINT('Ctrl Pts',(3.99554974205346,3.73408553749332,1.24036939451578));
#79493=CARTESIAN_POINT('Ctrl Pts',(4.00141458244493,3.69434266252296,1.34919282975518));
#79494=CARTESIAN_POINT('Ctrl Pts',(4.00727339402476,3.65464064157266,1.45790439903596));
#79495=CARTESIAN_POINT('Ctrl Pts',(4.0131322056046,3.6100934786871,1.56497861072361));
#79496=CARTESIAN_POINT('Ctrl Pts',(4.01899101718443,3.56086176930219,1.66995582573974));
#79497=CARTESIAN_POINT('Ctrl Pts',(4.02507680552314,3.50972276973085,1.77899997270889));
#79498=CARTESIAN_POINT('Ctrl Pts',(4.03116259386185,3.45352903145065,1.88578091814643));
#79499=CARTESIAN_POINT('Ctrl Pts',(4.03724838220057,3.39251635754362,1.98980445365844));
#79500=CARTESIAN_POINT('Ctrl Pts',(4.04310041376238,3.33384719695139,2.08983241702266));
#79501=CARTESIAN_POINT('Ctrl Pts',(4.04895244532419,3.2707226938025,2.18731049930099));
#79502=CARTESIAN_POINT('Ctrl Pts',(4.054804476886,3.20339962252632,2.28182380090976));
#79503=CARTESIAN_POINT('Ctrl Pts',(4.0606556187543,3.13608678648191,2.37632273351351));
#79504=CARTESIAN_POINT('Ctrl Pts',(4.0665067606226,3.06457689124168,2.46785744508208));
#79505=CARTESIAN_POINT('Ctrl Pts',(4.07235790249091,2.98916960253729,2.55604266147243));
#79506=CARTESIAN_POINT('Ctrl Pts',(4.07820957155287,2.91375551956173,2.64423582343785));
#79507=CARTESIAN_POINT('Ctrl Pts',(4.08406124061483,2.83444361370559,2.72907857610939));
#79508=CARTESIAN_POINT('Ctrl Pts',(4.0899129096768,2.75157285938732,2.81021988454339));
#79509=CARTESIAN_POINT('Ctrl Pts',(4.09576652285861,2.66867457263748,2.8913881508293));
#79510=CARTESIAN_POINT('Ctrl Pts',(4.10162013604041,2.5822153815549,2.96885223857184));
#79511=CARTESIAN_POINT('Ctrl Pts',(4.10747374922222,2.49256948012377,3.04229952285365));
#79512=CARTESIAN_POINT('Ctrl Pts',(4.11333401681674,2.40282166884527,3.11583030232498));
#79513=CARTESIAN_POINT('Ctrl Pts',(4.11919428441125,2.30988023643114,3.18533490199171));
#79514=CARTESIAN_POINT('Ctrl Pts',(4.12505455200577,2.21415074672552,3.25054233486888));
#79515=CARTESIAN_POINT('Ctrl Pts',(4.13091876667184,2.11835678024655,3.31579368696972));
#79516=CARTESIAN_POINT('Ctrl Pts',(4.13678298133791,2.01977136804527,3.37674189236581));
#79517=CARTESIAN_POINT('Ctrl Pts',(4.14264719600398,1.91882569072704,3.43316136652588));
#79518=CARTESIAN_POINT('Ctrl Pts',(4.14852004606164,1.81773136512377,3.48966392158946));
#79519=CARTESIAN_POINT('Ctrl Pts',(4.1543928961193,1.71427020574622,3.5416242509723));
#79520=CARTESIAN_POINT('Ctrl Pts',(4.16026574617696,1.60889448067025,3.58886438167686));
#79521=CARTESIAN_POINT('Ctrl Pts',(4.16186047655583,1.58028045710011,3.60169210089267));
#79522=CARTESIAN_POINT('Ctrl Pts',(4.1634552069347,1.55152535239075,3.61417205672211));
#79523=CARTESIAN_POINT('Ctrl Pts',(4.16504993731357,1.52263840700106,3.62630132249449));
#79524=CARTESIAN_POINT('Ctrl Pts',(4.17092238347021,1.41626491987186,3.67096621451127));
#79525=CARTESIAN_POINT('Ctrl Pts',(4.17679482962686,1.30774638193382,3.71102139669462));
#79526=CARTESIAN_POINT('Ctrl Pts',(4.18266727578351,1.19751972912854,3.74625619763891));
#79527=CARTESIAN_POINT('Ctrl Pts',(4.18853211475511,1.08743586427276,3.78144535531226));
#79528=CARTESIAN_POINT('Ctrl Pts',(4.19439695372671,0.975648674918339,3.81182642481333));
#79529=CARTESIAN_POINT('Ctrl Pts',(4.20026179269831,0.862616080010135,3.83723630996424));
#79530=CARTESIAN_POINT('Ctrl Pts',(4.20612060284905,0.749699678107125,3.86262007476535));
#79531=CARTESIAN_POINT('Ctrl Pts',(4.2119794129998,0.635540817963619,3.88304272952699));
#79532=CARTESIAN_POINT('Ctrl Pts',(4.21783822315054,0.520612987435137,3.89839083691128));
#79533=CARTESIAN_POINT('Ctrl Pts',(4.22392401202149,0.401232687682143,3.91433355202));
#79534=CARTESIAN_POINT('Ctrl Pts',(4.23000980089243,0.281023063252718,3.92480043865746));
#79535=CARTESIAN_POINT('Ctrl Pts',(4.23609558976338,0.160527348097331,3.92972263277103));
#79536=CARTESIAN_POINT('Ctrl Pts',(4.24194761988218,0.0446599446712767,
3.9344557624957));
#79537=CARTESIAN_POINT('Ctrl Pts',(4.24779965000098,-0.0714715258643642,
3.9340622739106));
#79538=CARTESIAN_POINT('Ctrl Pts',(4.25365168011978,-0.187379205918145,
3.9285338274208));
#79539=CARTESIAN_POINT('Ctrl Pts',(4.25950282054239,-0.303269264288719,
3.92300622143209));
#79540=CARTESIAN_POINT('Ctrl Pts',(4.265353960965,-0.418935187051956,3.91234522946963));
#79541=CARTESIAN_POINT('Ctrl Pts',(4.27120510138761,-0.533890846026035,
3.89659461126374));
#79542=CARTESIAN_POINT('Ctrl Pts',(4.27705676900275,-0.648856862598774,
3.8808425739143));
#79543=CARTESIAN_POINT('Ctrl Pts',(4.28290843661789,-0.763112078610132,
3.86000005482292));
#79544=CARTESIAN_POINT('Ctrl Pts',(4.28876010423303,-0.876177913582972,
3.8341623940242));
#79545=CARTESIAN_POINT('Ctrl Pts',(4.29461371596842,-0.9892813128185,3.80831614908795));
#79546=CARTESIAN_POINT('Ctrl Pts',(4.3004673277038,-1.10119414252346,3.77747155456045));
#79547=CARTESIAN_POINT('Ctrl Pts',(4.30632093943919,-1.21145108949488,3.74177434618413));
#79548=CARTESIAN_POINT('Ctrl Pts',(4.31218120559523,-1.32183337721955,3.70603655700896));
#79549=CARTESIAN_POINT('Ctrl Pts',(4.31804147175126,-1.43055563147713,3.66543527067302));
#79550=CARTESIAN_POINT('Ctrl Pts',(4.3239017379073,-1.53717060325931,3.62016512558135));
#79551=CARTESIAN_POINT('Ctrl Pts',(4.32976595113772,-1.64385738359312,3.5748644896168));
#79552=CARTESIAN_POINT('Ctrl Pts',(4.33563016436815,-1.74843368325179,3.52488891111368));
#79553=CARTESIAN_POINT('Ctrl Pts',(4.34149437759857,-1.85047659493403,3.4704791270949));
#79554=CARTESIAN_POINT('Ctrl Pts',(4.34736722623593,-1.95266977094539,3.41598922139439));
#79555=CARTESIAN_POINT('Ctrl Pts',(4.35324007487329,-2.05232175906285,3.35705228796));
#79556=CARTESIAN_POINT('Ctrl Pts',(4.35911292351064,-2.14903830102412,3.29395254682446));
#79557=CARTESIAN_POINT('Ctrl Pts',(4.3607076676915,-2.17530121907452,3.27681811152685));
#79558=CARTESIAN_POINT('Ctrl Pts',(4.36230241187236,-2.20134787576329,3.25937695296744));
#79559=CARTESIAN_POINT('Ctrl Pts',(4.36389715605321,-2.22717081254393,3.24163526198621));
#79560=CARTESIAN_POINT('Ctrl Pts',(4.36974003646156,-2.32178180608944,3.17663262401477));
#79561=CARTESIAN_POINT('Ctrl Pts',(4.37558291686992,-2.41371090712612,3.10737017371693));
#79562=CARTESIAN_POINT('Ctrl Pts',(4.38142579727827,-2.50254700172264,3.03409747769729));
#79563=CARTESIAN_POINT('Ctrl Pts',(4.38726109196053,-2.59126776171811,2.96091991054617));
#79564=CARTESIAN_POINT('Ctrl Pts',(4.39309638664279,-2.67690317974983,2.88374271258626));
#79565=CARTESIAN_POINT('Ctrl Pts',(4.39893168132505,-2.75907060592688,2.80285896746702));
#79566=CARTESIAN_POINT('Ctrl Pts',(4.40476100216875,-2.84115391382613,2.72205802646686));
#79567=CARTESIAN_POINT('Ctrl Pts',(4.41059032301245,-2.91977599414055,2.6375583757563));
#79568=CARTESIAN_POINT('Ctrl Pts',(4.41641964385614,-2.99458740595752,2.54969317136016));
#79569=CARTESIAN_POINT('Ctrl Pts',(4.42226201194214,-3.06956626140006,2.46163130621363));
#79570=CARTESIAN_POINT('Ctrl Pts',(4.42810438002813,-3.1407170507501,2.37018908122731));
#79571=CARTESIAN_POINT('Ctrl Pts',(4.43394674811412,-3.20772511407505,2.27573913103681));
#79572=CARTESIAN_POINT('Ctrl Pts',(4.43976956158102,-3.27450889896778,2.1816053082749));
#79573=CARTESIAN_POINT('Ctrl Pts',(4.44559237504791,-3.33717740148251,2.08448420439446));
#79574=CARTESIAN_POINT('Ctrl Pts',(4.4514151885148,-3.39546011366069,1.98477696896638));
#79575=CARTESIAN_POINT('Ctrl Pts',(4.4572371989607,-3.45373478810213,1.88508348410822));
#79576=CARTESIAN_POINT('Ctrl Pts',(4.4630592094066,-3.50762466383906,1.78280493759554));
#79577=CARTESIAN_POINT('Ctrl Pts',(4.46888121985249,-3.55690388340501,1.6783693765731));
#79578=CARTESIAN_POINT('Ctrl Pts',(4.47470387391394,-3.60618855072346,1.57392227033761));
#79579=CARTESIAN_POINT('Ctrl Pts',(4.48052652797539,-3.65086137070472,1.46731805383295));
#79580=CARTESIAN_POINT('Ctrl Pts',(4.48634918203684,-3.69074389137489,1.35900644894677));
#79581=CARTESIAN_POINT('Ctrl Pts',(4.49220645669377,-3.73086354731027,1.25005084010303));
#79582=CARTESIAN_POINT('Ctrl Pts',(4.4980637313507,-3.76613559788889,1.13936787157651));
#79583=CARTESIAN_POINT('Ctrl Pts',(4.50392100600763,-3.79642909718072,1.02743131647794));
#79584=CARTESIAN_POINT('Ctrl Pts',(4.50975234755442,-3.82658847186685,0.915990360985462));
#79585=CARTESIAN_POINT('Ctrl Pts',(4.5155836891012,-3.85181325390274,0.803307319074836));
#79586=CARTESIAN_POINT('Ctrl Pts',(4.52141503064799,-3.87202571242438,0.689859320676657));
#79587=CARTESIAN_POINT('Ctrl Pts',(4.52728527185999,-3.89237300404805,0.57565453430403));
#79588=CARTESIAN_POINT('Ctrl Pts',(4.53315551307199,-3.90764080592582,0.460674975547904));
#79589=CARTESIAN_POINT('Ctrl Pts',(4.539025754284,-3.91780300444119,0.345410796576432));
#79590=CARTESIAN_POINT('Ctrl Pts',(4.544895995496,-3.92796520295657,0.230146617604964));
#79591=CARTESIAN_POINT('Ctrl Pts',(4.550766236708,-3.93302184218556,0.114598245955288));
#79592=CARTESIAN_POINT('Ctrl Pts',(4.55663647792001,-3.93299992902536,-0.000747185703453174));
#79593=CARTESIAN_POINT('',(5.8066364641403,-3.93299833356548,0.00362052083856629));
#79594=CARTESIAN_POINT('Ctrl Pts',(4.5566364779651,-3.9329999290252,-0.000747186589495274));
#79595=CARTESIAN_POINT('Ctrl Pts',(4.55867244357435,-3.93299232891272,-0.0407522432060994));
#79596=CARTESIAN_POINT('Ctrl Pts',(4.5607084091836,-3.93237437087316,-0.0807508249110428));
#79597=CARTESIAN_POINT('Ctrl Pts',(4.56274437479285,-3.93114654101444,-0.120730580509577));
#79598=CARTESIAN_POINT('Ctrl Pts',(4.56861682114895,-3.92760504456334,-0.236046364340019));
#79599=CARTESIAN_POINT('Ctrl Pts',(4.57448926750506,-3.91897932797847,-0.351399251435818));
#79600=CARTESIAN_POINT('Ctrl Pts',(4.58036171386116,-3.90525918752465,-0.466304276470143));
#79601=CARTESIAN_POINT('Ctrl Pts',(4.58622655303069,-3.89155682018647,-0.581060453152324));
#79602=CARTESIAN_POINT('Ctrl Pts',(4.59209139220022,-3.8727732012637,-0.695369514851362));
#79603=CARTESIAN_POINT('Ctrl Pts',(4.59795623136976,-3.84895011973601,-0.808747164312879));
#79604=CARTESIAN_POINT('Ctrl Pts',(4.60381504171668,-3.82515152739351,-0.922008266036873));
#79605=CARTESIAN_POINT('Ctrl Pts',(4.6096738520636,-3.79632386097098,-1.03433945785894));
#79606=CARTESIAN_POINT('Ctrl Pts',(4.61553266241053,-3.76256054934362,-1.1452629010507));
#79607=CARTESIAN_POINT('Ctrl Pts',(4.62161845120728,-3.72748920013178,-1.26048367248725));
#79608=CARTESIAN_POINT('Ctrl Pts',(4.62770424000403,-3.68709209753127,-1.37418496181102));
#79609=CARTESIAN_POINT('Ctrl Pts',(4.63379002880078,-3.64153218184008,-1.48584399202038));
#79610=CARTESIAN_POINT('Ctrl Pts',(4.63964205911007,-3.59772224751303,-1.59321413760295));
#79611=CARTESIAN_POINT('Ctrl Pts',(4.64549408941937,-3.54913896763112,-1.69869560053916));
#79612=CARTESIAN_POINT('Ctrl Pts',(4.65134611972866,-3.4959773457879,-1.80184111334428));
#79613=CARTESIAN_POINT('Ctrl Pts',(4.65719726033934,-3.44282380623736,-1.90497094468233));
#79614=CARTESIAN_POINT('Ctrl Pts',(4.66304840095001,-3.38509349803426,-2.00576516469815));
#79615=CARTESIAN_POINT('Ctrl Pts',(4.66889954156068,-3.32302810139414,-2.10379971417074));
#79616=CARTESIAN_POINT('Ctrl Pts',(4.67475120936123,-3.26095711263941,-2.20184309659157));
#79617=CARTESIAN_POINT('Ctrl Pts',(4.68060287716179,-3.19455048010673,-2.2971259649112));
#79618=CARTESIAN_POINT('Ctrl Pts',(4.68645454496234,-3.12409367234671,-2.38925254554709));
#79619=CARTESIAN_POINT('Ctrl Pts',(4.69230815688027,-3.05361345650737,-2.48140973367678));
#79620=CARTESIAN_POINT('Ctrl Pts',(4.69816176879819,-2.97908064076982,-2.57040822083238));
#79621=CARTESIAN_POINT('Ctrl Pts',(4.70401538071611,-2.90082102925586,-2.65588523024377));
#79622=CARTESIAN_POINT('Ctrl Pts',(4.70987564704947,-2.82247245182242,-2.74145941034881));
#79623=CARTESIAN_POINT('Ctrl Pts',(4.71573591338282,-2.74038890171791,-2.82350381733387));
#79624=CARTESIAN_POINT('Ctrl Pts',(4.72159617971618,-2.65493316841876,-2.90169241499335));
#79625=CARTESIAN_POINT('Ctrl Pts',(4.72746039312111,-2.56941987802637,-2.97993367510427));
#79626=CARTESIAN_POINT('Ctrl Pts',(4.73332460652603,-2.4805301981218,-3.05431369010774));
#79627=CARTESIAN_POINT('Ctrl Pts',(4.73918881993096,-2.38865874586569,-3.12454771059738));
#79628=CARTESIAN_POINT('Ctrl Pts',(4.74506166873729,-2.29665200745726,-3.1948851548401));
#79629=CARTESIAN_POINT('Ctrl Pts',(4.75093451754363,-2.20165507135535,-3.26106418437028));
#79630=CARTESIAN_POINT('Ctrl Pts',(4.75680736634997,-2.10409021430103,-3.32284416879315));
#79631=CARTESIAN_POINT('Ctrl Pts',(4.75840210874414,-2.07759697075655,-3.33962021113981));
#79632=CARTESIAN_POINT('Ctrl Pts',(4.75999685113832,-2.05091450706119,-3.35607214973232));
#79633=CARTESIAN_POINT('Ctrl Pts',(4.76159159353249,-2.02405155226804,-3.3721957703789));
#79634=CARTESIAN_POINT('Ctrl Pts',(4.76746403965121,-1.92513196802138,-3.43156905463566));
#79635=CARTESIAN_POINT('Ctrl Pts',(4.77333648576992,-1.82343208240723,-3.48668551016047));
#79636=CARTESIAN_POINT('Ctrl Pts',(4.77920893188864,-1.71935433526915,-3.53727432775452));
#79637=CARTESIAN_POINT('Ctrl Pts',(4.7850737708186,-1.61541141083544,-3.58779761240434));
#79638=CARTESIAN_POINT('Ctrl Pts',(4.79093860974857,-1.50909711881973,-3.63380474372197));
#79639=CARTESIAN_POINT('Ctrl Pts',(4.79680344867854,-1.4008414500738,-3.67506901047519));
#79640=CARTESIAN_POINT('Ctrl Pts',(4.80266225878403,-1.29269706391098,-3.71629085918004));
#79641=CARTESIAN_POINT('Ctrl Pts',(4.80852106888951,-1.18261565442301,-3.75277939457094));
#79642=CARTESIAN_POINT('Ctrl Pts',(4.814379878995,-1.07104970171551,-3.78435483754564));
#79643=CARTESIAN_POINT('Ctrl Pts',(4.82046566788155,-0.955161522566597,
-3.81715355887017));
#79644=CARTESIAN_POINT('Ctrl Pts',(4.82655145676809,-0.83767185572949,-3.84465060929839));
#79645=CARTESIAN_POINT('Ctrl Pts',(4.83263724565464,-0.71910856941166,-3.8667003847465));
#79646=CARTESIAN_POINT('Ctrl Pts',(4.83848927571933,-0.605099370434301,
-3.88790321502003));
#79647=CARTESIAN_POINT('Ctrl Pts',(4.84434130578403,-0.490097951290665,
-3.90406943482824));
#79648=CARTESIAN_POINT('Ctrl Pts',(4.85019333584872,-0.374585997779909,
-3.91512124081327));
#79649=CARTESIAN_POINT('Ctrl Pts',(4.85604447621404,-0.259091605852325,
-3.92617136656345));
#79650=CARTESIAN_POINT('Ctrl Pts',(4.86189561657936,-0.143087245252928,
-3.93210858517045));
#79651=CARTESIAN_POINT('Ctrl Pts',(4.86774675694468,-0.0270603173116924,
-3.93290690701255));
#79652=CARTESIAN_POINT('Ctrl Pts',(4.87359842449938,0.0889770646881643,
-3.93370530078366));
#79653=CARTESIAN_POINT('Ctrl Pts',(4.87945009205407,0.205036604699887,-3.92936387451259));
#79654=CARTESIAN_POINT('Ctrl Pts',(4.88530175960877,0.320631018722372,-3.91990876804972));
#79655=CARTESIAN_POINT('Ctrl Pts',(4.89115537128061,0.436263837025392,-3.91045052028833));
#79656=CARTESIAN_POINT('Ctrl Pts',(4.89700898295247,0.551430810302264,-3.89587524779013));
#79657=CARTESIAN_POINT('Ctrl Pts',(4.90286259462431,0.665650601907628,-3.87626086276195));
#79658=CARTESIAN_POINT('Ctrl Pts',(4.90872286071249,0.780000239168845,-3.85662417999839));
#79659=CARTESIAN_POINT('Ctrl Pts',(4.91458312680066,0.893400137945136,-3.8319370208324));
#79660=CARTESIAN_POINT('Ctrl Pts',(4.92044339288884,1.00537986972123,-3.80232827588036));
#79661=CARTESIAN_POINT('Ctrl Pts',(4.92630760604881,1.11743502333547,-3.77269958851612));
#79662=CARTESIAN_POINT('Ctrl Pts',(4.93217181920878,1.22806771172037,-3.73814283779098));
#79663=CARTESIAN_POINT('Ctrl Pts',(4.93803603236875,1.33682502762982,-3.69883601224798));
#79664=CARTESIAN_POINT('Ctrl Pts',(4.94390888093235,1.4457424951736,-3.65947130505998));
#79665=CARTESIAN_POINT('Ctrl Pts',(4.94978172949596,1.5527786979277,-3.61534271984959));
#79666=CARTESIAN_POINT('Ctrl Pts',(4.95565457805957,1.65750288613398,-3.56667536824667));
#79667=CARTESIAN_POINT('Ctrl Pts',(4.95724932279709,1.68594025280957,-3.5534599750661));
#79668=CARTESIAN_POINT('Ctrl Pts',(4.95884406753462,1.71420729329543,-3.53991016100368));
#79669=CARTESIAN_POINT('Ctrl Pts',(4.96043881227214,1.74229574265083,-3.52603099038292));
#79670=CARTESIAN_POINT('Ctrl Pts',(4.96631125835394,1.84572790986844,-3.47492269749273));
#79671=CARTESIAN_POINT('Ctrl Pts',(4.97218370443574,1.94708253229897,-3.41917387948225));
#79672=CARTESIAN_POINT('Ctrl Pts',(4.97805615051755,2.04591419948807,-3.3589766430169));
#79673=CARTESIAN_POINT('Ctrl Pts',(4.98392098940941,2.14461783974361,-3.29885738629036));
#79674=CARTESIAN_POINT('Ctrl Pts',(4.98978582830127,2.24080467436438,-3.23430138371258));
#79675=CARTESIAN_POINT('Ctrl Pts',(4.99565066719313,2.33405149138522,-3.16554776232525));
#79676=CARTESIAN_POINT('Ctrl Pts',(5.00150947725937,2.4272024543152,-3.09686481697902));
#79677=CARTESIAN_POINT('Ctrl Pts',(5.0073682873256,2.51741908031261,-3.02399307940692));
#79678=CARTESIAN_POINT('Ctrl Pts',(5.01322709739184,2.60430547696755,-2.94721597149528));
#79679=CARTESIAN_POINT('Ctrl Pts',(5.01931288629267,2.69455797916813,-2.86746440660682));
#79680=CARTESIAN_POINT('Ctrl Pts',(5.0253986751935,2.78121660935734,-2.78349898821209));
#79681=CARTESIAN_POINT('Ctrl Pts',(5.03148446409433,2.86387346032466,-2.69568503413289));
#79682=CARTESIAN_POINT('Ctrl Pts',(5.03733649411715,2.94335541103549,-2.61124406779842));
#79683=CARTESIAN_POINT('Ctrl Pts',(5.04318852413997,3.01913702380235,-2.52324509018783));
#79684=CARTESIAN_POINT('Ctrl Pts',(5.04904055416279,3.09089239730181,-2.43205123060799));
#79685=CARTESIAN_POINT('Ctrl Pts',(5.05489169448533,3.16263686163381,-2.3408712354823));
#79686=CARTESIAN_POINT('Ctrl Pts',(5.06074283480786,3.23035604825503,-2.24649764893359));
#79687=CARTESIAN_POINT('Ctrl Pts',(5.06659397513041,3.29376455157214,-2.1493264244425));
#79688=CARTESIAN_POINT('Ctrl Pts',(5.07244564264147,3.35717876800379,-2.05214644481121));
#79689=CARTESIAN_POINT('Ctrl Pts',(5.07829731015253,3.41628130313462,-1.95216867234492));
#79690=CARTESIAN_POINT('Ctrl Pts',(5.08414897766359,3.47083066658839,-1.84981714876623));
#79691=CARTESIAN_POINT('Ctrl Pts',(5.09000258929098,3.52539815313408,-1.74743162064646));
#79692=CARTESIAN_POINT('Ctrl Pts',(5.09585620091836,3.5754092657523,-1.64267113784546));
#79693=CARTESIAN_POINT('Ctrl Pts',(5.10170981254575,3.62066928123041,-1.53598273296104));
#79694=CARTESIAN_POINT('Ctrl Pts',(5.10757007858847,3.66598074852326,-1.42917304415781));
#79695=CARTESIAN_POINT('Ctrl Pts',(5.1134303446312,3.70653017679169,-1.32043143952382));
#79696=CARTESIAN_POINT('Ctrl Pts',(5.11929061067393,3.74217162445302,-1.21022334018918));
#79697=CARTESIAN_POINT('Ctrl Pts',(5.1251548237878,3.77783707773611,-1.09994101227738));
#79698=CARTESIAN_POINT('Ctrl Pts',(5.13101903690168,3.80858785874347,-0.988190620465026));
#79699=CARTESIAN_POINT('Ctrl Pts',(5.13688325001556,3.83432880143551,-0.875449394586642));
#79700=CARTESIAN_POINT('Ctrl Pts',(5.14275609853249,3.86010764919865,-0.762542150538906));
#79701=CARTESIAN_POINT('Ctrl Pts',(5.14862894704941,3.88086186123423,-0.648641565558515));
#79702=CARTESIAN_POINT('Ctrl Pts',(5.15450179556634,3.89654789264389,-0.534231710339649));
#79703=CARTESIAN_POINT('Ctrl Pts',(5.15609654071482,3.9008073627149,-0.503164237541329));
#79704=CARTESIAN_POINT('Ctrl Pts',(5.15769128586329,3.9046934176504,-0.472059219835393));
#79705=CARTESIAN_POINT('Ctrl Pts',(5.15928603101177,3.9082058486662,-0.440926348102861));
#79706=CARTESIAN_POINT('Ctrl Pts',(5.1651584771793,3.92113992912232,-0.326283507856984));
#79707=CARTESIAN_POINT('Ctrl Pts',(5.17103092334683,3.92904700856901,-0.210879137396811));
#79708=CARTESIAN_POINT('Ctrl Pts',(5.17690336951435,3.93184785086485,-0.0951917940235433));
#79709=CARTESIAN_POINT('Ctrl Pts',(5.18276820849321,3.93464506493914,0.020345687533596));
#79710=CARTESIAN_POINT('Ctrl Pts',(5.18863304747207,3.93234918611412,0.136165003611755));
#79711=CARTESIAN_POINT('Ctrl Pts',(5.19449788645093,3.92493253515872,0.251780846079617));
#79712=CARTESIAN_POINT('Ctrl Pts',(5.20035669660532,3.91752350822963,0.36727783999562));
#79713=CARTESIAN_POINT('Ctrl Pts',(5.20621550675971,3.9050042057642,0.482571366305245));
#79714=CARTESIAN_POINT('Ctrl Pts',(5.2120743169141,3.88739898171281,0.597175147656201));
#79715=CARTESIAN_POINT('Ctrl Pts',(5.21816010578232,3.869111706015,0.716218843973764));
#79716=CARTESIAN_POINT('Ctrl Pts',(5.22424589465055,3.84533645586416,0.834517816800412));
#79717=CARTESIAN_POINT('Ctrl Pts',(5.23033168351877,3.8161599802714,0.951531399889123));
#79718=CARTESIAN_POINT('Ctrl Pts',(5.23618371363209,3.78810419038673,1.06405042194691));
#79719=CARTESIAN_POINT('Ctrl Pts',(5.24203574374541,3.75505455895332,1.17538053978761));
#79720=CARTESIAN_POINT('Ctrl Pts',(5.24788777385873,3.71714033540991,1.28505125456875));
#79721=CARTESIAN_POINT('Ctrl Pts',(5.25373891427248,3.67923187606583,1.39470529582209));
#79722=CARTESIAN_POINT('Ctrl Pts',(5.25959005468625,3.63646043015309,1.50270004507394));
#79723=CARTESIAN_POINT('Ctrl Pts',(5.2654411951,3.58900475555364,1.60858132048503));
#79724=CARTESIAN_POINT('Ctrl Pts',(5.2712928627029,3.54154480518665,1.71447213582416));
#79725=CARTESIAN_POINT('Ctrl Pts',(5.27714453030579,3.48939995620785,1.81824872155039));
#79726=CARTESIAN_POINT('Ctrl Pts',(5.28299619790869,3.43279633998593,1.91947865009726));
#79727=CARTESIAN_POINT('Ctrl Pts',(5.28884980962844,3.37617391817692,2.02074221056314));
#79728=CARTESIAN_POINT('Ctrl Pts',(5.2947034213482,3.31508998518154,2.11945707086956));
#79729=CARTESIAN_POINT('Ctrl Pts',(5.30055703306796,3.24981529998154,2.21521771300383));
#79730=CARTESIAN_POINT('Ctrl Pts',(5.30641729920336,3.1844664101866,2.3110872163243));
#79731=CARTESIAN_POINT('Ctrl Pts',(5.31227756533877,3.11491749222178,2.4039954565216));
#79732=CARTESIAN_POINT('Ctrl Pts',(5.31813783147417,3.04148115039268,2.49356800825765));
#79733=CARTESIAN_POINT('Ctrl Pts',(5.32400204468104,2.96799534690394,2.58320088989244));
#79734=CARTESIAN_POINT('Ctrl Pts',(5.3298662578879,2.89061718127177,2.6694933024567));
#79735=CARTESIAN_POINT('Ctrl Pts',(5.33573047109477,2.80969664624507,2.75210714836454));
#79736=CARTESIAN_POINT('Ctrl Pts',(5.3416033197044,2.72865695091712,2.83484264807464));
#79737=CARTESIAN_POINT('Ctrl Pts',(5.34747616831404,2.64406477628405,2.91388848890184));
#79738=CARTESIAN_POINT('Ctrl Pts',(5.35334901692367,2.55630378176638,2.98894629850168));
#79739=CARTESIAN_POINT('Ctrl Pts',(5.35494376119959,2.53247269859723,3.009327891861));
#79740=CARTESIAN_POINT('Ctrl Pts',(5.35653850547551,2.5084081231882,3.02941566631621));
#79741=CARTESIAN_POINT('Ctrl Pts',(5.35813324975143,2.48411809468964,3.04920420628654));
#79742=CARTESIAN_POINT('Ctrl Pts',(5.36400569588059,2.39467310593038,3.12207302714088));
#79743=CARTESIAN_POINT('Ctrl Pts',(5.36987814200974,2.30186936027663,3.19112485718943));
#79744=CARTESIAN_POINT('Ctrl Pts',(5.3757505881389,2.20606658059504,3.25603428145063));
#79745=CARTESIAN_POINT('Ctrl Pts',(5.381615427079,2.11038790419881,3.32085962179663));
#79746=CARTESIAN_POINT('Ctrl Pts',(5.3874802660191,2.01171825863209,3.38155299787701));
#79747=CARTESIAN_POINT('Ctrl Pts',(5.39334510495919,1.91045092296981,3.43782871459935));
#79748=CARTESIAN_POINT('Ctrl Pts',(5.39920391507448,1.80928768616376,3.4940465820882));
#79749=CARTESIAN_POINT('Ctrl Pts',(5.40506272518976,1.70553242982779,3.54585562329428));
#79750=CARTESIAN_POINT('Ctrl Pts',(5.41092153530505,1.59960738322865,3.59301338983316));
#79751=CARTESIAN_POINT('Ctrl Pts',(5.4170073241878,1.48957864730563,3.64199811637156));
#79752=CARTESIAN_POINT('Ctrl Pts',(5.42309311307055,1.37720897540698,3.68596363024611));
#79753=CARTESIAN_POINT('Ctrl Pts',(5.4291789019533,1.26300008688424,3.72469056171521));
#79754=CARTESIAN_POINT('Ctrl Pts',(5.4350309320269,1.15317803042048,3.76192996846788));
#79755=CARTESIAN_POINT('Ctrl Pts',(5.44088296210051,1.04165586952818,3.79432565857732));
#79756=CARTESIAN_POINT('Ctrl Pts',(5.44673499217412,0.928899278516613,3.82173195428085));
#79757=CARTESIAN_POINT('Ctrl Pts',(5.452586132548,0.816159830189972,3.84913408333223));
#79758=CARTESIAN_POINT('Ctrl Pts',(5.45843727292188,0.702186726453746,3.87154822862387));
#79759=CARTESIAN_POINT('Ctrl Pts',(5.46428841329576,0.587458685331134,3.88887918210749));
#79760=CARTESIAN_POINT('Ctrl Pts',(5.47014008085867,0.472720307186906,3.90621169711381));
#79761=CARTESIAN_POINT('Ctrl Pts',(5.47599174842159,0.357227265183229,3.91846004811158));
#79762=CARTESIAN_POINT('Ctrl Pts',(5.4818434159845,0.241465592784657,3.92558064080986));
#79763=CARTESIAN_POINT('Ctrl Pts',(5.48769702766419,0.125665460544065,3.93270359920367));
#79764=CARTESIAN_POINT('Ctrl Pts',(5.49355063934388,0.00959693280344369,
3.93469538640835));
#79765=CARTESIAN_POINT('Ctrl Pts',(5.49940425102358,-0.106252462921666,
3.93156449955016));
#79766=CARTESIAN_POINT('Ctrl Pts',(5.50526451711901,-0.222233556833263,
3.92843005348375));
#79767=CARTESIAN_POINT('Ctrl Pts',(5.51112478321445,-0.337994608063186,
3.92016132105254));
#79768=CARTESIAN_POINT('Ctrl Pts',(5.51698504930989,-0.453051618335803,
3.90681881216973));
#79769=CARTESIAN_POINT('Ctrl Pts',(5.52284926247678,-0.568186123082922,
3.89346731669226));
#79770=CARTESIAN_POINT('Ctrl Pts',(5.52871347564367,-0.682615235559708,
3.87503530571441));
#79771=CARTESIAN_POINT('Ctrl Pts',(5.53457768881057,-0.795865300405437,
3.85163438342875));
#79772=CARTESIAN_POINT('Ctrl Pts',(5.54045053738055,-0.909282132715467,
3.82819900189155));
#79773=CARTESIAN_POINT('Ctrl Pts',(5.54632338595054,-1.02151605304674,3.79978020681874));
#79774=CARTESIAN_POINT('Ctrl Pts',(5.55219623452053,-1.1321086193517,3.76653940295194));
#79775=CARTESIAN_POINT('Ctrl Pts',(5.55379097917738,-1.16213951527903,3.75751301759154));
#79776=CARTESIAN_POINT('Ctrl Pts',(5.55538572383423,-1.19204949971307,3.74813134541748));
#79777=CARTESIAN_POINT('Ctrl Pts',(5.55698046849108,-1.22182967016167,3.73839822077753));
#79778=CARTESIAN_POINT('Ctrl Pts',(5.5628529146185,-1.33149139304234,3.70255721648003));
#79779=CARTESIAN_POINT('Ctrl Pts',(5.56872536074592,-1.43975834348045,3.66182690993442));
#79780=CARTESIAN_POINT('Ctrl Pts',(5.57459780687335,-1.54616227365557,3.61633394800926));
#79781=CARTESIAN_POINT('Ctrl Pts',(5.58046264581158,-1.65242836777232,3.57089991784108));
#79782=CARTESIAN_POINT('Ctrl Pts',(5.58632748474981,-1.75683586437637,3.52071566236118));
#79783=CARTESIAN_POINT('Ctrl Pts',(5.59219232368805,-1.85893178418655,3.46595753317045));
#79784=CARTESIAN_POINT('Ctrl Pts',(5.59805113380136,-1.96092275338637,3.41125569319375));
#79785=CARTESIAN_POINT('Ctrl Pts',(5.60390994391467,-2.06060651012118,3.35198952577101));
#79786=CARTESIAN_POINT('Ctrl Pts',(5.60976875402798,-2.15755080096085,3.28838311960045));
#79787=CARTESIAN_POINT('Ctrl Pts',(5.61585454291143,-2.25825085371823,3.2223125093396));
#79788=CARTESIAN_POINT('Ctrl Pts',(5.62194033179488,-2.35599446809467,3.15155874318567));
#79789=CARTESIAN_POINT('Ctrl Pts',(5.62802612067832,-2.45032582351664,3.07642525646366));
#79790=CARTESIAN_POINT('Ctrl Pts',(5.63387815074965,-2.5410338548287,3.00417769216567));
#79791=CARTESIAN_POINT('Ctrl Pts',(5.63973018082097,-2.62858657239987,2.92788093768364));
#79792=CARTESIAN_POINT('Ctrl Pts',(5.6455822108923,-2.7126096359302,2.84784795293896));
#79793=CARTESIAN_POINT('Ctrl Pts',(5.6514333512638,-2.79661992520883,2.76782713582359));
#79794=CARTESIAN_POINT('Ctrl Pts',(5.6572844916353,-2.87710132820144,2.68407150288923));
#79795=CARTESIAN_POINT('Ctrl Pts',(5.6631356320068,-2.95371490731195,2.59693227603709));
#79796=CARTESIAN_POINT('Ctrl Pts',(5.66898729956722,-3.03033538932134,2.50978519792309));
#79797=CARTESIAN_POINT('Ctrl Pts',(5.67483896712764,-3.10308708172622,2.41925423030597));
#79798=CARTESIAN_POINT('Ctrl Pts',(5.68069063468806,-3.1716705093492,2.32572465698857));
#79799=CARTESIAN_POINT('Ctrl Pts',(5.68654424636516,-3.24027672264545,2.23216401006677));
#79800=CARTESIAN_POINT('Ctrl Pts',(5.69239785804226,-3.30471167319672,2.13560310965609));
#79801=CARTESIAN_POINT('Ctrl Pts',(5.69825146971936,-3.36471889774139,2.03645666273111));
#79802=CARTESIAN_POINT('Ctrl Pts',(5.70411173581206,-3.42479433880496,1.93719750561965));
#79803=CARTESIAN_POINT('Ctrl Pts',(5.70997200190475,-3.48043179308373,1.83534728916393));
#79804=CARTESIAN_POINT('Ctrl Pts',(5.71583226799745,-3.53142045923226,1.73134587535703));
#79805=CARTESIAN_POINT('Ctrl Pts',(5.72169648116154,-3.58244346783244,1.62727441336501));
#79806=CARTESIAN_POINT('Ctrl Pts',(5.72756069432563,-3.6288112886858,1.52104924688573));
#79807=CARTESIAN_POINT('Ctrl Pts',(5.73342490748972,-3.67036169393012,1.41312916456012));
#79808=CARTESIAN_POINT('Ctrl Pts',(5.73929775605678,-3.71197328461965,1.30505016348884));
#79809=CARTESIAN_POINT('Ctrl Pts',(5.74517060462384,-3.74875317080466,1.19527165579196));
#79810=CARTESIAN_POINT('Ctrl Pts',(5.7510434531909,-3.7805892432829,1.08426656020261));
#79811=CARTESIAN_POINT('Ctrl Pts',(5.75263819787084,-3.78923418051141,1.05412364341946));
#79812=CARTESIAN_POINT('Ctrl Pts',(5.75423294255078,-3.79751486921203,1.02389033124141));
#79813=CARTESIAN_POINT('Ctrl Pts',(5.75582768723071,-3.80542972120358,0.993576185795752));
#79814=CARTESIAN_POINT('Ctrl Pts',(5.76345579314931,-3.84328865253039,0.848575224074156));
#79815=CARTESIAN_POINT('Ctrl Pts',(5.7710838990679,-3.87287613987567,0.70133166860417));
#79816=CARTESIAN_POINT('Ctrl Pts',(5.7787120049865,-3.89397603459136,0.552665940716588));
#79817=CARTESIAN_POINT('Ctrl Pts',(5.78618099959784,-3.91463581588087,0.407101165878184));
#79818=CARTESIAN_POINT('Ctrl Pts',(5.79364999420918,-3.92715842132982,0.260172687026572));
#79819=CARTESIAN_POINT('Ctrl Pts',(5.80111898882052,-3.9313857410616,0.112672778334271));
#79820=CARTESIAN_POINT('Ctrl Pts',(5.80295814726045,-3.93242667242753,0.0763525349714642));
#79821=CARTESIAN_POINT('Ctrl Pts',(5.80479730570037,-3.93296484650485,0.0399977603377867));
#79822=CARTESIAN_POINT('Ctrl Pts',(5.8066364641403,-3.93299833356548,0.00362052083856629));
#79823=CARTESIAN_POINT('',(7.05663650576764,-3.93060739270548,-0.000901275032790407));
#79824=CARTESIAN_POINT('Ctrl Pts',(5.80663647796509,-3.93210781031187,0.00361942768470874));
#79825=CARTESIAN_POINT('Ctrl Pts',(5.85598262063352,-3.92329404442754,-0.972199952904983));
#79826=CARTESIAN_POINT('Ctrl Pts',(5.97161116954849,-3.06253954822306,-3.27263336896532));
#79827=CARTESIAN_POINT('Ctrl Pts',(6.15352212470999,0.80000188434543,-4.58235619056535));
#79828=CARTESIAN_POINT('Ctrl Pts',(6.35236934344966,4.28728808542873,-1.80475819528463));
#79829=CARTESIAN_POINT('Ctrl Pts',(6.55121656218928,3.83635924797249,2.63065371934916));
#79830=CARTESIAN_POINT('Ctrl Pts',(6.75006378092894,-0.138570632095021,
4.64960099912353));
#79831=CARTESIAN_POINT('Ctrl Pts',(6.91853708618754,-3.39848507636798,2.74152539667428));
#79832=CARTESIAN_POINT('Ctrl Pts',(7.02072798519958,-3.92523164958614,0.711663097972118));
#79833=CARTESIAN_POINT('Ctrl Pts',(7.05663647796509,-3.92668421635667,-0.000899823416283008));
#79834=CARTESIAN_POINT('',(8.3066364779651,-3.93344384724419,-0.00329189189212218));
#79835=CARTESIAN_POINT('Ctrl Pts',(7.05663652272271,-3.93299989653023,-0.000902160284366488));
#79836=CARTESIAN_POINT('Ctrl Pts',(7.06288361214318,-3.93297141513468,-0.125067818755675));
#79837=CARTESIAN_POINT('Ctrl Pts',(7.06913070156365,-3.92705879239068,-0.249078431000784));
#79838=CARTESIAN_POINT('Ctrl Pts',(7.07537779098412,-3.91533128588655,-0.372384105136066));
#79839=CARTESIAN_POINT('Ctrl Pts',(7.08164686886942,-3.90356250098108,-0.496123789783527));
#79840=CARTESIAN_POINT('Ctrl Pts',(7.08791594675472,-3.88593791112278,-0.619153250419358));
#79841=CARTESIAN_POINT('Ctrl Pts',(7.09418502464002,-3.86257841551443,-0.740929810442296));
#79842=CARTESIAN_POINT('Ctrl Pts',(7.10046521277651,-3.83917752149492,-0.862922186602119));
#79843=CARTESIAN_POINT('Ctrl Pts',(7.106745400913,-3.81002150458914,-0.983656917383635));
#79844=CARTESIAN_POINT('Ctrl Pts',(7.11302558904949,-3.77528127951279,-1.10260612213077));
#79845=CARTESIAN_POINT('Ctrl Pts',(7.1193249248549,-3.74043513494592,-1.22191799117091));
#79846=CARTESIAN_POINT('Ctrl Pts',(7.12562426066031,-3.69997082401521,-1.33943313800122));
#79847=CARTESIAN_POINT('Ctrl Pts',(7.13192359646571,-3.65410841841374,-1.45464107823127));
#79848=CARTESIAN_POINT('Ctrl Pts',(7.13720180377988,-3.61568035358776,-1.55117369874183));
#79849=CARTESIAN_POINT('Ctrl Pts',(7.14248001109405,-3.57346331290171,-1.64608680048987));
#79850=CARTESIAN_POINT('Ctrl Pts',(7.14775821840821,-3.52761112971304,-1.73909422330265));
#79851=CARTESIAN_POINT('Ctrl Pts',(7.15363066454209,-3.47659674928628,-1.8425727431882));
#79852=CARTESIAN_POINT('Ctrl Pts',(7.15950311067597,-3.4209399596555,-1.94397793156341));
#79853=CARTESIAN_POINT('Ctrl Pts',(7.16537555680985,-3.36083246309158,-2.04286420376632));
#79854=CARTESIAN_POINT('Ctrl Pts',(7.17124039575466,-3.30080283000746,-2.14162237831588));
#79855=CARTESIAN_POINT('Ctrl Pts',(7.17710523469946,-3.23633416817014,-2.2378677757007));
#79856=CARTESIAN_POINT('Ctrl Pts',(7.18297007364427,-3.16766522035791,-2.33117696705652));
#79857=CARTESIAN_POINT('Ctrl Pts',(7.18882888376425,-3.09906686153566,-2.42439024021667));
#79858=CARTESIAN_POINT('Ctrl Pts',(7.19468769388423,-3.02627704847413,-2.51467297999974));
#79859=CARTESIAN_POINT('Ctrl Pts',(7.20054650400421,-2.94957884357713,-2.60162903687712));
#79860=CARTESIAN_POINT('Ctrl Pts',(7.20663229288519,-2.86990923951165,-2.6919538969155));
#79861=CARTESIAN_POINT('Ctrl Pts',(7.21271808176618,-2.78602252134734,-2.77868871160012));
#79862=CARTESIAN_POINT('Ctrl Pts',(7.21880387064716,-2.69828363646979,-2.86142524228038));
#79863=CARTESIAN_POINT('Ctrl Pts',(7.22465590072539,-2.61391485480897,-2.94098381317034));
#79864=CARTESIAN_POINT('Ctrl Pts',(7.23050793080362,-2.52598470426606,-3.01684527738739));
#79865=CARTESIAN_POINT('Ctrl Pts',(7.23635996088185,-2.43485601816631,-3.08868340410592));
#79866=CARTESIAN_POINT('Ctrl Pts',(7.24221110126033,-2.34374118660395,-3.16051060908229));
#79867=CARTESIAN_POINT('Ctrl Pts',(7.2480622416388,-2.24942911090274,-3.22831543694416));
#79868=CARTESIAN_POINT('Ctrl Pts',(7.25391338201728,-2.15231548530825,-3.29181212278318));
#79869=CARTESIAN_POINT('Ctrl Pts',(7.25976504958474,-2.05519310975554,-3.35531452968703));
#79870=CARTESIAN_POINT('Ctrl Pts',(7.26561671715221,-1.95526902851059,-3.41450779671165));
#79871=CARTESIAN_POINT('Ctrl Pts',(7.27146838471967,-1.85296706391351,-3.4691500486505));
#79872=CARTESIAN_POINT('Ctrl Pts',(7.27732199640388,-1.75063111123349,-3.52381045454561));
#79873=CARTESIAN_POINT('Ctrl Pts',(7.28317560808809,-1.64591606872578,-3.57391664419774));
#79874=CARTESIAN_POINT('Ctrl Pts',(7.2890292197723,-1.5392687920494,-3.6192734886746));
#79875=CARTESIAN_POINT('Ctrl Pts',(7.29488948587215,-1.43250027820454,-3.66468189504376));
#79876=CARTESIAN_POINT('Ctrl Pts',(7.30074975197199,-1.32379552651248,-3.70533001798262));
#79877=CARTESIAN_POINT('Ctrl Pts',(7.30661001807184,-1.21361982543884,-3.74107149347641));
#79878=CARTESIAN_POINT('Ctrl Pts',(7.31247423124311,-1.10336991760511,-3.77683704196516));
#79879=CARTESIAN_POINT('Ctrl Pts',(7.31833844441438,-0.991647485115964,
-3.80768925276693));
#79880=CARTESIAN_POINT('Ctrl Pts',(7.32420265758565,-0.878929671228565,
-3.83353252666963));
#79881=CARTESIAN_POINT('Ctrl Pts',(7.3300755061599,-0.766045873650185,-3.85941385633159));
#79882=CARTESIAN_POINT('Ctrl Pts',(7.33594835473416,-0.652164174375472,
-3.88027145396397));
#79883=CARTESIAN_POINT('Ctrl Pts',(7.34182120330841,-0.537768604378055,
-3.89606133526479));
#79884=CARTESIAN_POINT('Ctrl Pts',(7.34341594792156,-0.506705021397034,
-3.90034900381751));
#79885=CARTESIAN_POINT('Ctrl Pts',(7.34501069253471,-0.475603554578537,
-3.90426329172176));
#79886=CARTESIAN_POINT('Ctrl Pts',(7.34660543714786,-0.444473894600172,
-3.90780398139658));
#79887=CARTESIAN_POINT('Ctrl Pts',(7.35247788328177,-0.329842843406956,
-3.92084212507229));
#79888=CARTESIAN_POINT('Ctrl Pts',(7.35835032941567,-0.214445698971003,
-3.92885396116556));
#79889=CARTESIAN_POINT('Ctrl Pts',(7.36422277554958,-0.0987609464627275,
-3.93175981914636));
#79890=CARTESIAN_POINT('Ctrl Pts',(7.37008761449442,0.0167739475768885,
-3.93466191286766));
#79891=CARTESIAN_POINT('Ctrl Pts',(7.37595245343926,0.132595299365251,-3.93247117168982));
#79892=CARTESIAN_POINT('Ctrl Pts',(7.3818172923841,0.248217826102488,-3.92515947584362));
#79893=CARTESIAN_POINT('Ctrl Pts',(7.38767610250411,0.363721497408917,-3.91785529613449));
#79894=CARTESIAN_POINT('Ctrl Pts',(7.39353491262413,0.47902634013968,-3.90544065835273));
#79895=CARTESIAN_POINT('Ctrl Pts',(7.39939372274414,0.593646055039921,-3.88793947500929));
#79896=CARTESIAN_POINT('Ctrl Pts',(7.40547951162512,0.712706303143439,-3.86976027056101));
#79897=CARTESIAN_POINT('Ctrl Pts',(7.41156530050609,0.831026809866332,-3.84609241785892));
#79898=CARTESIAN_POINT('Ctrl Pts',(7.41765108938706,0.948066830428479,-3.81702217507854));
#79899=CARTESIAN_POINT('Ctrl Pts',(7.42350311946532,1.06061127357061,-3.78906853776704));
#79900=CARTESIAN_POINT('Ctrl Pts',(7.42935514954358,1.17197134624308,-3.75611998177188));
#79901=CARTESIAN_POINT('Ctrl Pts',(7.43520717962184,1.28167643247323,-3.71830532937287));
#79902=CARTESIAN_POINT('Ctrl Pts',(7.44105832000035,1.3913648399463,-3.6804964260364));
#79903=CARTESIAN_POINT('Ctrl Pts',(7.44690946037885,1.49939837057773,-3.63782303193787));
#79904=CARTESIAN_POINT('Ctrl Pts',(7.45276060075736,1.60532268044908,-3.59046349259198));
#79905=CARTESIAN_POINT('Ctrl Pts',(7.45861226832485,1.71125653412312,-3.54309968614159));
#79906=CARTESIAN_POINT('Ctrl Pts',(7.46446393589234,1.81508041187348,-3.4910490638332));
#79907=CARTESIAN_POINT('Ctrl Pts',(7.47031560345983,1.91636168104144,-3.43453736439655));
#79908=CARTESIAN_POINT('Ctrl Pts',(7.47616921514406,2.01767659918357,-3.37800688991166));
#79909=CARTESIAN_POINT('Ctrl Pts',(7.48202282682829,2.116446868255,-3.31701259250204));
#79910=CARTESIAN_POINT('Ctrl Pts',(7.48787643851252,2.21226672462819,-3.25182486291972));
#79911=CARTESIAN_POINT('Ctrl Pts',(7.4937367046124,2.30819550950339,-3.18656302759355));
#79912=CARTESIAN_POINT('Ctrl Pts',(7.49959697071228,2.40116684515268,-3.11709847773811));
#79913=CARTESIAN_POINT('Ctrl Pts',(7.50545723681217,2.49080602262458,-3.04374347763689));
#79914=CARTESIAN_POINT('Ctrl Pts',(7.51132144998346,2.58050557486939,-2.9703390706625));
#79915=CARTESIAN_POINT('Ctrl Pts',(7.51718566315476,2.66686819281238,-2.89303927082564));
#79916=CARTESIAN_POINT('Ctrl Pts',(7.52304987632606,2.74955546129944,-2.81219376381472));
#79917=CARTESIAN_POINT('Ctrl Pts',(7.52892272490034,2.83236449171167,-2.73122920698205));
#79918=CARTESIAN_POINT('Ctrl Pts',(7.53479557347462,2.91148708962327,-2.64670882299955));
#79919=CARTESIAN_POINT('Ctrl Pts',(7.54066842204891,2.9866245345438,-2.55901600027452));
#79920=CARTESIAN_POINT('Ctrl Pts',(7.54226316666178,3.00702775693175,-2.53520342365873));
#79921=CARTESIAN_POINT('Ctrl Pts',(7.54385791127464,3.02713737236875,-2.51115708808148));
#79922=CARTESIAN_POINT('Ctrl Pts',(7.54545265588751,3.04694795797518,-2.48688502777891));
#79923=CARTESIAN_POINT('Ctrl Pts',(7.55132510202144,3.11989794377009,-2.39750622346376));
#79924=CARTESIAN_POINT('Ctrl Pts',(7.55719754815538,3.18903398928196,-2.30476519870854));
#79925=CARTESIAN_POINT('Ctrl Pts',(7.56306999428931,3.25403035311977,-2.20902138083252));
#79926=CARTESIAN_POINT('Ctrl Pts',(7.56893483323417,3.31894252042051,-2.11340158986255));
#79927=CARTESIAN_POINT('Ctrl Pts',(7.57479967217902,3.37972544024367,-2.01478708010426));
#79928=CARTESIAN_POINT('Ctrl Pts',(7.58066451112388,3.43609306060994,-1.91357087112765));
#79929=CARTESIAN_POINT('Ctrl Pts',(7.58652332124391,3.49240273726927,-1.81245870845122));
#79930=CARTESIAN_POINT('Ctrl Pts',(7.59238213136395,3.54430594239584,-1.70875052513813));
#79931=CARTESIAN_POINT('Ctrl Pts',(7.59824094148399,3.59155984442061,-1.60286833019602));
#79932=CARTESIAN_POINT('Ctrl Pts',(7.60432673036495,3.64064443081831,-1.49288410618655));
#79933=CARTESIAN_POINT('Ctrl Pts',(7.61041251924591,3.68471193163949,-1.38055439091041));
#79934=CARTESIAN_POINT('Ctrl Pts',(7.61649830812688,3.72354252179092,-1.26638070437564));
#79935=CARTESIAN_POINT('Ctrl Pts',(7.62235033820516,3.7608816056744,-1.15659249765038));
#79936=CARTESIAN_POINT('Ctrl Pts',(7.62820236828344,3.79337851819582,-1.04509979024559));
#79937=CARTESIAN_POINT('Ctrl Pts',(7.63405439836172,3.82088715893014,-0.93236812403833));
#79938=CARTESIAN_POINT('Ctrl Pts',(7.63990553874025,3.84839161745238,-0.819653596727187));
#79939=CARTESIAN_POINT('Ctrl Pts',(7.64575667911878,3.87090921412992,-0.705700886603481));
#79940=CARTESIAN_POINT('Ctrl Pts',(7.65160781949731,3.8883443063907,-0.590988625067398));
#79941=CARTESIAN_POINT('Ctrl Pts',(7.65745948706482,3.90578096955697,-0.476266027932311));
#79942=CARTESIAN_POINT('Ctrl Pts',(7.66331115463233,3.91813415585814,-0.360784152029154));
#79943=CARTESIAN_POINT('Ctrl Pts',(7.66916282219984,3.92535982981755,-0.245028991049561));
#79944=CARTESIAN_POINT('Ctrl Pts',(7.6750164338841,3.93258790438388,-0.129235372392126));
#79945=CARTESIAN_POINT('Ctrl Pts',(7.68087004556835,3.93468505350706,-0.0131687004549297));
#79946=CARTESIAN_POINT('Ctrl Pts',(7.6867236572526,3.93165933174991,0.1026834897333));
#79947=CARTESIAN_POINT('Ctrl Pts',(7.6925839233525,3.92863017033682,0.218667381282902));
#79948=CARTESIAN_POINT('Ctrl Pts',(7.6984441894524,3.92046652491974,0.334435890958983));
#79949=CARTESIAN_POINT('Ctrl Pts',(7.70430445555231,3.90722846603072,0.449504965755925));
#79950=CARTESIAN_POINT('Ctrl Pts',(7.71016866872363,3.89398149089746,0.56465154315226));
#79951=CARTESIAN_POINT('Ctrl Pts',(7.71603288189495,3.87565336201966,0.679097340474461));
#79952=CARTESIAN_POINT('Ctrl Pts',(7.72189709506627,3.85235525357663,0.792368601245983));
#79953=CARTESIAN_POINT('Ctrl Pts',(7.72776994364057,3.82902283728201,0.905806660691923));
#79954=CARTESIAN_POINT('Ctrl Pts',(7.73364279221488,3.80070593569257,1.01806633240571));
#79955=CARTESIAN_POINT('Ctrl Pts',(7.73951564078919,3.76756553732628,1.12868902801052));
#79956=CARTESIAN_POINT('Ctrl Pts',(7.74111038540184,3.75856641686759,1.15872810455419));
#79957=CARTESIAN_POINT('Ctrl Pts',(7.74270513001449,3.74921190000219,1.18864659217748));
#79958=CARTESIAN_POINT('Ctrl Pts',(7.74429987462715,3.73950581299458,1.21843558491194));
#79959=CARTESIAN_POINT('Ctrl Pts',(7.75017232076106,3.70376437033916,1.32812979790921));
#79960=CARTESIAN_POINT('Ctrl Pts',(7.75604476689497,3.66313236131554,1.43643367736083));
#79961=CARTESIAN_POINT('Ctrl Pts',(7.76191721302888,3.61773600768323,1.5428788606732));
#79962=CARTESIAN_POINT('Ctrl Pts',(7.76778205197371,3.57239846066019,1.64918615448997));
#79963=CARTESIAN_POINT('Ctrl Pts',(7.77364689091855,3.52230900310579,1.75363916363233));
#79964=CARTESIAN_POINT('Ctrl Pts',(7.77951172986338,3.46764357535158,1.85578474891968));
#79965=CARTESIAN_POINT('Ctrl Pts',(7.7853705399834,3.4130343415169,1.95782533254445));
#79966=CARTESIAN_POINT('Ctrl Pts',(7.79122935010342,3.35385868770488,2.05756284797543));
#79967=CARTESIAN_POINT('Ctrl Pts',(7.79708816022343,3.29034031013881,2.15456483854063));
#79968=CARTESIAN_POINT('Ctrl Pts',(7.80317394910441,3.22436113894012,2.25532482623803));
#79969=CARTESIAN_POINT('Ctrl Pts',(7.80925973798537,3.15369613003769,2.35313262796932));
#79970=CARTESIAN_POINT('Ctrl Pts',(7.81534552686635,3.07864830485412,2.44753214790303));
#79971=CARTESIAN_POINT('Ctrl Pts',(7.82119755694461,3.00648311166854,2.53830572563136));
#79972=CARTESIAN_POINT('Ctrl Pts',(7.82704958702288,2.93026586568177,2.62592766661633));
#79973=CARTESIAN_POINT('Ctrl Pts',(7.83290161710114,2.85030918687491,2.71002334661834));
#79974=CARTESIAN_POINT('Ctrl Pts',(7.83875275747964,2.77036466409535,2.79410624132966));
#79975=CARTESIAN_POINT('Ctrl Pts',(7.84460389785815,2.68668212363562,2.87466364152844));
#79976=CARTESIAN_POINT('Ctrl Pts',(7.85045503823666,2.59961247957813,2.95135629093162));
#79977=CARTESIAN_POINT('Ctrl Pts',(7.85630670580415,2.51253499052731,3.02805585035871));
#79978=CARTESIAN_POINT('Ctrl Pts',(7.86215837337164,2.42207010141677,3.10088969353643));
#79979=CARTESIAN_POINT('Ctrl Pts',(7.86801004093913,2.32860282403901,3.16955799566399));
#79980=CARTESIAN_POINT('Ctrl Pts',(7.87386365262336,2.23510449375257,3.2382491116637));
#79981=CARTESIAN_POINT('Ctrl Pts',(7.87971726430759,2.13860212468947,3.30277169014711));
#79982=CARTESIAN_POINT('Ctrl Pts',(7.88557087599182,2.03951019084641,3.36286889150226));
#79983=CARTESIAN_POINT('Ctrl Pts',(7.89143114209171,1.940305608787,3.42303441166277));
#79984=CARTESIAN_POINT('Ctrl Pts',(7.89729140819159,1.83850593980556,3.47876429892532));
#79985=CARTESIAN_POINT('Ctrl Pts',(7.90315167429147,1.73455085435709,3.5298473527405));
#79986=CARTESIAN_POINT('Ctrl Pts',(7.90901588746277,1.6305257519266,3.58096481258059));
#79987=CARTESIAN_POINT('Ctrl Pts',(7.91488010063406,1.52434272008469,3.62742904163521));
#79988=CARTESIAN_POINT('Ctrl Pts',(7.92074431380535,1.41646040001964,3.66907739563725));
#79989=CARTESIAN_POINT('Ctrl Pts',(7.92661716237964,1.30841921681614,3.71078707931985));
#79990=CARTESIAN_POINT('Ctrl Pts',(7.93249001095393,1.19867414164117,3.74766660322759));
#79991=CARTESIAN_POINT('Ctrl Pts',(7.93836285952821,1.08769799126529,3.77960342890593));
#79992=CARTESIAN_POINT('Ctrl Pts',(7.93995760414107,1.05756293572458,3.78827572482132));
#79993=CARTESIAN_POINT('Ctrl Pts',(7.94155234875394,1.02733715418253,3.79658385444725));
#79994=CARTESIAN_POINT('Ctrl Pts',(7.9431470933668,0.997030207319577,3.80452622092321));
#79995=CARTESIAN_POINT('Ctrl Pts',(7.94901953950072,0.88542869350939,3.83377298490644));
#79996=CARTESIAN_POINT('Ctrl Pts',(7.95489198563463,0.772352361360635,3.85815399328153));
#79997=CARTESIAN_POINT('Ctrl Pts',(7.96076443176855,0.658263451059872,3.87752217646769));
#79998=CARTESIAN_POINT('Ctrl Pts',(7.96662927071339,0.544322331967745,3.89686527003564));
#79999=CARTESIAN_POINT('Ctrl Pts',(7.97249410965824,0.429371646992982,3.91120838339557));
#80000=CARTESIAN_POINT('Ctrl Pts',(7.97835894860308,0.31388771359242,3.920454502128));
#80001=CARTESIAN_POINT('Ctrl Pts',(7.9842177587231,0.198522493154094,3.92969111621237));
#80002=CARTESIAN_POINT('Ctrl Pts',(7.99007656884313,0.0826255241719993,
3.93384112455213));
#80003=CARTESIAN_POINT('Ctrl Pts',(7.99593537896315,-0.0333184521080177,
3.93285886865384));
#80004=CARTESIAN_POINT('Ctrl Pts',(8.00202116784412,-0.153754265388441,
3.9318385587442));
#80005=CARTESIAN_POINT('Ctrl Pts',(8.00810695672509,-0.274240353943659,
3.92528020320809));
#80006=CARTESIAN_POINT('Ctrl Pts',(8.01419274560606,-0.394229199108612,
3.91319209068124));
#80007=CARTESIAN_POINT('Ctrl Pts',(8.02004477568432,-0.50960920073134,3.90156828981002));
#80008=CARTESIAN_POINT('Ctrl Pts',(8.0258968057626,-0.624529003870829,3.8848317437445));
#80009=CARTESIAN_POINT('Ctrl Pts',(8.03174883584087,-0.738504434452509,
3.86304286803732));
#80010=CARTESIAN_POINT('Ctrl Pts',(8.03759997621938,-0.852462537045229,
3.84125730495107));
#80011=CARTESIAN_POINT('Ctrl Pts',(8.04345111659789,-0.965476146661259,
3.81442101708987));
#80012=CARTESIAN_POINT('Ctrl Pts',(8.0493022569764,-1.07707013505366,3.78264575716198));
#80013=CARTESIAN_POINT('Ctrl Pts',(8.0551539245439,-1.18867417808802,3.75086763427644));
#80014=CARTESIAN_POINT('Ctrl Pts',(8.0610055921114,-1.29885794805044,3.71414976790702));
#80015=CARTESIAN_POINT('Ctrl Pts',(8.0668572596789,-1.40716104982742,3.67265391506586));
#80016=CARTESIAN_POINT('Ctrl Pts',(8.07271087136315,-1.51550013346278,3.63114427593534));
#80017=CARTESIAN_POINT('Ctrl Pts',(8.0785644830474,-1.62195692070602,3.58485364168991));
#80018=CARTESIAN_POINT('Ctrl Pts',(8.08441809473164,-1.72609124545215,3.53399179574224));
#80019=CARTESIAN_POINT('Ctrl Pts',(8.09027836083153,-1.83034395063028,3.48307212978844));
#80020=CARTESIAN_POINT('Ctrl Pts',(8.09613862693142,-1.93226855194517,3.42757106145758));
#80021=CARTESIAN_POINT('Ctrl Pts',(8.10199889303131,-2.0314496512951,3.3677442471561));
#80022=CARTESIAN_POINT('Ctrl Pts',(8.10786310620262,-2.13069755219898,3.30787713763518));
#80023=CARTESIAN_POINT('Ctrl Pts',(8.11372731937392,-2.22719792841481,3.24367870912619));
#80024=CARTESIAN_POINT('Ctrl Pts',(8.11959153254523,-2.32056597014865,3.17544683126455));
#80025=CARTESIAN_POINT('Ctrl Pts',(8.12546438111952,-2.41407150188209,3.10711447790095));
#80026=CARTESIAN_POINT('Ctrl Pts',(8.13133722969382,-2.50443517199168,3.03473707857497));
#80027=CARTESIAN_POINT('Ctrl Pts',(8.13721007826811,-2.59130665525716,2.95865152027405));
#80028=CARTESIAN_POINT('Ctrl Pts',(8.13880482288089,-2.61489620097573,2.93799084212519));
#80029=CARTESIAN_POINT('Ctrl Pts',(8.14039956749366,-2.63822846324328,2.91705693601381));
#80030=CARTESIAN_POINT('Ctrl Pts',(8.14199431210644,-2.66129692920873,2.89585698103069));
#80031=CARTESIAN_POINT('Ctrl Pts',(8.14777911715162,-2.74497589399877,2.81895588629643));
#80032=CARTESIAN_POINT('Ctrl Pts',(8.15356392219681,-2.82547909158505,2.73827726983921));
#80033=CARTESIAN_POINT('Ctrl Pts',(8.15934872724199,-2.90243816768425,2.65411787281004));
#80034=CARTESIAN_POINT('Ctrl Pts',(8.1651259627185,-2.97929654081986,2.57006860055269));
#80035=CARTESIAN_POINT('Ctrl Pts',(8.17090319819501,-3.05261972432337,2.48254791182106));
#80036=CARTESIAN_POINT('Ctrl Pts',(8.17668043367151,-3.12207335630604,2.39189192018451));
#80037=CARTESIAN_POINT('Ctrl Pts',(8.18245105966144,-3.19144752937611,2.30133964416816));
#80038=CARTESIAN_POINT('Ctrl Pts',(8.18822168565136,-3.25696069928966,2.20765953720203));
#80039=CARTESIAN_POINT('Ctrl Pts',(8.19399231164128,-3.3183169287146,2.11122281169139));
#80040=CARTESIAN_POINT('Ctrl Pts',(8.19975929030372,-3.37963437789929,2.01484703906882));
#80041=CARTESIAN_POINT('Ctrl Pts',(8.20552626896615,-3.43679987836929,1.91571846826686));
#80042=CARTESIAN_POINT('Ctrl Pts',(8.21129324762859,-3.48955952594087,1.81423904569253));
#80043=CARTESIAN_POINT('Ctrl Pts',(8.21705807448063,-3.54229948750974,1.71279748774162));
#80044=CARTESIAN_POINT('Ctrl Pts',(8.22282290133268,-3.59063666711438,1.60900719962662));
#80045=CARTESIAN_POINT('Ctrl Pts',(8.22858772818473,-3.63436248685362,1.50329581724661));
#80046=CARTESIAN_POINT('Ctrl Pts',(8.23435189644263,-3.67808331120104,1.39759651170765));
#80047=CARTESIAN_POINT('Ctrl Pts',(8.24011606470054,-3.7171936615783,1.28997694314073));
#80048=CARTESIAN_POINT('Ctrl Pts',(8.24588023295844,-3.75153295765055,1.18088503575145));
#80049=CARTESIAN_POINT('Ctrl Pts',(8.25164770053762,-3.78589190900785,1.07173068583187));
#80050=CARTESIAN_POINT('Ctrl Pts',(8.2574151681168,-3.81547422276402,0.961102721236819));
#80051=CARTESIAN_POINT('Ctrl Pts',(8.26318263569598,-3.84016919586695,0.849464270652149));
#80052=CARTESIAN_POINT('Ctrl Pts',(8.26895192380287,-3.86487196405191,0.737790580876233));
#80053=CARTESIAN_POINT('Ctrl Pts',(8.27472121190976,-3.88468424346046,0.625106189909439));
#80054=CARTESIAN_POINT('Ctrl Pts',(8.28049050001665,-3.89954676236548,0.511882846093653));
#80055=CARTESIAN_POINT('Ctrl Pts',(8.28626624305139,-3.91442591009634,0.398532823127594));
#80056=CARTESIAN_POINT('Ctrl Pts',(8.29204198608612,-3.92434420267456,0.284643068235318));
#80057=CARTESIAN_POINT('Ctrl Pts',(8.29781772912086,-3.92929438452151,0.170688721852677));
#80058=CARTESIAN_POINT('Ctrl Pts',(8.30075731206894,-3.93181379545439,0.11269129165692));
#80059=CARTESIAN_POINT('Ctrl Pts',(8.30369689501702,-3.93304713651331,0.0546771189250599));
#80060=CARTESIAN_POINT('Ctrl Pts',(8.3066364779651,-3.93299862266704,-0.00329151928449545));
#80061=CARTESIAN_POINT('',(9.55663647796509,-3.93447037223625,0.00250579399543049));
#80062=CARTESIAN_POINT('Ctrl Pts',(8.3066364779651,-3.93541974394845,-0.00329354551642644));
#80063=CARTESIAN_POINT('Ctrl Pts',(8.31803816225876,-3.93743804138694,-0.228275259319388));
#80064=CARTESIAN_POINT('Ctrl Pts',(8.39572225279899,-3.81735299180208,-1.75900887235532));
#80065=CARTESIAN_POINT('Ctrl Pts',(8.53968874958569,-1.80864929602783,-4.28564802508547));
#80066=CARTESIAN_POINT('Ctrl Pts',(8.73853596832538,2.62717012805726,-3.83874567914929));
#80067=CARTESIAN_POINT('Ctrl Pts',(8.93738318706501,4.64972487276848,0.134349836257429));
#80068=CARTESIAN_POINT('Ctrl Pts',(9.13623040580465,2.40113756831285,3.98403434334837));
#80069=CARTESIAN_POINT('Ctrl Pts',(9.3350776245443,-2.05308553492218,4.17406648931669));
#80070=CARTESIAN_POINT('Ctrl Pts',(9.47521298193112,-3.86306683227914,1.60587142326164));
#80071=CARTESIAN_POINT('Ctrl Pts',(9.54906593307138,-3.93857895538214,0.151689483416833));
#80072=CARTESIAN_POINT('Ctrl Pts',(9.55663647796509,-3.93747221447367,0.00250770581520343));
#80073=CARTESIAN_POINT('',(10.8066364494697,-3.93103660093039,0.00204695750207211));
#80074=CARTESIAN_POINT('Ctrl Pts',(9.55663647796509,-3.9329992023507,0.00250485703357371));
#80075=CARTESIAN_POINT('Ctrl Pts',(9.56242578790064,-3.93307177594825,-0.111446517220179));
#80076=CARTESIAN_POINT('Ctrl Pts',(9.56821509783619,-3.92818786930245,-0.225594949222398));
#80077=CARTESIAN_POINT('Ctrl Pts',(9.57400440777174,-3.91832254996172,-0.339466337744191));
#80078=CARTESIAN_POINT('Ctrl Pts',(9.57978709579029,-3.90846851475097,-0.453207478120546));
#80079=CARTESIAN_POINT('Ctrl Pts',(9.58556978380884,-3.89364442876225,-0.566671784410446));
#80080=CARTESIAN_POINT('Ctrl Pts',(9.5913524718274,-3.87387738108328,-0.679384306803833));
#80081=CARTESIAN_POINT('Ctrl Pts',(9.59724495475224,-3.85373501985801,-0.794236882541554));
#80082=CARTESIAN_POINT('Ctrl Pts',(9.60313743767708,-3.828460061154,-0.908308387270493));
#80083=CARTESIAN_POINT('Ctrl Pts',(9.60902992060192,-3.79813674705107,-1.02110050959752));
#80084=CARTESIAN_POINT('Ctrl Pts',(9.61480474556086,-3.76841891276068,-1.13164045879956));
#80085=CARTESIAN_POINT('Ctrl Pts',(9.6205795705198,-3.73385256954763,-1.24095121187066));
#80086=CARTESIAN_POINT('Ctrl Pts',(9.62635439547874,-3.69456856339101,-1.34857411008921));
#80087=CARTESIAN_POINT('Ctrl Pts',(9.63212798143693,-3.65529298569989,-1.45617391759037));
#80088=CARTESIAN_POINT('Ctrl Pts',(9.63790156739512,-3.61130190230417,-1.56208619036244));
#80089=CARTESIAN_POINT('Ctrl Pts',(9.64367515335332,-3.56277550140972,-1.66586906044704));
#80090=CARTESIAN_POINT('Ctrl Pts',(9.64944898682857,-3.51424702015963,-1.76965637976495));
#80091=CARTESIAN_POINT('Ctrl Pts',(9.65522282030383,-3.46118301601565,-1.87131372986746));
#80092=CARTESIAN_POINT('Ctrl Pts',(9.66099665377908,-3.40381076254495,-1.97042160280056));
#80093=CARTESIAN_POINT('Ctrl Pts',(9.66697793779946,-3.34437715671481,-2.07309036510705));
#80094=CARTESIAN_POINT('Ctrl Pts',(9.67295922181983,-3.28032013107761,-2.17302257094501));
#80095=CARTESIAN_POINT('Ctrl Pts',(9.67894050584021,-3.21194202257755,-2.26978356756772));
#80096=CARTESIAN_POINT('Ctrl Pts',(9.68472252244736,-3.14584194146343,-2.36332095644473));
#80097=CARTESIAN_POINT('Ctrl Pts',(9.69050453905452,-3.07570442656063,-2.45389477069358));
#80098=CARTESIAN_POINT('Ctrl Pts',(9.69628655566168,-3.00184350990193,-2.54114630473329));
#80099=CARTESIAN_POINT('Ctrl Pts',(9.70236747338866,-2.92416435607779,-2.63290830337435));
#80100=CARTESIAN_POINT('Ctrl Pts',(9.70844839111565,-2.84236692233796,-2.72099494731911));
#80101=CARTESIAN_POINT('Ctrl Pts',(9.71452930884263,-2.75685898198012,-2.80503432304767));
#80102=CARTESIAN_POINT('Ctrl Pts',(9.72061022656961,-2.6713510416223,-2.88907369877623));
#80103=CARTESIAN_POINT('Ctrl Pts',(9.7266911442966,-2.58213304953528,-2.96906550752146));
#80104=CARTESIAN_POINT('Ctrl Pts',(9.73277206202358,-2.48964991172429,-3.04468919876089));
#80105=CARTESIAN_POINT('Ctrl Pts',(9.7386445081575,-2.40033736557993,-3.11772028932825));
#80106=CARTESIAN_POINT('Ctrl Pts',(9.74451695429143,-2.30765913822446,-3.18694049328549));
#80107=CARTESIAN_POINT('Ctrl Pts',(9.75038940042535,-2.21197436113287,-3.25202374310072));
#80108=CARTESIAN_POINT('Ctrl Pts',(9.7562542393702,-2.11641353446579,-3.31702268382638));
#80109=CARTESIAN_POINT('Ctrl Pts',(9.76211907831504,-2.01785424186353,-3.37789509727265));
#80110=CARTESIAN_POINT('Ctrl Pts',(9.76798391725989,-1.91668924306658,-3.4343545748092));
#80111=CARTESIAN_POINT('Ctrl Pts',(9.77384272737991,-1.81562823792765,-3.49075601421329));
#80112=CARTESIAN_POINT('Ctrl Pts',(9.77970153749994,-1.71196721318701,-3.54275334047334));
#80113=CARTESIAN_POINT('Ctrl Pts',(9.78556034761997,-1.60612795724475,-3.59010333903591));
#80114=CARTESIAN_POINT('Ctrl Pts',(9.79164613650094,-1.49618833575372,-3.63928774489011));
#80115=CARTESIAN_POINT('Ctrl Pts',(9.79773192538191,-1.38389866963451,-3.68345719638661));
#80116=CARTESIAN_POINT('Ctrl Pts',(9.80381771426288,-1.26976027913928,-3.72239141326112));
#80117=CARTESIAN_POINT('Ctrl Pts',(9.80966974434114,-1.16000601271181,-3.75983014350298));
#80118=CARTESIAN_POINT('Ctrl Pts',(9.81552177441941,-1.04854285075996,-3.7924282516616));
#80119=CARTESIAN_POINT('Ctrl Pts',(9.82137380449768,-0.935836202344345,
-3.82003921477015));
#80120=CARTESIAN_POINT('Ctrl Pts',(9.8272249448762,-0.823146689021302,-3.84764598011028));
#80121=CARTESIAN_POINT('Ctrl Pts',(9.83307608525471,-0.709214466503963,
-3.87026700963775));
#80122=CARTESIAN_POINT('Ctrl Pts',(9.83892722563323,-0.594518079174452,
-3.88780622633571));
#80123=CARTESIAN_POINT('Ctrl Pts',(9.84477889320072,-0.479811357676326,
-3.90534702332079));
#80124=CARTESIAN_POINT('Ctrl Pts',(9.85063056076822,-0.364340743127473,
-3.91780503478093));
#80125=CARTESIAN_POINT('Ctrl Pts',(9.85648222833571,-0.248592189045484,
-3.92513578409022));
#80126=CARTESIAN_POINT('Ctrl Pts',(9.86233584001997,-0.132805179480328,
-3.93246896891596));
#80127=CARTESIAN_POINT('Ctrl Pts',(9.86818945170422,-0.0167404590803251,
-3.93467147828041));
#80128=CARTESIAN_POINT('Ctrl Pts',(9.87404306338847,0.0991144300150325,
-3.9317509241765));
#80129=CARTESIAN_POINT('Ctrl Pts',(9.87990332948836,0.215101023539559,-3.92882704997179));
#80130=CARTESIAN_POINT('Ctrl Pts',(9.88576359558825,0.33087689617723,-3.92076849836277));
#80131=CARTESIAN_POINT('Ctrl Pts',(9.89162386168814,0.445957940592019,-3.90763490045103));
#80132=CARTESIAN_POINT('Ctrl Pts',(9.89748807485944,0.561116495668119,-3.89449245665277));
#80133=CARTESIAN_POINT('Ctrl Pts',(9.90335228803074,0.675578883445476,-3.87626822506084));
#80134=CARTESIAN_POINT('Ctrl Pts',(9.90921650120204,0.788871246722858,-3.85307294974984));
#80135=CARTESIAN_POINT('Ctrl Pts',(9.91508934977633,0.902330439749382,-3.82984351801515));
#80136=CARTESIAN_POINT('Ctrl Pts',(9.92096219835063,1.01461577026381,-3.80162853334182));
#80137=CARTESIAN_POINT('Ctrl Pts',(9.92683504692492,1.12526850393877,-3.76858856789162));
#80138=CARTESIAN_POINT('Ctrl Pts',(9.92842979153769,1.15531573718245,-3.75961671952173));
#80139=CARTESIAN_POINT('Ctrl Pts',(9.93002453615046,1.18524270417137,-3.75028936542526));
#80140=CARTESIAN_POINT('Ctrl Pts',(9.93161928076323,1.21504049546738,-3.74061032378065));
#80141=CARTESIAN_POINT('Ctrl Pts',(9.93749172689715,1.32476710805129,-3.70496847226986));
#80142=CARTESIAN_POINT('Ctrl Pts',(9.94336417303108,1.43310782714073,-3.66443479431161));
#80143=CARTESIAN_POINT('Ctrl Pts',(9.949236619165,1.53959417575555,-3.61913508645085));
#80144=CARTESIAN_POINT('Ctrl Pts',(9.95510145810985,1.64594258154894,-3.57389406000412));
#80145=CARTESIAN_POINT('Ctrl Pts',(9.96096629705469,1.75044101704354,-3.52389944173168));
#80146=CARTESIAN_POINT('Ctrl Pts',(9.96683113599954,1.85263618353321,-3.4693267605493));
#80147=CARTESIAN_POINT('Ctrl Pts',(9.97268994611955,1.9547262973925,-3.41481017794675));
#80148=CARTESIAN_POINT('Ctrl Pts',(9.97854875623955,2.05451748923695,-3.35572508660673));
#80149=CARTESIAN_POINT('Ctrl Pts',(9.98440756635956,2.15157709950946,-3.29229479009193));
#80150=CARTESIAN_POINT('Ctrl Pts',(9.99049335524053,2.25239693918485,-3.22640711233154));
#80151=CARTESIAN_POINT('Ctrl Pts',(9.9965791441215,2.35026884774362,-3.15583091891095));
#80152=CARTESIAN_POINT('Ctrl Pts',(10.0026649330025,2.44473645447035,-3.08086881710074));
#80153=CARTESIAN_POINT('Ctrl Pts',(10.0085169630807,2.53557550373734,-3.00878605460214));
#80154=CARTESIAN_POINT('Ctrl Pts',(10.014368993159,2.6232665958657,-2.93264838003059));
#80155=CARTESIAN_POINT('Ctrl Pts',(10.0202210232373,2.70743482298513,-2.85276807316814));
#80156=CARTESIAN_POINT('Ctrl Pts',(10.0260721636158,2.79159025378436,-2.77289991072193));
#80157=CARTESIAN_POINT('Ctrl Pts',(10.0319233039943,2.87222358476016,-2.68929053181993));
#80158=CARTESIAN_POINT('Ctrl Pts',(10.0377744443728,2.94899524122218,-2.60229054243544));
#80159=CARTESIAN_POINT('Ctrl Pts',(10.0436261119403,3.02577381482653,-2.51528271433368));
#80160=CARTESIAN_POINT('Ctrl Pts',(10.0494777795078,3.09868974873285,-2.42488397841122));
#80161=CARTESIAN_POINT('Ctrl Pts',(10.0553294470753,3.16744286876422,-2.33147907413184));
#80162=CARTESIAN_POINT('Ctrl Pts',(10.0611830587595,3.23621883084693,-2.23804313766632));
#80163=CARTESIAN_POINT('Ctrl Pts',(10.0670366704437,3.30082898408807,-2.14159937961505));
#80164=CARTESIAN_POINT('Ctrl Pts',(10.072890282128,3.36101611273705,-2.04256204065431));
#80165=CARTESIAN_POINT('Ctrl Pts',(10.0787505482279,3.42127166242138,-1.94341211554066));
#80166=CARTESIAN_POINT('Ctrl Pts',(10.0846108143278,3.47709393676087,-1.8416630780679));
#80167=CARTESIAN_POINT('Ctrl Pts',(10.0904710804276,3.52827133617625,-1.73775440678971));
#80168=CARTESIAN_POINT('Ctrl Pts',(10.0963352935989,3.57948320516119,-1.633775749791));
#80169=CARTESIAN_POINT('Ctrl Pts',(10.1021995067702,3.62604380416773,-1.52763494023623));
#80170=CARTESIAN_POINT('Ctrl Pts',(10.1080637199415,3.66779007265798,-1.41979047148216));
#80171=CARTESIAN_POINT('Ctrl Pts',(10.1139365685158,3.70959781501364,-1.31178719532815));
#80172=CARTESIAN_POINT('Ctrl Pts',(10.1198094170901,3.74657694631575,-1.20207564326126));
#80173=CARTESIAN_POINT('Ctrl Pts',(10.1256822656644,3.77861449895025,-1.09112852969892));
#80174=CARTESIAN_POINT('Ctrl Pts',(10.1272770102772,3.78731414680017,-1.06100135896997));
#80175=CARTESIAN_POINT('Ctrl Pts',(10.12887175489,3.79564971086845,-1.03078313170016));
#80176=CARTESIAN_POINT('Ctrl Pts',(10.1304664995029,3.80361958561641,-1.0004834071164));
#80177=CARTESIAN_POINT('Ctrl Pts',(10.1363389456368,3.83296764534644,-0.888908488437121));
#80178=CARTESIAN_POINT('Ctrl Pts',(10.1422113917707,3.85745129025957,-0.775854335070879));
#80179=CARTESIAN_POINT('Ctrl Pts',(10.1480838379046,3.8769230312308,-0.661783053509366));
#80180=CARTESIAN_POINT('Ctrl Pts',(10.1539486768494,3.89636954843464,-0.547859540320254));
#80181=CARTESIAN_POINT('Ctrl Pts',(10.1598135157943,3.91081700393777,-0.432921922864211));
#80182=CARTESIAN_POINT('Ctrl Pts',(10.1656783547391,3.92016795097699,-0.317446430335651));
#80183=CARTESIAN_POINT('Ctrl Pts',(10.1715371648591,3.92950928560874,-0.202089642092598));
#80184=CARTESIAN_POINT('Ctrl Pts',(10.1773959749791,3.93376449929369,-0.0861964880890872));
#80185=CARTESIAN_POINT('Ctrl Pts',(10.1832547850991,3.9328874935267,0.0297483320758639));
#80186=CARTESIAN_POINT('Ctrl Pts',(10.1893405739801,3.93197651129038,0.150185021934936));
#80187=CARTESIAN_POINT('Ctrl Pts',(10.1954263628611,3.92552753134741,0.270677014284574));
#80188=CARTESIAN_POINT('Ctrl Pts',(10.2015121517421,3.91354834531258,0.390676783161187));
#80189=CARTESIAN_POINT('Ctrl Pts',(10.2073641818203,3.90202928700147,0.50606728890923));
#80190=CARTESIAN_POINT('Ctrl Pts',(10.2132162118986,3.88539706785114,0.621002237527868));
#80191=CARTESIAN_POINT('Ctrl Pts',(10.2190682419769,3.86371166387371,0.73499740029896));
#80192=CARTESIAN_POINT('Ctrl Pts',(10.2249193823554,3.84202955678616,0.848975232081036));
#80193=CARTESIAN_POINT('Ctrl Pts',(10.2307705227339,3.81529586962827,0.962013156139898));
#80194=CARTESIAN_POINT('Ctrl Pts',(10.2366216631124,3.78362192375809,1.07363594297933));
#80195=CARTESIAN_POINT('Ctrl Pts',(10.2424733306799,3.75194512405866,1.18526878705557));
#80196=CARTESIAN_POINT('Ctrl Pts',(10.2483249982474,3.71532729363835,1.2954858427646));
#80197=CARTESIAN_POINT('Ctrl Pts',(10.2541766658149,3.6739297715127,1.40382656834547));
#80198=CARTESIAN_POINT('Ctrl Pts',(10.2600302774992,3.63251849576636,1.5122032882847));
#80199=CARTESIAN_POINT('Ctrl Pts',(10.2658838891834,3.5863245181947,1.61870205262089));
#80200=CARTESIAN_POINT('Ctrl Pts',(10.2717375008677,3.5355572225572,1.72288250499667));
#80201=CARTESIAN_POINT('Ctrl Pts',(10.2775977669676,3.48473221439894,1.82718139024236));
#80202=CARTESIAN_POINT('Ctrl Pts',(10.2834580330675,3.42932369238321,1.92915633141456));
#80203=CARTESIAN_POINT('Ctrl Pts',(10.2893182991673,3.3695869357278,2.0283916985071));
#80204=CARTESIAN_POINT('Ctrl Pts',(10.2951825123387,3.30980994450955,2.12769390370464));
#80205=CARTESIAN_POINT('Ctrl Pts',(10.30104672551,3.24569914198479,2.22425251716007));
#80206=CARTESIAN_POINT('Ctrl Pts',(10.3069109386813,3.17755204834987,2.31768245884278));
#80207=CARTESIAN_POINT('Ctrl Pts',(10.3127837872556,3.10930460406272,2.41124998167659));
#80208=CARTESIAN_POINT('Ctrl Pts',(10.3186566358299,3.03700926341205,2.50167931612669));
#80209=CARTESIAN_POINT('Ctrl Pts',(10.3245294844042,2.961002595234,2.58861983130345));
#80210=CARTESIAN_POINT('Ctrl Pts',(10.326124229017,2.94036333932942,2.61222812231557));
#80211=CARTESIAN_POINT('Ctrl Pts',(10.3277189736297,2.91945062202231,2.6355793780091));
#80212=CARTESIAN_POINT('Ctrl Pts',(10.3293137182425,2.89827161648838,2.6586670790187));
#80213=CARTESIAN_POINT('Ctrl Pts',(10.3351861643765,2.82028259669823,2.74368462944437));
#80214=CARTESIAN_POINT('Ctrl Pts',(10.3410586105104,2.73841899260408,2.82541002810544));
#80215=CARTESIAN_POINT('Ctrl Pts',(10.3469310566443,2.65298978342595,2.90346934012356));
#80216=CARTESIAN_POINT('Ctrl Pts',(10.3527958955891,2.56767123957049,2.98142753381183));
#80217=CARTESIAN_POINT('Ctrl Pts',(10.358660734534,2.47879657831782,3.05572880879589));
#80218=CARTESIAN_POINT('Ctrl Pts',(10.3645255734788,2.38671371744883,3.12603368998826));
#80219=CARTESIAN_POINT('Ctrl Pts',(10.3703843835989,2.29472551415571,3.19626630051523));
#80220=CARTESIAN_POINT('Ctrl Pts',(10.3762431937189,2.19953599752989,3.26251043922199));
#80221=CARTESIAN_POINT('Ctrl Pts',(10.3821020038389,2.10152797526098,3.32446524559898));
#80222=CARTESIAN_POINT('Ctrl Pts',(10.3881877927199,1.99972298073973,3.38882027060366));
#80223=CARTESIAN_POINT('Ctrl Pts',(10.3942735816008,1.89487701320576,3.44854658519396));
#80224=CARTESIAN_POINT('Ctrl Pts',(10.4003593704818,1.78745486938629,3.50335469085094));
#80225=CARTESIAN_POINT('Ctrl Pts',(10.4062114005601,1.68415887456965,3.55605758428199));
#80226=CARTESIAN_POINT('Ctrl Pts',(10.4120634306383,1.57848136005072,3.60421291683126));
#80227=CARTESIAN_POINT('Ctrl Pts',(10.4179154607166,1.47086209298752,3.64760931342878));
#80228=CARTESIAN_POINT('Ctrl Pts',(10.4237666010951,1.36325918756878,3.69099911235628));
#80229=CARTESIAN_POINT('Ctrl Pts',(10.4296177414736,1.25371549983707,3.72963125936829));
#80230=CARTESIAN_POINT('Ctrl Pts',(10.4354688818521,1.14269098967903,3.76334243752895));
#80231=CARTESIAN_POINT('Ctrl Pts',(10.4413205494197,1.03165647618905,3.79705665307392));
#80232=CARTESIAN_POINT('Ctrl Pts',(10.4471722169872,0.919141270591103,3.82584889826477));
#80233=CARTESIAN_POINT('Ctrl Pts',(10.4530238845547,0.805620022377508,3.84960587327384));
#80234=CARTESIAN_POINT('Ctrl Pts',(10.4588774962389,0.692061058666013,3.87337074113254));
#80235=CARTESIAN_POINT('Ctrl Pts',(10.4647311079231,0.577495792100148,3.89209692775887));
#80236=CARTESIAN_POINT('Ctrl Pts',(10.4705847196073,0.462407870315806,3.90572246344642));
#80237=CARTESIAN_POINT('Ctrl Pts',(10.4764449857072,0.347189115993989,3.91936348871256));
#80238=CARTESIAN_POINT('Ctrl Pts',(10.4823052518071,0.231446931268476,3.92789224090785));
#80239=CARTESIAN_POINT('Ctrl Pts',(10.488165517907,0.115668979892364,3.93129872778585));
#80240=CARTESIAN_POINT('Ctrl Pts',(10.4940297310783,-0.000186951534076524,
3.93470750903869));
#80241=CARTESIAN_POINT('Ctrl Pts',(10.4998939442496,-0.116078285278519,
3.93298716144111));
#80242=CARTESIAN_POINT('Ctrl Pts',(10.5057581574209,-0.23152021637001,3.92617974491897));
#80243=CARTESIAN_POINT('Ctrl Pts',(10.5116310059952,-0.347132142576803,
3.91936230407078));
#80244=CARTESIAN_POINT('Ctrl Pts',(10.5175038545695,-0.462292935751987,
3.90744288612649));
#80245=CARTESIAN_POINT('Ctrl Pts',(10.5233767031438,-0.576525655849704,
3.89051502607908));
#80246=CARTESIAN_POINT('Ctrl Pts',(10.5249714477566,-0.607545017693227,
3.88591834471144));
#80247=CARTESIAN_POINT('Ctrl Pts',(10.5265661923694,-0.638496022515862,
3.88095264354574));
#80248=CARTESIAN_POINT('Ctrl Pts',(10.5281609369822,-0.669369307559842,
3.87562043163373));
#80249=CARTESIAN_POINT('Ctrl Pts',(10.5340333831161,-0.783056290381801,
3.85598523300877));
#80250=CARTESIAN_POINT('Ctrl Pts',(10.53990582925,-0.89606891319852,3.83131059936058));
#80251=CARTESIAN_POINT('Ctrl Pts',(10.5457782753839,-1.00792555042906,3.80165425634582));
#80252=CARTESIAN_POINT('Ctrl Pts',(10.5516431143287,-1.11963728814594,3.77203633027068));
#80253=CARTESIAN_POINT('Ctrl Pts',(10.5575079532736,-1.23019562233906,3.73744963315401));
#80254=CARTESIAN_POINT('Ctrl Pts',(10.5633727922184,-1.33912686083216,3.69800327887872));
#80255=CARTESIAN_POINT('Ctrl Pts',(10.5692316023384,-1.44794612227647,3.65859747391141));
#80256=CARTESIAN_POINT('Ctrl Pts',(10.5750904124584,-1.55514122856975,3.61434208807975));
#80257=CARTESIAN_POINT('Ctrl Pts',(10.5809492225784,-1.66025210513203,3.56539646426658));
#80258=CARTESIAN_POINT('Ctrl Pts',(10.5870350114594,-1.76943512877518,3.51455461633608));
#80259=CARTESIAN_POINT('Ctrl Pts',(10.5931208003404,-1.87636872520191,3.45865188368426));
#80260=CARTESIAN_POINT('Ctrl Pts',(10.5992065892213,-1.98055804532792,3.39792272264789));
#80261=CARTESIAN_POINT('Ctrl Pts',(10.6050586192996,-2.08074539114887,3.33952620512759));
#80262=CARTESIAN_POINT('Ctrl Pts',(10.6109106493779,-2.17839500030641,3.27666741927234));
#80263=CARTESIAN_POINT('Ctrl Pts',(10.6167626794561,-2.27309127560223,3.20960200847099));
#80264=CARTESIAN_POINT('Ctrl Pts',(10.6226138198347,-2.36777315397059,3.14254679380303));
#80265=CARTESIAN_POINT('Ctrl Pts',(10.6284649602132,-2.45950225400597,3.07128646464774));
#80266=CARTESIAN_POINT('Ctrl Pts',(10.6343161005917,-2.54789248702578,2.99611963622242));
#80267=CARTESIAN_POINT('Ctrl Pts',(10.6401677681592,-2.6362906840246,2.9209460352497));
#80268=CARTESIAN_POINT('Ctrl Pts',(10.6460194357267,-2.72134910107028,2.84186550310911));
#80269=CARTESIAN_POINT('Ctrl Pts',(10.6518711032943,-2.80271578149733,2.75921605680777));
#80270=CARTESIAN_POINT('Ctrl Pts',(10.6577247149785,-2.88410949461566,2.67653915163807));
#80271=CARTESIAN_POINT('Ctrl Pts',(10.6635783266627,-2.96180874242292,2.59029126900251));
#80272=CARTESIAN_POINT('Ctrl Pts',(10.669431938347,-3.03549988222078,2.50084574994893));
#80273=CARTESIAN_POINT('Ctrl Pts',(10.6752922044469,-3.10927479448281,2.41129854877237));
#80274=CARTESIAN_POINT('Ctrl Pts',(10.6811524705468,-3.17903224124492,2.31854677487927));
#80275=CARTESIAN_POINT('Ctrl Pts',(10.6870127366467,-3.24450013215575,2.22299525245587));
#80276=CARTESIAN_POINT('Ctrl Pts',(10.692876949818,-3.31001211772647,2.12737937311147));
#80277=CARTESIAN_POINT('Ctrl Pts',(10.6987411629893,-3.37122857678235,2.02896034053399));
#80278=CARTESIAN_POINT('Ctrl Pts',(10.7046053761606,-3.42792275149611,1.92816871921918));
#80279=CARTESIAN_POINT('Ctrl Pts',(10.7104782247349,-3.48470041175713,1.82722867624189));
#80280=CARTESIAN_POINT('Ctrl Pts',(10.7163510733092,-3.53694231115576,1.7239094391362));
#80281=CARTESIAN_POINT('Ctrl Pts',(10.7222239218835,-3.58446924579559,1.61866278944863));
#80282=CARTESIAN_POINT('Ctrl Pts',(10.7238186664962,-3.5973749630162,1.59008355307292));
#80283=CARTESIAN_POINT('Ctrl Pts',(10.725413411109,-3.60993329615207,1.56136228644923));
#80284=CARTESIAN_POINT('Ctrl Pts',(10.7270081557218,-3.6221412933009,1.53250822228284));
#80285=CARTESIAN_POINT('Ctrl Pts',(10.7336438455333,-3.67293844392245,1.41244723065286));
#80286=CARTESIAN_POINT('Ctrl Pts',(10.7402795353448,-3.71781296604215,1.28973834100993));
#80287=CARTESIAN_POINT('Ctrl Pts',(10.7469152251562,-3.75651119405273,1.16495177967011));
#80288=CARTESIAN_POINT('Ctrl Pts',(10.753420604165,-3.79444947135759,1.04261576038941));
#80289=CARTESIAN_POINT('Ctrl Pts',(10.7599259831737,-3.82645164497718,0.918283160435526));
#80290=CARTESIAN_POINT('Ctrl Pts',(10.7664313621825,-3.85232520642628,0.79251467111511));
#80291=CARTESIAN_POINT('Ctrl Pts',(10.7731322073953,-3.87897618712105,0.662967233763629));
#80292=CARTESIAN_POINT('Ctrl Pts',(10.7798330526081,-3.89912430388189,0.531896459975942));
#80293=CARTESIAN_POINT('Ctrl Pts',(10.7865338978209,-3.91261283787805,0.399937221163387));
#80294=CARTESIAN_POINT('Ctrl Pts',(10.7932347430338,-3.92610137187421,0.267977982350833));
#80295=CARTESIAN_POINT('Ctrl Pts',(10.7999355882466,-3.93293015768591,0.13513055279225));
#80296=CARTESIAN_POINT('Ctrl Pts',(10.8066364334594,-3.93299946662572,0.00204829729017384));
#80297=CARTESIAN_POINT('',(12.0566365093898,-3.93228720468563,-0.00328288393016922));
#80298=CARTESIAN_POINT('Ctrl Pts',(10.8066364779651,-3.92754306292935,0.00204457292697976));
#80299=CARTESIAN_POINT('Ctrl Pts',(10.8463761101305,-3.92384443896021,-0.786112286478094));
#80300=CARTESIAN_POINT('Ctrl Pts',(10.9523981485427,-3.31103251769868,-2.89414287706054));
#80301=CARTESIAN_POINT('Ctrl Pts',(11.124702593201,0.130128929703057,-4.64984491489734));
#80302=CARTESIAN_POINT('Ctrl Pts',(11.3235498119408,3.98185303646486,-2.40475314054045));
#80303=CARTESIAN_POINT('Ctrl Pts',(11.5223970306803,4.1759284859373,2.04929562320325));
#80304=CARTESIAN_POINT('Ctrl Pts',(11.7212442494201,0.534081544591076,4.62090339378258));
#80305=CARTESIAN_POINT('Ctrl Pts',(11.8993240651815,-3.16677355483953,3.122576578027));
#80306=CARTESIAN_POINT('Ctrl Pts',(12.0111214746966,-3.92290114994221,0.898019261252334));
#80307=CARTESIAN_POINT('Ctrl Pts',(12.0566364779651,-3.92997078819238,-0.00328032767339696));
#80308=CARTESIAN_POINT('',(13.3066364779246,-3.93299994461018,-0.000660072963464881));
#80309=CARTESIAN_POINT('Ctrl Pts',(12.056636519041,-3.93299862922908,-0.00328366901515391));
#80310=CARTESIAN_POINT('Ctrl Pts',(12.0635891360599,-3.93288359427993,-0.141066221162596));
#80311=CARTESIAN_POINT('Ctrl Pts',(12.0705417530788,-3.92552444896857,-0.278537064495642));
#80312=CARTESIAN_POINT('Ctrl Pts',(12.0774943700977,-3.9110422068447,-0.415015489204126));
#80313=CARTESIAN_POINT('Ctrl Pts',(12.0845298037661,-3.89638745834408,-0.55311958750304));
#80314=CARTESIAN_POINT('Ctrl Pts',(12.0915652374345,-3.87443898224943,-0.69020742892668));
#80315=CARTESIAN_POINT('Ctrl Pts',(12.0986006711029,-3.84537148345569,-0.825595030402807));
#80316=CARTESIAN_POINT('Ctrl Pts',(12.1053800097017,-3.81736206344984,-0.956054421499278));
#80317=CARTESIAN_POINT('Ctrl Pts',(12.1121593483005,-3.78274283410755,-1.08493521447258));
#80318=CARTESIAN_POINT('Ctrl Pts',(12.1189386868992,-3.741711752173,-1.21164440478651));
#80319=CARTESIAN_POINT('Ctrl Pts',(12.1248111330331,-3.70616952117716,-1.321403326538));
#80320=CARTESIAN_POINT('Ctrl Pts',(12.130683579167,-3.66573420768565,-1.42978079598826));
#80321=CARTESIAN_POINT('Ctrl Pts',(12.136556025301,-3.62053118292523,-1.53630822215661));
#80322=CARTESIAN_POINT('Ctrl Pts',(12.1424208642458,-3.57538671433511,-1.64269765229173));
#80323=CARTESIAN_POINT('Ctrl Pts',(12.1482857031906,-3.52548697654204,-1.74724142802812));
#80324=CARTESIAN_POINT('Ctrl Pts',(12.1541505421355,-3.47100708690141,-1.84948609150764));
#80325=CARTESIAN_POINT('Ctrl Pts',(12.1600093522555,-3.41658320045438,-1.95162565147609));
#80326=CARTESIAN_POINT('Ctrl Pts',(12.1658681623755,-3.35758872027433,-2.05147043750303));
#80327=CARTESIAN_POINT('Ctrl Pts',(12.1717269724956,-3.29424655707933,-2.14858758750277));
#80328=CARTESIAN_POINT('Ctrl Pts',(12.1778127613765,-3.22845042705099,-2.24946719607712));
#80329=CARTESIAN_POINT('Ctrl Pts',(12.1838985502575,-3.15796310726952,-2.34740313081352));
#80330=CARTESIAN_POINT('Ctrl Pts',(12.1899843391385,-3.08308679060405,-2.44193874648871));
#80331=CARTESIAN_POINT('Ctrl Pts',(12.1958363692168,-3.01108651819134,-2.53284319243957));
#80332=CARTESIAN_POINT('Ctrl Pts',(12.201688399295,-2.93502847777535,-2.62060336345059));
#80333=CARTESIAN_POINT('Ctrl Pts',(12.2075404293733,-2.8552246086817,-2.70484406832971));
#80334=CARTESIAN_POINT('Ctrl Pts',(12.2133915697518,-2.7754328723833,-2.7890719658696));
#80335=CARTESIAN_POINT('Ctrl Pts',(12.2192427101303,-2.69189672393637,-2.86978116117752));
#80336=CARTESIAN_POINT('Ctrl Pts',(12.2250938505088,-2.60496646091622,-2.9466317614357));
#80337=CARTESIAN_POINT('Ctrl Pts',(12.2309455180763,-2.51802836546109,-3.02348928594911));
#80338=CARTESIAN_POINT('Ctrl Pts',(12.2367971856438,-2.42769585721846,-3.09648725049883));
#80339=CARTESIAN_POINT('Ctrl Pts',(12.2426488532113,-2.33435340300642,-3.1653251317791));
#80340=CARTESIAN_POINT('Ctrl Pts',(12.2485024648956,-2.24097993735587,-3.23418588327142));
#80341=CARTESIAN_POINT('Ctrl Pts',(12.2543560765798,-2.14459486978902,-3.29888355802961));
#80342=CARTESIAN_POINT('Ctrl Pts',(12.2602096882641,-2.04561220732036,-3.35916056437645));
#80343=CARTESIAN_POINT('Ctrl Pts',(12.266069954364,-1.94651702085566,-3.41950609393184));
#80344=CARTESIAN_POINT('Ctrl Pts',(12.2719302204639,-1.84481869873655,-3.47542070934868));
#80345=CARTESIAN_POINT('Ctrl Pts',(12.2777904865638,-1.74095652725323,-3.52669241219225));
#80346=CARTESIAN_POINT('Ctrl Pts',(12.2836546997351,-1.63702440136828,-3.57799864812175));
#80347=CARTESIAN_POINT('Ctrl Pts',(12.2895189129064,-1.53092590156432,-3.62465557871271));
#80348=CARTESIAN_POINT('Ctrl Pts',(12.2953831260777,-1.42311937298879,-3.66649972729087));
#80349=CARTESIAN_POINT('Ctrl Pts',(12.301255974652,-1.31515409288238,-3.70840549386871));
#80350=CARTESIAN_POINT('Ctrl Pts',(12.3071288232263,-1.20547615432937,-3.74548420209323));
#80351=CARTESIAN_POINT('Ctrl Pts',(12.3130016718006,-1.0945581690045,-3.77762245528395));
#80352=CARTESIAN_POINT('Ctrl Pts',(12.3145964164134,-1.06443890791312,-3.78634944789959));
#80353=CARTESIAN_POINT('Ctrl Pts',(12.3161911610262,-1.03422825981636,-3.79471243954144));
#80354=CARTESIAN_POINT('Ctrl Pts',(12.317785905639,-1.00393578247977,-3.80270981599395));
#80355=CARTESIAN_POINT('Ctrl Pts',(12.3236583517729,-0.892387550872972,
-3.83215914728696));
#80356=CARTESIAN_POINT('Ctrl Pts',(12.3295307979068,-0.779355669449756,
-3.85674540856278));
#80357=CARTESIAN_POINT('Ctrl Pts',(12.3354032440407,-0.665302110626149,
-3.87632069127367));
#80358=CARTESIAN_POINT('Ctrl Pts',(12.3412680829856,-0.551396297216714,
-3.89587061608884));
#80359=CARTESIAN_POINT('Ctrl Pts',(12.3471329219304,-0.436471841991697,
-3.91042240182997));
#80360=CARTESIAN_POINT('Ctrl Pts',(12.3529977608753,-0.321004885490681,
-3.91987816947046));
#80361=CARTESIAN_POINT('Ctrl Pts',(12.3588565709953,-0.205656624500349,
-3.92932421695202));
#80362=CARTESIAN_POINT('Ctrl Pts',(12.3647153811153,-0.0897673809748686,
-3.93368463247566));
#80363=CARTESIAN_POINT('Ctrl Pts',(12.3705741912353,0.0261781875330107,
-3.93291287756257));
#80364=CARTESIAN_POINT('Ctrl Pts',(12.3766599801163,0.14661565472656,-3.93211122375015));
#80365=CARTESIAN_POINT('Ctrl Pts',(12.3827457689973,0.267113451580874,-3.92577162471444));
#80366=CARTESIAN_POINT('Ctrl Pts',(12.3888315578782,0.387124045285005,-3.91390137504283));
#80367=CARTESIAN_POINT('Ctrl Pts',(12.3946835879565,0.502524960072433,-3.90248706878387));
#80368=CARTESIAN_POINT('Ctrl Pts',(12.4005356180348,0.617474959459671,-3.88595919025421));
#80369=CARTESIAN_POINT('Ctrl Pts',(12.406387648113,0.731489760484053,-3.86437727587602));
#80370=CARTESIAN_POINT('Ctrl Pts',(12.4122387884915,0.845487227533909,-3.84279864265388));
#80371=CARTESIAN_POINT('Ctrl Pts',(12.41808992887,0.95854937288855,-3.81616757822868));
#80372=CARTESIAN_POINT('Ctrl Pts',(12.4239410692485,1.07020086619408,-3.78459497251654));
#80373=CARTESIAN_POINT('Ctrl Pts',(12.429792736816,1.18186241932278,-3.75301952210593));
#80374=CARTESIAN_POINT('Ctrl Pts',(12.4356444043835,1.29211266995565,-3.71650175780903));
#80375=CARTESIAN_POINT('Ctrl Pts',(12.441496071951,1.40049093006382,-3.67520260051184));
#80376=CARTESIAN_POINT('Ctrl Pts',(12.4473496836353,1.50890519700026,-3.63388972227409));
#80377=CARTESIAN_POINT('Ctrl Pts',(12.4532032953195,1.61544585067027,-3.58779243944179));
#80378=CARTESIAN_POINT('Ctrl Pts',(12.4590569070037,1.71967234482693,-3.53711973594865));
#80379=CARTESIAN_POINT('Ctrl Pts',(12.4649171731036,1.82401732419438,-3.48638942746741));
#80380=CARTESIAN_POINT('Ctrl Pts',(12.4707774392035,1.92604252119309,-3.43107349742524));
#80381=CARTESIAN_POINT('Ctrl Pts',(12.4766377053034,2.02533207425494,-3.37142684764095));
#80382=CARTESIAN_POINT('Ctrl Pts',(12.4825019184747,2.12468850191775,-3.31174002398357));
#80383=CARTESIAN_POINT('Ctrl Pts',(12.488366131646,2.22130527304521,-3.24771690027245));
#80384=CARTESIAN_POINT('Ctrl Pts',(12.4942303448173,2.31479703768735,-3.17965464701969));
#80385=CARTESIAN_POINT('Ctrl Pts',(12.5001031933916,2.40842647451834,-3.11149216804737));
#80386=CARTESIAN_POINT('Ctrl Pts',(12.5059760419659,2.49892139879179,-3.03927894564602));
#80387=CARTESIAN_POINT('Ctrl Pts',(12.5118488905401,2.58593087423756,-2.96335123022314));
#80388=CARTESIAN_POINT('Ctrl Pts',(12.5134436351529,2.60955789108877,-2.94273341357065));
#80389=CARTESIAN_POINT('Ctrl Pts',(12.5150383797657,2.6329281209656,-2.92184190230099));
#80390=CARTESIAN_POINT('Ctrl Pts',(12.5166331243785,2.65603503799387,-2.90068386366886));
#80391=CARTESIAN_POINT('Ctrl Pts',(12.5225055705125,2.74112334898775,-2.822772051853));
#80392=CARTESIAN_POINT('Ctrl Pts',(12.5283780166464,2.82292302678023,-2.74098266883384));
#80393=CARTESIAN_POINT('Ctrl Pts',(12.5342504627803,2.9010598561669,-2.65562435425963));
#80394=CARTESIAN_POINT('Ctrl Pts',(12.5401153017251,2.97909546680741,-2.57037661317097));
#80395=CARTESIAN_POINT('Ctrl Pts',(12.54598014067,3.05347738836451,-2.48156943653244));
#80396=CARTESIAN_POINT('Ctrl Pts',(12.5518449796148,3.12386583006348,-2.38955043381842));
#80397=CARTESIAN_POINT('Ctrl Pts',(12.5577037897349,3.19418191520013,-2.2976260230366));
#80398=CARTESIAN_POINT('Ctrl Pts',(12.5635625998549,3.26051243619574,-2.20249667965134));
#80399=CARTESIAN_POINT('Ctrl Pts',(12.5694214099749,3.32255618516582,-2.10454493808433));
#80400=CARTESIAN_POINT('Ctrl Pts',(12.5755071988559,3.38700359852803,-2.00279840466059));
#80401=CARTESIAN_POINT('Ctrl Pts',(12.5815929877368,3.44682506386771,-1.89800669770205));
#80402=CARTESIAN_POINT('Ctrl Pts',(12.5876787766178,3.50173066085964,-1.79063435094816));
#80403=CARTESIAN_POINT('Ctrl Pts',(12.5935308066961,3.55452730092494,-1.68738624046198));
#80404=CARTESIAN_POINT('Ctrl Pts',(12.5993828367744,3.60277854383915,-1.58175248314428));
#80405=CARTESIAN_POINT('Ctrl Pts',(12.6052348668526,3.64627261541475,-1.4741726540933));
#80406=CARTESIAN_POINT('Ctrl Pts',(12.6110860072312,3.68976007447055,-1.36660918069089));
#80407=CARTESIAN_POINT('Ctrl Pts',(12.6169371476097,3.72849164534272,-1.2571006069517));
#80408=CARTESIAN_POINT('Ctrl Pts',(12.6227882879882,3.76230359362784,-1.14610674431968));
#80409=CARTESIAN_POINT('Ctrl Pts',(12.6286399555557,3.79611858837664,-1.03510288111719));
#80410=CARTESIAN_POINT('Ctrl Pts',(12.6344916231232,3.82501295891772,-0.922613858431041));
#80411=CARTESIAN_POINT('Ctrl Pts',(12.6403432906907,3.84887297460058,-0.809114222708547));
#80412=CARTESIAN_POINT('Ctrl Pts',(12.6461969023749,3.87274091736668,-0.695576878668005));
#80413=CARTESIAN_POINT('Ctrl Pts',(12.6520505140592,3.89157109446155,-0.581028658256058));
#80414=CARTESIAN_POINT('Ctrl Pts',(12.6579041257434,3.90530109716657,-0.465953152655482));
#80415=CARTESIAN_POINT('Ctrl Pts',(12.6637643918433,3.91904670820877,-0.350746828632537));
#80416=CARTESIAN_POINT('Ctrl Pts',(12.6696246579432,3.92768052343756,-0.235012433685925));
#80417=CARTESIAN_POINT('Ctrl Pts',(12.6754849240431,3.93119210792718,-0.119237622297209));
#80418=CARTESIAN_POINT('Ctrl Pts',(12.6813491372144,3.93470605757812,-0.00338483297355624));
#80419=CARTESIAN_POINT('Ctrl Pts',(12.6872133503857,3.93309091262892,0.112508014690212));
#80420=CARTESIAN_POINT('Ctrl Pts',(12.693077563557,3.92638829289976,0.227956077742426));
#80421=CARTESIAN_POINT('Ctrl Pts',(12.6989504121313,3.91967580316405,0.343574144939991));
#80422=CARTESIAN_POINT('Ctrl Pts',(12.7048232607056,3.90786092891218,0.458745710681152));
#80423=CARTESIAN_POINT('Ctrl Pts',(12.7106961092799,3.89103677214975,0.57299375020889));
#80424=CARTESIAN_POINT('Ctrl Pts',(12.7122908538927,3.88646825092499,0.604017271972283));
#80425=CARTESIAN_POINT('Ctrl Pts',(12.7138855985055,3.88153064800218,0.634972771725714));
#80426=CARTESIAN_POINT('Ctrl Pts',(12.7154803431183,3.87622646393288,0.665850884437639));
#80427=CARTESIAN_POINT('Ctrl Pts',(12.7213527892522,3.85669447430789,0.77955564453807));
#80428=CARTESIAN_POINT('Ctrl Pts',(12.7272252353861,3.83212243957652,0.892590619527022));
#80429=CARTESIAN_POINT('Ctrl Pts',(12.73309768152,3.80256764816943,1.00447413162073));
#80430=CARTESIAN_POINT('Ctrl Pts',(12.7389625204649,3.77305114215161,1.11621270938705));
#80431=CARTESIAN_POINT('Ctrl Pts',(12.7448273594097,3.73856482012168,1.22680239457453));
#80432=CARTESIAN_POINT('Ctrl Pts',(12.7506921983545,3.69921736591707,1.33576939615249));
#80433=CARTESIAN_POINT('Ctrl Pts',(12.7565510084746,3.6599103593549,1.44462438391895));
#80434=CARTESIAN_POINT('Ctrl Pts',(12.7624098185946,3.61575229957747,1.55185961947675));
#80435=CARTESIAN_POINT('Ctrl Pts',(12.7682686287146,3.56690211176297,1.65701488378979));
#80436=CARTESIAN_POINT('Ctrl Pts',(12.7743544175956,3.51615939715971,1.76624401482874));
#80437=CARTESIAN_POINT('Ctrl Pts',(12.7804402064765,3.46035375797207,1.87322831366523));
#80438=CARTESIAN_POINT('Ctrl Pts',(12.7865259953575,3.3997192012342,1.97747271858791));
#80439=CARTESIAN_POINT('Ctrl Pts',(12.7923780254358,3.3414136542045,2.07771303336549));
#80440=CARTESIAN_POINT('Ctrl Pts',(12.798230055514,3.27864353701332,2.17541966321022));
#80441=CARTESIAN_POINT('Ctrl Pts',(12.8040820855923,3.21166411568012,2.27017677903124));
#80442=CARTESIAN_POINT('Ctrl Pts',(12.8099332259708,3.14469487740713,2.36491948867501));
#80443=CARTESIAN_POINT('Ctrl Pts',(12.8157843663493,3.07351784595457,2.45671323845246));
#80444=CARTESIAN_POINT('Ctrl Pts',(12.8216355067278,2.99843128593945,2.54517166876804));
#80445=CARTESIAN_POINT('Ctrl Pts',(12.8274871742953,2.92333796060942,2.63363806920687));
#80446=CARTESIAN_POINT('Ctrl Pts',(12.8333388418628,2.84433467399043,2.71876823763874));
#80447=CARTESIAN_POINT('Ctrl Pts',(12.8391905094303,2.76175912345691,2.80020991070357));
#80448=CARTESIAN_POINT('Ctrl Pts',(12.8450441211145,2.67915613860523,2.88167864137512));
#80449=CARTESIAN_POINT('Ctrl Pts',(12.8508977327988,2.5929788240577,2.95945614986129));
#80450=CARTESIAN_POINT('Ctrl Pts',(12.856751344483,2.50360023599489,3.03322845468757));
#80451=CARTESIAN_POINT('Ctrl Pts',(12.8626116105829,2.41412004189673,3.10708462424671));
#80452=CARTESIAN_POINT('Ctrl Pts',(12.8684718766828,2.32143162949325,3.17692623895583));
#80453=CARTESIAN_POINT('Ctrl Pts',(12.8743321427826,2.22593957581017,3.24248084109098));
#80454=CARTESIAN_POINT('Ctrl Pts',(12.8801963559539,2.13038320526011,3.30807959628874));
#80455=CARTESIAN_POINT('Ctrl Pts',(12.8860605691252,2.03201978330911,3.36938537134209));
#80456=CARTESIAN_POINT('Ctrl Pts',(12.8919247822965,1.93127966843302,3.4261710176664));
#80457=CARTESIAN_POINT('Ctrl Pts',(12.8977976308708,1.83039120774077,3.48304028423534));
#80458=CARTESIAN_POINT('Ctrl Pts',(12.9036704794451,1.72711943650159,3.53537595155666));
#80459=CARTESIAN_POINT('Ctrl Pts',(12.9095433280194,1.62191597340105,3.5829984056969));
#80460=CARTESIAN_POINT('Ctrl Pts',(12.9111380726322,1.59334846414105,3.59593006079208));
#80461=CARTESIAN_POINT('Ctrl Pts',(12.912732817245,1.56463860934895,3.60851446087554));
#80462=CARTESIAN_POINT('Ctrl Pts',(12.9143275618578,1.53579563904659,3.62074864566507));
#80463=CARTESIAN_POINT('Ctrl Pts',(12.9202000079918,1.42958503448824,3.66579948991424));
#80464=CARTESIAN_POINT('Ctrl Pts',(12.9260724541257,1.32121265514115,3.70624844362442));
#80465=CARTESIAN_POINT('Ctrl Pts',(12.9319449002596,1.21111466909181,3.7418832502245));
#80466=CARTESIAN_POINT('Ctrl Pts',(12.9378097392044,1.10115930439256,3.7774718953605));
#80467=CARTESIAN_POINT('Ctrl Pts',(12.9436745781493,0.989483167967315,3.80825866898438));
#80468=CARTESIAN_POINT('Ctrl Pts',(12.9495394170941,0.87654358351824,3.83407881324745));
#80469=CARTESIAN_POINT('Ctrl Pts',(12.9553982272142,0.763720096540402,3.85987241541308));
#80470=CARTESIAN_POINT('Ctrl Pts',(12.9612570373342,0.649636145414761,3.88070945176689));
#80471=CARTESIAN_POINT('Ctrl Pts',(12.9671158474542,0.53476480296806,3.89647476644037));
#80472=CARTESIAN_POINT('Ctrl Pts',(12.9732016363352,0.41544317890391,3.91285085216074));
#80473=CARTESIAN_POINT('Ctrl Pts',(12.9792874252162,0.295272352536118,3.92375415683198));
#80474=CARTESIAN_POINT('Ctrl Pts',(12.9853732140971,0.174795304188719,3.92911384432082));
#80475=CARTESIAN_POINT('Ctrl Pts',(12.9912252441754,0.058945851560767,3.93426766299713));
#80476=CARTESIAN_POINT('Ctrl Pts',(12.9970772742537,-0.0571862815160144,
3.9342958560697));
#80477=CARTESIAN_POINT('Ctrl Pts',(13.0029293043319,-0.1731132709532,3.92918831254241));
#80478=CARTESIAN_POINT('Ctrl Pts',(13.0087804447104,-0.289022635700781,
3.9240815455286));
#80479=CARTESIAN_POINT('Ctrl Pts',(13.014631585089,-0.404726505978026,3.91384061258856));
#80480=CARTESIAN_POINT('Ctrl Pts',(13.0204827254675,-0.519738597916684,
3.89850750798759));
#80481=CARTESIAN_POINT('Ctrl Pts',(13.026334393035,-0.634761052469176,3.88317302187064));
#80482=CARTESIAN_POINT('Ctrl Pts',(13.0321860606025,-0.749091195021596,
3.86274550665698));
#80483=CARTESIAN_POINT('Ctrl Pts',(13.03803772817,-0.862250102067256,3.83731856398254));
#80484=CARTESIAN_POINT('Ctrl Pts',(13.0438913398542,-0.975446604229726,
3.81188317364008));
#80485=CARTESIAN_POINT('Ctrl Pts',(13.0497449515385,-1.08747069405064,3.7814451436646));
#80486=CARTESIAN_POINT('Ctrl Pts',(13.0555985632227,-1.19785653221811,3.74614851924245));
#80487=CARTESIAN_POINT('Ctrl Pts',(13.0614588293226,-1.30836785756999,3.71081176943746));
#80488=CARTESIAN_POINT('Ctrl Pts',(13.0673190954225,-1.41723682008301,3.67060552688228));
#80489=CARTESIAN_POINT('Ctrl Pts',(13.0731793615224,-1.52401546695074,3.62572280469632));
#80490=CARTESIAN_POINT('Ctrl Pts',(13.0790435746937,-1.63086603255683,3.58080985260158));
#80491=CARTESIAN_POINT('Ctrl Pts',(13.084907787865,-1.73562310643167,3.53121432552517));
#80492=CARTESIAN_POINT('Ctrl Pts',(13.0907720010363,-1.83786290992666,3.47717542328769));
#80493=CARTESIAN_POINT('Ctrl Pts',(13.0966448496106,-1.9402532676185,3.42305694554979));
#80494=CARTESIAN_POINT('Ctrl Pts',(13.1025176981849,-2.04011860162605,3.36448224220103));
#80495=CARTESIAN_POINT('Ctrl Pts',(13.1083905467592,-2.13706362425989,3.30173409981258));
#80496=CARTESIAN_POINT('Ctrl Pts',(13.109985291372,-2.16338859256551,3.28469513468848));
#80497=CARTESIAN_POINT('Ctrl Pts',(13.1115800359848,-2.18949841454651,3.26734866289345));
#80498=CARTESIAN_POINT('Ctrl Pts',(13.1131747805975,-2.2153856092198,3.24970084814923));
#80499=CARTESIAN_POINT('Ctrl Pts',(13.1190208234721,-2.31028334315751,3.18500717819714));
#80500=CARTESIAN_POINT('Ctrl Pts',(13.1248668663467,-2.40251085169915,3.1160400027466));
#80501=CARTESIAN_POINT('Ctrl Pts',(13.1307129092213,-2.4916558632707,3.04304782397989));
#80502=CARTESIAN_POINT('Ctrl Pts',(13.1365513636227,-2.58068515989634,2.9701503929267));
#80503=CARTESIAN_POINT('Ctrl Pts',(13.142389818024,-2.6666395950843,2.89323860850244));
#80504=CARTESIAN_POINT('Ctrl Pts',(13.1482282724254,-2.749135225128,2.81260457831534));
#80505=CARTESIAN_POINT('Ctrl Pts',(13.1540607468928,-2.83154636047867,2.73205313611047));
#80506=CARTESIAN_POINT('Ctrl Pts',(13.1598932213603,-2.9105054390927,2.64778731995767));
#80507=CARTESIAN_POINT('Ctrl Pts',(13.1657256958278,-2.98566159569659,2.56013941729401));
#80508=CARTESIAN_POINT('Ctrl Pts',(13.1715969784151,-3.06131782635182,2.47190832299632));
#80509=CARTESIAN_POINT('Ctrl Pts',(13.1774682610025,-3.13312000555237,2.38025023652073));
#80510=CARTESIAN_POINT('Ctrl Pts',(13.1833395435899,-3.20074780223883,2.28554205965747));
#80511=CARTESIAN_POINT('Ctrl Pts',(13.1891654831846,-3.26785332008022,2.1915652991593));
#80512=CARTESIAN_POINT('Ctrl Pts',(13.1949914227793,-3.33084846868497,2.09458574588242));
#80513=CARTESIAN_POINT('Ctrl Pts',(13.200817362374,-3.38946127116969,1.99500408301356));
#80514=CARTESIAN_POINT('Ctrl Pts',(13.2066424913309,-3.44806591810223,1.89543627622071));
#80515=CARTESIAN_POINT('Ctrl Pts',(13.2124676202878,-3.50228921951273,1.79326743942917));
#80516=CARTESIAN_POINT('Ctrl Pts',(13.2182927492447,-3.55190376447066,1.68892529377092));
#80517=CARTESIAN_POINT('Ctrl Pts',(13.2241185112485,-3.60152370129814,1.58457180871131));
#80518=CARTESIAN_POINT('Ctrl Pts',(13.2299442732523,-3.64653370711372,1.47804492253806));
#80519=CARTESIAN_POINT('Ctrl Pts',(13.2357700352561,-3.68675370574358,1.36979418643313));
#80520=CARTESIAN_POINT('Ctrl Pts',(13.2416755721452,-3.72752445563517,1.26006112234401));
#80521=CARTESIAN_POINT('Ctrl Pts',(13.2475811090342,-3.76337287285803,1.14855705555912));
#80522=CARTESIAN_POINT('Ctrl Pts',(13.2534866459232,-3.79416341890537,1.03576684183282));
#80523=CARTESIAN_POINT('Ctrl Pts',(13.2593211256594,-3.8245834840667,0.924333753058107));
#80524=CARTESIAN_POINT('Ctrl Pts',(13.2651556053955,-3.85006669718843,0.811645722880928));
#80525=CARTESIAN_POINT('Ctrl Pts',(13.2709900851316,-3.87053400840513,0.69818012702979));
#80526=CARTESIAN_POINT('Ctrl Pts',(13.2769311505971,-3.89137522156222,0.58264171340562));
#80527=CARTESIAN_POINT('Ctrl Pts',(13.2828722160626,-3.90701541620972,0.466297498712091));
#80528=CARTESIAN_POINT('Ctrl Pts',(13.2888132815281,-3.917426483295,0.349655184401622));
#80529=CARTESIAN_POINT('Ctrl Pts',(13.2947543469936,-3.92783755038029,0.233012870091152));
#80530=CARTESIAN_POINT('Ctrl Pts',(13.3006954124591,-3.9330195358347,0.116072908435258));
#80531=CARTESIAN_POINT('Ctrl Pts',(13.3066364779246,-3.93299994461018,-0.000660072963477499));
#80532=CARTESIAN_POINT('',(14.5566364620208,-3.93299834093028,0.00361251154098325));
#80533=CARTESIAN_POINT('Ctrl Pts',(13.3066364779651,-3.93299994461005,-0.0006600737587242));
#80534=CARTESIAN_POINT('Ctrl Pts',(13.3084316517558,-3.93299402484778,-0.0359325328708672));
#80535=CARTESIAN_POINT('Ctrl Pts',(13.3102268255465,-3.93251361331012,-0.0712005153535426));
#80536=CARTESIAN_POINT('Ctrl Pts',(13.3120219993372,-3.93155900442503,-0.106455599779701));
#80537=CARTESIAN_POINT('Ctrl Pts',(13.3178944454711,-3.92843624868645,-0.221783477956529));
#80538=CARTESIAN_POINT('Ctrl Pts',(13.3237668916051,-3.92022944147405,-0.337166920342933));
#80539=CARTESIAN_POINT('Ctrl Pts',(13.329639337739,-3.90692661815479,-0.45212100189397));
#80540=CARTESIAN_POINT('Ctrl Pts',(13.3355041766838,-3.89364102736347,-0.566926171490323));
#80541=CARTESIAN_POINT('Ctrl Pts',(13.3413690156287,-3.87527259537927,-0.681302679495434));
#80542=CARTESIAN_POINT('Ctrl Pts',(13.3472338545736,-3.851861352367,-0.794766080140218));
#80543=CARTESIAN_POINT('Ctrl Pts',(13.3530926646936,-3.82847417519594,-0.908112844851515));
#80544=CARTESIAN_POINT('Ctrl Pts',(13.3589514748136,-3.80005458091169,-1.02054796680724));
#80545=CARTESIAN_POINT('Ctrl Pts',(13.3648102849337,-3.76669426268574,-1.13159327121115));
#80546=CARTESIAN_POINT('Ctrl Pts',(13.3708960738146,-3.73204151757779,-1.24694063099592));
#80547=CARTESIAN_POINT('Ctrl Pts',(13.3769818626956,-3.69205753667132,-1.36078785684508));
#80548=CARTESIAN_POINT('Ctrl Pts',(13.3830676515766,-3.64690336095326,-1.47261158350319));
#80549=CARTESIAN_POINT('Ctrl Pts',(13.3889196816548,-3.60348358421941,-1.58014009372028));
#80550=CARTESIAN_POINT('Ctrl Pts',(13.3947717117331,-3.55528363581229,-1.68579726622336));
#80551=CARTESIAN_POINT('Ctrl Pts',(13.4006237418113,-3.50249689396205,-1.78913512843112));
#80552=CARTESIAN_POINT('Ctrl Pts',(13.4064748821899,-3.44971817742105,-1.89245727990787));
#80553=CARTESIAN_POINT('Ctrl Pts',(13.4123260225684,-3.39235424196728,-1.99346045418398));
#80554=CARTESIAN_POINT('Ctrl Pts',(13.4181771629469,-3.33064522641628,-2.09171971730211));
#80555=CARTESIAN_POINT('Ctrl Pts',(13.4240288305143,-3.26893065086997,-2.18998783360057));
#80556=CARTESIAN_POINT('Ctrl Pts',(13.4298804980818,-3.20287043682752,-2.28551119720595));
#80557=CARTESIAN_POINT('Ctrl Pts',(13.4357321656493,-3.13274861385817,-2.37789300061414));
#80558=CARTESIAN_POINT('Ctrl Pts',(13.4415857773335,-3.06260349410916,-2.47030549630081));
#80559=CARTESIAN_POINT('Ctrl Pts',(13.4474393890177,-2.98839433201654,-2.55957402732073));
#80560=CARTESIAN_POINT('Ctrl Pts',(13.453293000702,-2.91044561226842,-2.6453346363036));
#80561=CARTESIAN_POINT('Ctrl Pts',(13.4591532668018,-2.83240828001768,-2.73119273838465));
#80562=CARTESIAN_POINT('Ctrl Pts',(13.4650135329017,-2.75062318314964,-2.8135346527984));
#80563=CARTESIAN_POINT('Ctrl Pts',(13.4708737990016,-2.66545192487042,-2.89203302820085));
#80564=CARTESIAN_POINT('Ctrl Pts',(13.4767380121729,-2.58022330110081,-2.97058427469961));
#80565=CARTESIAN_POINT('Ctrl Pts',(13.4826022253441,-2.49160428989289,-3.04528656171485));
#80566=CARTESIAN_POINT('Ctrl Pts',(13.4884664385154,-2.39998847184148,-3.11585370886183));
#80567=CARTESIAN_POINT('Ctrl Pts',(13.4943392870897,-2.30823774404417,-3.18652477033379));
#80568=CARTESIAN_POINT('Ctrl Pts',(13.500212135664,-2.21348173901715,-3.2530483024118));
#80569=CARTESIAN_POINT('Ctrl Pts',(13.5060849842382,-2.11614185695144,-3.3151821429988));
#80570=CARTESIAN_POINT('Ctrl Pts',(13.5076797288511,-2.08970966640956,-3.3320542973372));
#80571=CARTESIAN_POINT('Ctrl Pts',(13.5092744734639,-2.06308707959257,-3.34860303622743));
#80572=CARTESIAN_POINT('Ctrl Pts',(13.5108692180768,-2.03628281023104,-3.36482411379221));
#80573=CARTESIAN_POINT('Ctrl Pts',(13.5167416642107,-1.93757946505785,-3.42455618842418));
#80574=CARTESIAN_POINT('Ctrl Pts',(13.5226141103446,-1.83608038008772,-3.48004155777348));
#80575=CARTESIAN_POINT('Ctrl Pts',(13.5284865564785,-1.73218700919155,-3.53100795314709));
#80576=CARTESIAN_POINT('Ctrl Pts',(13.5343513954233,-1.6284282221635,-3.58190832645814));
#80577=CARTESIAN_POINT('Ctrl Pts',(13.5402162343682,-1.52228168480992,-3.62830118673706));
#80578=CARTESIAN_POINT('Ctrl Pts',(13.546081073313,-1.41417656195017,-3.66995826292763));
#80579=CARTESIAN_POINT('Ctrl Pts',(13.551939883433,-1.3061825669243,-3.7115725172748));
#80580=CARTESIAN_POINT('Ctrl Pts',(13.5577986935531,-1.19623437444989,-3.74846052291427));
#80581=CARTESIAN_POINT('Ctrl Pts',(13.5636575036731,-1.08478380886473,-3.78044085895083));
#80582=CARTESIAN_POINT('Ctrl Pts',(13.569743292554,-0.969015487495461,-3.81366015936748));
#80583=CARTESIAN_POINT('Ctrl Pts',(13.575829081435,-0.851626438381354,-3.84158363892788));
#80584=CARTESIAN_POINT('Ctrl Pts',(13.581914870316,-0.733143997551199,-3.86406377779335));
#80585=CARTESIAN_POINT('Ctrl Pts',(13.5877669003943,-0.619212538368887,
-3.88568044103577));
#80586=CARTESIAN_POINT('Ctrl Pts',(13.5936189304725,-0.504270577384078,
-3.90226412979255));
#80587=CARTESIAN_POINT('Ctrl Pts',(13.5994709605508,-0.388799514714528,
-3.91373529219309));
#80588=CARTESIAN_POINT('Ctrl Pts',(13.6053221009293,-0.273346007418829,
-3.9252047106022));
#80589=CARTESIAN_POINT('Ctrl Pts',(13.6111732413078,-0.157363969600864,
-3.93156310727175));
#80590=CARTESIAN_POINT('Ctrl Pts',(13.6170243816864,-0.0413407050098623,
-3.93278272297228));
#80591=CARTESIAN_POINT('Ctrl Pts',(13.6228760492539,0.0746930133017308,
-3.93400244856045));
#80592=CARTESIAN_POINT('Ctrl Pts',(13.6287277168214,0.190767552411546,-3.93008246842282));
#80593=CARTESIAN_POINT('Ctrl Pts',(13.6345793843889,0.306395536613611,-3.92104715288445));
#80594=CARTESIAN_POINT('Ctrl Pts',(13.6404329960731,0.422061936241297,-3.9120088355166));
#80595=CARTESIAN_POINT('Ctrl Pts',(13.6462866077574,0.537281074073332,-3.89785183561486));
#80596=CARTESIAN_POINT('Ctrl Pts',(13.6521402194416,0.651571333732123,-3.87865231711461));
#80597=CARTESIAN_POINT('Ctrl Pts',(13.6580004855415,0.765991519141649,-3.8594309725037));
#80598=CARTESIAN_POINT('Ctrl Pts',(13.6638607516414,0.879480310844347,-3.83515573621396));
#80599=CARTESIAN_POINT('Ctrl Pts',(13.6697210177413,0.991566815415545,-3.80595378986223));
#80600=CARTESIAN_POINT('Ctrl Pts',(13.6755852309126,1.10372881373231,-3.77673217509175));
#80601=CARTESIAN_POINT('Ctrl Pts',(13.6814494440839,1.21448625022413,-3.74257736438277));
#80602=CARTESIAN_POINT('Ctrl Pts',(13.6873136572552,1.32338557434277,-3.70366570057578));
#80603=CARTESIAN_POINT('Ctrl Pts',(13.6931865058295,1.43244525919888,-3.66469673702744));
#80604=CARTESIAN_POINT('Ctrl Pts',(13.6990593544038,1.53964098952691,-3.62095709587331));
#80605=CARTESIAN_POINT('Ctrl Pts',(13.7049322029781,1.64454120101405,-3.57267032318506));
#80606=CARTESIAN_POINT('Ctrl Pts',(13.7065269475909,1.67302636371384,-3.55955827548971));
#80607=CARTESIAN_POINT('Ctrl Pts',(13.7081216922037,1.70134241567111,-3.54611119070619));
#80608=CARTESIAN_POINT('Ctrl Pts',(13.7097164368165,1.72948107361273,-3.53233410311303));
#80609=CARTESIAN_POINT('Ctrl Pts',(13.7155888829504,1.83309813663172,-3.48160171366076));
#80610=CARTESIAN_POINT('Ctrl Pts',(13.7214613290843,1.93465451844559,-3.42622128594048));
#80611=CARTESIAN_POINT('Ctrl Pts',(13.7273337752182,2.03370411398415,-3.36638330805687));
#80612=CARTESIAN_POINT('Ctrl Pts',(13.7331986141631,2.13262540029965,-3.30662284451758));
#80613=CARTESIAN_POINT('Ctrl Pts',(13.7390634531079,2.22904600752161,-3.2424165256699));
#80614=CARTESIAN_POINT('Ctrl Pts',(13.7449282920528,2.32254185819059,-3.1740019402881));
#80615=CARTESIAN_POINT('Ctrl Pts',(13.7507871021728,2.41594159878554,-3.10565768242157));
#80616=CARTESIAN_POINT('Ctrl Pts',(13.7566459122928,2.50642223140701,-3.03311400517208));
#80617=CARTESIAN_POINT('Ctrl Pts',(13.7625047224128,2.59358683713495,-2.95665289106454));
#80618=CARTESIAN_POINT('Ctrl Pts',(13.7685905112938,2.68412832550653,-2.8772295630287));
#80619=CARTESIAN_POINT('Ctrl Pts',(13.7746763001748,2.77109126625278,-2.79357935980456));
#80620=CARTESIAN_POINT('Ctrl Pts',(13.7807620890557,2.8540664283801,-2.70606611567302));
#80621=CARTESIAN_POINT('Ctrl Pts',(13.786614119134,2.93385446474073,-2.62191430776104));
#80622=CARTESIAN_POINT('Ctrl Pts',(13.7924661492123,3.00995510677078,-2.53419107588701));
#80623=CARTESIAN_POINT('Ctrl Pts',(13.7983181792905,3.08204113675473,-2.44325836361028));
#80624=CARTESIAN_POINT('Ctrl Pts',(13.804169319669,3.15411620730715,-2.3523394760765));
#80625=CARTESIAN_POINT('Ctrl Pts',(13.8100204600475,3.22217762267703,-2.25821240216862));
#80626=CARTESIAN_POINT('Ctrl Pts',(13.815871600426,3.28593854142631,-2.1612720564448));
#80627=CARTESIAN_POINT('Ctrl Pts',(13.8217232679935,3.34970520504785,-2.06432297637532));
#80628=CARTESIAN_POINT('Ctrl Pts',(13.827574935561,3.40917037462039,-1.96456046597406));
#80629=CARTESIAN_POINT('Ctrl Pts',(13.8334266031285,3.46409102164404,-1.8624076873137));
#80630=CARTESIAN_POINT('Ctrl Pts',(13.8392802148128,3.51902991511588,-1.76022097013505));
#80631=CARTESIAN_POINT('Ctrl Pts',(13.845133826497,3.56942108817908,-1.65564276950856));
#80632=CARTESIAN_POINT('Ctrl Pts',(13.8509874381812,3.61506819570829,-1.54911940804395));
#80633=CARTESIAN_POINT('Ctrl Pts',(13.8568477042811,3.66076719510241,-1.4424749502781));
#80634=CARTESIAN_POINT('Ctrl Pts',(13.862707970381,3.70171120165123,-1.33388129822243));
#80635=CARTESIAN_POINT('Ctrl Pts',(13.8685682364809,3.73775258476823,-1.22380334002585));
#80636=CARTESIAN_POINT('Ctrl Pts',(13.8744324496522,3.77381824287729,-1.11365124090209));
#80637=CARTESIAN_POINT('Ctrl Pts',(13.8802966628235,3.80497459162737,-1.00201324214997));
#80638=CARTESIAN_POINT('Ctrl Pts',(13.8861608759948,3.83112473276239,-0.889366224913153));
#80639=CARTESIAN_POINT('Ctrl Pts',(13.8920337245691,3.85731338153694,-0.776553328237669));
#80640=CARTESIAN_POINT('Ctrl Pts',(13.8979065731434,3.87848103448428,-0.662728852497358));
#80641=CARTESIAN_POINT('Ctrl Pts',(13.9037794217177,3.89458238930981,-0.548376707089073));
#80642=CARTESIAN_POINT('Ctrl Pts',(13.9053741663305,3.89895463704307,-0.517324915859616));
#80643=CARTESIAN_POINT('Ctrl Pts',(13.9069689109433,3.90295360868116,-0.486234224110163));
#80644=CARTESIAN_POINT('Ctrl Pts',(13.908563655556,3.90657906025345,-0.455114321889844));
#80645=CARTESIAN_POINT('Ctrl Pts',(13.91443610169,3.91992932894139,-0.340519202385656));
#80646=CARTESIAN_POINT('Ctrl Pts',(13.9203085478239,3.92825539497768,-0.225144304396692));
#80647=CARTESIAN_POINT('Ctrl Pts',(13.9261809939578,3.93147628507484,-0.109467894353272));
#80648=CARTESIAN_POINT('Ctrl Pts',(13.9320458329026,3.9346930028187,0.0060586680283022));
#80649=CARTESIAN_POINT('Ctrl Pts',(13.9379106718475,3.93281768465536,0.121885556352266));
#80650=CARTESIAN_POINT('Ctrl Pts',(13.9437755107923,3.92582088935509,0.237527566196477));
#80651=CARTESIAN_POINT('Ctrl Pts',(13.9496343209124,3.91883128648645,0.353050700582037));
#80652=CARTESIAN_POINT('Ctrl Pts',(13.9554931310324,3.90673070302807,0.468388924378064));
#80653=CARTESIAN_POINT('Ctrl Pts',(13.9613519411524,3.88954172706935,0.583055875012324));
#80654=CARTESIAN_POINT('Ctrl Pts',(13.9674377300334,3.87168682537056,0.70216518883016));
#80655=CARTESIAN_POINT('Ctrl Pts',(13.9735235189143,3.84834128124193,0.820549711180056));
#80656=CARTESIAN_POINT('Ctrl Pts',(13.9796093077953,3.81958987993541,0.937668464381209));
#80657=CARTESIAN_POINT('Ctrl Pts',(13.9854613378736,3.79194283720538,1.05028861599465));
#80658=CARTESIAN_POINT('Ctrl Pts',(13.9913133679519,3.7592976689318,1.16173800413208));
#80659=CARTESIAN_POINT('Ctrl Pts',(13.9971653980301,3.72178191529397,1.27154566374581));
#80660=CARTESIAN_POINT('Ctrl Pts',(14.0030165384086,3.6842718652763,1.38133662900793));
#80661=CARTESIAN_POINT('Ctrl Pts',(14.0088676787872,3.64189283582871,1.48948597097399));
#80662=CARTESIAN_POINT('Ctrl Pts',(14.0147188191657,3.59482193449524,1.59553886172413));
#80663=CARTESIAN_POINT('Ctrl Pts',(14.0205704867332,3.5477467920636,1.70160130786216));
#80664=CARTESIAN_POINT('Ctrl Pts',(14.0264221543007,3.49597910508139,1.80556654944974));
#80665=CARTESIAN_POINT('Ctrl Pts',(14.0322738218682,3.43974343325799,1.90700134068085));
#80666=CARTESIAN_POINT('Ctrl Pts',(14.0381274335524,3.38348907809181,2.00846983189121));
#80667=CARTESIAN_POINT('Ctrl Pts',(14.0439810452367,3.32276398674131,2.10740583974196));
#80668=CARTESIAN_POINT('Ctrl Pts',(14.0498346569209,3.25783744394467,2.20340286575833));
#80669=CARTESIAN_POINT('Ctrl Pts',(14.0556949230208,3.19283709232267,2.29950902168405));
#80670=CARTESIAN_POINT('Ctrl Pts',(14.0615551891207,3.12362598776988,2.39266918455233));
#80671=CARTESIAN_POINT('Ctrl Pts',(14.0674154552206,3.05051537297152,2.48250779641563));
#80672=CARTESIAN_POINT('Ctrl Pts',(14.0732796683919,2.97735551590106,2.57240691737713));
#80673=CARTESIAN_POINT('Ctrl Pts',(14.0791438815632,2.90029119297989,2.65897972468709));
#80674=CARTESIAN_POINT('Ctrl Pts',(14.0850080947345,2.81967116699783,2.74188685215147));
#80675=CARTESIAN_POINT('Ctrl Pts',(14.0908809433088,2.73893242322828,2.82491606529642));
#80676=CARTESIAN_POINT('Ctrl Pts',(14.0967537918831,2.65462782627727,2.9042685431518));
#80677=CARTESIAN_POINT('Ctrl Pts',(14.1026266404574,2.56713994962853,2.97964452225785));
#80678=CARTESIAN_POINT('Ctrl Pts',(14.1042213850702,2.54338302516427,3.00011251748914));
#80679=CARTESIAN_POINT('Ctrl Pts',(14.105816129683,2.51939154302913,3.02028754345122));
#80680=CARTESIAN_POINT('Ctrl Pts',(14.1074108742958,2.49517352266139,3.04016415540503));
#80681=CARTESIAN_POINT('Ctrl Pts',(14.1132833204297,2.4059937135938,3.11335727491005));
#80682=CARTESIAN_POINT('Ctrl Pts',(14.1191557665636,2.3134413100962,3.18274562456913));
#80683=CARTESIAN_POINT('Ctrl Pts',(14.1250282126975,2.21787485106744,3.24800248537506));
#80684=CARTESIAN_POINT('Ctrl Pts',(14.1308930516423,2.12243218919344,3.31317481219513));
#80685=CARTESIAN_POINT('Ctrl Pts',(14.1367578905872,2.02398357450615,3.37422606233112));
#80686=CARTESIAN_POINT('Ctrl Pts',(14.142622729532,1.92292124611626,3.43086911455897));
#80687=CARTESIAN_POINT('Ctrl Pts',(14.148481539652,1.82196280584332,3.48745393994674));
#80688=CARTESIAN_POINT('Ctrl Pts',(14.1543403497721,1.71839635446936,3.53963937985336));
#80689=CARTESIAN_POINT('Ctrl Pts',(14.1601991598921,1.61264323813689,3.58718145435819));
#80690=CARTESIAN_POINT('Ctrl Pts',(14.166284948773,1.50279309342829,3.63656537745399));
#80691=CARTESIAN_POINT('Ctrl Pts',(14.172370737654,1.3905838031818,3.68093862102548));
#80692=CARTESIAN_POINT('Ctrl Pts',(14.178456526535,1.2765162868987,3.72007999501118));
#80693=CARTESIAN_POINT('Ctrl Pts',(14.1843085566132,1.16683017236244,3.75771792533524));
#80694=CARTESIAN_POINT('Ctrl Pts',(14.1901605866915,1.05542637684033,3.79051834409894));
#80695=CARTESIAN_POINT('Ctrl Pts',(14.1960126167698,0.942770042609576,3.81833388361441));
#80696=CARTESIAN_POINT('Ctrl Pts',(14.2018637571483,0.830130835822037,3.84614519425917));
#80697=CARTESIAN_POINT('Ctrl Pts',(14.2077148975268,0.716239870152568,3.86897303347964));
#80698=CARTESIAN_POINT('Ctrl Pts',(14.2135660379053,0.601575514764253,3.88672045560729));
#80699=CARTESIAN_POINT('Ctrl Pts',(14.2194177054728,0.486900828093242,3.90446947678143));
#80700=CARTESIAN_POINT('Ctrl Pts',(14.2252693730403,0.371453021698423,3.91713710767553));
#80701=CARTESIAN_POINT('Ctrl Pts',(14.2311210406078,0.255717967548004,3.92467798947546));
#80702=CARTESIAN_POINT('Ctrl Pts',(14.236974652292,0.139944462400024,3.93222137660473));
#80703=CARTESIAN_POINT('Ctrl Pts',(14.2428282639762,0.0238839319974031,
3.93463460091986));
#80704=CARTESIAN_POINT('Ctrl Pts',(14.2486818756605,-0.0919760685040969,
3.93192438925554));
#80705=CARTESIAN_POINT('Ctrl Pts',(14.2545421417604,-0.207967779245849,
3.92921109660875));
#80706=CARTESIAN_POINT('Ctrl Pts',(14.2604024078602,-0.323758091591143,
3.9213627524506));
#80707=CARTESIAN_POINT('Ctrl Pts',(14.2662626739601,-0.438862790739952,
3.90843810887469));
#80708=CARTESIAN_POINT('Ctrl Pts',(14.2721268871314,-0.554045016482335,
3.89550476014949));
#80709=CARTESIAN_POINT('Ctrl Pts',(14.2779911003027,-0.668540302193927,
3.87748836809554));
#80710=CARTESIAN_POINT('Ctrl Pts',(14.283855313474,-0.781874590395646,3.85449881630461));
#80711=CARTESIAN_POINT('Ctrl Pts',(14.2897281620483,-0.89537577008339,3.83147541103013));
#80712=CARTESIAN_POINT('Ctrl Pts',(14.2956010106226,-1.00771214059734,3.80346432985501));
#80713=CARTESIAN_POINT('Ctrl Pts',(14.3014738591969,-1.11842467684313,3.77062531183202));
#80714=CARTESIAN_POINT('Ctrl Pts',(14.3030686038097,-1.14848814919649,3.76170802979764));
#80715=CARTESIAN_POINT('Ctrl Pts',(14.3046633484225,-1.17843200092335,3.75243502427599));
#80716=CARTESIAN_POINT('Ctrl Pts',(14.3062580930353,-1.20824731566829,3.74281009726387));
#80717=CARTESIAN_POINT('Ctrl Pts',(14.3121305391693,-1.31803845614238,3.70736751607094));
#80718=CARTESIAN_POINT('Ctrl Pts',(14.3180029853032,-1.42645258664682,3.66703060036621));
#80719=CARTESIAN_POINT('Ctrl Pts',(14.3238754314371,-1.53302100258657,3.62192429595491));
#80720=CARTESIAN_POINT('Ctrl Pts',(14.3297402703819,-1.63945136939473,3.57687642242201));
#80721=CARTESIAN_POINT('Ctrl Pts',(14.3356051093268,-1.74404039922512,3.52707160622746));
#80722=CARTESIAN_POINT('Ctrl Pts',(14.3414699482716,-1.84633447544124,3.47268455302193));
#80723=CARTESIAN_POINT('Ctrl Pts',(14.3473287583917,-1.94852339735197,3.41835340757776));
#80724=CARTESIAN_POINT('Ctrl Pts',(14.3531875685117,-2.04842169528549,3.35944958717139));
#80725=CARTESIAN_POINT('Ctrl Pts',(14.3590463786317,-2.14559630498422,3.29619560949256));
#80726=CARTESIAN_POINT('Ctrl Pts',(14.3651321675127,-2.24653559932926,3.23049108141458));
#80727=CARTESIAN_POINT('Ctrl Pts',(14.3712179563937,-2.34453547954069,3.16009269335622));
#80728=CARTESIAN_POINT('Ctrl Pts',(14.3773037452746,-2.43913902626371,3.08530222353618));
#80729=CARTESIAN_POINT('Ctrl Pts',(14.3831557753529,-2.53010879399015,3.01338450054002));
#80730=CARTESIAN_POINT('Ctrl Pts',(14.3890078054312,-2.61793797156652,2.93740615695396));
#80731=CARTESIAN_POINT('Ctrl Pts',(14.3948598355095,-2.70225108478815,2.85767879139018));
#80732=CARTESIAN_POINT('Ctrl Pts',(14.400710975888,-2.7865513796621,2.77796354699063));
#80733=CARTESIAN_POINT('Ctrl Pts',(14.4065621162665,-2.86733637279507,2.69450069783535));
#80734=CARTESIAN_POINT('Ctrl Pts',(14.412413256645,-2.94426585352191,2.60764023281297));
#80735=CARTESIAN_POINT('Ctrl Pts',(14.4182649242125,-3.02120226561124,2.52077194164431));
#80736=CARTESIAN_POINT('Ctrl Pts',(14.42411659178,-3.09428220065159,2.43050573551848));
#80737=CARTESIAN_POINT('Ctrl Pts',(14.4299682593475,-3.16320478645603,2.33722580829103));
#80738=CARTESIAN_POINT('Ctrl Pts',(14.4358218710318,-3.23215027061418,2.24391489039856));
#80739=CARTESIAN_POINT('Ctrl Pts',(14.441675482716,-3.29693541357618,2.14758859274089));
#80740=CARTESIAN_POINT('Ctrl Pts',(14.4475290944003,-3.35730224795042,2.04866068832958));
#80741=CARTESIAN_POINT('Ctrl Pts',(14.4533893605002,-3.41773770765006,1.94962032217166));
#80742=CARTESIAN_POINT('Ctrl Pts',(14.4592496266001,-3.47374461806866,1.8479727992091));
#80743=CARTESIAN_POINT('Ctrl Pts',(14.4651098927,-3.52511058209074,1.74415721310663));
#80744=CARTESIAN_POINT('Ctrl Pts',(14.4709741058713,-3.57651114268652,1.64027170397937));
#80745=CARTESIAN_POINT('Ctrl Pts',(14.4768383190426,-3.62326436641486,1.53421560135532));
#80746=CARTESIAN_POINT('Ctrl Pts',(14.4827025322139,-3.66520636059976,1.42644710179489));
#80747=CARTESIAN_POINT('Ctrl Pts',(14.4885753807881,-3.70721011686793,1.31851990670335));
#80748=CARTESIAN_POINT('Ctrl Pts',(14.4944482293624,-3.74438837146067,1.20887567204276));
#80749=CARTESIAN_POINT('Ctrl Pts',(14.5003210779367,-3.77662729872452,1.09798690635577));
#80750=CARTESIAN_POINT('Ctrl Pts',(14.5019158225495,-3.78538162891455,1.06787557972124));
#80751=CARTESIAN_POINT('Ctrl Pts',(14.5035105671623,-3.79377204123858,1.03767253569214));
#80752=CARTESIAN_POINT('Ctrl Pts',(14.505105311775,-3.80179691280552,1.00738733056476));
#80753=CARTESIAN_POINT('Ctrl Pts',(14.5126879630412,-3.83995336874241,0.863388004800826));
#80754=CARTESIAN_POINT('Ctrl Pts',(14.5202706143073,-3.869945230132,0.717141104295974));
#80755=CARTESIAN_POINT('Ctrl Pts',(14.5278532655734,-3.89155635414203,0.569454249731109));
#80756=CARTESIAN_POINT('Ctrl Pts',(14.5352847910977,-3.91273675846922,0.424710862388383));
#80757=CARTESIAN_POINT('Ctrl Pts',(14.5427163166219,-3.92586718729728,0.278584130433398));
#80758=CARTESIAN_POINT('Ctrl Pts',(14.5501478421462,-3.93078909684648,0.131856270661835));
#80759=CARTESIAN_POINT('Ctrl Pts',(14.5523107154377,-3.93222157079446,0.0891525528335636));
#80760=CARTESIAN_POINT('Ctrl Pts',(14.5544735887293,-3.93295904182085,0.0463980723529652));
#80761=CARTESIAN_POINT('Ctrl Pts',(14.5566364620208,-3.93299834093028,0.00361251154098325));
#80762=CARTESIAN_POINT('',(15.8066365080151,-3.93062432271256,-0.000977886178903984));
#80763=CARTESIAN_POINT('Ctrl Pts',(14.5566364779651,-3.93196599139969,0.00361124798914868));
#80764=CARTESIAN_POINT('Ctrl Pts',(14.605741828815,-3.9232411870099,-0.967535612376183));
#80765=CARTESIAN_POINT('Ctrl Pts',(14.7211295859113,-3.06929600653939,-3.26324377639959));
#80766=CARTESIAN_POINT('Ctrl Pts',(14.9027997492544,0.783357859407177,-4.58523082680123));
#80767=CARTESIAN_POINT('Ctrl Pts',(15.1016469679939,4.28070666041439,-1.82031364287207));
#80768=CARTESIAN_POINT('Ctrl Pts',(15.3004941867337,3.84588598521871,2.6167063762759));
#80769=CARTESIAN_POINT('Ctrl Pts',(15.4993414054732,-0.121686798380474,
4.65007350415478));
#80770=CARTESIAN_POINT('Ctrl Pts',(15.6680555025504,-3.39317719519555,2.75113718683392));
#80771=CARTESIAN_POINT('Ctrl Pts',(15.770487193381,-3.92513071241371,0.716349405360537));
#80772=CARTESIAN_POINT('Ctrl Pts',(15.8066364779651,-3.92671809469238,-0.000976317707402457));
#80773=CARTESIAN_POINT('',(17.0566364779651,-3.93351353754304,-0.00325536527871665));
#80774=CARTESIAN_POINT('Ctrl Pts',(15.8066365262899,-3.93299987819377,-0.000978840037985765));
#80775=CARTESIAN_POINT('Ctrl Pts',(15.8128950481088,-3.93296892038583,-0.125367964021516));
#80776=CARTESIAN_POINT('Ctrl Pts',(15.8191535699278,-3.92703264506812,-0.249598067531602));
#80777=CARTESIAN_POINT('Ctrl Pts',(15.8254120917467,-3.91526147166832,-0.37311741914522));
#80778=CARTESIAN_POINT('Ctrl Pts',(15.8316932505353,-3.90344772212963,-0.497083538204289));
#80779=CARTESIAN_POINT('Ctrl Pts',(15.8379744093238,-3.88575687475537,-0.620333443228178));
#80780=CARTESIAN_POINT('Ctrl Pts',(15.8442555681124,-3.86231098173614,-0.742322625520993));
#80781=CARTESIAN_POINT('Ctrl Pts',(15.8505482106162,-3.83882222306597,-0.864534838163019));
#80782=CARTESIAN_POINT('Ctrl Pts',(15.8568408531201,-3.80955748416183,-0.985481417500003));
#80783=CARTESIAN_POINT('Ctrl Pts',(15.8631334956239,-3.77468881186758,-1.10463268716877));
#80784=CARTESIAN_POINT('Ctrl Pts',(15.8694454887733,-3.7397129141401,-1.22415036156907));
#80785=CARTESIAN_POINT('Ctrl Pts',(15.8757574819227,-3.69909870924959,-1.34186137941075));
#80786=CARTESIAN_POINT('Ctrl Pts',(15.8820694750721,-3.65306737819782,-1.45725348870637));
#80787=CARTESIAN_POINT('Ctrl Pts',(15.8870582643656,-3.61668574626613,-1.5484555711205));
#80788=CARTESIAN_POINT('Ctrl Pts',(15.8920470536591,-3.57692111262724,-1.63820947314562));
#80789=CARTESIAN_POINT('Ctrl Pts',(15.8970358429526,-3.5339026077732,-1.72627383655484));
#80790=CARTESIAN_POINT('Ctrl Pts',(15.9029082890865,-3.48326429902636,-1.82993690990061));
#80791=CARTESIAN_POINT('Ctrl Pts',(15.9087807352204,-3.42797608331511,-1.93154352221046));
#80792=CARTESIAN_POINT('Ctrl Pts',(15.9146531813543,-3.36822804370767,-2.03064739567982));
#80793=CARTESIAN_POINT('Ctrl Pts',(15.9205180202992,-3.30855740193817,-2.12962288961424));
#80794=CARTESIAN_POINT('Ctrl Pts',(15.926382859244,-3.24443863666649,-2.22610174127127));
#80795=CARTESIAN_POINT('Ctrl Pts',(15.9322476981889,-3.17610895160689,-2.31965965769174));
#80796=CARTESIAN_POINT('Ctrl Pts',(15.9381065083089,-3.10784950678848,-2.41312140023685));
#80797=CARTESIAN_POINT('Ctrl Pts',(15.9439653184289,-3.03538799445726,-2.50366784809147));
#80798=CARTESIAN_POINT('Ctrl Pts',(15.9498241285489,-2.9590060367134,-2.59090182652559));
#80799=CARTESIAN_POINT('Ctrl Pts',(15.9559099174299,-2.87966493167289,-2.68151537520228));
#80800=CARTESIAN_POINT('Ctrl Pts',(15.9619957063108,-2.79609370471019,-2.76855421473168));
#80801=CARTESIAN_POINT('Ctrl Pts',(15.9680814951918,-2.70865581847126,-2.85160878401329));
#80802=CARTESIAN_POINT('Ctrl Pts',(15.9739335252701,-2.62457647390999,-2.9314731774518));
#80803=CARTESIAN_POINT('Ctrl Pts',(15.9797855553483,-2.53692235957565,-3.00765342008782));
#80804=CARTESIAN_POINT('Ctrl Pts',(15.9856375854266,-2.4460551218421,-3.07982196578147));
#80805=CARTESIAN_POINT('Ctrl Pts',(15.9914887258051,-2.35520169889724,-3.15197953949849));
#80806=CARTESIAN_POINT('Ctrl Pts',(15.9973398661836,-2.26113644744985,-3.22012637196162));
#80807=CARTESIAN_POINT('Ctrl Pts',(16.0031910065621,-2.16425402151115,-3.2839752633619));
#80808=CARTESIAN_POINT('Ctrl Pts',(16.0090426741296,-2.06736286644548,-3.34782990756073));
#80809=CARTESIAN_POINT('Ctrl Pts',(16.0148943416971,-1.96765437746729,-3.40738561341262));
#80810=CARTESIAN_POINT('Ctrl Pts',(16.0207460092646,-1.8655514958625,-3.46239896838669));
#80811=CARTESIAN_POINT('Ctrl Pts',(16.0265996209488,-1.76341469231684,-3.51743060060959));
#80812=CARTESIAN_POINT('Ctrl Pts',(16.0324532326331,-1.65888227805341,-3.56791668519934));
#80813=CARTESIAN_POINT('Ctrl Pts',(16.0383068443173,-1.55240039726309,-3.61366047195602));
#80814=CARTESIAN_POINT('Ctrl Pts',(16.0441671104172,-1.44579746732689,-3.6594562604831));
#80815=CARTESIAN_POINT('Ctrl Pts',(16.0500273765171,-1.33724102749432,-3.70049882753172));
#80816=CARTESIAN_POINT('Ctrl Pts',(16.055887642617,-1.2271958317091,-3.73664012056765));
#80817=CARTESIAN_POINT('Ctrl Pts',(16.0617518557883,-1.1170765170631,-3.77280575588811));
#80818=CARTESIAN_POINT('Ctrl Pts',(16.0676160689596,-1.00546684690839,-3.80406343271795));
#80819=CARTESIAN_POINT('Ctrl Pts',(16.0734802821309,-0.892843614231449,
-3.83031581994568));
#80820=CARTESIAN_POINT('Ctrl Pts',(16.0793531307052,-0.780054537140163,
-3.85660686537635));
#80821=CARTESIAN_POINT('Ctrl Pts',(16.0852259792795,-0.666249323523363,
-3.87787783532325));
#80822=CARTESIAN_POINT('Ctrl Pts',(16.0910988278538,-0.551911841454746,
-3.8940829882351));
#80823=CARTESIAN_POINT('Ctrl Pts',(16.0926935724666,-0.520864031986637,
-3.89848342185412));
#80824=CARTESIAN_POINT('Ctrl Pts',(16.0942883170793,-0.489776983168089,
-3.90251061484425));
#80825=CARTESIAN_POINT('Ctrl Pts',(16.0958830616921,-0.458660384822775,
-3.90616431443868));
#80826=CARTESIAN_POINT('Ctrl Pts',(16.1017555078261,-0.344077431422402,
-3.91961860290947));
#80827=CARTESIAN_POINT('Ctrl Pts',(16.10762795396,-0.228710139070021,-3.92804939865324));
#80828=CARTESIAN_POINT('Ctrl Pts',(16.1135004000939,-0.113036700494293,
-3.93137529426298));
#80829=CARTESIAN_POINT('Ctrl Pts',(16.1193652390387,0.00248689426889545,
-3.93469688149489));
#80830=CARTESIAN_POINT('Ctrl Pts',(16.1252300779836,0.11831543721581,-3.93292670754258));
#80831=CARTESIAN_POINT('Ctrl Pts',(16.1310949169284,0.233963750849901,-3.9260348907375));
#80832=CARTESIAN_POINT('Ctrl Pts',(16.1369537270484,0.349493182545274,-3.91915015845029));
#80833=CARTESIAN_POINT('Ctrl Pts',(16.1428125371685,0.464842343289673,-3.90715427982403));
#80834=CARTESIAN_POINT('Ctrl Pts',(16.1486713472885,0.579524850206603,-3.89006940143656));
#80835=CARTESIAN_POINT('Ctrl Pts',(16.1547571361695,0.698650322979956,-3.8723226301992));
#80836=CARTESIAN_POINT('Ctrl Pts',(16.1608429250504,0.817055988789581,-3.8490845608549));
#80837=CARTESIAN_POINT('Ctrl Pts',(16.1669287139314,0.934200793212602,-3.82043948754079));
#80838=CARTESIAN_POINT('Ctrl Pts',(16.1727807440097,1.04684599540481,-3.7928946886812));
#80839=CARTESIAN_POINT('Ctrl Pts',(16.1786327740879,1.15832497172005,-3.76035070356085));
#80840=CARTESIAN_POINT('Ctrl Pts',(16.1844848041662,1.26816664152833,-3.72293464478155));
#80841=CARTESIAN_POINT('Ctrl Pts',(16.1903359445447,1.37799161181431,-3.68552427446556));
#80842=CARTESIAN_POINT('Ctrl Pts',(16.1961870849232,1.48617937936311,-3.64324343651981));
#80843=CARTESIAN_POINT('Ctrl Pts',(16.2020382253018,1.59227495567051,-3.59626882553911));
#80844=CARTESIAN_POINT('Ctrl Pts',(16.2078898928693,1.69838009121176,-3.54928998213604));
#80845=CARTESIAN_POINT('Ctrl Pts',(16.2137415604367,1.80239228278799,-3.49761669234978));
#80846=CARTESIAN_POINT('Ctrl Pts',(16.2195932280042,1.90387808092456,-3.44147312251237));
#80847=CARTESIAN_POINT('Ctrl Pts',(16.2254468396885,2.00539759598659,-3.38531089993147));
#80848=CARTESIAN_POINT('Ctrl Pts',(16.2313004513727,2.10438868710423,-3.32467564411195));
#80849=CARTESIAN_POINT('Ctrl Pts',(16.237154063057,2.20044461152328,-3.25983627067651));
#80850=CARTESIAN_POINT('Ctrl Pts',(16.2430143291569,2.29660973280769,-3.19492318751027));
#80851=CARTESIAN_POINT('Ctrl Pts',(16.2488745952568,2.38983268461691,-3.12579667888275));
#80852=CARTESIAN_POINT('Ctrl Pts',(16.2547348613566,2.47973762662331,-3.05276764643308));
#80853=CARTESIAN_POINT('Ctrl Pts',(16.2605990745279,2.56970312240332,-2.97968942665957));
#80854=CARTESIAN_POINT('Ctrl Pts',(16.2664632876993,2.65634585023443,-2.90270372313745));
#80855=CARTESIAN_POINT('Ctrl Pts',(16.2723275008706,2.73932612746827,-2.82215899044857));
#80856=CARTESIAN_POINT('Ctrl Pts',(16.2782003494449,2.82242859810006,-2.74149565084606));
#80857=CARTESIAN_POINT('Ctrl Pts',(16.2840731980191,2.90185757190905,-2.65726312192466));
#80858=CARTESIAN_POINT('Ctrl Pts',(16.2899460465934,2.97731293827268,-2.5698437048961));
#80859=CARTESIAN_POINT('Ctrl Pts',(16.2915407912062,2.99780249074346,-2.54610537032173));
#80860=CARTESIAN_POINT('Ctrl Pts',(16.293135535819,3.01799928698865,-2.52213221222626));
#80861=CARTESIAN_POINT('Ctrl Pts',(16.2947302804318,3.03789787499169,-2.49793224510213));
#80862=CARTESIAN_POINT('Ctrl Pts',(16.3006027265658,3.11117191852845,-2.40881891483113));
#80863=CARTESIAN_POINT('Ctrl Pts',(16.3064751726997,3.18064425530551,-2.31632953768794));
#80864=CARTESIAN_POINT('Ctrl Pts',(16.3123476188336,3.2459878409817,-2.22082235584005));
#80865=CARTESIAN_POINT('Ctrl Pts',(16.3182124577784,3.3112467803283,-2.12543889435905));
#80866=CARTESIAN_POINT('Ctrl Pts',(16.3240772967233,3.37238737338344,-2.02704574033967));
#80867=CARTESIAN_POINT('Ctrl Pts',(16.3299421356681,3.42912214298098,-1.92603487209279));
#80868=CARTESIAN_POINT('Ctrl Pts',(16.3358009457881,3.48579859145661,-1.82512783906379));
#80869=CARTESIAN_POINT('Ctrl Pts',(16.3416597559082,3.53807802372136,-1.72160880240612));
#80870=CARTESIAN_POINT('Ctrl Pts',(16.3475185660282,3.58571607747243,-1.61589888661257));
#80871=CARTESIAN_POINT('Ctrl Pts',(16.3536043549092,3.63519969818896,-1.50609361609421));
#80872=CARTESIAN_POINT('Ctrl Pts',(16.3596901437901,3.67967478299223,-1.39392465249725));
#80873=CARTESIAN_POINT('Ctrl Pts',(16.3657759326711,3.71891968719538,-1.27989271432829));
#80874=CARTESIAN_POINT('Ctrl Pts',(16.3716279627494,3.75665717107912,-1.17024081132944));
#80875=CARTESIAN_POINT('Ctrl Pts',(16.3774799928276,3.78955870464399,-1.05886683673531));
#80876=CARTESIAN_POINT('Ctrl Pts',(16.3833320229059,3.8174764980236,-0.946235798856451));
#80877=CARTESIAN_POINT('Ctrl Pts',(16.3891831632844,3.84539004698656,-0.833621884574917));
#80878=CARTESIAN_POINT('Ctrl Pts',(16.3950343036629,3.86832126287971,-0.719751688113013));
#80879=CARTESIAN_POINT('Ctrl Pts',(16.4008854440414,3.88617276582833,-0.605103490432974));
#80880=CARTESIAN_POINT('Ctrl Pts',(16.4067371116089,3.90402587720114,-0.490444962926106));
#80881=CARTESIAN_POINT('Ctrl Pts',(16.4125887791764,3.91679830219751,-0.375008703312604));
#80882=CARTESIAN_POINT('Ctrl Pts',(16.4184404467439,3.92444424096509,-0.259280542185409));
#80883=CARTESIAN_POINT('Ctrl Pts',(16.4242940584281,3.9320927199654,-0.14351393235063));
#80884=CARTESIAN_POINT('Ctrl Pts',(16.4301476701124,3.93461129881638,-0.0274556404041727));
#80885=CARTESIAN_POINT('Ctrl Pts',(16.4360012817966,3.93200626176507,0.0884067725927054));
#80886=CARTESIAN_POINT('Ctrl Pts',(16.4418615478965,3.92939826329435,0.204400898572298));
#80887=CARTESIAN_POINT('Ctrl Pts',(16.4477218139964,3.92165503260585,0.320198287651489));
#80888=CARTESIAN_POINT('Ctrl Pts',(16.4535820800963,3.90883488221637,0.435314671896743));
#80889=CARTESIAN_POINT('Ctrl Pts',(16.4594462932676,3.89600609705702,0.550508590605755));
#80890=CARTESIAN_POINT('Ctrl Pts',(16.4653105064389,3.87809364708405,0.66502018376895));
#80891=CARTESIAN_POINT('Ctrl Pts',(16.4711747196102,3.8552069855118,0.778375294354234));
#80892=CARTESIAN_POINT('Ctrl Pts',(16.4770475681845,3.83228662196796,0.891897327087797));
#80893=CARTESIAN_POINT('Ctrl Pts',(16.4829204167588,3.80437752720706,1.00425907875835));
#80894=CARTESIAN_POINT('Ctrl Pts',(16.488793265333,3.77163902352979,1.11500137945533));
#80895=CARTESIAN_POINT('Ctrl Pts',(16.4903880099458,3.76274903569678,1.14507293420628));
#80896=CARTESIAN_POINT('Ctrl Pts',(16.4919827545586,3.75350321593581,1.17502519129287));
#80897=CARTESIAN_POINT('Ctrl Pts',(16.4935774991715,3.74390535814819,1.20484923091203));
#80898=CARTESIAN_POINT('Ctrl Pts',(16.4994499453054,3.70856245596412,1.31467249963693));
#80899=CARTESIAN_POINT('Ctrl Pts',(16.5053223914393,3.6683239712852,1.42312320185847));
#80900=CARTESIAN_POINT('Ctrl Pts',(16.5111948375732,3.62331442439222,1.52973251975346));
#80901=CARTESIAN_POINT('Ctrl Pts',(16.517059676518,3.57836318303758,1.63620373553232));
#80902=CARTESIAN_POINT('Ctrl Pts',(16.5229245154629,3.52865332948246,1.74083793327168));
#80903=CARTESIAN_POINT('Ctrl Pts',(16.5287893544077,3.47435915752887,1.84318133793051));
#80904=CARTESIAN_POINT('Ctrl Pts',(16.5346481645278,3.4201207978584,1.94541953757613));
#80905=CARTESIAN_POINT('Ctrl Pts',(16.5405069746478,3.36130768576459,2.04537126509643));
#80906=CARTESIAN_POINT('Ctrl Pts',(16.5463657847678,3.29814194572552,2.14260325441877));
#80907=CARTESIAN_POINT('Ctrl Pts',(16.5524515736488,3.23252907374073,2.24360215135699));
#80908=CARTESIAN_POINT('Ctrl Pts',(16.5585373625298,3.16221967541623,2.34166589628814));
#80909=CARTESIAN_POINT('Ctrl Pts',(16.5646231514107,3.0875151140716,2.43633729610237));
#80910=CARTESIAN_POINT('Ctrl Pts',(16.570475181489,3.01567999975477,2.52737231064207));
#80911=CARTESIAN_POINT('Ctrl Pts',(16.5763272115673,2.93978141560752,2.61527042240941));
#80912=CARTESIAN_POINT('Ctrl Pts',(16.5821792416455,2.86013061927182,2.69965587449656));
#80913=CARTESIAN_POINT('Ctrl Pts',(16.5880303820241,2.78049193245931,2.78402849723817));
#80914=CARTESIAN_POINT('Ctrl Pts',(16.5938815224026,2.69710245137203,2.86488922162652));
#80915=CARTESIAN_POINT('Ctrl Pts',(16.5997326627811,2.61031185592353,2.94189751942944));
#80916=CARTESIAN_POINT('Ctrl Pts',(16.6055843303486,2.52351344062408,3.01891275569622));
#80917=CARTESIAN_POINT('Ctrl Pts',(16.6114359979161,2.43331361099781,3.09207460100663));
#80918=CARTESIAN_POINT('Ctrl Pts',(16.6172876654836,2.34009628762112,3.16108183454049));
#80919=CARTESIAN_POINT('Ctrl Pts',(16.6231412771678,2.24684799437861,3.23011199455073));
#80920=CARTESIAN_POINT('Ctrl Pts',(16.6289948888521,2.15058054600681,3.2949845523311));
#80921=CARTESIAN_POINT('Ctrl Pts',(16.6348485005363,2.05170748117339,3.35544116498817));
#80922=CARTESIAN_POINT('Ctrl Pts',(16.6407087666362,1.95272201693505,3.41596650503118));
#80923=CARTESIAN_POINT('Ctrl Pts',(16.6465690327361,1.85112537689023,3.47206566429996));
#80924=CARTESIAN_POINT('Ctrl Pts',(16.652429298836,1.74735646171636,3.52352584717327));
#80925=CARTESIAN_POINT('Ctrl Pts',(16.6582935120073,1.64351765495195,3.57502069007963));
#80926=CARTESIAN_POINT('Ctrl Pts',(16.6641577251786,1.53750403690162,3.6218701684192));
#80927=CARTESIAN_POINT('Ctrl Pts',(16.6700219383499,1.42977365516118,3.66390997364933));
#80928=CARTESIAN_POINT('Ctrl Pts',(16.6758947869242,1.32188463402051,3.70601168499526));
#80929=CARTESIAN_POINT('Ctrl Pts',(16.6817676354985,1.21227419360324,3.74328945532005));
#80930=CARTESIAN_POINT('Ctrl Pts',(16.6876404840728,1.10141473893056,3.77562903009108));
#80931=CARTESIAN_POINT('Ctrl Pts',(16.6892352286856,1.07131137156472,3.78441069064193));
#80932=CARTESIAN_POINT('Ctrl Pts',(16.6908299732984,1.0411159564907,3.79282851673441));
#80933=CARTESIAN_POINT('Ctrl Pts',(16.6924247179112,1.01083804852762,3.80088087680328));
#80934=CARTESIAN_POINT('Ctrl Pts',(16.6982971640451,0.899343466802657,3.830532678337));
#80935=CARTESIAN_POINT('Ctrl Pts',(16.704169610179,0.786356408673737,3.85532411147381));
#80936=CARTESIAN_POINT('Ctrl Pts',(16.7100420563129,0.672338577263635,3.87510642918657));
#80937=CARTESIAN_POINT('Ctrl Pts',(16.7159068952577,0.558468444986268,3.89486312080969));
#80938=CARTESIAN_POINT('Ctrl Pts',(16.7217717342026,0.443570598317961,3.90962353096729));
#80939=CARTESIAN_POINT('Ctrl Pts',(16.7276365731474,0.32812099931161,3.91928891634832));
#80940=CARTESIAN_POINT('Ctrl Pts',(16.7334953832675,0.212790077973007,3.92894436609158));
#80941=CARTESIAN_POINT('Ctrl Pts',(16.7393541933875,0.0969089418910236,
3.93351517442654));
#80942=CARTESIAN_POINT('Ctrl Pts',(16.7452130035075,-0.0190378366721754,
3.93295392304243));
#80943=CARTESIAN_POINT('Ctrl Pts',(16.7512987923885,-0.139476560800132,
3.93237092796956));
#80944=CARTESIAN_POINT('Ctrl Pts',(16.7573845812695,-0.259985668775966,
3.92625010633041));
#80945=CARTESIAN_POINT('Ctrl Pts',(16.7634703701504,-0.380017615447589,
3.91459775864003));
#80946=CARTESIAN_POINT('Ctrl Pts',(16.7693224002287,-0.49543906302227,3.90339298461643));
#80947=CARTESIAN_POINT('Ctrl Pts',(16.775174430307,-0.610418879766082,3.88707382810077));
#80948=CARTESIAN_POINT('Ctrl Pts',(16.7810264603852,-0.72447267542454,3.86569894618854));
#80949=CARTESIAN_POINT('Ctrl Pts',(16.7868776007637,-0.838509131179923,
3.84432731395668));
#80950=CARTESIAN_POINT('Ctrl Pts',(16.7927287411422,-0.95161943960452,3.81790156074716));
#80951=CARTESIAN_POINT('Ctrl Pts',(16.7985798815207,-1.06332806980422,3.78653171331846));
#80952=CARTESIAN_POINT('Ctrl Pts',(16.8044315490882,-1.17504676497526,3.75515903945984));
#80953=CARTESIAN_POINT('Ctrl Pts',(16.8102832166557,-1.28536313287844,3.71884149760305));
#80954=CARTESIAN_POINT('Ctrl Pts',(16.8161348842232,-1.39381619408798,3.67773917197755));
#80955=CARTESIAN_POINT('Ctrl Pts',(16.8219884959075,-1.50230528697723,3.63662319080544));
#80956=CARTESIAN_POINT('Ctrl Pts',(16.8278421075917,-1.60892945590143,3.59071941132919));
#80957=CARTESIAN_POINT('Ctrl Pts',(16.833695719276,-1.71324777592382,3.54023601731468));
#80958=CARTESIAN_POINT('Ctrl Pts',(16.8395559853758,-1.81768468554497,3.48969523352012));
#80959=CARTESIAN_POINT('Ctrl Pts',(16.8454162514757,-1.9198101419382,3.4345646240956));
#80960=CARTESIAN_POINT('Ctrl Pts',(16.8512765175756,-2.01920782143974,3.37509833543211));
#80961=CARTESIAN_POINT('Ctrl Pts',(16.8571407307469,-2.11867244836869,3.3155919943744));
#80962=CARTESIAN_POINT('Ctrl Pts',(16.8630049439182,-2.21540529594528,3.25174438649032));
#80963=CARTESIAN_POINT('Ctrl Pts',(16.8688691570895,-2.30902047533366,3.18385198218917));
#80964=CARTESIAN_POINT('Ctrl Pts',(16.8747420056638,-2.40277350864656,3.11585960228109));
#80965=CARTESIAN_POINT('Ctrl Pts',(16.8806148542381,-2.49339938880002,3.04381079482913));
#80966=CARTESIAN_POINT('Ctrl Pts',(16.8864877028124,-2.58054656963073,2.96804117255254));
#80967=CARTESIAN_POINT('Ctrl Pts',(16.8880824474251,-2.60421097973624,2.94746628535595));
#80968=CARTESIAN_POINT('Ctrl Pts',(16.8896771920379,-2.62761910019042,2.9266172377897));
#80969=CARTESIAN_POINT('Ctrl Pts',(16.8912719366507,-2.65076439211749,2.90550118524877));
#80970=CARTESIAN_POINT('Ctrl Pts',(16.8970566991093,-2.73472141869071,2.82890500361985));
#80971=CARTESIAN_POINT('Ctrl Pts',(16.9028414615679,-2.8155164682209,2.74851984382134));
#80972=CARTESIAN_POINT('Ctrl Pts',(16.9086262240266,-2.89278011612591,2.66464110148938));
#80973=CARTESIAN_POINT('Ctrl Pts',(16.9144034208435,-2.96994271423334,2.58087206055212));
#80974=CARTESIAN_POINT('Ctrl Pts',(16.9201806176604,-3.04358280363557,2.49361882875862));
#80975=CARTESIAN_POINT('Ctrl Pts',(16.9259578144773,-3.11336480779858,2.40321629770633));
#80976=CARTESIAN_POINT('Ctrl Pts',(16.9317284140713,-3.18306712496895,2.3129170010898));
#80977=CARTESIAN_POINT('Ctrl Pts',(16.9374990136653,-3.24891986163083,2.21947589476493));
#80978=CARTESIAN_POINT('Ctrl Pts',(16.9432696132592,-3.31062573586229,2.12326311064981));
#80979=CARTESIAN_POINT('Ctrl Pts',(16.9490365710708,-3.37229266797669,2.02711104570523));
#80980=CARTESIAN_POINT('Ctrl Pts',(16.9548035288824,-3.4298177075269,1.92819113610653));
#80981=CARTESIAN_POINT('Ctrl Pts',(16.960570486694,-3.48294549312191,1.82690440142383));
#80982=CARTESIAN_POINT('Ctrl Pts',(16.9663352982464,-3.53605350642034,1.72565536210779));
#80983=CARTESIAN_POINT('Ctrl Pts',(16.9721001097988,-3.58476732048757,1.62204162590005));
#80984=CARTESIAN_POINT('Ctrl Pts',(16.9778649213511,-3.62887680623236,1.51649006761958));
#80985=CARTESIAN_POINT('Ctrl Pts',(16.9836290798747,-3.67298129532408,1.41095046605338));
#80986=CARTESIAN_POINT('Ctrl Pts',(16.9893932383983,-3.71248233006194,1.30347387312784));
#80987=CARTESIAN_POINT('Ctrl Pts',(16.9951573969219,-3.7472177048882,1.194507627507));
#80988=CARTESIAN_POINT('Ctrl Pts',(17.0009249127067,-3.78197331089375,1.08547791587602));
#80989=CARTESIAN_POINT('Ctrl Pts',(17.0066924284914,-3.81195758242033,0.974957225464982));
#80990=CARTESIAN_POINT('Ctrl Pts',(17.0124599442761,-3.83705813313859,0.863408294444193));
#80991=CARTESIAN_POINT('Ctrl Pts',(17.0182292829875,-3.86216661733521,0.751824106386962));
#80992=CARTESIAN_POINT('Ctrl Pts',(17.0239986216988,-3.88238822930771,0.639211450260981));
#80993=CARTESIAN_POINT('Ctrl Pts',(17.0297679604102,-3.89766198503899,0.526041871320081));
#80994=CARTESIAN_POINT('Ctrl Pts',(17.0355438875975,-3.91295318311102,0.412743054856122));
#80995=CARTESIAN_POINT('Ctrl Pts',(17.0413198147847,-3.92328520357892,0.298886470476205));
#80996=CARTESIAN_POINT('Ctrl Pts',(17.047095741972,-3.92864906866525,0.184947277016033));
#80997=CARTESIAN_POINT('Ctrl Pts',(17.050275987303,-3.9316024311894,0.122211966082349));
#80998=CARTESIAN_POINT('Ctrl Pts',(17.0534562326341,-3.93305054888195,0.0594516086523946));
#80999=CARTESIAN_POINT('Ctrl Pts',(17.0566364779651,-3.93299865311076,-0.00325493916173806));
#81000=CARTESIAN_POINT('',(18.3066364779651,-3.93441244414383,0.00256739835708875));
#81001=CARTESIAN_POINT('Ctrl Pts',(17.0566364779651,-3.93555909411355,-0.00325705817586157));
#81002=CARTESIAN_POINT('Ctrl Pts',(17.0677973704402,-3.93752172051231,-0.223467208643121));
#81003=CARTESIAN_POINT('Ctrl Pts',(17.1452406691619,-3.82037057107914,-1.74937440102309));
#81004=CARTESIAN_POINT('Ctrl Pts',(17.28896637413,-1.82419876275297,-4.2790524821404));
#81005=CARTESIAN_POINT('Ctrl Pts',(17.4878135928696,2.61321414266571,-3.84825975156499));
#81006=CARTESIAN_POINT('Ctrl Pts',(17.6866608116094,4.650182051095,0.117465580568825));
#81007=CARTESIAN_POINT('Ctrl Pts',(17.8855080303489,2.41558795570895,3.97528943589974));
#81008=CARTESIAN_POINT('Ctrl Pts',(18.0843552490887,-2.03791576839781,4.18149382300865));
#81009=CARTESIAN_POINT('Ctrl Pts',(18.224731398294,-3.86033642911773,1.61548625749645));
#81010=CARTESIAN_POINT('Ctrl Pts',(18.2988251412528,-3.93851969709005,0.156507900232432));
#81011=CARTESIAN_POINT('Ctrl Pts',(18.3066364779651,-3.93735639800032,0.00256931943232003));
#81012=CARTESIAN_POINT('',(19.5566364501327,-3.93099991098921,0.0019806725685321));
#81013=CARTESIAN_POINT('Ctrl Pts',(18.3066364779651,-3.9329991626239,0.00256647612112477));
#81014=CARTESIAN_POINT('Ctrl Pts',(18.3124243982231,-3.93307351157268,-0.111369652441173));
#81015=CARTESIAN_POINT('Ctrl Pts',(18.3182123184812,-3.9281927071081,-0.225501921867932));
#81016=CARTESIAN_POINT('Ctrl Pts',(18.3240002387392,-3.91833207797461,-0.339356341793069));
#81017=CARTESIAN_POINT('Ctrl Pts',(18.3297815910592,-3.90848263835275,-0.453081563536361));
#81018=CARTESIAN_POINT('Ctrl Pts',(18.3355629433793,-3.89366464276368,-0.566529141787071));
#81019=CARTESIAN_POINT('Ctrl Pts',(18.3413442956993,-3.87390544353728,-0.679224274104115));
#81020=CARTESIAN_POINT('Ctrl Pts',(18.3472070203188,-3.85386813438285,-0.793505585839553));
#81021=CARTESIAN_POINT('Ctrl Pts',(18.3530697449383,-3.8287494430815,-0.907012664087174));
#81022=CARTESIAN_POINT('Ctrl Pts',(18.3589324695578,-3.79863253644424,-1.01925455754055));
#81023=CARTESIAN_POINT('Ctrl Pts',(18.3647060952287,-3.76897333247794,-1.12979065115714));
#81024=CARTESIAN_POINT('Ctrl Pts',(18.3704797208996,-3.73446689042605,-1.23909932194822));
#81025=CARTESIAN_POINT('Ctrl Pts',(18.3762533465705,-3.69524406185396,-1.34672206610461));
#81026=CARTESIAN_POINT('Ctrl Pts',(18.3820257767339,-3.65602935490084,-1.4543225255112));
#81027=CARTESIAN_POINT('Ctrl Pts',(18.3877982068972,-3.61210034781823,-1.56023735225455));
#81028=CARTESIAN_POINT('Ctrl Pts',(18.3935706370606,-3.56363722976075,-1.66402484797046));
#81029=CARTESIAN_POINT('Ctrl Pts',(18.3993433590193,-3.51517166190038,-1.76781759012774));
#81030=CARTESIAN_POINT('Ctrl Pts',(18.4051160809781,-3.46217170848123,-1.86948240220678));
#81031=CARTESIAN_POINT('Ctrl Pts',(18.4108888029369,-3.40486463611714,-1.96859996183046));
#81032=CARTESIAN_POINT('Ctrl Pts',(18.4168188765728,-3.34599549926883,-2.07041924766809));
#81033=CARTESIAN_POINT('Ctrl Pts',(18.4227489502087,-3.28258128171833,-2.16954999672107));
#81034=CARTESIAN_POINT('Ctrl Pts',(18.4286790238446,-3.21491656800035,-2.26556846305665));
#81035=CARTESIAN_POINT('Ctrl Pts',(18.4344599653401,-3.14895351672432,-2.35917221411569));
#81036=CARTESIAN_POINT('Ctrl Pts',(18.4402409068357,-3.0789515343617,-2.44981806250247));
#81037=CARTESIAN_POINT('Ctrl Pts',(18.4460218483312,-3.00522427957689,-2.53714722265807));
#81038=CARTESIAN_POINT('Ctrl Pts',(18.4520264880373,-2.92864408898966,-2.62785565535448));
#81039=CARTESIAN_POINT('Ctrl Pts',(18.4580311277434,-2.84804485615273,-2.71498515999039));
#81040=CARTESIAN_POINT('Ctrl Pts',(18.4640357674495,-2.76381877789818,-2.79817704281509));
#81041=CARTESIAN_POINT('Ctrl Pts',(18.4700404071556,-2.67959269964363,-2.88136892563979));
#81042=CARTESIAN_POINT('Ctrl Pts',(18.4760450468618,-2.5917402031067,-2.96062290501553));
#81043=CARTESIAN_POINT('Ctrl Pts',(18.4820496865679,-2.50068890915906,-3.03562909124433));
#81044=CARTESIAN_POINT('Ctrl Pts',(18.4879221327018,-2.41164213111716,-3.10898399843243));
#81045=CARTESIAN_POINT('Ctrl Pts',(18.4937945788357,-2.31921585654286,-3.17854026507982));
#81046=CARTESIAN_POINT('Ctrl Pts',(18.4996670249696,-2.22376803057712,-3.24397052178086));
#81047=CARTESIAN_POINT('Ctrl Pts',(18.5055318639145,-2.12844384808832,-3.30931601987839));
#81048=CARTESIAN_POINT('Ctrl Pts',(18.5113967028593,-2.03010623581613,-3.37054590547077));
#81049=CARTESIAN_POINT('Ctrl Pts',(18.5172615418042,-1.92914691094862,-3.42737234568662));
#81050=CARTESIAN_POINT('Ctrl Pts',(18.5231203519242,-1.82829136831464,-3.48414037054661));
#81051=CARTESIAN_POINT('Ctrl Pts',(18.5289791620442,-1.72481983167672,-3.53651375208932));
#81052=CARTESIAN_POINT('Ctrl Pts',(18.5348379721642,-1.61915320353093,-3.58424774583113));
#81053=CARTESIAN_POINT('Ctrl Pts',(18.5409237610452,-1.50939289768618,-3.63383102339216));
#81054=CARTESIAN_POINT('Ctrl Pts',(18.5470095499262,-1.39726435316989,-3.67840791277819));
#81055=CARTESIAN_POINT('Ctrl Pts',(18.5530953388071,-1.28326808708139,-3.71775631485961));
#81056=CARTESIAN_POINT('Ctrl Pts',(18.5589473688854,-1.1736504859769,-3.75559332120603));
#81057=CARTESIAN_POINT('Ctrl Pts',(18.5647993989637,-1.06230642408677,-3.78859594246006));
#81058=CARTESIAN_POINT('Ctrl Pts',(18.5706514290419,-0.949700775371681,
-3.81661596669857));
#81059=CARTESIAN_POINT('Ctrl Pts',(18.5765025694205,-0.837112246394062,
-3.84463173097796));
#81060=CARTESIAN_POINT('Ctrl Pts',(18.582353709799,-0.723262912972853,-3.86766630464765));
#81061=CARTESIAN_POINT('Ctrl Pts',(18.5882048501775,-0.608630967475324,
-3.88562187370697));
#81062=CARTESIAN_POINT('Ctrl Pts',(18.594056517745,-0.493988693615218,-3.90357906056686));
#81063=CARTESIAN_POINT('Ctrl Pts',(18.5999081853125,-0.378564075906531,
-3.91645626914058));
#81064=CARTESIAN_POINT('Ctrl Pts',(18.60575985288,-0.262842903166594,-3.92420725857529));
#81065=CARTESIAN_POINT('Ctrl Pts',(18.6116134645642,-0.14708328404066,-3.93196082314403));
#81066=CARTESIAN_POINT('Ctrl Pts',(18.6174670762485,-0.0310273261863687,
-3.93458475445545));
#81067=CARTESIAN_POINT('Ctrl Pts',(18.6233206879327,0.0848374038312977,
-3.9320848941638));
#81068=CARTESIAN_POINT('Ctrl Pts',(18.6291809540326,0.200833849465549,-3.92958219201821));
#81069=CARTESIAN_POINT('Ctrl Pts',(18.6350412201325,0.316638219857573,-3.92194408118004));
#81070=CARTESIAN_POINT('Ctrl Pts',(18.6409014862324,0.431766194339378,-3.90922843454123));
#81071=CARTESIAN_POINT('Ctrl Pts',(18.6467656994037,0.546971711091178,-3.8965042235191));
#81072=CARTESIAN_POINT('Ctrl Pts',(18.652629912575,0.66149951734439,-3.87869573038758));
#81073=CARTESIAN_POINT('Ctrl Pts',(18.6584941257463,0.774875356904638,-3.85591197789341));
#81074=CARTESIAN_POINT('Ctrl Pts',(18.6643669743206,0.888418149137797,-3.83309467496741));
#81075=CARTESIAN_POINT('Ctrl Pts',(18.6702398228949,1.00080518937484,-3.80528758961883));
#81076=CARTESIAN_POINT('Ctrl Pts',(18.6761126714692,1.11157716326739,-3.77264962726496));
#81077=CARTESIAN_POINT('Ctrl Pts',(18.677707416082,1.1416567756359,-3.76378694095899));
#81078=CARTESIAN_POINT('Ctrl Pts',(18.6793021606948,1.17161741340048,-3.7545683145776));
#81079=CARTESIAN_POINT('Ctrl Pts',(18.6808969053076,1.2014501533178,-3.74499753392344));
#81080=CARTESIAN_POINT('Ctrl Pts',(18.6867693514415,1.31130545979526,-3.70975433987203));
#81081=CARTESIAN_POINT('Ctrl Pts',(18.6926417975754,1.41979264436669,-3.66961431937687));
#81082=CARTESIAN_POINT('Ctrl Pts',(18.6985142437093,1.52644277636708,-3.62470156709166));
#81083=CARTESIAN_POINT('Ctrl Pts',(18.7043790826541,1.63295475338068,-3.57984699495666));
#81084=CARTESIAN_POINT('Ctrl Pts',(18.710243921599,1.73763403280681,-3.53023214500362));
#81085=CARTESIAN_POINT('Ctrl Pts',(18.7161087605438,1.84002668157384,-3.47603089904223));
#81086=CARTESIAN_POINT('Ctrl Pts',(18.7219675706639,1.94231407470667,-3.42188536983969));
#81087=CARTESIAN_POINT('Ctrl Pts',(18.7278263807839,2.04231914945018,-3.3631630145224));
#81088=CARTESIAN_POINT('Ctrl Pts',(18.7336851909039,2.13960843827371,-3.30008556417374));
#81089=CARTESIAN_POINT('Ctrl Pts',(18.7397709797849,2.24066685457846,-3.23456440234945));
#81090=CARTESIAN_POINT('Ctrl Pts',(18.7458567686658,2.33879438342135,-3.16434405169622));
#81091=CARTESIAN_POINT('Ctrl Pts',(18.7519425575468,2.43353355831423,-3.08972546038616));
#81092=CARTESIAN_POINT('Ctrl Pts',(18.7577945876251,2.52463374465121,-3.01797301394323));
#81093=CARTESIAN_POINT('Ctrl Pts',(18.7636466177034,2.61260071817849,-2.94215425177779));
#81094=CARTESIAN_POINT('Ctrl Pts',(18.7694986477816,2.69705843959465,-2.86258009030512));
#81095=CARTESIAN_POINT('Ctrl Pts',(18.7753497881601,2.78150332067783,-2.78301802670477));
#81096=CARTESIAN_POINT('Ctrl Pts',(18.7812009285386,2.8624397096894,-2.6997019824014));
#81097=CARTESIAN_POINT('Ctrl Pts',(18.7870520689171,2.93952676111078,-2.61298132804533));
#81098=CARTESIAN_POINT('Ctrl Pts',(18.7929037364846,3.01662075809179,-2.52625286013998));
#81099=CARTESIAN_POINT('Ctrl Pts',(18.7987554040521,3.08986445338437,-2.43611948134101));
#81100=CARTESIAN_POINT('Ctrl Pts',(18.8046070716196,3.15895627778329,-2.34296483862936));
#81101=CARTESIAN_POINT('Ctrl Pts',(18.8104606833039,3.22807105676253,-2.2497792468764));
#81102=CARTESIAN_POINT('Ctrl Pts',(18.8163142949881,3.29303097590415,-2.15357072711794));
#81103=CARTESIAN_POINT('Ctrl Pts',(18.8221679066724,3.35357731702582,-2.05475258333696));
#81104=CARTESIAN_POINT('Ctrl Pts',(18.8280281727722,3.41419248753713,-1.95582210258571));
#81105=CARTESIAN_POINT('Ctrl Pts',(18.8338884388721,3.47038384942836,-1.85427642917784));
#81106=CARTESIAN_POINT('Ctrl Pts',(18.839748704972,3.52193820874784,-1.7505542704418));
#81107=CARTESIAN_POINT('Ctrl Pts',(18.8456129181433,3.57352729153124,-1.64676225160697));
#81108=CARTESIAN_POINT('Ctrl Pts',(18.8514771313146,3.62047298587642,-1.5407912054892));
#81109=CARTESIAN_POINT('Ctrl Pts',(18.8573413444859,3.66261056750948,-1.43309903034226));
#81110=CARTESIAN_POINT('Ctrl Pts',(18.8632141930602,3.70481019923985,-1.32524827205673));
#81111=CARTESIAN_POINT('Ctrl Pts',(18.8690870416345,3.74218745457847,-1.21567171620558));
#81112=CARTESIAN_POINT('Ctrl Pts',(18.8749598902088,3.77462765020768,-1.10484166389924));
#81113=CARTESIAN_POINT('Ctrl Pts',(18.8765546348216,3.78343663388278,-1.07474628060885));
#81114=CARTESIAN_POINT('Ctrl Pts',(18.8781493794344,3.79188186680698,-1.0445585193725));
#81115=CARTESIAN_POINT('Ctrl Pts',(18.8797441240472,3.7999617087422,-1.01428793352432));
#81116=CARTESIAN_POINT('Ctrl Pts',(18.8856165701811,3.82971470878677,-0.902820314564572));
#81117=CARTESIAN_POINT('Ctrl Pts',(18.891489016315,3.85460869725281,-0.789855807750062));
#81118=CARTESIAN_POINT('Ctrl Pts',(18.8973614624489,3.87449450805717,-0.675855980986188));
#81119=CARTESIAN_POINT('Ctrl Pts',(18.9032263013937,3.89435455870654,-0.562003830031724));
#81120=CARTESIAN_POINT('Ctrl Pts',(18.9090911403386,3.90921926287072,-0.447119429667083));
#81121=CARTESIAN_POINT('Ctrl Pts',(18.9149559792834,3.91898944521827,-0.331678652113463));
#81122=CARTESIAN_POINT('Ctrl Pts',(18.9208147894035,3.92874958420086,-0.216356543159836));
#81123=CARTESIAN_POINT('Ctrl Pts',(18.9266735995235,3.93342558333507,-0.100479604036908));
#81124=CARTESIAN_POINT('Ctrl Pts',(18.9325324096435,3.9329695844526,0.0154676362374262));
#81125=CARTESIAN_POINT('Ctrl Pts',(18.9386181985245,3.93249591951521,0.135906839964299));
#81126=CARTESIAN_POINT('Ctrl Pts',(18.9447039874054,3.92648449418511,0.256421454547686));
#81127=CARTESIAN_POINT('Ctrl Pts',(18.9507897762864,3.91494111193318,0.37646392934171));
#81128=CARTESIAN_POINT('Ctrl Pts',(18.9566418063647,3.90384111792017,0.491895500647184));
#81129=CARTESIAN_POINT('Ctrl Pts',(18.9624938364429,3.8876263426259,0.606890083954243));
#81130=CARTESIAN_POINT('Ctrl Pts',(18.9683458665212,3.86635500340985,0.720963235961203));
#81131=CARTESIAN_POINT('Ctrl Pts',(18.9741970068997,3.84508689813226,0.835019045122419));
#81132=CARTESIAN_POINT('Ctrl Pts',(18.9800481472782,3.81876383323651,0.948153295281717));
#81133=CARTESIAN_POINT('Ctrl Pts',(18.9858992876567,3.78749540376611,1.05989035586263));
#81134=CARTESIAN_POINT('Ctrl Pts',(18.9917509552242,3.75622415700368,1.17163748397603));
#81135=CARTESIAN_POINT('Ctrl Pts',(18.9976026227917,3.72000677129877,1.28198677417077));
#81136=CARTESIAN_POINT('Ctrl Pts',(19.0034542903592,3.67900291235452,1.39047710189235));
#81137=CARTESIAN_POINT('Ctrl Pts',(19.0093079020435,3.63798543057736,1.4990034736753));
#81138=CARTESIAN_POINT('Ctrl Pts',(19.0151615137277,3.59217845955852,1.60566926845081));
#81139=CARTESIAN_POINT('Ctrl Pts',(19.021015125412,3.54178978272248,1.71003337248215));
#81140=CARTESIAN_POINT('Ctrl Pts',(19.0268753915119,3.4913438237814,1.81451611815967));
#81141=CARTESIAN_POINT('Ctrl Pts',(19.0327356576117,3.43630594284824,1.91669157803847));
#81142=CARTESIAN_POINT('Ctrl Pts',(19.0385959237116,3.37692990828578,2.01614319792147));
#81143=CARTESIAN_POINT('Ctrl Pts',(19.0444601368829,3.31751388211816,2.1156618015622));
#81144=CARTESIAN_POINT('Ctrl Pts',(19.0503243500542,3.25375411110288,2.21245256782033));
#81145=CARTESIAN_POINT('Ctrl Pts',(19.0561885632255,3.18594671523122,2.30612933889395));
#81146=CARTESIAN_POINT('Ctrl Pts',(19.0620614117998,3.11803946893254,2.39994405458956));
#81147=CARTESIAN_POINT('Ctrl Pts',(19.0679342603741,3.04607295804537,2.49063530069165));
#81148=CARTESIAN_POINT('Ctrl Pts',(19.0738071089484,2.97038247602983,2.5778512265247));
#81149=CARTESIAN_POINT('Ctrl Pts',(19.0754018535612,2.94982907900116,2.60153430401523));
#81150=CARTESIAN_POINT('Ctrl Pts',(19.076996598174,2.92900128906535,2.62496134083283));
#81151=CARTESIAN_POINT('Ctrl Pts',(19.0785913427869,2.90790625567867,2.64812579160901));
#81152=CARTESIAN_POINT('Ctrl Pts',(19.0844637889208,2.83022645274341,2.73342596337996));
#81153=CARTESIAN_POINT('Ctrl Pts',(19.0903362350547,2.74866013708834,2.81544807388718));
#81154=CARTESIAN_POINT('Ctrl Pts',(19.0962086811886,2.66351492812146,2.89381706879929));
#81155=CARTESIAN_POINT('Ctrl Pts',(19.1020735201335,2.57848001658223,2.97208454421722));
#81156=CARTESIAN_POINT('Ctrl Pts',(19.1079383590783,2.48987573264462,3.0467080374681));
#81157=CARTESIAN_POINT('Ctrl Pts',(19.1138031980232,2.39804875914592,3.11734681239651));
#81158=CARTESIAN_POINT('Ctrl Pts',(19.1196620081432,2.30631618018096,3.1879129734298));
#81159=CARTESIAN_POINT('Ctrl Pts',(19.1255208182632,2.21136782665817,3.25450231305547));
#81160=CARTESIAN_POINT('Ctrl Pts',(19.1313796283832,2.11358541130495,3.31681258275455));
#81161=CARTESIAN_POINT('Ctrl Pts',(19.1374654172642,2.01201476403699,3.38153684224348));
#81162=CARTESIAN_POINT('Ctrl Pts',(19.1435512061452,1.90738635673773,3.44164346374798));
#81163=CARTESIAN_POINT('Ctrl Pts',(19.1496369950261,1.80016393188753,3.49684126295879));
#81164=CARTESIAN_POINT('Ctrl Pts',(19.1554890251044,1.69705998471473,3.54991888158042));
#81165=CARTESIAN_POINT('Ctrl Pts',(19.1613410551827,1.59155802113151,3.59845761670925));
#81166=CARTESIAN_POINT('Ctrl Pts',(19.1671930852609,1.48409703788399,3.64224449785348));
#81167=CARTESIAN_POINT('Ctrl Pts',(19.1730442256394,1.37665239221657,3.68602472196131));
#81168=CARTESIAN_POINT('Ctrl Pts',(19.178895366018,1.26724970177216,3.72505437258937));
#81169=CARTESIAN_POINT('Ctrl Pts',(19.1847465063965,1.15634833039371,3.75916846374244));
#81170=CARTESIAN_POINT('Ctrl Pts',(19.1905981739639,1.04543696677868,3.7932856285822));
#81171=CARTESIAN_POINT('Ctrl Pts',(19.1964498415314,0.933027048910614,3.82248623197764));
#81172=CARTESIAN_POINT('Ctrl Pts',(19.2023015090989,0.819592811755834,3.84665525137335));
#81173=CARTESIAN_POINT('Ctrl Pts',(19.2081551207831,0.706120888010383,3.87083230051355));
#81174=CARTESIAN_POINT('Ctrl Pts',(19.2140087324674,0.591624372355505,3.88997435557079));
#81175=CARTESIAN_POINT('Ctrl Pts',(19.2198623441516,0.476586684223825,3.90401769109984));
#81176=CARTESIAN_POINT('Ctrl Pts',(19.2257226102515,0.361418220660793,3.91807699116444));
#81177=CARTESIAN_POINT('Ctrl Pts',(19.2315828763514,0.245707767240356,3.92702595246014));
#81178=CARTESIAN_POINT('Ctrl Pts',(19.2374431424512,0.129942948218467,3.93085281207632));
#81179=CARTESIAN_POINT('Ctrl Pts',(19.2433073556225,0.0141001579920049,
3.93468224920142));
#81180=CARTESIAN_POINT('Ctrl Pts',(19.2491715687938,-0.101796658427518,
3.93338271983628));
#81181=CARTESIAN_POINT('Ctrl Pts',(19.2550357819651,-0.217262546543552,
3.92699452327978));
#81182=CARTESIAN_POINT('Ctrl Pts',(19.2609086305394,-0.332898465053581,
3.92059691972356));
#81183=CARTESIAN_POINT('Ctrl Pts',(19.2667814791137,-0.448101779025144,
3.9090957346196));
#81184=CARTESIAN_POINT('Ctrl Pts',(19.272654327688,-0.562395211926534,3.89258277055249));
#81185=CARTESIAN_POINT('Ctrl Pts',(19.2742490723008,-0.59343106004965,3.88809875225118));
#81186=CARTESIAN_POINT('Ctrl Pts',(19.2758438169136,-0.624399891530775,
3.8832454683769));
#81187=CARTESIAN_POINT('Ctrl Pts',(19.2774385615265,-0.655292334563368,
3.87802539396824));
#81188=CARTESIAN_POINT('Ctrl Pts',(19.2833110076604,-0.769049864260871,
3.85880312757318));
#81189=CARTESIAN_POINT('Ctrl Pts',(19.2891834537943,-0.882151336824631,
3.83453901074328));
#81190=CARTESIAN_POINT('Ctrl Pts',(19.2950558999282,-0.994114920244128,
3.80528901994947));
#81191=CARTESIAN_POINT('Ctrl Pts',(19.3009207388731,-1.10593346561165,3.77607691970503));
#81192=CARTESIAN_POINT('Ctrl Pts',(19.3067855778179,-1.21661665690062,3.741891893112));
#81193=CARTESIAN_POINT('Ctrl Pts',(19.3126504167628,-1.32569040885986,3.70284133333538));
#81194=CARTESIAN_POINT('Ctrl Pts',(19.3185092268828,-1.43465203727234,3.66383091600539));
#81195=CARTESIAN_POINT('Ctrl Pts',(19.3243680370029,-1.54200713029718,3.61996505239691));
#81196=CARTESIAN_POINT('Ctrl Pts',(19.3302268471229,-1.64729503780582,3.57140141378987));
#81197=CARTESIAN_POINT('Ctrl Pts',(19.3363126360039,-1.75666195082899,3.52095634972411));
#81198=CARTESIAN_POINT('Ctrl Pts',(19.3423984248848,-1.86379782777535,3.46544226652362));
#81199=CARTESIAN_POINT('Ctrl Pts',(19.3484842137658,-1.96820697150083,3.40509182215921));
#81200=CARTESIAN_POINT('Ctrl Pts',(19.3543362438441,-2.06860569736493,3.34705947457623));
#81201=CARTESIAN_POINT('Ctrl Pts',(19.3601882739223,-2.16648290600157,3.28455567343344));
#81202=CARTESIAN_POINT('Ctrl Pts',(19.3660403040006,-2.26142207469899,3.21783455138143));
#81203=CARTESIAN_POINT('Ctrl Pts',(19.3718914443791,-2.35634680954133,3.15112357311959));
#81204=CARTESIAN_POINT('Ctrl Pts',(19.3777425847576,-2.44833405448497,3.08019678641447));
#81205=CARTESIAN_POINT('Ctrl Pts',(19.3835937251362,-2.53699663910662,3.00535140260864));
#81206=CARTESIAN_POINT('Ctrl Pts',(19.3894453927037,-2.62566721224589,2.9304992752179));
#81207=CARTESIAN_POINT('Ctrl Pts',(19.3952970602712,-2.71101221369989,2.85172811551655));
#81208=CARTESIAN_POINT('Ctrl Pts',(19.4011487278387,-2.79267846176761,2.7693746603122));
#81209=CARTESIAN_POINT('Ctrl Pts',(19.4070023395229,-2.87437184205344,2.68699384457688));
#81210=CARTESIAN_POINT('Ctrl Pts',(19.4128559512072,-2.95238374777046,2.60102866013899));
#81211=CARTESIAN_POINT('Ctrl Pts',(19.4187095628915,-3.02639918266904,2.51185130673378));
#81212=CARTESIAN_POINT('Ctrl Pts',(19.4245698289913,-3.10049875869173,2.42257257605811));
#81213=CARTESIAN_POINT('Ctrl Pts',(19.4304300950912,-3.17059253165322,2.33007470618488));
#81214=CARTESIAN_POINT('Ctrl Pts',(19.4362903611911,-3.23640694306014,2.23476153065873));
#81215=CARTESIAN_POINT('Ctrl Pts',(19.4421545743625,-3.30226568251972,2.13938415874498));
#81216=CARTESIAN_POINT('Ctrl Pts',(19.4480187875338,-3.36383910216311,2.04118805481818));
#81217=CARTESIAN_POINT('Ctrl Pts',(19.4538830007052,-3.42089888225791,1.94060295716732));
#81218=CARTESIAN_POINT('Ctrl Pts',(19.4597558492795,-3.47804268627537,1.83986974197289));
#81219=CARTESIAN_POINT('Ctrl Pts',(19.4656286978538,-3.53065939829735,1.73674087877304));
#81220=CARTESIAN_POINT('Ctrl Pts',(19.4715015464281,-3.57856817516872,1.63166749543821));
#81221=CARTESIAN_POINT('Ctrl Pts',(19.4730962910408,-3.5915775798639,1.60313530873337));
#81222=CARTESIAN_POINT('Ctrl Pts',(19.4746910356535,-3.60424011848294,1.57445983134891));
#81223=CARTESIAN_POINT('Ctrl Pts',(19.4762857802662,-3.61655280561863,1.54565028521073));
#81224=CARTESIAN_POINT('Ctrl Pts',(19.482981668108,-3.66825034479546,1.42468703618701));
#81225=CARTESIAN_POINT('Ctrl Pts',(19.4896775559498,-3.71392777890546,1.30100391030865));
#81226=CARTESIAN_POINT('Ctrl Pts',(19.4963734437916,-3.75332172710987,1.1751872245753));
#81227=CARTESIAN_POINT('Ctrl Pts',(19.5028625956307,-3.791499384424,1.05325513776327));
#81228=CARTESIAN_POINT('Ctrl Pts',(19.5093517474698,-3.82377565411695,0.929319551209696));
#81229=CARTESIAN_POINT('Ctrl Pts',(19.5158408993089,-3.84995753952759,0.803937773608565));
#81230=CARTESIAN_POINT('Ctrl Pts',(19.522640155152,-3.87739060655682,0.672564243580846));
#81231=CARTESIAN_POINT('Ctrl Pts',(19.5294394109952,-3.89813228339126,0.539603086248654));
#81232=CARTESIAN_POINT('Ctrl Pts',(19.5362386668384,-3.91201753782734,0.405718848134176));
#81233=CARTESIAN_POINT('Ctrl Pts',(19.5426799998392,-3.92517185201789,0.278882473516147));
#81234=CARTESIAN_POINT('Ctrl Pts',(19.54912133284,-3.93217292772303,0.151218048903424));
#81235=CARTESIAN_POINT('Ctrl Pts',(19.5555626658407,-3.93293094111045,0.0233069186303194));
#81236=CARTESIAN_POINT('Ctrl Pts',(19.5559205886831,-3.93297306132162,0.0161993346382784));
#81237=CARTESIAN_POINT('Ctrl Pts',(19.5562785115256,-3.93299591809394,0.00909099241931421));
#81238=CARTESIAN_POINT('Ctrl Pts',(19.556636434368,-3.932999500598,0.00198199291543827));
#81239=CARTESIAN_POINT('',(20.8066365087508,-3.93233693810469,-0.00331674980543856));
#81240=CARTESIAN_POINT('Ctrl Pts',(19.5566364779651,-3.92746964905172,0.00197834150499453));
#81241=CARTESIAN_POINT('Ctrl Pts',(19.596135318312,-3.92391641524205,-0.78143951356653));
#81242=CARTESIAN_POINT('Ctrl Pts',(19.7019165649055,-3.31671944988108,-2.88457228488614));
#81243=CARTESIAN_POINT('Ctrl Pts',(19.8739802177454,0.113244265961148,-4.65028676612202));
#81244=CARTESIAN_POINT('Ctrl Pts',(20.072827436485,3.9730950150831,-2.41919558367359));
#81245=CARTESIAN_POINT('Ctrl Pts',(20.2716746552246,4.18334204600648,2.03411912066562));
#81246=CARTESIAN_POINT('Ctrl Pts',(20.4705218739644,0.550856741649847,4.61893365628057));
#81247=CARTESIAN_POINT('Ctrl Pts',(20.6488424815444,-3.16042591545766,3.13204690802899));
#81248=CARTESIAN_POINT('Ctrl Pts',(20.7608806828781,-3.92289919341051,0.902680882788246));
#81249=CARTESIAN_POINT('Ctrl Pts',(20.8066364779651,-3.93009567427408,-0.00331424972451248));
#81250=CARTESIAN_POINT('',(22.0566364779294,-3.93299995833283,-0.000572497990083963));
#81251=CARTESIAN_POINT('Ctrl Pts',(20.8066365178393,-3.93299860084824,-0.00331748787579959));
#81252=CARTESIAN_POINT('Ctrl Pts',(20.8136152576822,-3.93288195755667,-0.1416022140626));
#81253=CARTESIAN_POINT('Ctrl Pts',(20.8205939975251,-3.92546834619834,-0.279571453062378));
#81254=CARTESIAN_POINT('Ctrl Pts',(20.827572737368,-3.91088023639587,-0.416539045670631));
#81255=CARTESIAN_POINT('Ctrl Pts',(20.8346373446069,-3.89611263243974,-0.555191906791886));
#81256=CARTESIAN_POINT('Ctrl Pts',(20.8417019518459,-3.87399296404665,-0.692818279067035));
#81257=CARTESIAN_POINT('Ctrl Pts',(20.8487665590848,-3.84469752196738,-0.828727919511514));
#81258=CARTESIAN_POINT('Ctrl Pts',(20.8552498098711,-3.81781284296527,-0.953453364744746));
#81259=CARTESIAN_POINT('Ctrl Pts',(20.8617330606573,-3.78488542051725,-1.07673324297054));
#81260=CARTESIAN_POINT('Ctrl Pts',(20.8682163114436,-3.74608662368957,-1.19805008568676));
#81261=CARTESIAN_POINT('Ctrl Pts',(20.8740887575775,-3.71094316681251,-1.30793733939193));
#81262=CARTESIAN_POINT('Ctrl Pts',(20.8799612037114,-3.67090164357798,-1.41646091691581));
#81263=CARTESIAN_POINT('Ctrl Pts',(20.8858336498453,-3.62608572291032,-1.52315177513797));
#81264=CARTESIAN_POINT('Ctrl Pts',(20.8916984887901,-3.58132785695687,-1.6297044256163));
#81265=CARTESIAN_POINT('Ctrl Pts',(20.897563327735,-3.53180805149049,-1.73442870046945));
#81266=CARTESIAN_POINT('Ctrl Pts',(20.9034281666798,-3.47769977618529,-1.8368705089692));
#81267=CARTESIAN_POINT('Ctrl Pts',(20.9092869767998,-3.42364712206868,-1.93920701130059));
#81268=CARTESIAN_POINT('Ctrl Pts',(20.9151457869198,-3.3650155719174,-2.03926535085938));
#81269=CARTESIAN_POINT('Ctrl Pts',(20.9210045970398,-3.30202646323742,-2.13661185901413));
#81270=CARTESIAN_POINT('Ctrl Pts',(20.9270903859208,-3.23659706556539,-2.23772971140984));
#81271=CARTESIAN_POINT('Ctrl Pts',(20.9331761748018,-3.16646582044746,-2.33592094330405));
#81272=CARTESIAN_POINT('Ctrl Pts',(20.9392619636827,-3.09193326066032,-2.4307278152073));
#81273=CARTESIAN_POINT('Ctrl Pts',(20.945113993761,-3.02026354121814,-2.52189309827153));
#81274=CARTESIAN_POINT('Ctrl Pts',(20.9509660238393,-2.94452466351218,-2.6099288610706));
#81275=CARTESIAN_POINT('Ctrl Pts',(20.9568180539175,-2.86502720247481,-2.69445878221942));
#81276=CARTESIAN_POINT('Ctrl Pts',(20.962669194296,-2.78554182764865,-2.77897585205869));
#81277=CARTESIAN_POINT('Ctrl Pts',(20.9685203346745,-2.70229928878462,-2.85998783899913));
#81278=CARTESIAN_POINT('Ctrl Pts',(20.974371475053,-2.61564864698193,-2.93715358051662));
#81279=CARTESIAN_POINT('Ctrl Pts',(20.9802231426205,-2.52899019793825,-3.01432627468359));
#81280=CARTESIAN_POINT('Ctrl Pts',(20.986074810188,-2.43892334423997,-3.08765175960288));
#81281=CARTESIAN_POINT('Ctrl Pts',(20.9919264777555,-2.34583145895638,-3.15682811793271));
#81282=CARTESIAN_POINT('Ctrl Pts',(20.9977800894397,-2.25270864548165,-3.22602745892775));
#81283=CARTESIAN_POINT('Ctrl Pts',(21.0036337011239,-2.15655913361623,-3.29107468590123));
#81284=CARTESIAN_POINT('Ctrl Pts',(21.0094873128082,-2.05779599231784,-3.35171070559508));
#81285=CARTESIAN_POINT('Ctrl Pts',(21.015347578908,-1.95892057657606,-3.41241565662577));
#81286=CARTESIAN_POINT('Ctrl Pts',(21.0212078450079,-1.85742595348252,-3.46869917483589));
#81287=CARTESIAN_POINT('Ctrl Pts',(21.0270681111078,-1.75375063665521,-3.52034766811908));
#81288=CARTESIAN_POINT('Ctrl Pts',(21.0329323242791,-1.65000549127859,-3.57203094826832));
#81289=CARTESIAN_POINT('Ctrl Pts',(21.0387965374504,-1.5440771044176,-3.61907281993428));
#81290=CARTESIAN_POINT('Ctrl Pts',(21.0446607506217,-1.43642322460665,-3.66130814324752));
#81291=CARTESIAN_POINT('Ctrl Pts',(21.050533599196,-1.32861081804929,-3.70360566058851));
#81292=CARTESIAN_POINT('Ctrl Pts',(21.0564064477703,-1.2190682370594,-3.74108237014096));
#81293=CARTESIAN_POINT('Ctrl Pts',(21.0622792963446,-1.10826767844745,-3.77362315989669));
#81294=CARTESIAN_POINT('Ctrl Pts',(21.0638740409575,-1.07818030402943,-3.78245945943799));
#81295=CARTESIAN_POINT('Ctrl Pts',(21.0654687855704,-1.04800022150378,-3.79093209223556));
#81296=CARTESIAN_POINT('Ctrl Pts',(21.0670635301833,-1.01773698271176,-3.79903940937979));
#81297=CARTESIAN_POINT('Ctrl Pts',(21.0729359763172,-0.906296418370578,
-3.82889358341765));
#81298=CARTESIAN_POINT('Ctrl Pts',(21.0788084224511,-0.793354555957315,
-3.85389010669937));
#81299=CARTESIAN_POINT('Ctrl Pts',(21.084680868585,-0.679372827779649,-3.87387939420869));
#81300=CARTESIAN_POINT('Ctrl Pts',(21.0905457075299,-0.56553875196647,-3.89384278751889));
#81301=CARTESIAN_POINT('Ctrl Pts',(21.0964105464747,-0.450667892574487,
-3.90881177344058));
#81302=CARTESIAN_POINT('Ctrl Pts',(21.1022753854195,-0.335236031601066,
-3.91868674470369));
#81303=CARTESIAN_POINT('Ctrl Pts',(21.1081341955395,-0.219922830061613,
-3.92855156488293));
#81304=CARTESIAN_POINT('Ctrl Pts',(21.1139930056596,-0.104050183384135,
-3.93333275096322));
#81305=CARTESIAN_POINT('Ctrl Pts',(21.1198518157796,0.0118974230570147,
-3.93298200495815));
#81306=CARTESIAN_POINT('Ctrl Pts',(21.1259376046605,0.132337007136651,-3.93261767054655));
#81307=CARTESIAN_POINT('Ctrl Pts',(21.1320233935415,0.252857029019293,-3.92671564647913));
#81308=CARTESIAN_POINT('Ctrl Pts',(21.1381091824225,0.372909933016485,-3.9152812391778));
#81309=CARTESIAN_POINT('Ctrl Pts',(21.1439612125007,0.488351532933007,-3.90428603432216));
#81310=CARTESIAN_POINT('Ctrl Pts',(21.149813242579,0.603360788043665,-3.88817565361085));
#81311=CARTESIAN_POINT('Ctrl Pts',(21.1556652726573,0.717453202398772,-3.86700787461931));
#81312=CARTESIAN_POINT('Ctrl Pts',(21.1615164130358,0.831528270979573,-3.84584331382172));
#81313=CARTESIAN_POINT('Ctrl Pts',(21.1673675534143,0.94468636964673,-3.81962295893095));
#81314=CARTESIAN_POINT('Ctrl Pts',(21.1732186937928,1.05645176853335,-3.78845597318522));
#81315=CARTESIAN_POINT('Ctrl Pts',(21.1790703613603,1.16822723750603,-3.75728617928748));
#81316=CARTESIAN_POINT('Ctrl Pts',(21.1849220289277,1.27860935906109,-3.72116897957871));
#81317=CARTESIAN_POINT('Ctrl Pts',(21.1907736964952,1.38713686389532,-3.68026362110415));
#81318=CARTESIAN_POINT('Ctrl Pts',(21.1966273081795,1.4957004251418,-3.639344672522));
#81319=CARTESIAN_POINT('Ctrl Pts',(21.2024809198637,1.60240775787166,-3.5936345477074));
#81320=CARTESIAN_POINT('Ctrl Pts',(21.2083345315479,1.70681755991168,-3.5433406295722));
#81321=CARTESIAN_POINT('Ctrl Pts',(21.2141947976478,1.81134605554794,-3.49298953705399));
#81322=CARTESIAN_POINT('Ctrl Pts',(21.2200550637477,1.91357143471598,-3.43804442996549));
#81323=CARTESIAN_POINT('Ctrl Pts',(21.2259153298475,2.01307691302864,-3.37875869843217));
#81324=CARTESIAN_POINT('Ctrl Pts',(21.2317795430188,2.11264941137453,-3.3194330361155));
#81325=CARTESIAN_POINT('Ctrl Pts',(21.2376437561901,2.20949801655538,-3.25576115450926));
#81326=CARTESIAN_POINT('Ctrl Pts',(21.2435079693614,2.30323630212144,-3.18803882294272));
#81327=CARTESIAN_POINT('Ctrl Pts',(21.2493808179357,2.39711262289315,-3.12021676621148));
#81328=CARTESIAN_POINT('Ctrl Pts',(21.25525366651,2.48786916021109,-3.04833261119209));
#81329=CARTESIAN_POINT('Ctrl Pts',(21.2611265150842,2.57515375917751,-2.97272133180928));
#81330=CARTESIAN_POINT('Ctrl Pts',(21.2627212596971,2.59885548453773,-2.95218944188497));
#81331=CARTESIAN_POINT('Ctrl Pts',(21.26431600431,2.6223014184144,-2.93138292674213));
#81332=CARTESIAN_POINT('Ctrl Pts',(21.2659107489229,2.64548500895171,-2.91030892989246));
#81333=CARTESIAN_POINT('Ctrl Pts',(21.2717831950568,2.7308556604786,-2.83270659135749));
#81334=CARTESIAN_POINT('Ctrl Pts',(21.2776556411907,2.81295178012734,-2.75121476599919));
#81335=CARTESIAN_POINT('Ctrl Pts',(21.2835280873247,2.89139803447535,-2.66614073263811));
#81336=CARTESIAN_POINT('Ctrl Pts',(21.2893929262695,2.9697426692469,-2.58117690450365));
#81337=CARTESIAN_POINT('Ctrl Pts',(21.2952577652144,3.04444656349929,-2.49264039756693));
#81338=CARTESIAN_POINT('Ctrl Pts',(21.3011226041592,3.11516866651142,-2.4008775852145));
#81339=CARTESIAN_POINT('Ctrl Pts',(21.3069814142792,3.18581806997047,-2.30920910144061));
#81340=CARTESIAN_POINT('Ctrl Pts',(21.3128402243992,3.25249357282365,-2.21432123441996));
#81341=CARTESIAN_POINT('Ctrl Pts',(21.3186990345193,3.3148925801716,-2.11659542235244));
#81342=CARTESIAN_POINT('Ctrl Pts',(21.3247848234002,3.37970901513408,-2.01508357126305));
#81343=CARTESIAN_POINT('Ctrl Pts',(21.3308706122812,3.43991058973808,-1.91050976967832));
#81344=CARTESIAN_POINT('Ctrl Pts',(21.3369564011622,3.49520569882572,-1.803337495561));
#81345=CARTESIAN_POINT('Ctrl Pts',(21.3428084312404,3.54837688959339,-1.7002817728014));
#81346=CARTESIAN_POINT('Ctrl Pts',(21.3486604613187,3.59701137557048,-1.59482391438598));
#81347=CARTESIAN_POINT('Ctrl Pts',(21.354512491397,3.64089578784765,-1.48740272355311));
#81348=CARTESIAN_POINT('Ctrl Pts',(21.3603636317755,3.68477352826048,-1.37999786425063));
#81349=CARTESIAN_POINT('Ctrl Pts',(21.366214772154,3.72390247459274,-1.27063064858002));
#81350=CARTESIAN_POINT('Ctrl Pts',(21.3720659125325,3.75811722392336,-1.15976029042667));
#81351=CARTESIAN_POINT('Ctrl Pts',(21.3779175801,3.79233505601014,-1.04887994283061));
#81352=CARTESIAN_POINT('Ctrl Pts',(21.3837692476675,3.82163768901133,-0.936496578523215));
#81353=CARTESIAN_POINT('Ctrl Pts',(21.389620915235,3.84590966992567,-0.823084327862094));
#81354=CARTESIAN_POINT('Ctrl Pts',(21.3954745269192,3.87018971479168,-0.709634397915104));
#81355=CARTESIAN_POINT('Ctrl Pts',(21.4013281386035,3.8894356977365,-0.595155305896249));
#81356=CARTESIAN_POINT('Ctrl Pts',(21.4071817502877,3.90358345451057,-0.480130413191341));
#81357=CARTESIAN_POINT('Ctrl Pts',(21.4130420163876,3.91774729452678,-0.364974759601082));
#81358=CARTESIAN_POINT('Ctrl Pts',(21.4189022824875,3.92680128987833,-0.249272477396976));
#81359=CARTESIAN_POINT('Ctrl Pts',(21.4247625485874,3.93073323501185,-0.13351117995613));
#81360=CARTESIAN_POINT('Ctrl Pts',(21.4306267617587,3.93466782843266,-0.0176719136824199));
#81361=CARTESIAN_POINT('Ctrl Pts',(21.43649097493,3.93347350651945,0.0982260346514063));
#81362=CARTESIAN_POINT('Ctrl Pts',(21.4423551881013,3.92719012833042,0.213697674166369));
#81363=CARTESIAN_POINT('Ctrl Pts',(21.4482280366756,3.92089749749296,0.329339352544417));
#81364=CARTESIAN_POINT('Ctrl Pts',(21.4541008852499,3.90950089450785,0.444553059408025));
#81365=CARTESIAN_POINT('Ctrl Pts',(21.4599737338241,3.89309168866756,0.558861435087084));
#81366=CARTESIAN_POINT('Ctrl Pts',(21.4615684784369,3.88863584542845,0.589901340850946));
#81367=CARTESIAN_POINT('Ctrl Pts',(21.4631632230497,3.88381067593326,0.620874565206294));
#81368=CARTESIAN_POINT('Ctrl Pts',(21.4647579676625,3.87861864671218,0.6517717341037));
#81369=CARTESIAN_POINT('Ctrl Pts',(21.4706304137965,3.85949965318686,0.765546666205749));
#81370=CARTESIAN_POINT('Ctrl Pts',(21.4765028599304,3.83533821575921,0.878670118252889));
#81371=CARTESIAN_POINT('Ctrl Pts',(21.4823753060643,3.80618987348751,0.990660207619714));
#81372=CARTESIAN_POINT('Ctrl Pts',(21.4882401450091,3.77707929008933,1.10250522459853));
#81373=CARTESIAN_POINT('Ctrl Pts',(21.494104983954,3.74299475175835,1.21321940220833));
#81374=CARTESIAN_POINT('Ctrl Pts',(21.4999698228988,3.70404322125797,1.32232855790567));
#81375=CARTESIAN_POINT('Ctrl Pts',(21.5058286330189,3.66513173140596,1.43132555366265));
#81376=CARTESIAN_POINT('Ctrl Pts',(21.5116874431389,3.62136333892159,1.53872042229152));
#81377=CARTESIAN_POINT('Ctrl Pts',(21.5175462532589,3.57289529685836,1.64405237072527));
#81378=CARTESIAN_POINT('Ctrl Pts',(21.5236320421399,3.52254953288448,1.7534650308826));
#81379=CARTESIAN_POINT('Ctrl Pts',(21.5297178310209,3.46713272661096,1.86065125735366));
#81380=CARTESIAN_POINT('Ctrl Pts',(21.5358036199018,3.4068770859369,1.96511514200011));
#81381=CARTESIAN_POINT('Ctrl Pts',(21.5416556499801,3.34893590057752,2.06556650615375));
#81382=CARTESIAN_POINT('Ctrl Pts',(21.5475076800584,3.28652097455898,2.1635004131418));
#81383=CARTESIAN_POINT('Ctrl Pts',(21.5533597101366,3.21988606232296,2.25850010973175));
#81384=CARTESIAN_POINT('Ctrl Pts',(21.5592108505152,3.15326128077052,2.35348536326424));
#81385=CARTESIAN_POINT('Ctrl Pts',(21.5650619908937,3.08241802596525,2.44553695506596));
#81386=CARTESIAN_POINT('Ctrl Pts',(21.5709131312722,3.00765315766804,2.53426744507549));
#81387=CARTESIAN_POINT('Ctrl Pts',(21.5767647988397,2.93288155304041,2.6230059297209));
#81388=CARTESIAN_POINT('Ctrl Pts',(21.5826164664072,2.85418789888381,2.70842240160628));
#81389=CARTESIAN_POINT('Ctrl Pts',(21.5884681339747,2.7719086112616,2.79016337349872));
#81390=CARTESIAN_POINT('Ctrl Pts',(21.594321745659,2.68960198774951,2.87193150243483));
#81391=CARTESIAN_POINT('Ctrl Pts',(21.6001753573432,2.60370765510291,2.95002141207857));
#81392=CARTESIAN_POINT('Ctrl Pts',(21.6060289690274,2.51459752696156,3.02411776844071));
#81393=CARTESIAN_POINT('Ctrl Pts',(21.6118892351273,2.42538609797146,3.09829835791917));
#81394=CARTESIAN_POINT('Ctrl Pts',(21.6177495012272,2.33295189478774,3.1684760682044));
#81395=CARTESIAN_POINT('Ctrl Pts',(21.6236097673271,2.23769850246221,3.23437697433035));
#81396=CARTESIAN_POINT('Ctrl Pts',(21.6294739804984,2.14238095401548,3.30032226676547));
#81397=CARTESIAN_POINT('Ctrl Pts',(21.6353381936698,2.04424078465955,3.36198479989251));
#81398=CARTESIAN_POINT('Ctrl Pts',(21.6412024068411,1.943707525246,3.41913586397237));
#81399=CARTESIAN_POINT('Ctrl Pts',(21.6470752554154,1.84302622462333,3.47637108639622));
#81400=CARTESIAN_POINT('Ctrl Pts',(21.6529481039897,1.73994516745276,3.52908139337201));
#81401=CARTESIAN_POINT('Ctrl Pts',(21.658820952564,1.63491531725601,3.57708553230164));
#81402=CARTESIAN_POINT('Ctrl Pts',(21.6604156971767,1.60639495177096,3.59012083211882));
#81403=CARTESIAN_POINT('Ctrl Pts',(21.6620104417894,1.57773098079289,3.60280939607684));
#81404=CARTESIAN_POINT('Ctrl Pts',(21.6636051864022,1.54893262353388,3.61514823039837));
#81405=CARTESIAN_POINT('Ctrl Pts',(21.6694776325361,1.44288630088227,3.66058443336778));
#81406=CARTESIAN_POINT('Ctrl Pts',(21.67535007867,1.33466150801162,3.70142662564121));
#81407=CARTESIAN_POINT('Ctrl Pts',(21.6812225248039,1.2246936394195,3.73746096829993));
#81408=CARTESIAN_POINT('Ctrl Pts',(21.6870873637488,1.11486822362282,3.77344863193404));
#81409=CARTESIAN_POINT('Ctrl Pts',(21.6929522026936,1.00330461162231,3.80464070391446));
#81410=CARTESIAN_POINT('Ctrl Pts',(21.6988170416385,0.890459525861827,3.83087076691474));
#81411=CARTESIAN_POINT('Ctrl Pts',(21.7046758517585,0.777730440431554,3.85707386643718));
#81412=CARTESIAN_POINT('Ctrl Pts',(21.7105346618785,0.663722901638883,3.87832500962752));
#81413=CARTESIAN_POINT('Ctrl Pts',(21.7163934719985,0.548909561055544,3.89450732362668));
#81414=CARTESIAN_POINT('Ctrl Pts',(21.7224792608795,0.429648185930714,3.91131656382851));
#81415=CARTESIAN_POINT('Ctrl Pts',(21.7285650497605,0.309517742174652,3.92265614255285));
#81416=CARTESIAN_POINT('Ctrl Pts',(21.7346508386414,0.189060949322586,3.92845325254625));
#81417=CARTESIAN_POINT('Ctrl Pts',(21.7405028687197,0.0732309741642367,
3.93402769206625));
#81418=CARTESIAN_POINT('Ctrl Pts',(21.746354898798,-0.0429002909674251,
3.93447756619805));
#81419=CARTESIAN_POINT('Ctrl Pts',(21.7522069288763,-0.158845061913345,
3.92979099269996));
#81420=CARTESIAN_POINT('Ctrl Pts',(21.7580580692548,-0.27477220546626,3.92510513171415));
#81421=CARTESIAN_POINT('Ctrl Pts',(21.7639092096333,-0.390512498301815,
3.91528439248784));
#81422=CARTESIAN_POINT('Ctrl Pts',(21.7697603500118,-0.505579507274324,
3.90036900328985));
#81423=CARTESIAN_POINT('Ctrl Pts',(21.7756120175793,-0.620656883808554,
3.88545227021215));
#81424=CARTESIAN_POINT('Ctrl Pts',(21.7814636851468,-0.735060445935161,
3.86544002779491));
#81425=CARTESIAN_POINT('Ctrl Pts',(21.7873153527143,-0.848310933432702,
3.84042413806321));
#81426=CARTESIAN_POINT('Ctrl Pts',(21.7931689643985,-0.961599046472934,
3.81539993722886));
#81427=CARTESIAN_POINT('Ctrl Pts',(21.7990225760827,-1.07373291972062,3.78536887265583));
#81428=CARTESIAN_POINT('Ctrl Pts',(21.804876187767,-1.18424619389995,3.75047329709645));
#81429=CARTESIAN_POINT('Ctrl Pts',(21.8107364538669,-1.29488510013388,3.71553805206851));
#81430=CARTESIAN_POINT('Ctrl Pts',(21.8165967199668,-1.40389933571341,3.6757273828946));
#81431=CARTESIAN_POINT('Ctrl Pts',(21.8224569860666,-1.51084024994538,3.63123267488397));
#81432=CARTESIAN_POINT('Ctrl Pts',(21.8283211992379,-1.6178531922078,3.58670799830419));
#81433=CARTESIAN_POINT('Ctrl Pts',(21.8341854124092,-1.72278965919017,3.53749317604446));
#81434=CARTESIAN_POINT('Ctrl Pts',(21.8400496255805,-1.8252250064917,3.4838258675883));
#81435=CARTESIAN_POINT('Ctrl Pts',(21.8459224741548,-1.92781119594008,3.43007953082564));
#81436=CARTESIAN_POINT('Ctrl Pts',(21.8517953227291,-2.02788855911491,3.37186782934882));
#81437=CARTESIAN_POINT('Ctrl Pts',(21.8576681713034,-2.12506078412123,3.30947211255663));
#81438=CARTESIAN_POINT('Ctrl Pts',(21.8592629159162,-2.15144744817087,3.29252884695759));
#81439=CARTESIAN_POINT('Ctrl Pts',(21.8608576605291,-2.17762008388537,3.27527729550833));
#81440=CARTESIAN_POINT('Ctrl Pts',(21.8624524051419,-2.20357118795022,3.25772359472618));
#81441=CARTESIAN_POINT('Ctrl Pts',(21.8683016986376,-2.2987560990595,3.19333914910054));
#81442=CARTESIAN_POINT('Ctrl Pts',(21.8741509921333,-2.39128240582993,3.12466742122805));
#81443=CARTESIAN_POINT('Ctrl Pts',(21.880000285629,-2.48073667426204,3.05195585698275));
#81444=CARTESIAN_POINT('Ctrl Pts',(21.8858419879227,-2.57007484911417,2.97933865766768));
#81445=CARTESIAN_POINT('Ctrl Pts',(21.8916836902164,-2.6563485922422,2.90269230695721));
#81446=CARTESIAN_POINT('Ctrl Pts',(21.8975253925101,-2.73917266184636,2.82230794361522));
#81447=CARTESIAN_POINT('Ctrl Pts',(21.9033611086428,-2.82191185923516,2.74200595245112));
#81448=CARTESIAN_POINT('Ctrl Pts',(21.9091968247755,-2.90120811580661,2.6579738550509));
#81449=CARTESIAN_POINT('Ctrl Pts',(21.9150325409082,-2.9767091378659,2.5705430765785));
#81450=CARTESIAN_POINT('Ctrl Pts',(21.9209327049507,-3.05304397071259,2.48214673864408));
#81451=CARTESIAN_POINT('Ctrl Pts',(21.9268328689933,-3.12549889273747,2.39027646314334));
#81452=CARTESIAN_POINT('Ctrl Pts',(21.9327330330358,-3.19374784495553,2.29531342148342));
#81453=CARTESIAN_POINT('Ctrl Pts',(21.9385621855732,-3.2611753859737,2.20149330881303));
#81454=CARTESIAN_POINT('Ctrl Pts',(21.9443913381105,-3.32449740350828,2.10465482189322));
#81455=CARTESIAN_POINT('Ctrl Pts',(21.9502204906479,-3.38344044542388,2.00519818279137));
#81456=CARTESIAN_POINT('Ctrl Pts',(21.956048824259,-3.4423752065467,1.90575551615842));
#81457=CARTESIAN_POINT('Ctrl Pts',(21.9618771578701,-3.49693200260813,1.80369578730248));
#81458=CARTESIAN_POINT('Ctrl Pts',(21.9677054914812,-3.54688186239486,1.69944639639336));
#81459=CARTESIAN_POINT('Ctrl Pts',(21.9735344467611,-3.59683704999491,1.5951858859076));
#81460=CARTESIAN_POINT('Ctrl Pts',(21.9793634020411,-3.64218414461965,1.48873562533101));
#81461=CARTESIAN_POINT('Ctrl Pts',(21.9851923573211,-3.6827414384427,1.38054500019992));
#81462=CARTESIAN_POINT('Ctrl Pts',(21.9911460340385,-3.72416653168075,1.27003943360337));
#81463=CARTESIAN_POINT('Ctrl Pts',(21.9970997107558,-3.76059434010847,1.1577185980051));
#81464=CARTESIAN_POINT('Ctrl Pts',(22.0030533874732,-3.7918846222398,1.04407854667229));
#81465=CARTESIAN_POINT('Ctrl Pts',(22.0088910875013,-3.82256537457987,0.93265218572669));
#81466=CARTESIAN_POINT('Ctrl Pts',(22.0147287875294,-3.84830690806666,0.819957963166135));
#81467=CARTESIAN_POINT('Ctrl Pts',(22.0205664875576,-3.86902884222337,0.706473508380677));
#81468=CARTESIAN_POINT('Ctrl Pts',(22.0265781526195,-3.89036829560161,0.58960718626344));
#81469=CARTESIAN_POINT('Ctrl Pts',(22.0325898176815,-3.90638422816247,0.47190327475391));
#81470=CARTESIAN_POINT('Ctrl Pts',(22.0386014827435,-3.91704643023887,0.353887359696457));
#81471=CARTESIAN_POINT('Ctrl Pts',(22.0446131478055,-3.92770863231527,0.235871444638986));
#81472=CARTESIAN_POINT('Ctrl Pts',(22.0506248128675,-3.93301715168668,0.117544003992333));
#81473=CARTESIAN_POINT('Ctrl Pts',(22.0566364779294,-3.93299995833283,-0.000572497990078241));
#81474=CARTESIAN_POINT('',(23.3066364599429,-3.93299834994999,0.00360267826161876));
#81475=CARTESIAN_POINT('Ctrl Pts',(22.0566364779651,-3.93299995833273,-0.000572498690872157));
#81476=CARTESIAN_POINT('Ctrl Pts',(22.0581908599372,-3.93299551279697,-0.0311128164560471));
#81477=CARTESIAN_POINT('Ctrl Pts',(22.0597452419094,-3.93263534867649,-0.0616502033595227));
#81478=CARTESIAN_POINT('Ctrl Pts',(22.0612996238815,-3.93191963181071,-0.0921792220707062));
#81479=CARTESIAN_POINT('Ctrl Pts',(22.0671720700154,-3.92921565761587,-0.207517678848141));
#81480=CARTESIAN_POINT('Ctrl Pts',(22.0730445161493,-3.92142786721891,-0.322930159899214));
#81481=CARTESIAN_POINT('Ctrl Pts',(22.0789169622832,-3.90854253527997,-0.437931786819878));
#81482=CARTESIAN_POINT('Ctrl Pts',(22.0847818012281,-3.89567389504906,-0.552784440195304));
#81483=CARTESIAN_POINT('Ctrl Pts',(22.0906466401729,-3.87772089064231,-0.667226890841104));
#81484=CARTESIAN_POINT('Ctrl Pts',(22.0965114791178,-3.85472179291523,-0.780774550830383));
#81485=CARTESIAN_POINT('Ctrl Pts',(22.1023702892378,-3.83174633736018,-0.89420548827065));
#81486=CARTESIAN_POINT('Ctrl Pts',(22.1082290993578,-3.80373518764924,-1.0067430619087));
#81487=CARTESIAN_POINT('Ctrl Pts',(22.1140879094778,-3.77077830007421,-1.11790876715833));
#81488=CARTESIAN_POINT('Ctrl Pts',(22.1201736983588,-3.73654461510292,-1.23338119229143));
#81489=CARTESIAN_POINT('Ctrl Pts',(22.1262594872398,-3.69697428242109,-1.34737285134649));
#81490=CARTESIAN_POINT('Ctrl Pts',(22.1323452761207,-3.65222644159015,-1.45935979777085));
#81491=CARTESIAN_POINT('Ctrl Pts',(22.138197306199,-3.60919739217649,-1.56704525838521));
#81492=CARTESIAN_POINT('Ctrl Pts',(22.1440493362773,-3.56138140768638,-1.6728767506504));
#81493=CARTESIAN_POINT('Ctrl Pts',(22.1499013663556,-3.5089702384656,-1.77640560277282));
#81494=CARTESIAN_POINT('Ctrl Pts',(22.1557525067341,-3.45656703745475,-1.87991871512755));
#81495=CARTESIAN_POINT('Ctrl Pts',(22.1616036471126,-3.39957022744269,-1.98112951471479));
#81496=CARTESIAN_POINT('Ctrl Pts',(22.1674547874911,-3.3382184027067,-2.07961219842314));
#81497=CARTESIAN_POINT('Ctrl Pts',(22.1733064550586,-3.27686105015837,-2.17810375544204));
#81498=CARTESIAN_POINT('Ctrl Pts',(22.1791581226261,-3.21114812143522,-2.27386635708007));
#81499=CARTESIAN_POINT('Ctrl Pts',(22.1850097901936,-3.14136220340735,-2.36650216712425));
#81500=CARTESIAN_POINT('Ctrl Pts',(22.1908634018779,-3.07155310019859,-2.45916875383616));
#81501=CARTESIAN_POINT('Ctrl Pts',(22.1967170135621,-2.99766856555371,-2.54870615333636));
#81502=CARTESIAN_POINT('Ctrl Pts',(22.2025706252463,-2.92003176047537,-2.63474923243467));
#81503=CARTESIAN_POINT('Ctrl Pts',(22.2084308913462,-2.84230669748049,-2.72089012574476));
#81504=CARTESIAN_POINT('Ctrl Pts',(22.2142911574461,-2.76082112713157,-2.80352846287704));
#81505=CARTESIAN_POINT('Ctrl Pts',(22.220151423546,-2.67593546162276,-2.88233558164725));
#81506=CARTESIAN_POINT('Ctrl Pts',(22.2260156367173,-2.59099262297914,-2.96119577946206));
#81507=CARTESIAN_POINT('Ctrl Pts',(22.2318798498886,-2.50264544349439,-3.03621935382319));
#81508=CARTESIAN_POINT('Ctrl Pts',(22.23774406306,-2.41128646203427,-3.10711869712283));
#81509=CARTESIAN_POINT('Ctrl Pts',(22.2436169116343,-2.31979294903535,-3.17812244392611));
#81510=CARTESIAN_POINT('Ctrl Pts',(22.2494897602086,-2.22527911874374,-3.24498960098023));
#81511=CARTESIAN_POINT('Ctrl Pts',(22.2553626087829,-2.1281654892705,-3.30747647766058));
#81512=CARTESIAN_POINT('Ctrl Pts',(22.2569573533956,-2.10179473656521,-3.3244444973011));
#81513=CARTESIAN_POINT('Ctrl Pts',(22.2585520980084,-2.07523241450326,-3.34108979496335));
#81514=CARTESIAN_POINT('Ctrl Pts',(22.2601468426212,-2.04848722134078,-3.3574080931581));
#81515=CARTESIAN_POINT('Ctrl Pts',(22.2660192887551,-1.9500014168234,-3.41749817051523));
#81516=CARTESIAN_POINT('Ctrl Pts',(22.271891734889,-1.84870447095246,-3.47335172204802));
#81517=CARTESIAN_POINT('Ctrl Pts',(22.2777641810229,-1.74499684633191,-3.5246950231604));
#81518=CARTESIAN_POINT('Ctrl Pts',(22.2836290199677,-1.64142356496303,-3.5759718139651));
#81519=CARTESIAN_POINT('Ctrl Pts',(22.2894938589126,-1.53544618201719,-3.62274979148631));
#81520=CARTESIAN_POINT('Ctrl Pts',(22.2953586978574,-1.42749303062162,-3.66479912785499));
#81521=CARTESIAN_POINT('Ctrl Pts',(22.3012175079775,-1.31965085083926,-3.70680523915214));
#81522=CARTESIAN_POINT('Ctrl Pts',(22.3070763180975,-1.20983732525929,-3.7440922286813));
#81523=CARTESIAN_POINT('Ctrl Pts',(22.3129351282175,-1.09850361649316,-3.77647703614777));
#81524=CARTESIAN_POINT('Ctrl Pts',(22.3190209170985,-0.982856679144769,
-3.81011647780135));
#81525=CARTESIAN_POINT('Ctrl Pts',(22.3251067059794,-0.865569795360856,
-3.83846601844896));
#81526=CARTESIAN_POINT('Ctrl Pts',(22.3311924948604,-0.747169762042387,
-3.86137622444246));
#81527=CARTESIAN_POINT('Ctrl Pts',(22.3370445249387,-0.633317545049769,
-3.88340643567645));
#81528=CARTESIAN_POINT('Ctrl Pts',(22.3428965550169,-0.518436557948746,
-3.90040737478319));
#81529=CARTESIAN_POINT('Ctrl Pts',(22.3487485850952,-0.40300790882696,-3.91229774243001));
#81530=CARTESIAN_POINT('Ctrl Pts',(22.3545997254737,-0.2875968086308,-3.92418630235249));
#81531=CARTESIAN_POINT('Ctrl Pts',(22.3604508658522,-0.17163862303592,-3.93096579334788));
#81532=CARTESIAN_POINT('Ctrl Pts',(22.3663020062307,-0.0556205517840449,
-3.93260668694687));
#81533=CARTESIAN_POINT('Ctrl Pts',(22.3721536737982,0.0604079727206123,
-3.93424772839072));
#81534=CARTESIAN_POINT('Ctrl Pts',(22.3780053413657,0.17649598026796,-3.93074924621335));
#81535=CARTESIAN_POINT('Ctrl Pts',(22.3838570089332,0.292156009875148,-3.92213384089501));
#81536=CARTESIAN_POINT('Ctrl Pts',(22.3897106206175,0.407854465554346,-3.91351557325521));
#81537=CARTESIAN_POINT('Ctrl Pts',(22.3955642323017,0.523124248563739,-3.89977703279664));
#81538=CARTESIAN_POINT('Ctrl Pts',(22.4014178439859,0.637483469145844,-3.88099263418082));
#81539=CARTESIAN_POINT('Ctrl Pts',(22.4072781100858,0.751972693873832,-3.86218688136474));
#81540=CARTESIAN_POINT('Ctrl Pts',(22.4131383761857,0.865548881953724,-3.83832388825205));
#81541=CARTESIAN_POINT('Ctrl Pts',(22.4189986422856,0.97774068126266,-3.80952912578497));
#81542=CARTESIAN_POINT('Ctrl Pts',(22.4248628554569,1.09000804523644,-3.78071496915015));
#81543=CARTESIAN_POINT('Ctrl Pts',(22.4307270686282,1.20088876931135,-3.74696254906766));
#81544=CARTESIAN_POINT('Ctrl Pts',(22.4365912817995,1.3099286656199,-3.70844656035209));
#81545=CARTESIAN_POINT('Ctrl Pts',(22.4424641303738,1.41912912966684,-3.66987385455031));
#81546=CARTESIAN_POINT('Ctrl Pts',(22.4483369789481,1.52648297402847,-3.62652373448567));
#81547=CARTESIAN_POINT('Ctrl Pts',(22.4542098275224,1.63155782553067,-3.57861817772581));
#81548=CARTESIAN_POINT('Ctrl Pts',(22.4558045721352,1.6600904109113,-3.56560964743607));
#81549=CARTESIAN_POINT('Ctrl Pts',(22.457399316748,1.68845510319967,-3.55226546821775));
#81550=CARTESIAN_POINT('Ctrl Pts',(22.4589940613608,1.71664360089758,-3.53859064423923));
#81551=CARTESIAN_POINT('Ctrl Pts',(22.4648665074947,1.82044419254028,-3.48823482766493));
#81552=CARTESIAN_POINT('Ctrl Pts',(22.4707389536286,1.9222009938083,-3.43322352103325));
#81553=CARTESIAN_POINT('Ctrl Pts',(22.4766113997625,2.02146721090104,-3.37374559136459));
#81554=CARTESIAN_POINT('Ctrl Pts',(22.4824762387074,2.12060483815836,-3.31434470963238));
#81555=CARTESIAN_POINT('Ctrl Pts',(22.4883410776522,2.21725794591733,-3.25048892181649));
#81556=CARTESIAN_POINT('Ctrl Pts',(22.4942059165971,2.3110015968181,-3.18241427527972));
#81557=CARTESIAN_POINT('Ctrl Pts',(22.5000647267171,2.40464888291587,-3.11440960681443));
#81558=CARTESIAN_POINT('Ctrl Pts',(22.5059235368371,2.49539232857328,-3.04219494723135));
#81559=CARTESIAN_POINT('Ctrl Pts',(22.5117823469572,2.58283399359506,-2.96605083596519));
#81560=CARTESIAN_POINT('Ctrl Pts',(22.5178681358381,2.67366327493734,-2.88695679191847));
#81561=CARTESIAN_POINT('Ctrl Pts',(22.5239539247191,2.76092938022794,-2.80362290667319));
#81562=CARTESIAN_POINT('Ctrl Pts',(22.5300397136001,2.84422176007164,-2.71641152617474));
#81563=CARTESIAN_POINT('Ctrl Pts',(22.5358917436784,2.92431482962595,-2.63254998713243));
#81564=CARTESIAN_POINT('Ctrl Pts',(22.5417437737566,3.00073349716659,-2.54510365856938));
#81565=CARTESIAN_POINT('Ctrl Pts',(22.5475958038349,3.07314923290107,-2.45443329351596));
#81566=CARTESIAN_POINT('Ctrl Pts',(22.5534469442134,3.14555395907795,-2.36377671332015));
#81567=CARTESIAN_POINT('Ctrl Pts',(22.5592980845919,3.21395670560722,-2.26989739412847));
#81568=CARTESIAN_POINT('Ctrl Pts',(22.5651492249705,3.2780691989884,-2.1731892063609));
#81569=CARTESIAN_POINT('Ctrl Pts',(22.571000892538,3.3421874689188,-2.07647230516516));
#81570=CARTESIAN_POINT('Ctrl Pts',(22.5768525601055,3.40201448885485,-1.97692637325704));
#81571=CARTESIAN_POINT('Ctrl Pts',(22.582704227673,3.45730569537737,-1.87497368747169));
#81572=CARTESIAN_POINT('Ctrl Pts',(22.5885578393572,3.51261527146017,-1.77298712964547));
#81573=CARTESIAN_POINT('Ctrl Pts',(22.5944114510415,3.56338584070317,-1.66859259114971));
#81574=CARTESIAN_POINT('Ctrl Pts',(22.6002650627257,3.60941943865695,-1.56223567871347));
#81575=CARTESIAN_POINT('Ctrl Pts',(22.6061253288256,3.65550536783994,-1.4557578591961));
#81576=CARTESIAN_POINT('Ctrl Pts',(22.6119855949255,3.69684341314009,-1.34731359263554));
#81577=CARTESIAN_POINT('Ctrl Pts',(22.6178458610254,3.73328425691335,-1.23736722806243));
#81578=CARTESIAN_POINT('Ctrl Pts',(22.6237100741968,3.76974964472785,-1.12734681119453));
#81579=CARTESIAN_POINT('Ctrl Pts',(22.6295742873681,3.8013111509184,-1.0158226785602));
#81580=CARTESIAN_POINT('Ctrl Pts',(22.6354385005394,3.82787014628981,-0.903271356317258));
#81581=CARTESIAN_POINT('Ctrl Pts',(22.6413113491137,3.85446825136294,-0.790554295552259));
#81582=CARTESIAN_POINT('Ctrl Pts',(22.647184197688,3.87604906679985,-0.676807430918695));
#81583=CARTESIAN_POINT('Ctrl Pts',(22.6530570462623,3.89256553350679,-0.56251450412859));
#81584=CARTESIAN_POINT('Ctrl Pts',(22.654651790875,3.8970505029333,-0.531478793439604));
#81585=CARTESIAN_POINT('Ctrl Pts',(22.6562465354877,3.90116233997505,-0.500402827103983));
#81586=CARTESIAN_POINT('Ctrl Pts',(22.6578412801005,3.90490076547796,-0.469296294221111));
#81587=CARTESIAN_POINT('Ctrl Pts',(22.6637137262344,3.91866704643364,-0.354750405613924));
#81588=CARTESIAN_POINT('Ctrl Pts',(22.6695861723683,3.92741198927103,-0.239406500546002));
#81589=CARTESIAN_POINT('Ctrl Pts',(22.6754586185022,3.93105288462848,-0.12374254827698));
#81590=CARTESIAN_POINT('Ctrl Pts',(22.681323457447,3.93468906355624,-0.00822842753193724));
#81591=CARTESIAN_POINT('Ctrl Pts',(22.6871882963919,3.93323433064254,0.107604506597884));
#81592=CARTESIAN_POINT('Ctrl Pts',(22.6930531353367,3.92665748305163,0.223271159791434));
#81593=CARTESIAN_POINT('Ctrl Pts',(22.6989119454567,3.92008739620257,0.338818912193898));
#81594=CARTESIAN_POINT('Ctrl Pts',(22.7047707555767,3.9084056910377,0.454200313437066));
#81595=CARTESIAN_POINT('Ctrl Pts',(22.7106295656967,3.89163318949212,0.568928922136524));
#81596=CARTESIAN_POINT('Ctrl Pts',(22.7167153545777,3.87421089702634,0.688102282742312));
#81597=CARTESIAN_POINT('Ctrl Pts',(22.7228011434587,3.85129536657459,0.80657079343946));
#81598=CARTESIAN_POINT('Ctrl Pts',(22.7288869323396,3.82296941851443,0.923793172254195));
#81599=CARTESIAN_POINT('Ctrl Pts',(22.7347389624179,3.79573148711634,1.03651296915895));
#81600=CARTESIAN_POINT('Ctrl Pts',(22.7405909924961,3.7634912120264,1.14808015873495));
#81601=CARTESIAN_POINT('Ctrl Pts',(22.7464430225744,3.72637442248686,1.25802331593485));
#81602=CARTESIAN_POINT('Ctrl Pts',(22.7522941629529,3.68926327591191,1.3679497581831));
#81603=CARTESIAN_POINT('Ctrl Pts',(22.7581453033314,3.64727722119318,1.47625226745097));
#81604=CARTESIAN_POINT('Ctrl Pts',(22.7639964437099,3.60059171320558,1.58247537573111));
#81605=CARTESIAN_POINT('Ctrl Pts',(22.7698481112774,3.55390199884383,1.68870805473579));
#81606=CARTESIAN_POINT('Ctrl Pts',(22.7756997788449,3.50251215581756,1.79286058186567));
#81607=CARTESIAN_POINT('Ctrl Pts',(22.7815514464124,3.44664516921986,1.89449889878391));
#81608=CARTESIAN_POINT('Ctrl Pts',(22.7874050580966,3.3907596217688,1.99617098329925));
#81609=CARTESIAN_POINT('Ctrl Pts',(22.7932586697808,3.3303941720394,2.09532683460348));
#81610=CARTESIAN_POINT('Ctrl Pts',(22.799112281465,3.26581662697953,2.19155897911601));
#81611=CARTESIAN_POINT('Ctrl Pts',(22.8049725475649,3.20116566983665,2.28790052082187));
#81612=CARTESIAN_POINT('Ctrl Pts',(22.8108328136648,3.1322932904819,2.38131137833333));
#81613=CARTESIAN_POINT('Ctrl Pts',(22.8166930797647,3.05950936588006,2.47141486604175));
#81614=CARTESIAN_POINT('Ctrl Pts',(22.822557292936,2.98667641904217,2.56157904125045));
#81615=CARTESIAN_POINT('Ctrl Pts',(22.8284215061072,2.90992695409135,2.64843110203499));
#81616=CARTESIAN_POINT('Ctrl Pts',(22.8342857192785,2.82960849926366,2.73163041806443));
#81617=CARTESIAN_POINT('Ctrl Pts',(22.8401585678528,2.74917177072991,2.81495225003954));
#81618=CARTESIAN_POINT('Ctrl Pts',(22.8460314164271,2.66515586212278,2.894610318744));
#81619=CARTESIAN_POINT('Ctrl Pts',(22.8519042650014,2.57794225594872,2.97030347355182));
#81620=CARTESIAN_POINT('Ctrl Pts',(22.8534990096143,2.55425980834995,2.99085759636546));
#81621=CARTESIAN_POINT('Ctrl Pts',(22.8550937542271,2.53034174084131,3.01111960353115));
#81622=CARTESIAN_POINT('Ctrl Pts',(22.85668849884,2.50619605303813,3.03108402122675));
#81623=CARTESIAN_POINT('Ctrl Pts',(22.8625609449739,2.41728259953259,3.10460047430989));
#81624=CARTESIAN_POINT('Ctrl Pts',(22.8684333911079,2.32498275853158,3.1743244286784));
#81625=CARTESIAN_POINT('Ctrl Pts',(22.8743058372418,2.22965388023827,3.23992786560726));
#81626=CARTESIAN_POINT('Ctrl Pts',(22.8801706761866,2.13444849133673,3.30544631959424));
#81627=CARTESIAN_POINT('Ctrl Pts',(22.8860355151315,2.03622220561441,3.36685463882064));
#81628=CARTESIAN_POINT('Ctrl Pts',(22.8919003540763,1.93536621704558,3.42386427971651));
#81629=CARTESIAN_POINT('Ctrl Pts',(22.8977591641963,1.83461390448438,3.48081531693353));
#81630=CARTESIAN_POINT('Ctrl Pts',(22.9036179743163,1.731237623639,3.53337646748249));
#81631=CARTESIAN_POINT('Ctrl Pts',(22.9094767844364,1.62565783197171,3.58130222312346));
#81632=CARTESIAN_POINT('Ctrl Pts',(22.9155625733173,1.51598772677603,3.63108469171641));
#81633=CARTESIAN_POINT('Ctrl Pts',(22.9216483621983,1.40394029758123,3.67586507998539));
#81634=CARTESIAN_POINT('Ctrl Pts',(22.9277341510793,1.29001565743486,3.71542038046476));
#81635=CARTESIAN_POINT('Ctrl Pts',(22.9335861811576,1.18046693107724,3.75345633811747));
#81636=CARTESIAN_POINT('Ctrl Pts',(22.9394382112358,1.06918296982486,3.78666105308058));
#81637=CARTESIAN_POINT('Ctrl Pts',(22.9452902413141,0.956628377789582,3.8148854696842));
#81638=CARTESIAN_POINT('Ctrl Pts',(22.9511413816926,0.844090897729359,3.84310559525444));
#81639=CARTESIAN_POINT('Ctrl Pts',(22.9569925220711,0.730283571819675,3.86634682744824));
#81640=CARTESIAN_POINT('Ctrl Pts',(22.9628436624496,0.615684414055787,3.88451048425523));
#81641=CARTESIAN_POINT('Ctrl Pts',(22.9686953300171,0.501074930883504,3.90267577761154));
#81642=CARTESIAN_POINT('Ctrl Pts',(22.9745469975846,0.385673882316584,3.91576252141985));
#81643=CARTESIAN_POINT('Ctrl Pts',(22.9803986651521,0.269966972420246,3.92372359294105));
#81644=CARTESIAN_POINT('Ctrl Pts',(22.9862522768364,0.154221620876628,3.93168730939248));
#81645=CARTESIAN_POINT('Ctrl Pts',(22.9921058885206,0.0381706181077041,
3.9345219390514));
#81646=CARTESIAN_POINT('Ctrl Pts',(22.9979595002049,-0.0776984595194039,
3.93223243837242));
#81647=CARTESIAN_POINT('Ctrl Pts',(23.0038197663047,-0.193699257705575,
3.92994033497738));
#81648=CARTESIAN_POINT('Ctrl Pts',(23.0096800324046,-0.30951730443686,3.92251248263557));
#81649=CARTESIAN_POINT('Ctrl Pts',(23.0155402985045,-0.424668174773692,
3.91000587484653));
#81650=CARTESIAN_POINT('Ctrl Pts',(23.0214045116758,-0.539896602801737,
3.89749084346831));
#81651=CARTESIAN_POINT('Ctrl Pts',(23.0272687248471,-0.654456552097231,
3.87989030795856));
#81652=CARTESIAN_POINT('Ctrl Pts',(23.0331329380184,-0.767873569313706,
3.85731242985961));
#81653=CARTESIAN_POINT('Ctrl Pts',(23.0390057865927,-0.881457599839678,
3.83470130449111));
#81654=CARTESIAN_POINT('Ctrl Pts',(23.044878635167,-0.993894939356715,3.80709830662511));
#81655=CARTESIAN_POINT('Ctrl Pts',(23.0507514837413,-1.10472598577643,3.77466150751962));
#81656=CARTESIAN_POINT('Ctrl Pts',(23.0523462283541,-1.13482163901424,3.76585344615452));
#81657=CARTESIAN_POINT('Ctrl Pts',(23.0539409729669,-1.16479896406286,3.75668922929904));
#81658=CARTESIAN_POINT('Ctrl Pts',(23.0555357175798,-1.19464903082042,3.74717262654923));
#81659=CARTESIAN_POINT('Ctrl Pts',(23.0614081637137,-1.30456814120325,3.71212893580567));
#81660=CARTESIAN_POINT('Ctrl Pts',(23.0672806098476,-1.41312802225318,3.67218594282703));
#81661=CARTESIAN_POINT('Ctrl Pts',(23.0731530559815,-1.5198595187809,3.62746689070639));
#81662=CARTESIAN_POINT('Ctrl Pts',(23.0790178949264,-1.62645275492183,3.58280576781606));
#81663=CARTESIAN_POINT('Ctrl Pts',(23.0848827338713,-1.73122193890643,3.53338104764182));
#81664=CARTESIAN_POINT('Ctrl Pts',(23.0907475728161,-1.83371282272411,3.47936578757928));
#81665=CARTESIAN_POINT('Ctrl Pts',(23.0966063829362,-1.93609834992588,3.42540605308931));
#81666=CARTESIAN_POINT('Ctrl Pts',(23.1024651930562,-2.03620987184902,3.36686535641789));
#81667=CARTESIAN_POINT('Ctrl Pts',(23.1083240031762,-2.13361351911859,3.30396464131116));
#81668=CARTESIAN_POINT('Ctrl Pts',(23.1144097920572,-2.23479072428027,3.23862706170743));
#81669=CARTESIAN_POINT('Ctrl Pts',(23.1204955809382,-2.33304557831242,3.16858497991537));
#81670=CARTESIAN_POINT('Ctrl Pts',(23.1265813698191,-2.42792006910148,3.09413851306859));
#81671=CARTESIAN_POINT('Ctrl Pts',(23.1324333998974,-2.51915037377007,3.02255157968484));
#81672=CARTESIAN_POINT('Ctrl Pts',(23.1382854299757,-2.60725485329683,2.94689264884913));
#81673=CARTESIAN_POINT('Ctrl Pts',(23.144137460054,-2.69185690452306,2.867471953755));
#81674=CARTESIAN_POINT('Ctrl Pts',(23.1499886004325,-2.77644609347362,2.78806333320114));
#81675=CARTESIAN_POINT('Ctrl Pts',(23.155839740811,-2.85753361158639,2.70489436837059));
#81676=CARTESIAN_POINT('Ctrl Pts',(23.1616908811895,-2.93477797961284,2.61831381052378));
#81677=CARTESIAN_POINT('Ctrl Pts',(23.1675425487571,-3.01202930737322,2.53172545175037));
#81678=CARTESIAN_POINT('Ctrl Pts',(23.1733942163246,-3.0854365214968,2.44172519736995));
#81679=CARTESIAN_POINT('Ctrl Pts',(23.1792458838921,-3.15469735675409,2.34869614622427));
#81680=CARTESIAN_POINT('Ctrl Pts',(23.1850994955763,-3.22398120274239,2.25563618776331));
#81681=CARTESIAN_POINT('Ctrl Pts',(23.1909531072606,-3.28911568394661,2.15954576302053));
#81682=CARTESIAN_POINT('Ctrl Pts',(23.1968067189448,-3.34984133224644,2.06083770558804));
#81683=CARTESIAN_POINT('Ctrl Pts',(23.2026669850447,-3.4106360137734,1.96201743633174));
#81684=CARTESIAN_POINT('Ctrl Pts',(23.2085272511446,-3.46701164192267,1.86057394718685));
#81685=CARTESIAN_POINT('Ctrl Pts',(23.2143875172445,-3.51875422660916,1.75694555769955));
#81686=CARTESIAN_POINT('Ctrl Pts',(23.2202517304159,-3.57053166153517,1.65324737127));
#81687=CARTESIAN_POINT('Ctrl Pts',(23.2261159435872,-3.61766967175745,1.54736173095373));
#81688=CARTESIAN_POINT('Ctrl Pts',(23.2319801567585,-3.66000270194713,1.43974623518858));
#81689=CARTESIAN_POINT('Ctrl Pts',(23.2378530053328,-3.7023980700438,1.33197226919968));
#81690=CARTESIAN_POINT('Ctrl Pts',(23.2437258539071,-3.73997420292759,1.22246375333706));
#81691=CARTESIAN_POINT('Ctrl Pts',(23.2495987024814,-3.77261555999464,1.11169277972213));
#81692=CARTESIAN_POINT('Ctrl Pts',(23.2511934470941,-3.78147916811835,1.08161343897699));
#81693=CARTESIAN_POINT('Ctrl Pts',(23.2527881917068,-3.78997919380532,1.051441060039));
#81694=CARTESIAN_POINT('Ctrl Pts',(23.2543829363194,-3.79811397947583,1.02118519324866));
#81695=CARTESIAN_POINT('Ctrl Pts',(23.2619216566848,-3.83656896086636,0.8781588319525));
#81696=CARTESIAN_POINT('Ctrl Pts',(23.2694603770502,-3.866962272519,0.73287961600431));
#81697=CARTESIAN_POINT('Ctrl Pts',(23.2769990974156,-3.88907771444612,0.586142927107849));
#81698=CARTESIAN_POINT('Ctrl Pts',(23.2843940960392,-3.9107715370956,0.442203696068143));
#81699=CARTESIAN_POINT('Ctrl Pts',(23.2917890946628,-3.92450013026313,0.296861841860589));
#81700=CARTESIAN_POINT('Ctrl Pts',(23.2991840932864,-3.9301044830118,0.150889869144963));
#81701=CARTESIAN_POINT('Ctrl Pts',(23.3016682155052,-3.93198709285311,0.101855076954787));
#81702=CARTESIAN_POINT('Ctrl Pts',(23.3041523377241,-3.93295333092603,0.0527493780525428));
#81703=CARTESIAN_POINT('Ctrl Pts',(23.3066364599429,-3.93299834994999,0.00360267826161876));
#81704=CARTESIAN_POINT('',(24.5566365102202,-3.9306426375169,-0.00105404585137062));
#81705=CARTESIAN_POINT('Ctrl Pts',(23.3066364779651,-3.93182490893431,0.00360124692383467));
#81706=CARTESIAN_POINT('Ctrl Pts',(23.3555010369964,-3.92319230971691,-0.962871716430977));
#81707=CARTESIAN_POINT('Ctrl Pts',(23.4706480022741,-3.07602472218424,-3.25384824264235));
#81708=CARTESIAN_POINT('Ctrl Pts',(23.6520773737987,0.766703506199793,-4.5880450089923));
#81709=CARTESIAN_POINT('Ctrl Pts',(23.8509245925382,4.27406879625159,-1.83584509037353));
#81710=CARTESIAN_POINT('Ctrl Pts',(24.049771811278,3.85536201618789,2.60272453307588));
#81711=CARTESIAN_POINT('Ctrl Pts',(24.2486190300175,-0.104801360273113,
4.65048470009646));
#81712=CARTESIAN_POINT('Ctrl Pts',(24.4175739189133,-3.38784425822317,2.76074661215668));
#81713=CARTESIAN_POINT('Ctrl Pts',(24.5202464015625,-3.9250314248909,0.721034683795631));
#81714=CARTESIAN_POINT('Ctrl Pts',(24.5566364779651,-3.92675474403147,-0.00105236284854396));
#81715=CARTESIAN_POINT('',(25.8066364779651,-3.9335827204154,-0.00321703522350915));
#81716=CARTESIAN_POINT('Ctrl Pts',(24.5566365297764,-3.932999858484,-0.00105506625215207));
#81717=CARTESIAN_POINT('Ctrl Pts',(24.5629066911867,-3.93296642890169,-0.125671451479569));
#81718=CARTESIAN_POINT('Ctrl Pts',(24.569176852597,-3.92700610699965,-0.250124843395846));
#81719=CARTESIAN_POINT('Ctrl Pts',(24.5754470140074,-3.91519047823295,-0.373861631026793));
#81720=CARTESIAN_POINT('Ctrl Pts',(24.5817404834431,-3.9033309273154,-0.498058384518136));
#81721=CARTESIAN_POINT('Ctrl Pts',(24.5880339528788,-3.88557254366928,-0.621532888384749));
#81722=CARTESIAN_POINT('Ctrl Pts',(24.5943274223145,-3.86203853726118,-0.743738755686087));
#81723=CARTESIAN_POINT('Ctrl Pts',(24.6006327607509,-3.83846014752159,-0.866175093882362));
#81724=CARTESIAN_POINT('Ctrl Pts',(24.6069380991874,-3.80908445827578,-0.987337713059643));
#81725=CARTESIAN_POINT('Ctrl Pts',(24.6132434376239,-3.77408465406791,-1.10669509076761));
#81726=CARTESIAN_POINT('Ctrl Pts',(24.6195683362665,-3.7389762746595,-1.22642273486743));
#81727=CARTESIAN_POINT('Ctrl Pts',(24.6258932349091,-3.69820897668527,-1.34433363505084));
#81728=CARTESIAN_POINT('Ctrl Pts',(24.6322181335517,-3.65200505726233,-1.45991371722112));
#81729=CARTESIAN_POINT('Ctrl Pts',(24.6369165782001,-3.61768252180174,-1.54577226598434));
#81730=CARTESIAN_POINT('Ctrl Pts',(24.6416150228484,-3.58036092298856,-1.63034505658126));
#81731=CARTESIAN_POINT('Ctrl Pts',(24.6463134674968,-3.54014749293069,-1.71343068966812));
#81732=CARTESIAN_POINT('Ctrl Pts',(24.6521859136307,-3.48988592350725,-1.81727694972292));
#81733=CARTESIAN_POINT('Ctrl Pts',(24.6580583597647,-3.43496701066595,-1.91908364632974));
#81734=CARTESIAN_POINT('Ctrl Pts',(24.6639308058986,-3.37557921576622,-2.01840381442542));
#81735=CARTESIAN_POINT('Ctrl Pts',(24.6697956448435,-3.31626835204206,-2.11759532279731));
#81736=CARTESIAN_POINT('Ctrl Pts',(24.6756604837883,-3.25250032871324,-2.21430635669629));
#81737=CARTESIAN_POINT('Ctrl Pts',(24.6815253227332,-3.18451080730261,-2.30811176466238));
#81738=CARTESIAN_POINT('Ctrl Pts',(24.6873841328532,-3.11659117645802,-2.40182074434181));
#81739=CARTESIAN_POINT('Ctrl Pts',(24.6932429429733,-3.04445892022942,-2.49262970645418));
#81740=CARTESIAN_POINT('Ctrl Pts',(24.6991017530933,-2.96839421670032,-2.58014045630468));
#81741=CARTESIAN_POINT('Ctrl Pts',(24.7051875419743,-2.88938265676124,-2.67104149892138));
#81742=CARTESIAN_POINT('Ctrl Pts',(24.7112733308552,-2.80612802284882,-2.75838321572819));
#81743=CARTESIAN_POINT('Ctrl Pts',(24.7173591197362,-2.71899228807735,-2.84175472857457));
#81744=CARTESIAN_POINT('Ctrl Pts',(24.7232111498145,-2.63520348916414,-2.92192389158554));
#81745=CARTESIAN_POINT('Ctrl Pts',(24.7290631798928,-2.54782656671861,-2.99842190823836));
#81746=CARTESIAN_POINT('Ctrl Pts',(24.7349152099711,-2.45722197539512,-3.07091992139738));
#81747=CARTESIAN_POINT('Ctrl Pts',(24.7407663503496,-2.36663115892949,-3.14340691248995));
#81748=CARTESIAN_POINT('Ctrl Pts',(24.7466174907281,-2.27281397194419,-3.21189485106909));
#81749=CARTESIAN_POINT('Ctrl Pts',(24.7524686311066,-2.17616402301271,-3.27609510621184));
#81750=CARTESIAN_POINT('Ctrl Pts',(24.7583202986742,-2.07950536590031,-3.3403011458112));
#81751=CARTESIAN_POINT('Ctrl Pts',(24.7641719662417,-1.9800137838004,-3.40021850527551));
#81752=CARTESIAN_POINT('Ctrl Pts',(24.7700236338092,-1.87811133136837,-3.45560223795878));
#81753=CARTESIAN_POINT('Ctrl Pts',(24.7758772454935,-1.77617502358462,-3.51100437094258));
#81754=CARTESIAN_POINT('Ctrl Pts',(24.7817308571777,-1.67182661577805,-3.56186968483403));
#81755=CARTESIAN_POINT('Ctrl Pts',(24.787584468862,-1.56551153478921,-3.60799981075968));
#81756=CARTESIAN_POINT('Ctrl Pts',(24.7934447349619,-1.45907559427354,-3.654182377648));
#81757=CARTESIAN_POINT('Ctrl Pts',(24.7993050010618,-1.35066889756852,-3.6956188476788));
#81758=CARTESIAN_POINT('Ctrl Pts',(24.8051652671617,-1.24075565796832,-3.73215948175042));
#81759=CARTESIAN_POINT('Ctrl Pts',(24.811029480333,-1.13076838838416,-3.76872472707511));
#81760=CARTESIAN_POINT('Ctrl Pts',(24.8168936935043,-1.01927295208768,-3.80038745781482));
#81761=CARTESIAN_POINT('Ctrl Pts',(24.8227579066756,-0.90674578550836,-3.82704861224192));
#81762=CARTESIAN_POINT('Ctrl Pts',(24.8286307552499,-0.794052915977578,
-3.85374902680604));
#81763=CARTESIAN_POINT('Ctrl Pts',(24.8345036038242,-0.680325688489406,
-3.87543308861966));
#81764=CARTESIAN_POINT('Ctrl Pts',(24.8403764523985,-0.566047801838025,
-3.89205329948529));
#81765=CARTESIAN_POINT('Ctrl Pts',(24.8419711970112,-0.535016175229567,
-3.89656644015361));
#81766=CARTESIAN_POINT('Ctrl Pts',(24.8435659416239,-0.50394395427505,-3.90070648513353));
#81767=CARTESIAN_POINT('Ctrl Pts',(24.8451606862366,-0.472840827816458,
-3.9044731464757));
#81768=CARTESIAN_POINT('Ctrl Pts',(24.8510331323705,-0.358307482933332,
-3.91834340235286));
#81769=CARTESIAN_POINT('Ctrl Pts',(24.8569055785044,-0.242971563730075,
-3.92719304659092));
#81770=CARTESIAN_POINT('Ctrl Pts',(24.8627780246383,-0.127310964188841,
-3.9309389359792));
#81771=CARTESIAN_POINT('Ctrl Pts',(24.8686428635831,-0.0118001918284861,
-3.93467997292811));
#81772=CARTESIAN_POINT('Ctrl Pts',(24.874507702528,0.104034015129978,-3.93333038954029));
#81773=CARTESIAN_POINT('Ctrl Pts',(24.8803725414728,0.219706590890167,-3.92685854264187));
#81774=CARTESIAN_POINT('Ctrl Pts',(24.8862313515928,0.33526025977114,-3.92039334854868));
#81775=CARTESIAN_POINT('Ctrl Pts',(24.8920901617129,0.450652217702628,-3.90881638723821));
#81776=CARTESIAN_POINT('Ctrl Pts',(24.8979489718329,0.565396004599239,-3.89214803906316));
#81777=CARTESIAN_POINT('Ctrl Pts',(24.9040347607139,0.684585131427196,-3.87483393501988));
#81778=CARTESIAN_POINT('Ctrl Pts',(24.9101205495948,0.803074395198658,-3.85202595541681));
#81779=CARTESIAN_POINT('Ctrl Pts',(24.9162063384758,0.920322438981543,-3.82380642924129));
#81780=CARTESIAN_POINT('Ctrl Pts',(24.9220583685541,1.03306691504787,-3.79667083199935));
#81781=CARTESIAN_POINT('Ctrl Pts',(24.9279103986323,1.14466332520609,-3.76453184683155));
#81782=CARTESIAN_POINT('Ctrl Pts',(24.9337624287106,1.25464013037985,-3.7275148749858));
#81783=CARTESIAN_POINT('Ctrl Pts',(24.9396135690891,1.36460021548638,-3.69050353092909));
#81784=CARTESIAN_POINT('Ctrl Pts',(24.9454647094676,1.47294079354598,-3.6486158065898));
#81785=CARTESIAN_POINT('Ctrl Pts',(24.9513158498461,1.57920623746743,-3.60202674331326));
#81786=CARTESIAN_POINT('Ctrl Pts',(24.9571675174136,1.68548125592786,-3.55543348235227));
#81787=CARTESIAN_POINT('Ctrl Pts',(24.9630191849811,1.78968038997646,-3.50413820637703));
#81788=CARTESIAN_POINT('Ctrl Pts',(24.9688708525486,1.89136937903747,-3.44836350636637));
#81789=CARTESIAN_POINT('Ctrl Pts',(24.9747244642329,1.9930921525307,-3.39257027616293));
#81790=CARTESIAN_POINT('Ctrl Pts',(24.9805780759171,2.09230276054195,-3.33229486138188));
#81791=CARTESIAN_POINT('Ctrl Pts',(24.9864316876013,2.1885934865531,-3.26780469897106));
#81792=CARTESIAN_POINT('Ctrl Pts',(24.9922919537012,2.28499367635317,-3.20324122381437));
#81793=CARTESIAN_POINT('Ctrl Pts',(24.9981522198011,2.37846701521994,-3.13445366781653));
#81794=CARTESIAN_POINT('Ctrl Pts',(25.004012485901,2.46863653640493,-3.06175156587315));
#81795=CARTESIAN_POINT('Ctrl Pts',(25.0098766990723,2.55886678956589,-2.98900049680374));
#81796=CARTESIAN_POINT('Ctrl Pts',(25.0157409122436,2.64578848494008,-2.91232990461799));
#81797=CARTESIAN_POINT('Ctrl Pts',(25.0216051254149,2.72906067686341,-2.83208700819693));
#81798=CARTESIAN_POINT('Ctrl Pts',(25.0274779739892,2.81245549204637,-2.75172594933419));
#81799=CARTESIAN_POINT('Ctrl Pts',(25.0333508225635,2.89218979451776,-2.66778238604164));
#81800=CARTESIAN_POINT('Ctrl Pts',(25.0392236711378,2.9679620874797,-2.58063752729497));
#81801=CARTESIAN_POINT('Ctrl Pts',(25.0408184157506,2.98853769988835,-2.55697374774065));
#81802=CARTESIAN_POINT('Ctrl Pts',(25.0424131603633,3.00882141065661,-2.5330740832016));
#81803=CARTESIAN_POINT('Ctrl Pts',(25.0440079049761,3.02880773870287,-2.50894652832092));
#81804=CARTESIAN_POINT('Ctrl Pts',(25.04988035111,3.10240487389666,-2.42009984701261));
#81805=CARTESIAN_POINT('Ctrl Pts',(25.055752797244,3.17221258597784,-2.32786333691163));
#81806=CARTESIAN_POINT('Ctrl Pts',(25.0616252433779,3.23790253196703,-2.23259405031042));
#81807=CARTESIAN_POINT('Ctrl Pts',(25.0674900823227,3.30350738295017,-2.13744817590568));
#81808=CARTESIAN_POINT('Ctrl Pts',(25.0733549212676,3.36500484312648,-2.0392776748939));
#81809=CARTESIAN_POINT('Ctrl Pts',(25.0792197602124,3.42210601393322,-1.93847347915882));
#81810=CARTESIAN_POINT('Ctrl Pts',(25.0850785703324,3.47914848697196,-1.83777290619033));
#81811=CARTESIAN_POINT('Ctrl Pts',(25.0909373804525,3.53180345709436,-1.73444438103925));
#81812=CARTESIAN_POINT('Ctrl Pts',(25.0967961905725,3.57982503448564,-1.62890813813115));
#81813=CARTESIAN_POINT('Ctrl Pts',(25.1028819794535,3.62970703710172,-1.51928326883669));
#81814=CARTESIAN_POINT('Ctrl Pts',(25.1089677683344,3.67458911950307,-1.40727653581594));
#81815=CARTESIAN_POINT('Ctrl Pts',(25.1150535572154,3.71424782033151,-1.29338784947233));
#81816=CARTESIAN_POINT('Ctrl Pts',(25.1209055872937,3.7523832066639,-1.18387369591013));
#81817=CARTESIAN_POINT('Ctrl Pts',(25.126757617372,3.7856889274804,-1.07261992254162));
#81818=CARTESIAN_POINT('Ctrl Pts',(25.1326096474502,3.81401550542179,-0.960090997979949));
#81819=CARTESIAN_POINT('Ctrl Pts',(25.1384607878287,3.84233777679793,-0.847579181491054));
#81820=CARTESIAN_POINT('Ctrl Pts',(25.1443119282073,3.86568230956893,-0.733793000017495));
#81821=CARTESIAN_POINT('Ctrl Pts',(25.1501630685858,3.88394998784131,-0.619210377777634));
#81822=CARTESIAN_POINT('Ctrl Pts',(25.1560147361533,3.90221931203536,-0.504617431619288));
#81823=CARTESIAN_POINT('Ctrl Pts',(25.1618664037208,3.91541080732815,-0.389228310269791));
#81824=CARTESIAN_POINT('Ctrl Pts',(25.1677180712883,3.92347691009548,-0.273528674817936));
#81825=CARTESIAN_POINT('Ctrl Pts',(25.1735716829725,3.93154569268787,-0.157790600135666));
#81826=CARTESIAN_POINT('Ctrl Pts',(25.1794252946568,3.93448566806009,-0.0417422183555004));
#81827=CARTESIAN_POINT('Ctrl Pts',(25.185278906341,3.93230135006062,0.0741288898570414));
#81828=CARTESIAN_POINT('Ctrl Pts',(25.1911391724409,3.93011454891729,0.190131720937063));
#81829=CARTESIAN_POINT('Ctrl Pts',(25.1969994385408,3.92279183504807,0.305956462683684));
#81830=CARTESIAN_POINT('Ctrl Pts',(25.2028597046407,3.91038976218568,0.421118638620297));
#81831=CARTESIAN_POINT('Ctrl Pts',(25.208723917812,3.89797933614163,0.536358379862815));
#81832=CARTESIAN_POINT('Ctrl Pts',(25.2145881309833,3.88048280124066,0.650934259083974));
#81833=CARTESIAN_POINT('Ctrl Pts',(25.2204523441546,3.85800788828905,0.764371724947675));
#81834=CARTESIAN_POINT('Ctrl Pts',(25.2263251927289,3.8354998796902,0.877976234232687));
#81835=CARTESIAN_POINT('Ctrl Pts',(25.2321980413032,3.80799895972618,0.990438584421596));
#81836=CARTESIAN_POINT('Ctrl Pts',(25.2380708898775,3.77566278237978,1.10129903012404));
#81837=CARTESIAN_POINT('Ctrl Pts',(25.2396656344903,3.76688204438392,1.13140266659876));
#81838=CARTESIAN_POINT('Ctrl Pts',(25.241260379103,3.75774504363042,1.16138829823806));
#81839=CARTESIAN_POINT('Ctrl Pts',(25.2428551237158,3.74825554160734,1.19124699152184));
#81840=CARTESIAN_POINT('Ctrl Pts',(25.2487275698497,3.71331164587487,1.30119786800404));
#81841=CARTESIAN_POINT('Ctrl Pts',(25.2546000159836,3.67346721606696,1.40979396312183));
#81842=CARTESIAN_POINT('Ctrl Pts',(25.2604724621175,3.62884506934392,1.51656601000362));
#81843=CARTESIAN_POINT('Ctrl Pts',(25.2663373010624,3.58428072631959,1.62319974396949));
#81844=CARTESIAN_POINT('Ctrl Pts',(25.2722021400072,3.53495113216584,1.72801375075103));
#81845=CARTESIAN_POINT('Ctrl Pts',(25.278066978952,3.48102893185714,1.83055362542962));
#81846=CARTESIAN_POINT('Ctrl Pts',(25.283925789072,3.42716216145924,1.93298809313159));
#81847=CARTESIAN_POINT('Ctrl Pts',(25.289784599192,3.36871236650804,2.03315271492282));
#81848=CARTESIAN_POINT('Ctrl Pts',(25.2956434093121,3.3059000968078,2.13061342104244));
#81849=CARTESIAN_POINT('Ctrl Pts',(25.301729198193,3.2406543891129,2.23184989559695));
#81850=CARTESIAN_POINT('Ctrl Pts',(25.307814987074,3.17070152836388,2.33016829080207));
#81851=CARTESIAN_POINT('Ctrl Pts',(25.313900775955,3.09634121580394,2.42511032229747));
#81852=CARTESIAN_POINT('Ctrl Pts',(25.3197528060332,3.02483712746957,2.51640557339288));
#81853=CARTESIAN_POINT('Ctrl Pts',(25.3256048361115,2.94925820585057,2.60457869704562));
#81854=CARTESIAN_POINT('Ctrl Pts',(25.3314568661898,2.86991434214601,2.68925280863377));
#81855=CARTESIAN_POINT('Ctrl Pts',(25.3373080065683,2.79058254130082,2.77391404699073));
#81856=CARTESIAN_POINT('Ctrl Pts',(25.3431591469468,2.70748721903882,2.85507702945651));
#81857=CARTESIAN_POINT('Ctrl Pts',(25.3490102873253,2.62097681649429,2.93239996033956));
#81858=CARTESIAN_POINT('Ctrl Pts',(25.3548619548928,2.53445861934421,3.00972985803502));
#81859=CARTESIAN_POINT('Ctrl Pts',(25.3607136224603,2.44452503844631,3.08321874087236));
#81860=CARTESIAN_POINT('Ctrl Pts',(25.3665652900278,2.3515588980991,3.15256399598342));
#81861=CARTESIAN_POINT('Ctrl Pts',(25.372418901712,2.25856187133742,3.22193228987271));
#81862=CARTESIAN_POINT('Ctrl Pts',(25.3782725133962,2.16253061290004,3.28715397163468));
#81863=CARTESIAN_POINT('Ctrl Pts',(25.3841261250804,2.06387772067324,3.34796919850058));
#81864=CARTESIAN_POINT('Ctrl Pts',(25.3899863911803,1.96511267933486,3.40885356042689));
#81865=CARTESIAN_POINT('Ctrl Pts',(25.3958466572802,1.86372040773272,3.46532125205994));
#81866=CARTESIAN_POINT('Ctrl Pts',(25.4017069233801,1.76013903097998,3.51715788551223));
#81867=CARTESIAN_POINT('Ctrl Pts',(25.4075711365514,1.65648788894963,3.56902943254877));
#81868=CARTESIAN_POINT('Ctrl Pts',(25.4134353497227,1.55064508243277,3.61626354248425));
#81869=CARTESIAN_POINT('Ctrl Pts',(25.419299562894,1.44306805939358,3.65869424466681));
#81870=CARTESIAN_POINT('Ctrl Pts',(25.4251724114682,1.33533262278401,3.70118742858419));
#81871=CARTESIAN_POINT('Ctrl Pts',(25.4310452600425,1.22585826228886,3.73886295383567));
#81872=CARTESIAN_POINT('Ctrl Pts',(25.4369181086168,1.1151169649515,3.77160485131692));
#81873=CARTESIAN_POINT('Ctrl Pts',(25.4385128532297,1.08504568265685,3.78049576072195));
#81874=CARTESIAN_POINT('Ctrl Pts',(25.4401075978425,1.05488103216075,3.78902317229664));
#81875=CARTESIAN_POINT('Ctrl Pts',(25.4417023424554,1.02463256229506,3.79718541979249));
#81876=CARTESIAN_POINT('Ctrl Pts',(25.4475747885893,0.913246382660954,3.82724186793112));
#81877=CARTESIAN_POINT('Ctrl Pts',(25.4534472347232,0.800350088235134,3.85244339896585));
#81878=CARTESIAN_POINT('Ctrl Pts',(25.4593196808571,0.686404838989232,3.87263959038434));
#81879=CARTESIAN_POINT('Ctrl Pts',(25.465184519802,0.572607194852999,3.89280961957957));
#81880=CARTESIAN_POINT('Ctrl Pts',(25.4710493587468,0.457763701367477,3.90798713192554));
#81881=CARTESIAN_POINT('Ctrl Pts',(25.4769141976916,0.342349958906268,3.91807165652147));
#81882=CARTESIAN_POINT('Ctrl Pts',(25.4827730078117,0.227054857253721,3.92814581462094));
#81883=CARTESIAN_POINT('Ctrl Pts',(25.4886318179317,0.111191081912517,3.93313736268711));
#81884=CARTESIAN_POINT('Ctrl Pts',(25.4944906280517,-0.004756970227735,
3.93299712321713));
#81885=CARTESIAN_POINT('Ctrl Pts',(25.5005764169327,-0.125197017273399,
3.93285145066766));
#81886=CARTESIAN_POINT('Ctrl Pts',(25.5066622058136,-0.245727555812056,
3.92716824362582));
#81887=CARTESIAN_POINT('Ctrl Pts',(25.5127479946946,-0.365801021423707,
3.9159518144029));
#81888=CARTESIAN_POINT('Ctrl Pts',(25.5186000247729,-0.481262393170798,
3.90516621495688));
#81889=CARTESIAN_POINT('Ctrl Pts',(25.5244520548511,-0.596300707562093,
3.88926466315186));
#81890=CARTESIAN_POINT('Ctrl Pts',(25.5303040849294,-0.710431364549665,
3.86830405685283));
#81891=CARTESIAN_POINT('Ctrl Pts',(25.5361552253079,-0.824544669948839,
3.84734663725073));
#81892=CARTESIAN_POINT('Ctrl Pts',(25.5420063656864,-0.937750185873964,
3.82133176710452));
#81893=CARTESIAN_POINT('Ctrl Pts',(25.5478575060649,-1.04957198505342,3.7903677457723));
#81894=CARTESIAN_POINT('Ctrl Pts',(25.5537091736324,-1.16140385940057,3.75940093457524));
#81895=CARTESIAN_POINT('Ctrl Pts',(25.5595608411999,-1.271851370773,3.72348419606158));
#81896=CARTESIAN_POINT('Ctrl Pts',(25.5654125087674,-1.38045296151046,3.68277593956746));
#81897=CARTESIAN_POINT('Ctrl Pts',(25.5712661204516,-1.48909063327404,3.64205415844948));
#81898=CARTESIAN_POINT('Ctrl Pts',(25.5771197321358,-1.59588077808782,3.59653783896309));
#81899=CARTESIAN_POINT('Ctrl Pts',(25.5829733438201,-1.70038171799668,3.54643356248255));
#81900=CARTESIAN_POINT('Ctrl Pts',(25.58883360992,-1.80500145510774,3.49627232720461));
#81901=CARTESIAN_POINT('Ctrl Pts',(25.5946938760198,-1.90732642010164,3.44151290355854));
#81902=CARTESIAN_POINT('Ctrl Pts',(25.6005541421197,-2.00693936924165,3.38240792456911));
#81903=CARTESIAN_POINT('Ctrl Pts',(25.606418355291,-2.10661941079979,3.3232631365388));
#81904=CARTESIAN_POINT('Ctrl Pts',(25.6122825684623,-2.20358345435853,3.25976719108145));
#81905=CARTESIAN_POINT('Ctrl Pts',(25.6181467816336,-2.2974445371279,3.19221515547138));
#81906=CARTESIAN_POINT('Ctrl Pts',(25.6240196302079,-2.39144383592908,3.12456364546759));
#81907=CARTESIAN_POINT('Ctrl Pts',(25.6298924787822,-2.48233073126536,3.0528443798206));
#81908=CARTESIAN_POINT('Ctrl Pts',(25.6357653273565,-2.56975246066532,2.97739169255652));
#81909=CARTESIAN_POINT('Ctrl Pts',(25.6373600719693,-2.59349142315416,2.956902867582));
#81910=CARTESIAN_POINT('Ctrl Pts',(25.6389548165822,-2.61697509317041,2.93613895344535));
#81911=CARTESIAN_POINT('Ctrl Pts',(25.640549561195,-2.64019690589979,2.9151070817514));
#81912=CARTESIAN_POINT('Ctrl Pts',(25.6463343613492,-2.72443205225064,2.83881575984568));
#81913=CARTESIAN_POINT('Ctrl Pts',(25.6521191615033,-2.80551894687543,2.7587239653442));
#81914=CARTESIAN_POINT('Ctrl Pts',(25.6579039616575,-2.88308709437247,2.67512575522402));
#81915=CARTESIAN_POINT('Ctrl Pts',(25.6636811997646,-2.96055384269176,2.59163682694235));
#81916=CARTESIAN_POINT('Ctrl Pts',(25.6694584378717,-3.03451069836479,2.50465090261323));
#81917=CARTESIAN_POINT('Ctrl Pts',(25.6752356759788,-3.10462086965447,2.41450165783872));
#81918=CARTESIAN_POINT('Ctrl Pts',(25.6810063285583,-3.17465112170482,2.32445517503063));
#81919=CARTESIAN_POINT('Ctrl Pts',(25.6867769811377,-3.24084315136317,2.23125287937215));
#81920=CARTESIAN_POINT('Ctrl Pts',(25.6925476337171,-3.30289833132539,2.13526382747612));
#81921=CARTESIAN_POINT('Ctrl Pts',(25.6983146496206,-3.36491440399852,2.03933526805798));
#81922=CARTESIAN_POINT('Ctrl Pts',(25.7040816655241,-3.42279857562265,1.94062379863746));
#81923=CARTESIAN_POINT('Ctrl Pts',(25.7098486814276,-3.47629402636826,1.83952951654394));
#81924=CARTESIAN_POINT('Ctrl Pts',(25.715613556132,-3.52976961512355,1.73847276911222));
#81925=CARTESIAN_POINT('Ctrl Pts',(25.7213784308363,-3.57885952230643,1.63503534409878));
#81926=CARTESIAN_POINT('Ctrl Pts',(25.7271433055407,-3.62335206581951,1.52964335945392));
#81927=CARTESIAN_POINT('Ctrl Pts',(25.7329075322382,-3.66783960810145,1.42426322150593));
#81928=CARTESIAN_POINT('Ctrl Pts',(25.7386717589358,-3.70773064965458,1.31692935439913));
#81929=CARTESIAN_POINT('Ctrl Pts',(25.7444359856333,-3.7428613571943,1.20808851530905));
#81930=CARTESIAN_POINT('Ctrl Pts',(25.7502036269295,-3.7780128753776,1.09918320134592));
#81931=CARTESIAN_POINT('Ctrl Pts',(25.7559712682257,-3.80839829491612,0.988769538700377));
#81932=CARTESIAN_POINT('Ctrl Pts',(25.7617389095219,-3.83390354286085,0.877309879141372));
#81933=CARTESIAN_POINT('Ctrl Pts',(25.7675083756034,-3.85941686023952,0.765814955609947));
#81934=CARTESIAN_POINT('Ctrl Pts',(25.7732778416849,-3.88004685222984,0.65327379560468));
#81935=CARTESIAN_POINT('Ctrl Pts',(25.7790473077664,-3.89573081843034,0.540157745785523));
#81936=CARTESIAN_POINT('Ctrl Pts',(25.7848234966307,-3.9114330601346,0.426909889204726));
#81937=CARTESIAN_POINT('Ctrl Pts',(25.790599685495,-3.9221777268169,0.313086229874658));
#81938=CARTESIAN_POINT('Ctrl Pts',(25.7963758743593,-3.92795411346371,0.1991619504914));
#81939=CARTESIAN_POINT('Ctrl Pts',(25.7997960755613,-3.93137443177674,0.131705022328782));
#81940=CARTESIAN_POINT('Ctrl Pts',(25.8032162767632,-3.93305383103106,0.0642128260551774));
#81941=CARTESIAN_POINT('Ctrl Pts',(25.8066364779651,-3.93299868468798,-0.00321655757663048));
#81942=CARTESIAN_POINT('',(27.0566364779651,-3.93435343806616,0.00262747460303034));
#81943=CARTESIAN_POINT('Ctrl Pts',(25.8066364779651,-3.93569742829264,-0.00321876471293834));
#81944=CARTESIAN_POINT('Ctrl Pts',(25.8175565786217,-3.93760386311818,-0.218658353487745));
#81945=CARTESIAN_POINT('Ctrl Pts',(25.8947590855247,-3.82336855807856,-1.73974115160522));
#81946=CARTESIAN_POINT('Ctrl Pts',(26.0382439986743,-1.83972417824563,-4.27240052182587));
#81947=CARTESIAN_POINT('Ctrl Pts',(26.237091217414,2.59922370323215,-3.85772308642246));
#81948=CARTESIAN_POINT('Ctrl Pts',(26.4359384361537,4.65057791887957,0.100579776150997));
#81949=CARTESIAN_POINT('Ctrl Pts',(26.6347856548932,2.43000649467348,3.9664921160622));
#81950=CARTESIAN_POINT('Ctrl Pts',(26.8336328736329,-2.02271913287657,4.18886602560103));
#81951=CARTESIAN_POINT('Ctrl Pts',(26.9742498146569,-3.85758709369341,1.62510249400492));
#81952=CARTESIAN_POINT('Ctrl Pts',(27.0485843494343,-3.93845870985197,0.161325734877928));
#81953=CARTESIAN_POINT('Ctrl Pts',(27.0566364779651,-3.93723842550275,0.00262940128077819));
#81954=CARTESIAN_POINT('',(28.3066364508351,-3.93096447206993,0.00191346378281269));
#81955=CARTESIAN_POINT('Ctrl Pts',(27.0566364779651,-3.93299912295048,0.00262657015236832));
#81956=CARTESIAN_POINT('Ctrl Pts',(27.0624230850425,-3.93307520374763,-0.111296032760114));
#81957=CARTESIAN_POINT('Ctrl Pts',(27.0682096921198,-3.92819730815862,-0.225413803237607));
#81958=CARTESIAN_POINT('Ctrl Pts',(27.0739962991972,-3.91834103977739,-0.339252849650841));
#81959=CARTESIAN_POINT('Ctrl Pts',(27.0797763934189,-3.90849586467629,-0.452963769639129));
#81960=CARTESIAN_POINT('Ctrl Pts',(27.0855564876406,-3.89368349056366,-0.566396168206476));
#81961=CARTESIAN_POINT('Ctrl Pts',(27.0913365818623,-3.87393154667742,-0.679075379952401));
#81962=CARTESIAN_POINT('Ctrl Pts',(27.0971695289144,-3.85399899221638,-0.792784923564359));
#81963=CARTESIAN_POINT('Ctrl Pts',(27.1030024759665,-3.82903606102631,-0.905726996853392));
#81964=CARTESIAN_POINT('Ctrl Pts',(27.1088354230185,-3.79912486104711,-1.01741795255133));
#81965=CARTESIAN_POINT('Ctrl Pts',(27.1146079286819,-3.76952360292889,-1.12795155907285));
#81966=CARTESIAN_POINT('Ctrl Pts',(27.1203804343453,-3.73507626101903,-1.23725943527664));
#81967=CARTESIAN_POINT('Ctrl Pts',(27.1261529400087,-3.6959137047072,-1.3448832244316));
#81968=CARTESIAN_POINT('Ctrl Pts',(27.1319242944339,-3.65675895876952,-1.45248554966436));
#81969=CARTESIAN_POINT('Ctrl Pts',(27.1376956488591,-3.61289101273658,-1.55840405530356));
#81970=CARTESIAN_POINT('Ctrl Pts',(27.1434670032844,-3.56449006855692,-1.66219720585709));
#81971=CARTESIAN_POINT('Ctrl Pts',(27.1492386945002,-3.5160862999131,-1.76599641331795));
#81972=CARTESIAN_POINT('Ctrl Pts',(27.1550103857161,-3.46314918823332,-1.86766963364983));
#81973=CARTESIAN_POINT('Ctrl Pts',(27.1607820769319,-3.40590600456802,-1.96679772423285));
#81974=CARTESIAN_POINT('Ctrl Pts',(27.1666608464469,-3.34760082667656,-2.0677648715054));
#81975=CARTESIAN_POINT('Ctrl Pts',(27.172539615962,-3.28482842684045,-2.1660911070396));
#81976=CARTESIAN_POINT('Ctrl Pts',(27.178418385477,-3.21787575663264,-2.26136344157146));
#81977=CARTESIAN_POINT('Ctrl Pts',(27.1841983330029,-3.1520485593716,-2.35503425020812));
#81978=CARTESIAN_POINT('Ctrl Pts',(27.1899782805287,-3.0821808544064,-2.44575273197191));
#81979=CARTESIAN_POINT('Ctrl Pts',(27.1957582280546,-3.00858593618571,-2.53316001559032));
#81980=CARTESIAN_POINT('Ctrl Pts',(27.2016864085642,-2.93310359696907,-2.62280895320181));
#81981=CARTESIAN_POINT('Ctrl Pts',(27.2076145890738,-2.85370060363789,-2.70897419680968));
#81982=CARTESIAN_POINT('Ctrl Pts',(27.2135427695834,-2.77075394578029,-2.79131001000301));
#81983=CARTESIAN_POINT('Ctrl Pts',(27.219470950093,-2.68780728792268,-2.87364582319633));
#81984=CARTESIAN_POINT('Ctrl Pts',(27.2253991306026,-2.60131736618754,-2.95215194076755));
#81985=CARTESIAN_POINT('Ctrl Pts',(27.2313273111122,-2.51169493614476,-3.02652896033472));
#81986=CARTESIAN_POINT('Ctrl Pts',(27.2371997572461,-2.4229151002466,-3.10020671699247));
#81987=CARTESIAN_POINT('Ctrl Pts',(27.24307220338,-2.3307419970519,-3.17009812926226));
#81988=CARTESIAN_POINT('Ctrl Pts',(27.2489446495139,-2.23553238064819,-3.2358745301809));
#81989=CARTESIAN_POINT('Ctrl Pts',(27.2548094884588,-2.14044609914401,-3.30156572409939));
#81990=CARTESIAN_POINT('Ctrl Pts',(27.2606743274036,-2.04233146373895,-3.36315227454946));
#81991=CARTESIAN_POINT('Ctrl Pts',(27.2665391663485,-1.94157914390406,-3.42034492821364));
#81992=CARTESIAN_POINT('Ctrl Pts',(27.2723979764685,-1.84093039350915,-3.47747879006915));
#81993=CARTESIAN_POINT('Ctrl Pts',(27.2782567865885,-1.73764970919876,-3.53022753637549));
#81994=CARTESIAN_POINT('Ctrl Pts',(27.2841155967086,-1.6321571020155,-3.57834489594566));
#81995=CARTESIAN_POINT('Ctrl Pts',(27.2902013855895,-1.52257755895691,-3.62832639148047));
#81996=CARTESIAN_POINT('Ctrl Pts',(27.2962871744705,-1.4106116144076,-3.6733101310299));
#81997=CARTESIAN_POINT('Ctrl Pts',(27.3023729633515,-1.29675897571493,-3.71307219952734));
#81998=CARTESIAN_POINT('Ctrl Pts',(27.3082249934298,-1.18727948519185,-3.75130698311451));
#81999=CARTESIAN_POINT('Ctrl Pts',(27.314077023508,-1.07605599138446,-3.78471368233932));
#82000=CARTESIAN_POINT('Ctrl Pts',(27.3199290535863,-0.963552827024398,
-3.81314239827643));
#82001=CARTESIAN_POINT('Ctrl Pts',(27.3257801939648,-0.851066766820581,
-3.84156679212));
#82002=CARTESIAN_POINT('Ctrl Pts',(27.3316313343433,-0.737301823547027,
-3.86501460623153));
#82003=CARTESIAN_POINT('Ctrl Pts',(27.3374824747218,-0.622735831251369,
-3.88338629091617));
#82004=CARTESIAN_POINT('Ctrl Pts',(27.3433341422893,-0.508159516535937,
-3.90175963089343));
#82005=CARTESIAN_POINT('Ctrl Pts',(27.3491858098568,-0.392782417488927,
-3.9150558668005));
#82006=CARTESIAN_POINT('Ctrl Pts',(27.3550374774243,-0.277090151822499,
-3.9232269941673));
#82007=CARTESIAN_POINT('Ctrl Pts',(27.3608910891085,-0.161359449374253,
-3.93140083625178));
#82008=CARTESIAN_POINT('Ctrl Pts',(27.3667447007928,-0.0453137842112288,
-3.9344461549148));
#82009=CARTESIAN_POINT('Ctrl Pts',(27.372598312477,0.0705592591044405,-3.93236702139496));
#82010=CARTESIAN_POINT('Ctrl Pts',(27.3784585785769,0.186564027487612,-3.9302855243055));
#82011=CARTESIAN_POINT('Ctrl Pts',(27.3843188446767,0.302395368805617,-3.92306795494325));
#82012=CARTESIAN_POINT('Ctrl Pts',(27.3901791107766,0.417568755444039,-3.91077042722747));
#82013=CARTESIAN_POINT('Ctrl Pts',(27.3960433239479,0.532819714939232,-3.89846461674443));
#82014=CARTESIAN_POINT('Ctrl Pts',(27.4019075371192,0.64741142967131,-3.88107209687023));
#82015=CARTESIAN_POINT('Ctrl Pts',(27.4077717502905,0.760869250705581,-3.85870016758632));
#82016=CARTESIAN_POINT('Ctrl Pts',(27.4136445988648,0.874494145135491,-3.83629529430474));
#82017=CARTESIAN_POINT('Ctrl Pts',(27.4195174474391,0.986981413323301,-3.80889647490465));
#82018=CARTESIAN_POINT('Ctrl Pts',(27.4253902960134,1.09787116695553,-3.77666094596374));
#82019=CARTESIAN_POINT('Ctrl Pts',(27.4269850406262,1.12798276186274,-3.76790753857221));
#82020=CARTESIAN_POINT('Ctrl Pts',(27.4285797852391,1.15797667538553,-3.75879776144932));
#82021=CARTESIAN_POINT('Ctrl Pts',(27.4301745298519,1.18784397059293,-3.74933536797204));
#82022=CARTESIAN_POINT('Ctrl Pts',(27.4360469759858,1.29782652257194,-3.7144912960454));
#82023=CARTESIAN_POINT('Ctrl Pts',(27.4419194221197,1.40645874227142,-3.67474546224114));
#82024=CARTESIAN_POINT('Ctrl Pts',(27.4477918682536,1.51327125152412,-3.63022025768556));
#82025=CARTESIAN_POINT('Ctrl Pts',(27.4536567071985,1.61994539544582,-3.58575273124942));
#82026=CARTESIAN_POINT('Ctrl Pts',(27.4595215461433,1.72480413865467,-3.53651830376502));
#82027=CARTESIAN_POINT('Ctrl Pts',(27.4653863850882,1.82739291969843,-3.48268920764343));
#82028=CARTESIAN_POINT('Ctrl Pts',(27.4712451952082,1.92987624349184,-3.42891544572514));
#82029=CARTESIAN_POINT('Ctrl Pts',(27.4771040053283,2.03009388261276,-3.3705566006582));
#82030=CARTESIAN_POINT('Ctrl Pts',(27.4829628154483,2.1276115672721,-3.30783282812326));
#82031=CARTESIAN_POINT('Ctrl Pts',(27.4890486043293,2.22890722779675,-3.24267904610188));
#82032=CARTESIAN_POINT('Ctrl Pts',(27.4951343932102,2.32728908315672,-3.17281546403948));
#82033=CARTESIAN_POINT('Ctrl Pts',(27.5012201820912,2.42229857712262,-3.09854136704187));
#82034=CARTESIAN_POINT('Ctrl Pts',(27.5070722121695,2.51365869941481,-3.02712018267815));
#82035=CARTESIAN_POINT('Ctrl Pts',(27.5129242422478,2.60190039453619,-2.95162133255492));
#82036=CARTESIAN_POINT('Ctrl Pts',(27.518776272326,2.68664649671219,-2.87235436562137));
#82037=CARTESIAN_POINT('Ctrl Pts',(27.5246274127046,2.7713797147121,-2.79309944985634));
#82038=CARTESIAN_POINT('Ctrl Pts',(27.5304785530831,2.85261809465008,-2.71007783863559));
#82039=CARTESIAN_POINT('Ctrl Pts',(27.5363296934616,2.93001952467321,-2.62363766268015));
#82040=CARTESIAN_POINT('Ctrl Pts',(27.5421813610291,3.00742792858161,-2.53718969844651));
#82041=CARTESIAN_POINT('Ctrl Pts',(27.5480330285966,3.08099841957563,-2.44732286513857));
#82042=CARTESIAN_POINT('Ctrl Pts',(27.5538846961641,3.1504280373978,-2.35441971219616));
#82043=CARTESIAN_POINT('Ctrl Pts',(27.5597383078484,3.21988072202623,-2.26148569376584));
#82044=CARTESIAN_POINT('Ctrl Pts',(27.5655919195326,3.28518955060098,-2.16551368076623));
#82045=CARTESIAN_POINT('Ctrl Pts',(27.5714455312169,3.34609430591902,-2.06691603503778));
#82046=CARTESIAN_POINT('Ctrl Pts',(27.5773057973168,3.40706829807387,-1.96820630300226));
#82047=CARTESIAN_POINT('Ctrl Pts',(27.5831660634167,3.46362800665929,-1.86686533249271));
#82048=CARTESIAN_POINT('Ctrl Pts',(27.5890263295166,3.51555864616209,-1.76333105382824));
#82049=CARTESIAN_POINT('Ctrl Pts',(27.5948905426879,3.56752426256507,-1.65972704160829));
#82050=CARTESIAN_POINT('Ctrl Pts',(27.6007547558592,3.61485443329103,-1.55392715610801));
#82051=CARTESIAN_POINT('Ctrl Pts',(27.6066189690305,3.65738277250184,-1.446388694441));
#82052=CARTESIAN_POINT('Ctrl Pts',(27.6124918176048,3.69997373722392,-1.33869187598726));
#82053=CARTESIAN_POINT('Ctrl Pts',(27.6183646661791,3.73774862379689,-1.229251761069));
#82054=CARTESIAN_POINT('Ctrl Pts',(27.6242375147534,3.77059103471154,-1.11854023126259));
#82055=CARTESIAN_POINT('Ctrl Pts',(27.6258322593661,3.77950923806932,-1.0884770322048));
#82056=CARTESIAN_POINT('Ctrl Pts',(27.6274270039788,3.78806402850286,-1.05832013501393));
#82057=CARTESIAN_POINT('Ctrl Pts',(27.6290217485916,3.79625373109626,-1.02807908700534));
#82058=CARTESIAN_POINT('Ctrl Pts',(27.6348941947255,3.82641127917549,-0.916720237415284));
#82059=CARTESIAN_POINT('Ctrl Pts',(27.6407666408594,3.85171528297846,-0.803846866538452));
#82060=CARTESIAN_POINT('Ctrl Pts',(27.6466390869933,3.87201490143052,-0.689919997608392));
#82061=CARTESIAN_POINT('Ctrl Pts',(27.6525039259381,3.89228822367954,-0.576140709978197));
#82062=CARTESIAN_POINT('Ctrl Pts',(27.6583687648829,3.90756998052033,-0.461311041404331));
#82063=CARTESIAN_POINT('Ctrl Pts',(27.6642336038278,3.91775926936079,-0.345906500860604));
#82064=CARTESIAN_POINT('Ctrl Pts',(27.6700924139478,3.92793808401126,-0.230620591666161));
#82065=CARTESIAN_POINT('Ctrl Pts',(27.6759512240678,3.93303480694386,-0.114761395208751));
#82066=CARTESIAN_POINT('Ctrl Pts',(27.6818100341878,3.93299982095811,0.00118673646314422));
#82067=CARTESIAN_POINT('Ctrl Pts',(27.6878958230688,3.93296347956478,0.121626866121606));
#82068=CARTESIAN_POINT('Ctrl Pts',(27.6939816119497,3.92738968810554,0.24216251400827));
#82069=CARTESIAN_POINT('Ctrl Pts',(27.7000674008307,3.9162822618308,0.362246112014192));
#82070=CARTESIAN_POINT('Ctrl Pts',(27.705919430909,3.90560147846434,0.477717226964077));
#82071=CARTESIAN_POINT('Ctrl Pts',(27.7117714609872,3.88980436081067,0.592769928808034));
#82072=CARTESIAN_POINT('Ctrl Pts',(27.7176234910655,3.86894736680903,0.706919566047993));
#82073=CARTESIAN_POINT('Ctrl Pts',(27.723474631444,3.84809354375188,0.821051848813789));
#82074=CARTESIAN_POINT('Ctrl Pts',(27.7293257718224,3.82218144817613,0.934280933449317));
#82075=CARTESIAN_POINT('Ctrl Pts',(27.7351769122009,3.79131894736579,1.04613079456882));
#82076=CARTESIAN_POINT('Ctrl Pts',(27.7410285797684,3.76045366583752,1.15799073338472));
#82077=CARTESIAN_POINT('Ctrl Pts',(27.7468802473359,3.72463720235774,1.26847080316033));
#82078=CARTESIAN_POINT('Ctrl Pts',(27.7527319149034,3.68402754721204,1.37710930262737));
#82079=CARTESIAN_POINT('Ctrl Pts',(27.7585855265876,3.64340440020117,1.48578389538262));
#82080=CARTESIAN_POINT('Ctrl Pts',(27.7644391382719,3.59798503967955,1.5926153142569));
#82081=CARTESIAN_POINT('Ctrl Pts',(27.7702927499561,3.54797564599711,1.69716169395004));
#82082=CARTESIAN_POINT('Ctrl Pts',(27.776153016056,3.49790940138059,1.80182692250145));
#82083=CARTESIAN_POINT('Ctrl Pts',(27.7820132821558,3.44324288717978,1.90420155394945));
#82084=CARTESIAN_POINT('Ctrl Pts',(27.7878735482557,3.38422835755668,2.00386811539812));
#82085=CARTESIAN_POINT('Ctrl Pts',(27.793737761427,3.32517407981299,2.10360180537477));
#82086=CARTESIAN_POINT('Ctrl Pts',(27.7996019745983,3.26176618095077,2.20062344829359));
#82087=CARTESIAN_POINT('Ctrl Pts',(27.8054661877696,3.19429937685201,2.29454581367269));
#82088=CARTESIAN_POINT('Ctrl Pts',(27.8113390363439,3.12673322386795,2.38860648532596));
#82089=CARTESIAN_POINT('Ctrl Pts',(27.8172118849182,3.05509649158996,2.47955844735739));
#82090=CARTESIAN_POINT('Ctrl Pts',(27.8230847334924,2.97972319368144,2.56704863394461));
#82091=CARTESIAN_POINT('Ctrl Pts',(27.8246794781053,2.95925592651549,2.59080618566342));
#82092=CARTESIAN_POINT('Ctrl Pts',(27.8262742227182,2.93851333855551,2.61430869473074));
#82093=CARTESIAN_POINT('Ctrl Pts',(27.8278689673311,2.91750255544411,2.63754958986122));
#82094=CARTESIAN_POINT('Ctrl Pts',(27.833741413465,2.84013299353676,2.72313125833334));
#82095=CARTESIAN_POINT('Ctrl Pts',(27.8396138595989,2.75886504173572,2.80544899926235));
#82096=CARTESIAN_POINT('Ctrl Pts',(27.8454863057328,2.67400495558111,2.88412664380877));
#82097=CARTESIAN_POINT('Ctrl Pts',(27.8513511446777,2.58925479750527,2.96270236903483));
#82098=CARTESIAN_POINT('Ctrl Pts',(27.8572159836225,2.50092205909048,3.03764709667529));
#82099=CARTESIAN_POINT('Ctrl Pts',(27.8630808225673,2.40935218365957,3.10861883399925));
#82100=CARTESIAN_POINT('Ctrl Pts',(27.8689396326873,2.31787643847565,3.17951761515577));
#82101=CARTESIAN_POINT('Ctrl Pts',(27.8747984428073,2.22317049990736,3.24645127774988));
#82102=CARTESIAN_POINT('Ctrl Pts',(27.8806572529273,2.12561498068711,3.30911618923823));
#82103=CARTESIAN_POINT('Ctrl Pts',(27.8867430418083,2.0242800198353,3.37420882985159));
#82104=CARTESIAN_POINT('Ctrl Pts',(27.8928288306893,1.91987055224875,3.43469496579195));
#82105=CARTESIAN_POINT('Ctrl Pts',(27.8989146195703,1.81284926004676,3.4902817307988));
#82106=CARTESIAN_POINT('Ctrl Pts',(27.9047666496485,1.70993871989666,3.54373337480676));
#82107=CARTESIAN_POINT('Ctrl Pts',(27.9106186797268,1.60461369824476,3.59265487255402));
#82108=CARTESIAN_POINT('Ctrl Pts',(27.916470709805,1.49731241563733,3.63683166093487));
#82109=CARTESIAN_POINT('Ctrl Pts',(27.9223218501836,1.39002744633031,3.68100173300067));
#82110=CARTESIAN_POINT('Ctrl Pts',(27.9281729905621,1.28076719559822,3.7204283726566));
#82111=CARTESIAN_POINT('Ctrl Pts',(27.9340241309406,1.16999042518382,3.75494492702332));
#82112=CARTESIAN_POINT('Ctrl Pts',(27.9398757985081,1.05920367375901,3.78946459133888));
#82113=CARTESIAN_POINT('Ctrl Pts',(27.9457274660756,0.946900525693874,3.81907316794247));
#82114=CARTESIAN_POINT('Ctrl Pts',(27.9515791336431,0.833554795176103,3.84365391306748));
#82115=CARTESIAN_POINT('Ctrl Pts',(27.9574327453273,0.720171407472755,3.86824282472576));
#82116=CARTESIAN_POINT('Ctrl Pts',(27.9632863570115,0.605745152313695,3.88780049583462));
#82117=CARTESIAN_POINT('Ctrl Pts',(27.9691399686957,0.490759214554631,3.90226144605019));
#82118=CARTESIAN_POINT('Ctrl Pts',(27.9750002347956,0.375642560194304,3.91673883554781));
#82119=CARTESIAN_POINT('Ctrl Pts',(27.9808605008955,0.259965363668743,3.92610788795599));
#82120=CARTESIAN_POINT('Ctrl Pts',(27.9867207669954,0.14421520330767,3.930355069855));
#82121=CARTESIAN_POINT('Ctrl Pts',(27.9925849801667,0.0283870816149384,
3.93460511236307));
#82122=CARTESIAN_POINT('Ctrl Pts',(27.998449193338,-0.0875136894336054,
3.93372641836407));
#82123=CARTESIAN_POINT('Ctrl Pts',(28.0043134065093,-0.203002012209708,
3.92775752599862));
#82124=CARTESIAN_POINT('Ctrl Pts',(28.0101862550836,-0.318660398416178,
3.92177984408383));
#82125=CARTESIAN_POINT('Ctrl Pts',(28.0160591036579,-0.433904714281006,
3.91069704345804));
#82126=CARTESIAN_POINT('Ctrl Pts',(28.0219319522322,-0.548257353079323,
3.89459919308707));
#82127=CARTESIAN_POINT('Ctrl Pts',(28.023526696845,-0.579309278287869,3.89022789697191));
#82128=CARTESIAN_POINT('Ctrl Pts',(28.0251214414579,-0.610295528116905,
3.88548709437747));
#82129=CARTESIAN_POINT('Ctrl Pts',(28.0267161860708,-0.641206721834683,
3.88037922629658));
#82130=CARTESIAN_POINT('Ctrl Pts',(28.0325886322047,-0.755033298566156,
3.86157014556832));
#82131=CARTESIAN_POINT('Ctrl Pts',(28.0384610783386,-0.868222129685195,
3.83771686546812));
#82132=CARTESIAN_POINT('Ctrl Pts',(28.0443335244725,-0.980291183104439,
3.80887361254318));
#82133=CARTESIAN_POINT('Ctrl Pts',(28.0501983634174,-1.09221506184536,3.78006772327784));
#82134=CARTESIAN_POINT('Ctrl Pts',(28.0560632023622,-1.2030216509221,3.74628481792268));
#82135=CARTESIAN_POINT('Ctrl Pts',(28.0619280413071,-1.31223647825913,3.70763056750886));
#82136=CARTESIAN_POINT('Ctrl Pts',(28.0677868514271,-1.42133903702995,3.66901605215096));
#82137=CARTESIAN_POINT('Ctrl Pts',(28.0736456615472,-1.52885270135796,3.62554028911732));
#82138=CARTESIAN_POINT('Ctrl Pts',(28.0795044716673,-1.63431625163951,3.57735927600611));
#82139=CARTESIAN_POINT('Ctrl Pts',(28.0855902605482,-1.74386561208965,3.52731166090041));
#82140=CARTESIAN_POINT('Ctrl Pts',(28.0916760494292,-1.85120235701782,3.47218695907927));
#82141=CARTESIAN_POINT('Ctrl Pts',(28.0977618383102,-1.95582994775565,3.41221602708007));
#82142=CARTESIAN_POINT('Ctrl Pts',(28.1036138683884,-2.05643872995143,3.35454861456454));
#82143=CARTESIAN_POINT('Ctrl Pts',(28.1094658984667,-2.15454224760076,3.29240062221843));
#82144=CARTESIAN_POINT('Ctrl Pts',(28.115317928545,-2.24972305797007,3.22602466860342));
#82145=CARTESIAN_POINT('Ctrl Pts',(28.1211690689235,-2.34488939774674,3.15965880630179));
#82146=CARTESIAN_POINT('Ctrl Pts',(28.127020209302,-2.43713357478847,3.08906649718448));
#82147=CARTESIAN_POINT('Ctrl Pts',(28.1328713496805,-2.52606734203592,3.0145435448007));
#82148=CARTESIAN_POINT('Ctrl Pts',(28.138723017248,-2.61500912223483,2.94001387788297));
#82149=CARTESIAN_POINT('Ctrl Pts',(28.1445746848156,-2.70063958286243,2.86155312918251));
#82150=CARTESIAN_POINT('Ctrl Pts',(28.1504263523831,-2.78260432183879,2.7794967508677));
#82151=CARTESIAN_POINT('Ctrl Pts',(28.1562799640673,-2.86459629220127,2.69741311072115));
#82152=CARTESIAN_POINT('Ctrl Pts',(28.1621335757515,-2.94291982727585,2.61173175789363));
#82153=CARTESIAN_POINT('Ctrl Pts',(28.1679871874358,-3.01725858141465,2.52282374590054));
#82154=CARTESIAN_POINT('Ctrl Pts',(28.1738474535357,-3.09168184422896,2.43381466282518));
#82155=CARTESIAN_POINT('Ctrl Pts',(28.1797077196356,-3.16211101923544,2.34157191651411));
#82156=CARTESIAN_POINT('Ctrl Pts',(28.1855679857355,-3.2282710834055,2.24649834454599));
#82157=CARTESIAN_POINT('Ctrl Pts',(28.1914321989068,-3.29447570843561,2.15136073757143));
#82158=CARTESIAN_POINT('Ctrl Pts',(28.1972964120781,-3.35640527684828,2.05338885696761));
#82159=CARTESIAN_POINT('Ctrl Pts',(28.2031606252494,-3.4138299100163,1.95301160915087));
#82160=CARTESIAN_POINT('Ctrl Pts',(28.2090334738237,-3.47133910437526,1.85248654986108));
#82161=CARTESIAN_POINT('Ctrl Pts',(28.214906322398,-3.52432993529329,1.74954942027436));
#82162=CARTESIAN_POINT('Ctrl Pts',(28.2207791709723,-3.5726199227409,1.64465068863719));
#82163=CARTESIAN_POINT('Ctrl Pts',(28.222373915585,-3.58573284338834,1.61616592778553));
#82164=CARTESIAN_POINT('Ctrl Pts',(28.2239686601977,-3.59849942054148,1.58753661771179));
#82165=CARTESIAN_POINT('Ctrl Pts',(28.2255634048104,-3.61091663532755,1.55877196944093));
#82166=CARTESIAN_POINT('Ctrl Pts',(28.2323194906888,-3.66352177899585,1.43691143300609));
#82167=CARTESIAN_POINT('Ctrl Pts',(28.2390755765672,-3.71000883784057,1.31225778602846));
#82168=CARTESIAN_POINT('Ctrl Pts',(28.2458316624456,-3.75010443956021,1.18541372203582));
#82169=CARTESIAN_POINT('Ctrl Pts',(28.2523049043881,-3.78852143653605,1.06387999230453));
#82170=CARTESIAN_POINT('Ctrl Pts',(28.2587781463305,-3.82107110275934,0.940335813861802));
#82171=CARTESIAN_POINT('Ctrl Pts',(28.265251388273,-3.84755994505957,0.815335188234384));
#82172=CARTESIAN_POINT('Ctrl Pts',(28.2717062130248,-3.87397342325884,0.690690205170065));
#82173=CARTESIAN_POINT('Ctrl Pts',(28.2781610377765,-3.8943603892922,0.564597288335471));
#82174=CARTESIAN_POINT('Ctrl Pts',(28.2846158625283,-3.90857683972787,0.437625511074123));
#82175=CARTESIAN_POINT('Ctrl Pts',(28.2910434986928,-3.9227334085682,0.311188555962646));
#82176=CARTESIAN_POINT('Ctrl Pts',(28.2974711348572,-3.93077123230382,0.183880379132744));
#82177=CARTESIAN_POINT('Ctrl Pts',(28.3038987710217,-3.93259732066487,0.0562788903539033));
#82178=CARTESIAN_POINT('Ctrl Pts',(28.3048113257982,-3.93285657704056,0.0381628450309305));
#82179=CARTESIAN_POINT('Ctrl Pts',(28.3057238805747,-3.93299070927667,0.0200409103137733));
#82180=CARTESIAN_POINT('Ctrl Pts',(28.3066364353512,-3.93299953390383,0.00191476166166355));
#82181=CARTESIAN_POINT('',(29.5566365080617,-3.9323872535115,-0.00334900090502091));
#82182=CARTESIAN_POINT('Ctrl Pts',(28.3066364779651,-3.92739873788489,0.00191118970400611));
#82183=CARTESIAN_POINT('Ctrl Pts',(28.3458945264934,-3.92399062950395,-0.776765967029143));
#82184=CARTESIAN_POINT('Ctrl Pts',(28.4514349812685,-3.32238059726958,-2.87499851905737));
#82185=CARTESIAN_POINT('Ctrl Pts',(28.6232578422896,0.0963581091439014,
-4.65066730542375));
#82186=CARTESIAN_POINT('Ctrl Pts',(28.8221050610294,3.9642846102464,-2.43360613081016));
#82187=CARTESIAN_POINT('Ctrl Pts',(29.0209522797691,4.19070045060739,2.01891579919035));
#82188=CARTESIAN_POINT('Ctrl Pts',(29.2197994985086,0.567624675912214,4.61690302023292));
#82189=CARTESIAN_POINT('Ctrl Pts',(29.3983608979072,-3.15405118804572,3.14151233710411));
#82190=CARTESIAN_POINT('Ctrl Pts',(29.5106398910595,-3.92290060823451,0.907342439014413));
#82191=CARTESIAN_POINT('Ctrl Pts',(29.5566364779651,-3.93022207073951,-0.0033465609634104));
#82192=CARTESIAN_POINT('',(30.8066364779651,-3.93544205199766,-0.000484814710531748));
#82193=CARTESIAN_POINT('Ctrl Pts',(29.5566365165592,-3.93299857355406,-0.00334968980077072));
#82194=CARTESIAN_POINT('Ctrl Pts',(29.5636420149798,-3.93288035987524,-0.14214887951555));
#82195=CARTESIAN_POINT('Ctrl Pts',(29.5706475134005,-3.92541082729009,-0.280628809344632));
#82196=CARTESIAN_POINT('Ctrl Pts',(29.5776530118211,-3.91071391485967,-0.41809768729681));
#82197=CARTESIAN_POINT('Ctrl Pts',(29.5847475963944,-3.89583010760655,-0.557314702600614));
#82198=CARTESIAN_POINT('Ctrl Pts',(29.5918421809678,-3.87353400600672,-0.695494759666681));
#82199=CARTESIAN_POINT('Ctrl Pts',(29.5989367655412,-3.84400351079835,-0.83194110907562));
#82200=CARTESIAN_POINT('Ctrl Pts',(29.6051224890234,-3.81825605853182,-0.950907819371501));
#82201=CARTESIAN_POINT('Ctrl Pts',(29.6113082125057,-3.78700982382328,-1.06855691050145));
#82202=CARTESIAN_POINT('Ctrl Pts',(29.617493935988,-3.75041210475301,-1.18443997083941));
#82203=CARTESIAN_POINT('Ctrl Pts',(29.6233663821219,-3.71566788534505,-1.29445410768542));
#82204=CARTESIAN_POINT('Ctrl Pts',(29.6292388282558,-3.67602068029653,-1.40312236244948));
#82205=CARTESIAN_POINT('Ctrl Pts',(29.6351112743898,-3.63159245459888,-1.50997524605554));
#82206=CARTESIAN_POINT('Ctrl Pts',(29.6409761133346,-3.58722178139388,-1.61668971202953));
#82207=CARTESIAN_POINT('Ctrl Pts',(29.6468409522795,-3.5380825611499,-1.72159310525812));
#82208=CARTESIAN_POINT('Ctrl Pts',(29.6527057912243,-3.48434661357268,-1.82423070813003));
#82209=CARTESIAN_POINT('Ctrl Pts',(29.6585646013444,-3.4306659044457,-1.92676280356466));
#82210=CARTESIAN_POINT('Ctrl Pts',(29.6644234114644,-3.37239805735304,-2.0270333774321));
#82211=CARTESIAN_POINT('Ctrl Pts',(29.6702822215844,-3.30976283367029,-2.12460796027286));
#82212=CARTESIAN_POINT('Ctrl Pts',(29.6763680104654,-3.24470103101146,-2.2259627232966));
#82213=CARTESIAN_POINT('Ctrl Pts',(29.6824537993464,-3.17492678520572,-2.32440795774144));
#82214=CARTESIAN_POINT('Ctrl Pts',(29.6885395882273,-3.10073896497493,-2.41948483588681));
#82215=CARTESIAN_POINT('Ctrl Pts',(29.6943916183056,-3.02940074343561,-2.51090975409172));
#82216=CARTESIAN_POINT('Ctrl Pts',(29.7002436483839,-2.95398202702203,-2.59921994796741));
#82217=CARTESIAN_POINT('Ctrl Pts',(29.7060956784621,-2.87479202217847,-2.6840379708974));
#82218=CARTESIAN_POINT('Ctrl Pts',(29.7119468188406,-2.79561405680271,-2.76884309871697));
#82219=CARTESIAN_POINT('Ctrl Pts',(29.7177979592192,-2.71266622503623,-2.85015680918375));
#82220=CARTESIAN_POINT('Ctrl Pts',(29.7236490995977,-2.62629634689994,-2.92763667456535));
#82221=CARTESIAN_POINT('Ctrl Pts',(29.7295007671652,-2.53991868681935,-3.00512352089921));
#82222=CARTESIAN_POINT('Ctrl Pts',(29.7353524347327,-2.45011867515528,-3.07877555942503));
#82223=CARTESIAN_POINT('Ctrl Pts',(29.7412041023002,-2.35727858617364,-3.1482894827457));
#82224=CARTESIAN_POINT('Ctrl Pts',(29.7470577139844,-2.26440765265608,-3.21782650088165));
#82225=CARTESIAN_POINT('Ctrl Pts',(29.7529113256686,-2.16849496417907,-3.2832224224523));
#82226=CARTESIAN_POINT('Ctrl Pts',(29.7587649373529,-2.06995264619744,-3.34421665603475));
#82227=CARTESIAN_POINT('Ctrl Pts',(29.7646252034527,-1.97129830480545,-3.40528022817344));
#82228=CARTESIAN_POINT('Ctrl Pts',(29.7704854695526,-1.87000871889741,-3.4619319071041));
#82229=CARTESIAN_POINT('Ctrl Pts',(29.7763457356525,-1.7665216236375,-3.51395650986479));
#82230=CARTESIAN_POINT('Ctrl Pts',(29.7822099488238,-1.66296482660153,-3.56601615281288));
#82231=CARTESIAN_POINT('Ctrl Pts',(29.7880741619951,-1.55720794930092,-3.61344234532776));
#82232=CARTESIAN_POINT('Ctrl Pts',(29.7939383751664,-1.44970813762182,-3.65606828652216));
#82233=CARTESIAN_POINT('Ctrl Pts',(29.7998112237407,-1.3420500260706,-3.69875699695247));
#82234=CARTESIAN_POINT('Ctrl Pts',(29.805684072315,-1.23264424691249,-3.73663121371915));
#82235=CARTESIAN_POINT('Ctrl Pts',(29.8115569208893,-1.12196257586798,-3.76957411100401));
#82236=CARTESIAN_POINT('Ctrl Pts',(29.813151665502,-1.09190748481735,-3.77851960096657));
#82237=CARTESIAN_POINT('Ctrl Pts',(29.8147464101148,-1.06175836577921,-3.78710176321037));
#82238=CARTESIAN_POINT('Ctrl Pts',(29.8163411547275,-1.03152476454455,-3.7953189141535));
#82239=CARTESIAN_POINT('Ctrl Pts',(29.8222136008614,-0.920193336761872,
-3.8255775373226));
#82240=CARTESIAN_POINT('Ctrl Pts',(29.8280860469953,-0.807342982445388,
-3.85098399304252));
#82241=CARTESIAN_POINT('Ctrl Pts',(29.8339584931293,-0.693434587710648,
-3.87138702180066));
#82242=CARTESIAN_POINT('Ctrl Pts',(29.8398233320741,-0.579673750344011,
-3.89176362039768));
#82243=CARTESIAN_POINT('Ctrl Pts',(29.8456881710189,-0.464858001304861,
-3.90714960914067));
#82244=CARTESIAN_POINT('Ctrl Pts',(29.8515530099638,-0.349462757775396,
-3.91744365382937));
#82245=CARTESIAN_POINT('Ctrl Pts',(29.8574118200838,-0.234186136038471,
-3.92772711664315));
#82246=CARTESIAN_POINT('Ctrl Pts',(29.8632706302038,-0.118331613936684,
-3.93292901024229));
#82247=CARTESIAN_POINT('Ctrl Pts',(29.8691294403239,-0.0023834982782619,
-3.93299927776957));
#82248=CARTESIAN_POINT('Ctrl Pts',(29.8752152292048,0.118056614746108,-3.93307226756228));
#82249=CARTESIAN_POINT('Ctrl Pts',(29.8813010180858,0.238597272655179,-3.9276078962786));
#82250=CARTESIAN_POINT('Ctrl Pts',(29.8873868069668,0.358690904102268,-3.91660948210494));
#82251=CARTESIAN_POINT('Ctrl Pts',(29.8932388370451,0.474171667103122,-3.9060335236193));
#82252=CARTESIAN_POINT('Ctrl Pts',(29.8990908671233,0.589238661592703,-3.89034085313425));
#82253=CARTESIAN_POINT('Ctrl Pts',(29.9049428972016,0.703407185022154,-3.86958748861674));
#82254=CARTESIAN_POINT('Ctrl Pts',(29.9107940375801,0.817558351106234,-3.84883727928864));
#82255=CARTESIAN_POINT('Ctrl Pts',(29.9166451779586,0.930810911148064,-3.82302797963558));
#82256=CARTESIAN_POINT('Ctrl Pts',(29.9224963183372,1.04268874204003,-3.79226702477858));
#82257=CARTESIAN_POINT('Ctrl Pts',(29.9283479859047,1.15457665314818,-3.76150329835305));
#82258=CARTESIAN_POINT('Ctrl Pts',(29.9341996534722,1.26508919028757,-3.72578713942102));
#82259=CARTESIAN_POINT('Ctrl Pts',(29.9400513210397,1.37376450896226,-3.68527611908737));
#82260=CARTESIAN_POINT('Ctrl Pts',(29.9459049327239,1.48247593315799,-3.64475163965818));
#82261=CARTESIAN_POINT('Ctrl Pts',(29.9517585444082,1.58934853806043,-3.59942927552809));
#82262=CARTESIAN_POINT('Ctrl Pts',(29.9576121560924,1.69394027138842,-3.54951480585284));
#82263=CARTESIAN_POINT('Ctrl Pts',(29.9634724221923,1.79865090513289,-3.49954359315361));
#82264=CARTESIAN_POINT('Ctrl Pts',(29.9693326882922,1.90107511867518,-3.44497003344469));
#82265=CARTESIAN_POINT('Ctrl Pts',(29.9751929543921,2.00079521030422,-3.38604600181741));
#82266=CARTESIAN_POINT('Ctrl Pts',(29.9810571675634,2.10058246651529,-3.32708228302288));
#82267=CARTESIAN_POINT('Ctrl Pts',(29.9869213807347,2.19766162884491,-3.26376248300584));
#82268=CARTESIAN_POINT('Ctrl Pts',(29.992785593906,2.29164519943838,-3.19638096601313));
#82269=CARTESIAN_POINT('Ctrl Pts',(29.9986584424803,2.38576716643431,-3.12890022572548));
#82270=CARTESIAN_POINT('Ctrl Pts',(30.0045312910546,2.47678412021313,-3.05734608584746));
#82271=CARTESIAN_POINT('Ctrl Pts',(30.0104041396289,2.56434269189248,-2.98205223940454));
#82272=CARTESIAN_POINT('Ctrl Pts',(30.0119988842417,2.58811881326234,-2.96160654691442));
#82273=CARTESIAN_POINT('Ctrl Pts',(30.0135936288545,2.61164014201203,-2.94088530222528));
#82274=CARTESIAN_POINT('Ctrl Pts',(30.0151883734673,2.6349001003905,-2.91989562501164));
#82275=CARTESIAN_POINT('Ctrl Pts',(30.0210608196012,2.7205519668771,-2.84260378290915));
#82276=CARTESIAN_POINT('Ctrl Pts',(30.0269332657351,2.80294344598199,-2.76141058964439));
#82277=CARTESIAN_POINT('Ctrl Pts',(30.032805711869,2.88169809101305,-2.67662195915893));
#82278=CARTESIAN_POINT('Ctrl Pts',(30.0386705508139,2.96035071697719,-2.5919431641881));
#82279=CARTESIAN_POINT('Ctrl Pts',(30.0445353897587,3.03537559898794,-2.50367849426677));
#82280=CARTESIAN_POINT('Ctrl Pts',(30.0504002287036,3.10643043087439,-2.41217308212689));
#82281=CARTESIAN_POINT('Ctrl Pts',(30.0562590388236,3.17741222117548,-2.32076173396823));
#82282=CARTESIAN_POINT('Ctrl Pts',(30.0621178489436,3.24443182679994,-2.2261165943656));
#82283=CARTESIAN_POINT('Ctrl Pts',(30.0679766590636,3.30718526982313,-2.128618000268));
#82284=CARTESIAN_POINT('Ctrl Pts',(30.0740624479446,3.37236987181047,-2.02734216990075));
#82285=CARTESIAN_POINT('Ctrl Pts',(30.0801482368256,3.43295076194822,-1.92298765244804));
#82286=CARTESIAN_POINT('Ctrl Pts',(30.0862340257065,3.48863465409053,-1.8160168639852));
#82287=CARTESIAN_POINT('Ctrl Pts',(30.0920860557848,3.54217969452251,-1.7131548876951));
#82288=CARTESIAN_POINT('Ctrl Pts',(30.0979380858631,3.5911967823388,-1.60787431859592));
#82289=CARTESIAN_POINT('Ctrl Pts',(30.1037901159414,3.63547095672144,-1.50061318228079));
#82290=CARTESIAN_POINT('Ctrl Pts',(30.1096412563199,3.67973839998318,-1.39336835316249));
#82291=CARTESIAN_POINT('Ctrl Pts',(30.1154923966984,3.71926420587809,-1.28414393751746));
#82292=CARTESIAN_POINT('Ctrl Pts',(30.1213435370769,3.75388130514824,-1.17339854561805));
#82293=CARTESIAN_POINT('Ctrl Pts',(30.1271952046444,3.78850152342635,-1.06264317553542));
#82294=CARTESIAN_POINT('Ctrl Pts',(30.1330468722119,3.81821203254567,-0.950366951330369));
#82295=CARTESIAN_POINT('Ctrl Pts',(30.1388985397794,3.84289565867639,-0.837043581019613));
#82296=CARTESIAN_POINT('Ctrl Pts',(30.1447521514636,3.86758748552087,-0.723682560952003));
#82297=CARTESIAN_POINT('Ctrl Pts',(30.1506057631479,3.88724902056602,-0.6092741066811));
#82298=CARTESIAN_POINT('Ctrl Pts',(30.1564593748321,3.90181434487731,-0.494301343422853));
#82299=CARTESIAN_POINT('Ctrl Pts',(30.162319640932,3.91639622712365,-0.379197878540295));
#82300=CARTESIAN_POINT('Ctrl Pts',(30.1681799070319,3.92587028322505,-0.263529234560758));
#82301=CARTESIAN_POINT('Ctrl Pts',(30.1740401731318,3.93022253716149,-0.14778297732793));
#82302=CARTESIAN_POINT('Ctrl Pts',(30.1799043863031,3.93457772247626,-0.0319587613922855));
#82303=CARTESIAN_POINT('Ctrl Pts',(30.1857685994744,3.93380423934554,0.0839427595497822));
#82304=CARTESIAN_POINT('Ctrl Pts',(30.1916328126457,3.92794018554004,0.199436453086367));
#82305=CARTESIAN_POINT('Ctrl Pts',(30.19750566122,3.92206749656623,0.315100217961935));
#82306=CARTESIAN_POINT('Ctrl Pts',(30.2033785097943,3.91108931510681,0.430354546907637));
#82307=CARTESIAN_POINT('Ctrl Pts',(30.2092513583686,3.89509527653647,0.544721751634045));
#82308=CARTESIAN_POINT('Ctrl Pts',(30.2108461029814,3.89075217003141,0.575777632150334));
#82309=CARTESIAN_POINT('Ctrl Pts',(30.2124408475941,3.88603949758164,0.606768172738725));
#82310=CARTESIAN_POINT('Ctrl Pts',(30.2140355922069,3.88095969166349,0.637683990455502));
#82311=CARTESIAN_POINT('Ctrl Pts',(30.2199080383408,3.86225394631316,0.751527594487761));
#82312=CARTESIAN_POINT('Ctrl Pts',(30.2257804844747,3.83850342474694,0.864738032111168));
#82313=CARTESIAN_POINT('Ctrl Pts',(30.2316529306086,3.80976191591847,0.976833222212087));
#82314=CARTESIAN_POINT('Ctrl Pts',(30.2375177695534,3.78105763894991,1.08878320377716));
#82315=CARTESIAN_POINT('Ctrl Pts',(30.2433826084983,3.74737533370723,1.19962041409267));
#82316=CARTESIAN_POINT('Ctrl Pts',(30.2492474474431,3.70882024046955,1.30887028535427));
#82317=CARTESIAN_POINT('Ctrl Pts',(30.2551062575631,3.67030478035827,1.4180078520254));
#82318=CARTESIAN_POINT('Ctrl Pts',(30.2609650676831,3.62692663223362,1.52556093777231));
#82319=CARTESIAN_POINT('Ctrl Pts',(30.2668238778031,3.57884137495112,1.63106818157243));
#82320=CARTESIAN_POINT('Ctrl Pts',(30.2729096666841,3.52889322539274,1.740662928292));
#82321=CARTESIAN_POINT('Ctrl Pts',(30.2789954555651,3.47386598267881,1.848049669196));
#82322=CARTESIAN_POINT('Ctrl Pts',(30.2850812444461,3.41399005251188,1.95273165625744));
#82323=CARTESIAN_POINT('Ctrl Pts',(30.2909332745243,3.35641399275139,2.05339274538111));
#82324=CARTESIAN_POINT('Ctrl Pts',(30.2967853046026,3.29435508081834,2.15155263829803));
#82325=CARTESIAN_POINT('Ctrl Pts',(30.3026373346808,3.22806555623097,2.24679366312869));
#82326=CARTESIAN_POINT('Ctrl Pts',(30.3084884750593,3.16178610981697,2.34202020821212));
#82327=CARTESIAN_POINT('Ctrl Pts',(30.3143396154379,3.09127756569557,2.43432842837938));
#82328=CARTESIAN_POINT('Ctrl Pts',(30.3201907558164,3.01683537485756,2.52332980821138));
#82329=CARTESIAN_POINT('Ctrl Pts',(30.3260424233839,2.94238647676238,2.61233920708655));
#82330=CARTESIAN_POINT('Ctrl Pts',(30.3318940909514,2.86400349260866,2.69804085624789));
#82331=CARTESIAN_POINT('Ctrl Pts',(30.3377457585188,2.78202155271323,2.78008004925022));
#82332=CARTESIAN_POINT('Ctrl Pts',(30.3435993702031,2.70001237571666,2.86214649837504));
#82333=CARTESIAN_POINT('Ctrl Pts',(30.3494529818873,2.61440215744926,2.94054777959619));
#82334=CARTESIAN_POINT('Ctrl Pts',(30.3553065935715,2.52556166410646,3.01496721056727));
#82335=CARTESIAN_POINT('Ctrl Pts',(30.3611668596714,2.43662017643716,3.08947124192751));
#82336=CARTESIAN_POINT('Ctrl Pts',(30.3670271257713,2.34444140117678,3.15998412252751));
#82337=CARTESIAN_POINT('Ctrl Pts',(30.3728873918712,2.24942792608211,3.22623046377067));
#82338=CARTESIAN_POINT('Ctrl Pts',(30.3787516050425,2.15435045645802,3.29252142398425));
#82339=CARTESIAN_POINT('Ctrl Pts',(30.3846158182138,2.05643483363147,3.35453990219237));
#82340=CARTESIAN_POINT('Ctrl Pts',(30.3904800313851,1.95610975516662,3.41205563051689));
#82341=CARTESIAN_POINT('Ctrl Pts',(30.3963528799594,1.85563694205142,3.46965605417525));
#82342=CARTESIAN_POINT('Ctrl Pts',(30.4022257285336,1.75274795802705,3.52274030584411));
#82343=CARTESIAN_POINT('Ctrl Pts',(30.4080985771079,1.64789310550567,3.57112549665044));
#82344=CARTESIAN_POINT('Ctrl Pts',(30.4096933217208,1.61942025981996,3.58426426932691));
#82345=CARTESIAN_POINT('Ctrl Pts',(30.4112880663337,1.59080255057366,3.59705682986824));
#82346=CARTESIAN_POINT('Ctrl Pts',(30.4128828109465,1.56204918604753,3.60950015104145));
#82347=CARTESIAN_POINT('Ctrl Pts',(30.4187552570804,1.45616854347534,3.65532111367539));
#82348=CARTESIAN_POINT('Ctrl Pts',(30.4246277032144,1.34809276397599,3.6965560060263));
#82349=CARTESIAN_POINT('Ctrl Pts',(30.4305001493483,1.23825646271758,3.7329894096472));
#82350=CARTESIAN_POINT('Ctrl Pts',(30.4363649882931,1.12856244382185,3.76937561729839));
#82351=CARTESIAN_POINT('Ctrl Pts',(30.4422298272379,1.01711282716177,3.80097257638203));
#82352=CARTESIAN_POINT('Ctrl Pts',(30.4480946661828,0.904363727901238,3.82761221228804));
#82353=CARTESIAN_POINT('Ctrl Pts',(30.4539534763028,0.791730530300531,3.85422446369131));
#82354=CARTESIAN_POINT('Ctrl Pts',(30.4598122864228,0.677800906978657,3.8758894335315));
#82355=CARTESIAN_POINT('Ctrl Pts',(30.4656710965428,0.563047082020645,3.89248853349988));
#82356=CARTESIAN_POINT('Ctrl Pts',(30.4717568854238,0.443847528242206,3.90973070656102));
#82357=CARTESIAN_POINT('Ctrl Pts',(30.4778426743048,0.323759050963221,3.92150640983129));
#82358=CARTESIAN_POINT('Ctrl Pts',(30.4839284631858,0.203324101774599,3.92774086589703));
#82359=CARTESIAN_POINT('Ctrl Pts',(30.489780493264,0.0875151312516204,3.93373585276428));
#82360=CARTESIAN_POINT('Ctrl Pts',(30.4956325233423,-0.0286137347967784,
3.93460740202397));
#82361=CARTESIAN_POINT('Ctrl Pts',(30.5014845534205,-0.14457475857213,3.93034186034546));
#82362=CARTESIAN_POINT('Ctrl Pts',(30.507335693799,-0.260518152483535,3.92607696716864));
#82363=CARTESIAN_POINT('Ctrl Pts',(30.5131868341776,-0.376293341894099,
3.91667655113809));
#82364=CARTESIAN_POINT('Ctrl Pts',(30.5190379745561,-0.491413750794095,
3.90217907399577));
#82365=CARTESIAN_POINT('Ctrl Pts',(30.5248896421236,-0.606544532067361,
3.88768029062768));
#82366=CARTESIAN_POINT('Ctrl Pts',(30.5307413096911,-0.721020005409382,
3.86808358485917));
#82367=CARTESIAN_POINT('Ctrl Pts',(30.5365929772586,-0.834360580202792,
3.84347907789332));
#82368=CARTESIAN_POINT('Ctrl Pts',(30.5424465889428,-0.947738810468877,
3.81886639649971));
#82369=CARTESIAN_POINT('Ctrl Pts',(30.548300200627,-1.05998098870953,3.78924269327498));
#82370=CARTESIAN_POINT('Ctrl Pts',(30.5541538123112,-1.17062024183378,3.75474862666052));
#82371=CARTESIAN_POINT('Ctrl Pts',(30.5600140784111,-1.28138527022589,3.720215347015));
#82372=CARTESIAN_POINT('Ctrl Pts',(30.565874344511,-1.39054334156857,3.68080077610797));
#82373=CARTESIAN_POINT('Ctrl Pts',(30.5717346106109,-1.49764511319724,3.63669466891523));
#82374=CARTESIAN_POINT('Ctrl Pts',(30.5775988237822,-1.60481902119897,3.592558854888));
#82375=CARTESIAN_POINT('Ctrl Pts',(30.5834630369535,-1.70993349774922,3.54372538632));
#82376=CARTESIAN_POINT('Ctrl Pts',(30.5893272501248,-1.8125630382938,3.4904303792242));
#82377=CARTESIAN_POINT('Ctrl Pts',(30.5952000986991,-1.91534370694621,3.43705689205787));
#82378=CARTESIAN_POINT('Ctrl Pts',(30.6010729472734,-2.01563177981354,3.37920895994793));
#82379=CARTESIAN_POINT('Ctrl Pts',(30.6069457958477,-2.11302992602051,3.31716649141127));
#82380=CARTESIAN_POINT('Ctrl Pts',(30.6085405404605,-2.13947793791766,3.30031914872675));
#82381=CARTESIAN_POINT('Ctrl Pts',(30.6101352850733,-2.16571304229105,3.28316274507734));
#82382=CARTESIAN_POINT('Ctrl Pts',(30.6117300296861,-2.19172771359365,3.26570338969502));
#82383=CARTESIAN_POINT('Ctrl Pts',(30.6175826628863,-2.28720025993826,3.2016284261294));
#82384=CARTESIAN_POINT('Ctrl Pts',(30.6234352960864,-2.38002577654119,3.13325231778851));
#82385=CARTESIAN_POINT('Ctrl Pts',(30.6292879292865,-2.46978966200441,3.0608214625254));
#82386=CARTESIAN_POINT('Ctrl Pts',(30.6351329685946,-2.55943707728573,2.98848458754003));
#82387=CARTESIAN_POINT('Ctrl Pts',(30.6409780079027,-2.64603043913017,2.91210368561626));
#82388=CARTESIAN_POINT('Ctrl Pts',(30.6468230472108,-2.72918320320198,2.83196893403868));
#82389=CARTESIAN_POINT('Ctrl Pts',(30.6526620940125,-2.81225071661165,2.75191633896797));
#82390=CARTESIAN_POINT('Ctrl Pts',(30.6585011408142,-2.8918843493997,2.66811783541977));
#82391=CARTESIAN_POINT('Ctrl Pts',(30.6643401876159,-2.9677303752455,2.58090399276013));
#82392=CARTESIAN_POINT('Ctrl Pts',(30.6702691997138,-3.04474500110615,2.49234640009262));
#82393=CARTESIAN_POINT('Ctrl Pts',(30.6761982118117,-3.11785398546651,2.40026761360309));
#82394=CARTESIAN_POINT('Ctrl Pts',(30.6821272239096,-3.18672548496361,2.30505307606646));
#82395=CARTESIAN_POINT('Ctrl Pts',(30.6879596771534,-3.25447535526495,2.21138918583592));
#82396=CARTESIAN_POINT('Ctrl Pts',(30.6937921303972,-3.31812447955412,2.11469126848677));
#82397=CARTESIAN_POINT('Ctrl Pts',(30.699624583641,-3.37739792399084,2.01535909034156));
#82398=CARTESIAN_POINT('Ctrl Pts',(30.705456208986,-3.43666295474479,1.91604101209293));
#82399=CARTESIAN_POINT('Ctrl Pts',(30.711287834331,-3.49155332717248,1.81408977406003));
#82400=CARTESIAN_POINT('Ctrl Pts',(30.717119459676,-3.54183850283713,1.709932460602));
#82401=CARTESIAN_POINT('Ctrl Pts',(30.7229516944836,-3.59212893380038,1.60576426167373));
#82402=CARTESIAN_POINT('Ctrl Pts',(30.7287839292912,-3.63781303043699,1.49938990421546));
#82403=CARTESIAN_POINT('Ctrl Pts',(30.7346161640988,-3.67870744569314,1.3912586132714));
#82404=CARTESIAN_POINT('Ctrl Pts',(30.740617856921,-3.72079006523903,1.27998552257424));
#82405=CARTESIAN_POINT('Ctrl Pts',(30.7466195497432,-3.75780023394118,1.16685227392636));
#82406=CARTESIAN_POINT('Ctrl Pts',(30.7526212425654,-3.78959289579709,1.05236623098816));
#82407=CARTESIAN_POINT('Ctrl Pts',(30.7584622457792,-3.82053433941606,0.940945442795381));
#82408=CARTESIAN_POINT('Ctrl Pts',(30.764303248993,-3.84653408883727,0.828243806335129));
#82409=CARTESIAN_POINT('Ctrl Pts',(30.7701442522068,-3.86751042118617,0.714739212591838));
#82410=CARTESIAN_POINT('Ctrl Pts',(30.7762262898332,-3.88935236133569,0.596550746562568));
#82411=CARTESIAN_POINT('Ctrl Pts',(30.7823083274596,-3.90574732588091,0.477492137902916));
#82412=CARTESIAN_POINT('Ctrl Pts',(30.788390365086,-3.91666289591793,0.358107190293335));
#82413=CARTESIAN_POINT('Ctrl Pts',(30.7944724027123,-3.92757846595495,0.238722242683717));
#82414=CARTESIAN_POINT('Ctrl Pts',(30.8005544403387,-3.9330146910959,0.119011460734204));
#82415=CARTESIAN_POINT('Ctrl Pts',(30.8066364779651,-3.9329999701559,-0.000484513865750852));
#82416=CARTESIAN_POINT('',(32.0566364779651,-3.93299836096378,0.0035906345187518));
#82417=CARTESIAN_POINT('Ctrl Pts',(30.8066364779651,-3.93943799754381,-0.000485306978784902));
#82418=CARTESIAN_POINT('Ctrl Pts',(30.8079500681187,-3.9394828345648,-0.026336136481718));
#82419=CARTESIAN_POINT('Ctrl Pts',(30.8092636582722,-3.93925047646468,-0.0521861383401698));
#82420=CARTESIAN_POINT('Ctrl Pts',(30.8768596546724,-3.91290316029452,-1.38211552106476));
#82421=CARTESIAN_POINT('Ctrl Pts',(31.0094244671653,-2.43720376157095,-3.96207383771694));
#82422=CARTESIAN_POINT('Ctrl Pts',(31.2082716859051,2.01511080184506,-4.19253142233196));
#82423=CARTESIAN_POINT('Ctrl Pts',(31.4071189046448,4.61638584894327,-0.571815498755066));
#82424=CARTESIAN_POINT('Ctrl Pts',(31.6059661233843,2.97714339143227,3.57415843210569));
#82425=CARTESIAN_POINT('Ctrl Pts',(31.8048133421241,-1.39684201829475,4.43698362030694));
#82426=CARTESIAN_POINT('Ctrl Pts',(31.9550365843866,-3.73190738848403,2.00973408201049));
#82427=CARTESIAN_POINT('Ctrl Pts',(32.0389774204028,-3.93478407738548,0.352892674307761));
#82428=CARTESIAN_POINT('Ctrl Pts',(32.0566358501724,-3.93168473390337,0.00360185313312367));
#82429=CARTESIAN_POINT('',(33.3066367910396,-3.93066234985505,-0.00113524685437975));
#82430=CARTESIAN_POINT('Ctrl Pts',(32.0566364779651,-3.93299836096378,0.0035906345187518));
#82431=CARTESIAN_POINT('Ctrl Pts',(32.0627144488667,-3.93310815591637,-0.116673170205319));
#82432=CARTESIAN_POINT('Ctrl Pts',(32.0687924197683,-3.92769665718947,-0.237065644027127));
#82433=CARTESIAN_POINT('Ctrl Pts',(32.0748703906699,-3.91676081377956,-0.357034630870517));
#82434=CARTESIAN_POINT('Ctrl Pts',(32.0806648687197,-3.90633504741434,-0.471407942650909));
#82435=CARTESIAN_POINT('Ctrl Pts',(32.0864593467694,-3.89088869568617,-0.585395908830107));
#82436=CARTESIAN_POINT('Ctrl Pts',(32.0922538248192,-3.8704724238071,-0.698521450313995));
#82437=CARTESIAN_POINT('Ctrl Pts',(32.0980469710849,-3.85006084433813,-0.811620991388227));
#82438=CARTESIAN_POINT('Ctrl Pts',(32.1038401173505,-3.82468168979032,-0.923858086228779));
#82439=CARTESIAN_POINT('Ctrl Pts',(32.1096332636162,-3.79443712046992,-1.03476371157863));
#82440=CARTESIAN_POINT('Ctrl Pts',(32.1154265492162,-3.76419182371933,-1.14567200438586));
#82441=CARTESIAN_POINT('Ctrl Pts',(32.1212198348163,-3.72908099129357,-1.25524835663895));
#82442=CARTESIAN_POINT('Ctrl Pts',(32.1270131204164,-3.68925702660706,-1.36303763397436));
#82443=CARTESIAN_POINT('Ctrl Pts',(32.1328080163116,-3.64942199249616,-1.47085687229595));
#82444=CARTESIAN_POINT('Ctrl Pts',(32.1386029122068,-3.60487136932325,-1.57688765259656));
#82445=CARTESIAN_POINT('Ctrl Pts',(32.144397808102,-3.55580587480623,-1.68069437456473));
#82446=CARTESIAN_POINT('Ctrl Pts',(32.1501990994925,-3.50668622950756,-1.78461566207819));
#82447=CARTESIAN_POINT('Ctrl Pts',(32.1560003908831,-3.45304194941713,-1.88630761058477));
#82448=CARTESIAN_POINT('Ctrl Pts',(32.1618016822737,-3.39511992355919,-1.98535883523645));
#82449=CARTESIAN_POINT('Ctrl Pts',(32.1676067205749,-3.33716048729706,-2.08447403462477));
#82450=CARTESIAN_POINT('Ctrl Pts',(32.1734117588761,-3.27491803530903,-2.18094476193633));
#82451=CARTESIAN_POINT('Ctrl Pts',(32.1792167971773,-3.20868197266625,-2.27438980790158));
#82452=CARTESIAN_POINT('Ctrl Pts',(32.1850305171287,-3.14234685153438,-2.36797460439998));
#82453=CARTESIAN_POINT('Ctrl Pts',(32.1908442370801,-3.07200646015585,-2.45852435822425));
#82454=CARTESIAN_POINT('Ctrl Pts',(32.1966579570314,-2.99798951063316,-2.54569202656832));
#82455=CARTESIAN_POINT('Ctrl Pts',(32.1986078978887,-2.9731639815029,-2.57492835018944));
#82456=CARTESIAN_POINT('Ctrl Pts',(32.200557838746,-2.94792515245973,-2.60378452284406));
#82457=CARTESIAN_POINT('Ctrl Pts',(32.2025077796034,-2.9222862884835,-2.63224843966927));
#82458=CARTESIAN_POINT('Ctrl Pts',(32.2083802257373,-2.84507222987714,-2.71797043359014));
#82459=CARTESIAN_POINT('Ctrl Pts',(32.2142526718712,-2.76395386205481,-2.80043558297738));
#82460=CARTESIAN_POINT('Ctrl Pts',(32.2201251180051,-2.6792367571074,-2.87926716359643));
#82461=CARTESIAN_POINT('Ctrl Pts',(32.22598995695,-2.5946293950203,-2.95799662548579));
#82462=CARTESIAN_POINT('Ctrl Pts',(32.2318547958948,-2.50643286632609,-3.03310160004337));
#82463=CARTESIAN_POINT('Ctrl Pts',(32.2377196348396,-2.41499199288139,-3.10423946794038));
#82464=CARTESIAN_POINT('Ctrl Pts',(32.2435784449597,-2.32364511707433,-3.17530420889451));
#82465=CARTESIAN_POINT('Ctrl Pts',(32.2494372550797,-2.22906085442845,-3.2424097023228));
#82466=CARTESIAN_POINT('Ctrl Pts',(32.2552960651997,-2.13161926579595,-3.30525162516979));
#82467=CARTESIAN_POINT('Ctrl Pts',(32.2613818540807,-2.03040264936802,-3.37052813481688));
#82468=CARTESIAN_POINT('Ctrl Pts',(32.2674676429617,-1.92610316804087,-3.43120372923139));
#82469=CARTESIAN_POINT('Ctrl Pts',(32.2735534318426,-1.81918297146479,-3.48698470262382));
#82470=CARTESIAN_POINT('Ctrl Pts',(32.2794054619209,-1.71636964379681,-3.5406230953568));
#82471=CARTESIAN_POINT('Ctrl Pts',(32.2852574919992,-1.61113361400549,-3.58973573285033));
#82472=CARTESIAN_POINT('Ctrl Pts',(32.2911095220774,-1.50391271236987,-3.63410725675128));
#82473=CARTESIAN_POINT('Ctrl Pts',(32.296960662456,-1.39670811181402,-3.67847203473106));
#82474=CARTESIAN_POINT('Ctrl Pts',(32.3028118028345,-1.28751962126107,-3.71809697429432));
#82475=CARTESIAN_POINT('Ctrl Pts',(32.308662943213,-1.17680569913497,-3.75281458994226));
#82476=CARTESIAN_POINT('Ctrl Pts',(32.3145146107805,-1.06608180166135,-3.78753533365462));
#82477=CARTESIAN_POINT('Ctrl Pts',(32.320366278348,-0.953832593836438,-3.81734775080719));
#82478=CARTESIAN_POINT('Ctrl Pts',(32.3262179459154,-0.840531677115653,
-3.84213423760352));
#82479=CARTESIAN_POINT('Ctrl Pts',(32.3320715575997,-0.727193118097655,
-3.86692895928734));
#82480=CARTESIAN_POINT('Ctrl Pts',(32.3379251692839,-0.612802558991906,
-3.88669434206711));
#82481=CARTESIAN_POINT('Ctrl Pts',(32.3437787809681,-0.497843064976492,
-3.90136402847194));
#82482=CARTESIAN_POINT('Ctrl Pts',(32.349639047068,-0.382752884421308,-3.91605039145118));
#82483=CARTESIAN_POINT('Ctrl Pts',(32.3554993131679,-0.267092888303129,
-3.92562944343905));
#82484=CARTESIAN_POINT('Ctrl Pts',(32.3613595792678,-0.151350629577838,
-3.93008676582673));
#82485=CARTESIAN_POINT('Ctrl Pts',(32.3672237924391,-0.0355304148425893,
-3.93454709035962));
#82486=CARTESIAN_POINT('Ctrl Pts',(32.3730880056104,0.0803717604859929,
-3.93387881873478));
#82487=CARTESIAN_POINT('Ctrl Pts',(32.3789522187817,0.195870729612114,-3.92811960832167));
#82488=CARTESIAN_POINT('Ctrl Pts',(32.384825067356,0.311539777845725,-3.9223519171284));
#82489=CARTESIAN_POINT('Ctrl Pts',(32.3906979159303,0.426804024898627,-3.911478363882));
#82490=CARTESIAN_POINT('Ctrl Pts',(32.3965707645046,0.541185701310483,-3.89558815029221));
#82491=CARTESIAN_POINT('Ctrl Pts',(32.3981655091174,0.572245511545825,-3.89127323697584));
#82492=CARTESIAN_POINT('Ctrl Pts',(32.3997602537302,0.603240317358721,-3.88658869855381));
#82493=CARTESIAN_POINT('Ctrl Pts',(32.401354998343,0.634160733601198,-3.88153695898395));
#82494=CARTESIAN_POINT('Ctrl Pts',(32.4072274444769,0.748021271123717,-3.86293456442569));
#82495=CARTESIAN_POINT('Ctrl Pts',(32.4130998906108,0.8612532219627,-3.83928682096459));
#82496=CARTESIAN_POINT('Ctrl Pts',(32.4189723367447,0.973374456375479,-3.81064707991645));
#82497=CARTESIAN_POINT('Ctrl Pts',(32.4248371756896,1.08535044851462,-3.78204443889782));
#82498=CARTESIAN_POINT('Ctrl Pts',(32.4307020146344,1.19621818873576,-3.74846276152279));
#82499=CARTESIAN_POINT('Ctrl Pts',(32.4365668535793,1.30550301389679,-3.71000685723172));
#82500=CARTESIAN_POINT('Ctrl Pts',(32.4424256636993,1.41467549853607,-3.67159048410471));
#82501=CARTESIAN_POINT('Ctrl Pts',(32.4482844738193,1.52226791707535,-3.62830998663364));
#82502=CARTESIAN_POINT('Ctrl Pts',(32.4541432839394,1.62781876745331,-3.58032052480316));
#82503=CARTESIAN_POINT('Ctrl Pts',(32.4602290728203,1.73745881013218,-3.53047188195104));
#82504=CARTESIAN_POINT('Ctrl Pts',(32.4663148617013,1.84489545852133,-3.47554214368864));
#82505=CARTESIAN_POINT('Ctrl Pts',(32.4724006505823,1.94963175564452,-3.41576126469378));
#82506=CARTESIAN_POINT('Ctrl Pts',(32.4782526806605,2.05034506874808,-3.3582766051327));
#82507=CARTESIAN_POINT('Ctrl Pts',(32.4841047107388,2.14856125604564,-3.29630682475106));
#82508=CARTESIAN_POINT('Ctrl Pts',(32.4899567408171,2.24386241685593,-3.23010378381585));
#82509=CARTESIAN_POINT('Ctrl Pts',(32.4958078811956,2.33914908877641,-3.16391080790563));
#82510=CARTESIAN_POINT('Ctrl Pts',(32.5016590215741,2.43152127600425,-3.09348608688119));
#82511=CARTESIAN_POINT('Ctrl Pts',(32.5075101619526,2.52059019508077,-3.01912471893141));
#82512=CARTESIAN_POINT('Ctrl Pts',(32.5133618295201,2.60966713928554,-2.94475665100682));
#82513=CARTESIAN_POINT('Ctrl Pts',(32.5192134970876,2.69543990635964,-2.86645149598967));
#82514=CARTESIAN_POINT('Ctrl Pts',(32.5250651646551,2.77755348578489,-2.78454406206908));
#82515=CARTESIAN_POINT('Ctrl Pts',(32.5309187763394,2.8596943460465,-2.70260941580047));
#82516=CARTESIAN_POINT('Ctrl Pts',(32.5367723880236,2.93817330880889,-2.61707040263851));
#82517=CARTESIAN_POINT('Ctrl Pts',(32.5426259997078,3.01267335528806,-2.52829750115318));
#82518=CARTESIAN_POINT('Ctrl Pts',(32.5484862658077,3.08725809380044,-2.43942368218017));
#82519=CARTESIAN_POINT('Ctrl Pts',(32.5543465319076,3.15785462188899,-2.34730895392833));
#82520=CARTESIAN_POINT('Ctrl Pts',(32.5602067980075,3.22418718561602,-2.25235565400082));
#82521=CARTESIAN_POINT('Ctrl Pts',(32.5660710111788,3.29056442638678,-2.15733840007403));
#82522=CARTESIAN_POINT('Ctrl Pts',(32.5719352243501,3.35267176328473,-2.05947911571031));
#82523=CARTESIAN_POINT('Ctrl Pts',(32.5777994375214,3.41027853937052,-1.9592062892684));
#82524=CARTESIAN_POINT('Ctrl Pts',(32.5836722860957,3.46797014486351,-1.85878580512019));
#82525=CARTESIAN_POINT('Ctrl Pts',(32.58954513467,3.52114777353984,-1.75594505144156));
#82526=CARTESIAN_POINT('Ctrl Pts',(32.5954179832442,3.56962812783369,-1.65113416443927));
#82527=CARTESIAN_POINT('Ctrl Pts',(32.597012727857,3.5827927417104,-1.62267325738612));
#82528=CARTESIAN_POINT('Ctrl Pts',(32.5986074724699,3.59561127509653,-1.5940671725533));
#82529=CARTESIAN_POINT('Ctrl Pts',(32.6002022170827,3.60808069240139,-1.56532511546973));
#82530=CARTESIAN_POINT('Ctrl Pts',(32.6060746632166,3.65399775075439,-1.45948611112614));
#82531=CARTESIAN_POINT('Ctrl Pts',(32.6119471093505,3.69533073337939,-1.35144780769194));
#82532=CARTESIAN_POINT('Ctrl Pts',(32.6178195554844,3.73186382739031,-1.24164462460713));
#82533=CARTESIAN_POINT('Ctrl Pts',(32.6236843944293,3.76834959629215,-1.13198368098376));
#82534=CARTESIAN_POINT('Ctrl Pts',(32.6295492333741,3.80004771226752,-1.02056279281366));
#82535=CARTESIAN_POINT('Ctrl Pts',(32.6354140723189,3.82678968673084,-0.907837922500752));
#82536=CARTESIAN_POINT('Ctrl Pts',(32.641272882439,3.85350417149142,-0.795228928941078));
#82537=CARTESIAN_POINT('Ctrl Pts',(32.647131692559,3.87527255357542,-0.681319019232035));
#82538=CARTESIAN_POINT('Ctrl Pts',(32.652990502679,3.8919758160551,-0.566580309613941));
#82539=CARTESIAN_POINT('Ctrl Pts',(32.65907629156,3.90932618703355,-0.447396456765771));
#82540=CARTESIAN_POINT('Ctrl Pts',(32.665162080441,3.92121089740585,-0.327318718520768));
#82541=CARTESIAN_POINT('Ctrl Pts',(32.6712478693219,3.92755467737133,-0.206889478366118));
#82542=CARTESIAN_POINT('Ctrl Pts',(32.6770998994002,3.93365478894175,-0.0910859975893578));
#82543=CARTESIAN_POINT('Ctrl Pts',(32.6829519294785,3.93463175540505,0.0250420294514206));
#82544=CARTESIAN_POINT('Ctrl Pts',(32.6888039595567,3.9304714806856,0.141006877552701));
#82545=CARTESIAN_POINT('Ctrl Pts',(32.6946550999352,3.92631183846382,0.256954095208426));
#82546=CARTESIAN_POINT('Ctrl Pts',(32.7005062403138,3.91701652281431,0.372737770273564));
#82547=CARTESIAN_POINT('Ctrl Pts',(32.7063573806923,3.90262355376715,0.487871292024686));
#82548=CARTESIAN_POINT('Ctrl Pts',(32.7122090482598,3.88822928791041,0.603015187330697));
#82549=CARTESIAN_POINT('Ctrl Pts',(32.7180607158273,3.86873650688895,0.717508402684074));
#82550=CARTESIAN_POINT('Ctrl Pts',(32.7239123833948,3.84423489651378,0.83087126585631));
#82551=CARTESIAN_POINT('Ctrl Pts',(32.729765995079,3.81972514589652,0.944271791906046));
#82552=CARTESIAN_POINT('Ctrl Pts',(32.7356196067633,3.79020334424603,1.05654081522187));
#82553=CARTESIAN_POINT('Ctrl Pts',(32.7414732184475,3.75580972613532,1.16721133522054));
#82554=CARTESIAN_POINT('Ctrl Pts',(32.7473334845474,3.72137700918388,1.27800766603159));
#82555=CARTESIAN_POINT('Ctrl Pts',(32.7531937506473,3.68206154424488,1.38720147151405));
#82556=CARTESIAN_POINT('Ctrl Pts',(32.7590540167472,3.63805267831903,1.4943432369358));
#82557=CARTESIAN_POINT('Ctrl Pts',(32.7649182299185,3.59401417105377,1.60155716566751));
#82558=CARTESIAN_POINT('Ctrl Pts',(32.7707824430898,3.54527614170624,1.70671592815627));
#82559=CARTESIAN_POINT('Ctrl Pts',(32.7766466562611,3.49207431993456,1.80939380568565));
#82560=CARTESIAN_POINT('Ctrl Pts',(32.7825195048354,3.43879415531324,1.91222288250206));
#82561=CARTESIAN_POINT('Ctrl Pts',(32.7883923534097,3.38103728490401,2.01256342629882));
#82562=CARTESIAN_POINT('Ctrl Pts',(32.794265201984,3.3190832564259,2.11001785227359));
#82563=CARTESIAN_POINT('Ctrl Pts',(32.7958599465968,3.30225992922728,2.13648114667755));
#82564=CARTESIAN_POINT('Ctrl Pts',(32.7974546912095,3.28512734792143,2.1627318141998));
#82565=CARTESIAN_POINT('Ctrl Pts',(32.7990494358223,3.2676916149064,2.18876232375066));
#82566=CARTESIAN_POINT('Ctrl Pts',(32.8049218819562,3.20348672459517,2.2846163959034));
#82567=CARTESIAN_POINT('Ctrl Pts',(32.81079432809,3.13495310760068,2.37780348622807));
#82568=CARTESIAN_POINT('Ctrl Pts',(32.8166667742239,3.06233950919108,2.46790715596178));
#82569=CARTESIAN_POINT('Ctrl Pts',(32.8225316131688,2.98981997471313,2.55789410505891));
#82570=CARTESIAN_POINT('Ctrl Pts',(32.8283964521136,2.91323122623499,2.64480525787337));
#82571=CARTESIAN_POINT('Ctrl Pts',(32.8342612910584,2.83286571989194,2.72825233676453));
#82572=CARTESIAN_POINT('Ctrl Pts',(32.8401201011784,2.75258282614324,2.8116136353254));
#82573=CARTESIAN_POINT('Ctrl Pts',(32.8459789112984,2.66853118177182,2.89151764690684));
#82574=CARTESIAN_POINT('Ctrl Pts',(32.8518377214184,2.58104358149604,2.96760897532308));
#82575=CARTESIAN_POINT('Ctrl Pts',(32.8579235102994,2.4901665853012,3.04664819163654));
#82576=CARTESIAN_POINT('Ctrl Pts',(32.8640092991804,2.39558230608856,3.12157297851322));
#82577=CARTESIAN_POINT('Ctrl Pts',(32.8700950880614,2.29770630253051,3.19202674602071));
#82578=CARTESIAN_POINT('Ctrl Pts',(32.8759471181396,2.20358977500006,3.25977434204214));
#82579=CARTESIAN_POINT('Ctrl Pts',(32.8817991482179,2.10643009924294,3.32338778821915));
#82580=CARTESIAN_POINT('Ctrl Pts',(32.8876511782961,2.00662993215558,3.38259150879578));
#82581=CARTESIAN_POINT('Ctrl Pts',(32.8935023186746,1.90684493795386,3.44178622847283));
#82582=CARTESIAN_POINT('Ctrl Pts',(32.8993534590531,1.80442060602961,3.49657234472912));
#82583=CARTESIAN_POINT('Ctrl Pts',(32.9052045994316,1.69978683548065,3.54671872495222));
#82584=CARTESIAN_POINT('Ctrl Pts',(32.9110562669991,1.59514363740686,3.59686962337476));
#82585=CARTESIAN_POINT('Ctrl Pts',(32.9169079345666,1.48829097775519,3.64237977607909));
#82586=CARTESIAN_POINT('Ctrl Pts',(32.9227596021341,1.37968085511645,3.68306526388349));
#82587=CARTESIAN_POINT('Ctrl Pts',(32.9286132138183,1.27103464861707,3.72376426874721));
#82588=CARTESIAN_POINT('Ctrl Pts',(32.9344668255026,1.16063020499076,3.7596352764898));
#82589=CARTESIAN_POINT('Ctrl Pts',(32.9403204371868,1.04893619556056,3.79054374168706));
#82590=CARTESIAN_POINT('Ctrl Pts',(32.9461807032867,0.93711521181,3.82148734378541));
#82591=CARTESIAN_POINT('Ctrl Pts',(32.9520409693866,0.824002134818662,3.84745703289744));
#82592=CARTESIAN_POINT('Ctrl Pts',(32.9579012354864,0.710077482248281,3.86836903218966));
#82593=CARTESIAN_POINT('Ctrl Pts',(32.9637654486577,0.596076097882421,3.88929511636356));
#82594=CARTESIAN_POINT('Ctrl Pts',(32.969629661829,0.481262457970925,3.90515667123887));
#82595=CARTESIAN_POINT('Ctrl Pts',(32.9754938750003,0.36612214233278,3.91592180423635));
#82596=CARTESIAN_POINT('Ctrl Pts',(32.9813667235746,0.250812275725717,3.92670278953299));
#82597=CARTESIAN_POINT('Ctrl Pts',(32.9872395721489,0.135175184620491,3.9323723547306));
#82598=CARTESIAN_POINT('Ctrl Pts',(32.9931124207232,0.0196964752109615,
3.93295067968876));
#82599=CARTESIAN_POINT('Ctrl Pts',(32.9947071653361,-0.0116612292154589,
3.93310772113123));
#82600=CARTESIAN_POINT('Ctrl Pts',(32.996301909949,-0.0430072868758966,
3.93288964572984));
#82601=CARTESIAN_POINT('Ctrl Pts',(32.9978966545618,-0.0743320629214669,
3.93229751473891));
#82602=CARTESIAN_POINT('Ctrl Pts',(33.0037691006957,-0.189681604470987,
3.93011706696041));
#82603=CARTESIAN_POINT('Ctrl Pts',(33.0096415468297,-0.305128243973245,
3.92285319132686));
#82604=CARTESIAN_POINT('Ctrl Pts',(33.0155139929636,-0.420187170315274,
3.9104899618721));
#82605=CARTESIAN_POINT('Ctrl Pts',(33.0213788319084,-0.535097048886176,
3.89814274779183));
#82606=CARTESIAN_POINT('Ctrl Pts',(33.0272436708533,-0.649619805881446,
3.88070936007733));
#82607=CARTESIAN_POINT('Ctrl Pts',(33.0331085097981,-0.763270684661763,
3.85822586974065));
#82608=CARTESIAN_POINT('Ctrl Pts',(33.0389673199181,-0.876804734788063,
3.83576549155181));
#82609=CARTESIAN_POINT('Ctrl Pts',(33.0448261300381,-0.989468286339254,
3.80826541627433));
#82610=CARTESIAN_POINT('Ctrl Pts',(33.0506849401581,-1.10078243136404,3.77581342743524));
#82611=CARTESIAN_POINT('Ctrl Pts',(33.0567707290391,-1.21640904704381,3.74210420170561));
#82612=CARTESIAN_POINT('Ctrl Pts',(33.0628565179201,-1.33057913389214,3.70305166232924));
#82613=CARTESIAN_POINT('Ctrl Pts',(33.0689423068011,-1.44276802845002,3.65881256913803));
#82614=CARTESIAN_POINT('Ctrl Pts',(33.0747943368793,-1.55064768024876,3.61627272606205));
#82615=CARTESIAN_POINT('Ctrl Pts',(33.0806463669576,-1.65669510975156,3.56893758241947));
#82616=CARTESIAN_POINT('Ctrl Pts',(33.0864983970359,-1.76046077946921,3.51699685014796));
#82617=CARTESIAN_POINT('Ctrl Pts',(33.0923495374144,-1.86421067341505,3.46506401456465));
#82618=CARTESIAN_POINT('Ctrl Pts',(33.0982006777929,-1.96567912779575,3.40852716755154));
#82619=CARTESIAN_POINT('Ctrl Pts',(33.1040518181714,-2.06443926095335,3.34762296829174));
#82620=CARTESIAN_POINT('Ctrl Pts',(33.1099034857389,-2.16320829241994,3.28671328155064));
#82621=CARTESIAN_POINT('Ctrl Pts',(33.1157551533064,-2.2592681657184,3.22143567730739));
#82622=CARTESIAN_POINT('Ctrl Pts',(33.1216068208739,-2.35221976612745,3.15207093382102));
#82623=CARTESIAN_POINT('Ctrl Pts',(33.1274604325581,-2.44520224811983,3.0826831450821));
#82624=CARTESIAN_POINT('Ctrl Pts',(33.1333140442423,-2.53507407271398,3.00920576412062));
#82625=CARTESIAN_POINT('Ctrl Pts',(33.1391676559265,-2.62146864371653,2.93196029134281));
#82626=CARTESIAN_POINT('Ctrl Pts',(33.1450279220264,-2.70796142850888,2.85462700551682));
#82627=CARTESIAN_POINT('Ctrl Pts',(33.1508881881263,-2.79096876140429,2.77351735365818));
#82628=CARTESIAN_POINT('Ctrl Pts',(33.1567484542262,-2.87016034776382,2.68899025251566));
#82629=CARTESIAN_POINT('Ctrl Pts',(33.1626126673975,-2.94940527211877,2.60440621974265));
#82630=CARTESIAN_POINT('Ctrl Pts',(33.1684768805688,-3.02482906417223,2.51640046751559));
#82631=CARTESIAN_POINT('Ctrl Pts',(33.1743410937401,-3.09614233762215,2.42536422526259));
#82632=CARTESIAN_POINT('Ctrl Pts',(33.1802139423144,-3.1675606241126,2.33419392672339));
#82633=CARTESIAN_POINT('Ctrl Pts',(33.1860867908887,-3.2348560720885,2.23998456683498));
#82634=CARTESIAN_POINT('Ctrl Pts',(33.1919596394629,-3.29778308478639,2.14315555331309));
#82635=CARTESIAN_POINT('Ctrl Pts',(33.1935543840758,-3.31487062130878,2.11686208673897));
#82636=CARTESIAN_POINT('Ctrl Pts',(33.1951491286887,-3.33163630867265,2.09037558800984));
#82637=CARTESIAN_POINT('Ctrl Pts',(33.1967438733015,-3.34807582995316,2.06370473587755));
#82638=CARTESIAN_POINT('Ctrl Pts',(33.2027912381652,-3.41041545635189,1.96256730436164));
#82639=CARTESIAN_POINT('Ctrl Pts',(33.2088386030289,-3.46825976736853,1.85845523200901));
#82640=CARTESIAN_POINT('Ctrl Pts',(33.2148859678926,-3.52132262059677,1.75179222560025));
#82641=CARTESIAN_POINT('Ctrl Pts',(33.2209239767828,-3.57430337944903,1.64529423920869));
#82642=CARTESIAN_POINT('Ctrl Pts',(33.226961985673,-3.62251723791411,1.53625351206916));
#82643=CARTESIAN_POINT('Ctrl Pts',(33.2329999945633,-3.66572201704252,1.42512143123654));
#82644=CARTESIAN_POINT('Ctrl Pts',(33.2391363681801,-3.70963064181988,1.31217890644078));
#82645=CARTESIAN_POINT('Ctrl Pts',(33.2452727417969,-3.74836531030906,1.19707660729187));
#82646=CARTESIAN_POINT('Ctrl Pts',(33.2514091154137,-3.78172039376651,1.08031470570869));
#82647=CARTESIAN_POINT('Ctrl Pts',(33.2574297674202,-3.81444645685911,0.965754735774939));
#82648=CARTESIAN_POINT('Ctrl Pts',(33.2634504194266,-3.84199391261333,0.849597585619082));
#82649=CARTESIAN_POINT('Ctrl Pts',(33.2694710714331,-3.86421710185485,0.732335435256624));
#82650=CARTESIAN_POINT('Ctrl Pts',(33.2756653058551,-3.88708101154747,0.611692480408314));
#82651=CARTESIAN_POINT('Ctrl Pts',(33.2818595402771,-3.90430882981542,0.489880217607703));
#82652=CARTESIAN_POINT('Ctrl Pts',(33.2880537746991,-3.91579739769619,0.367450323439404));
#82653=CARTESIAN_POINT('Ctrl Pts',(33.2942480091211,-3.92728596557697,0.245020429271104));
#82654=CARTESIAN_POINT('Ctrl Pts',(33.3004422435431,-3.93303519759643,0.121973337018079));
#82655=CARTESIAN_POINT('Ctrl Pts',(33.3066364779651,-3.93299983775287,-0.00112970610199267));
#82656=CARTESIAN_POINT('',(34.5566364779651,-3.93583466796628,-0.0031786779811645));
#82657=CARTESIAN_POINT('Ctrl Pts',(33.3066373091263,-3.9267941936085,-0.00114441588407893));
#82658=CARTESIAN_POINT('Ctrl Pts',(33.3362885700978,-3.92829771108111,-0.589498635609008));
#82659=CARTESIAN_POINT('Ctrl Pts',(33.4322222373162,-3.52779483796851,-2.49110991178401));
#82660=CARTESIAN_POINT('Ctrl Pts',(33.5944383107807,-0.576005850405059,
-4.61586487358942));
#82661=CARTESIAN_POINT('Ctrl Pts',(33.7932855295205,3.57145441695431,-2.98038665588391));
#82662=CARTESIAN_POINT('Ctrl Pts',(33.99213274826,4.43824979459357,1.39281371034701));
#82663=CARTESIAN_POINT('Ctrl Pts',(34.1909799669998,1.22815979920724,4.48660392485808));
#82664=CARTESIAN_POINT('Ctrl Pts',(34.3791478769013,-2.87710201293364,3.51427533050346));
#82665=CARTESIAN_POINT('Ctrl Pts',(34.5010333805565,-3.9262035401934,1.09370000885035));
#82666=CARTESIAN_POINT('Ctrl Pts',(34.5566364779651,-3.93583466796628,-0.0031786779811645));
#82667=CARTESIAN_POINT('',(35.8066364779651,-3.93429339661999,0.00268599589076086));
#82668=CARTESIAN_POINT('Ctrl Pts',(34.5566364779651,-3.93583466796628,-0.0031786779811645));
#82669=CARTESIAN_POINT('Ctrl Pts',(34.5673157868031,-3.93768445318938,-0.213848708976004));
#82670=CARTESIAN_POINT('Ctrl Pts',(34.6442775018874,-3.82634700125658,-1.7301091391965));
#82671=CARTESIAN_POINT('Ctrl Pts',(34.7875216232188,-1.85522533780729,-4.26569223184847));
#82672=CARTESIAN_POINT('Ctrl Pts',(34.9863688419583,2.58519899421029,-3.86713555895036));
#82673=CARTESIAN_POINT('Ctrl Pts',(35.1852160606979,4.65091247090342,0.0836926456322418));
#82674=CARTESIAN_POINT('Ctrl Pts',(35.3840632794377,2.44439299510388,3.95764249982663));
#82675=CARTESIAN_POINT('Ctrl Pts',(35.5829104981772,-2.00749582872452,4.19618299989382));
#82676=CARTESIAN_POINT('Ctrl Pts',(35.7237682310197,-3.85481877961169,1.63472012191788));
#82677=CARTESIAN_POINT('Ctrl Pts',(35.7983435576157,-3.93839600529667,0.166142970595259));
#82678=CARTESIAN_POINT('Ctrl Pts',(35.8066364779651,-3.93711838212695,0.00268792454698923));
#82679=CARTESIAN_POINT('',(37.056636451576,-3.93093029693069,0.00184536342784963));
#82680=CARTESIAN_POINT('Ctrl Pts',(35.8066364779651,-3.93299908341869,0.00268511224544268));
#82681=CARTESIAN_POINT('Ctrl Pts',(35.8124218483503,-3.93307685187136,-0.111225676248522));
#82682=CARTESIAN_POINT('Ctrl Pts',(35.8182072187354,-3.9282016719798,-0.225330603230136));
#82683=CARTESIAN_POINT('Ctrl Pts',(35.8239925891206,-3.91834943567708,-0.339155863769318));
#82684=CARTESIAN_POINT('Ctrl Pts',(35.8297715028224,-3.90850819482782,-0.452854091184537));
#82685=CARTESIAN_POINT('Ctrl Pts',(35.8355504165241,-3.89370097473932,-0.566272851449055));
#82686=CARTESIAN_POINT('Ctrl Pts',(35.8413293302259,-3.87395569505401,-0.67893760593928));
#82687=CARTESIAN_POINT('Ctrl Pts',(35.8471324804521,-3.85412760448416,-0.79207487173984));
#82688=CARTESIAN_POINT('Ctrl Pts',(35.8529356306784,-3.82931993226872,-0.904451358442189));
#82689=CARTESIAN_POINT('Ctrl Pts',(35.8587387809047,-3.79961374328103,-1.0155906664941));
#82690=CARTESIAN_POINT('Ctrl Pts',(35.8645102457723,-3.77006975089651,-1.12612315088873));
#82691=CARTESIAN_POINT('Ctrl Pts',(35.8702817106398,-3.73568071269343,-1.23543151752743));
#82692=CARTESIAN_POINT('Ctrl Pts',(35.8760531755074,-3.69657752796805,-1.34305754892396));
#82693=CARTESIAN_POINT('Ctrl Pts',(35.8818235341759,-3.65748183803049,-1.45066295196821));
#82694=CARTESIAN_POINT('Ctrl Pts',(35.8875938928444,-3.61367394256633,-1.55658626034691));
#82695=CARTESIAN_POINT('Ctrl Pts',(35.893364251513,-3.56533406801193,-1.66038609470011));
#82696=CARTESIAN_POINT('Ctrl Pts',(35.8991349926789,-3.51699098917224,-1.76419280959005));
#82697=CARTESIAN_POINT('Ctrl Pts',(35.9049057338448,-3.46411551493796,-1.86587538495103));
#82698=CARTESIAN_POINT('Ctrl Pts',(35.9106764750107,-3.40693493204139,-1.96501485206503));
#82699=CARTESIAN_POINT('Ctrl Pts',(35.9165038467312,-3.3491932135771,-2.06512721379367));
#82700=CARTESIAN_POINT('Ctrl Pts',(35.9223312184517,-3.28706164524794,-2.16264589458816));
#82701=CARTESIAN_POINT('Ctrl Pts',(35.9281585901722,-3.22081966464825,-2.25716851116951));
#82702=CARTESIAN_POINT('Ctrl Pts',(35.933937624766,-3.15512715079951,-2.35090707759782));
#82703=CARTESIAN_POINT('Ctrl Pts',(35.9397166593598,-3.08539247285777,-2.44169879756162));
#82704=CARTESIAN_POINT('Ctrl Pts',(35.9454956939537,-3.01192857010563,-2.52918470827685));
#82705=CARTESIAN_POINT('Ctrl Pts',(35.9513472342375,-2.93754296479728,-2.61776824632357));
#82706=CARTESIAN_POINT('Ctrl Pts',(35.9571987745213,-2.85933422874015,-2.70296212788809));
#82707=CARTESIAN_POINT('Ctrl Pts',(35.9630503148051,-2.77766451117824,-2.78443331098824));
#82708=CARTESIAN_POINT('Ctrl Pts',(35.9689018550889,-2.69599479361635,-2.86590449408837));
#82709=CARTESIAN_POINT('Ctrl Pts',(35.9747533953728,-2.61086446994547,-2.94365272926105));
#82710=CARTESIAN_POINT('Ctrl Pts',(35.9806049356566,-2.52266784757149,-3.01738892601352));
#82711=CARTESIAN_POINT('Ctrl Pts',(35.9864773817905,-2.43415612433894,-3.0913885607331));
#82712=CARTESIAN_POINT('Ctrl Pts',(35.9923498279244,-2.34223740778439,-3.16161419713871));
#82713=CARTESIAN_POINT('Ctrl Pts',(35.9982222740583,-2.2472672562383,-3.22773587504294));
#82714=CARTESIAN_POINT('Ctrl Pts',(36.0040871130032,-2.15242012938801,-3.29377189867393));
#82715=CARTESIAN_POINT('Ctrl Pts',(36.009951951948,-2.05452976444679,-3.35571430199108));
#82716=CARTESIAN_POINT('Ctrl Pts',(36.0158167908928,-1.9539857780179,-3.41327241504451));
#82717=CARTESIAN_POINT('Ctrl Pts',(36.0216756010129,-1.85354514687046,-3.47077136061129));
#82718=CARTESIAN_POINT('Ctrl Pts',(36.0275344111329,-1.75045667659687,-3.52389477621279));
#82719=CARTESIAN_POINT('Ctrl Pts',(36.033393221253,-1.64513948124863,-3.57239486720561));
#82720=CARTESIAN_POINT('Ctrl Pts',(36.0394790101339,-1.53574214573281,-3.62277392173081));
#82721=CARTESIAN_POINT('Ctrl Pts',(36.0455647990149,-1.42394027737069,-3.66816391835342));
#82722=CARTESIAN_POINT('Ctrl Pts',(36.0516505878958,-1.3102327671693,-3.70833912902203));
#82723=CARTESIAN_POINT('Ctrl Pts',(36.0575026179741,-1.20089283066499,-3.7469711857417));
#82724=CARTESIAN_POINT('Ctrl Pts',(36.0633546480524,-1.08979137137159,-3.78078152248512));
#82725=CARTESIAN_POINT('Ctrl Pts',(36.0692066781307,-0.977392174669665,
-3.80961855530111));
#82726=CARTESIAN_POINT('Ctrl Pts',(36.0750578185092,-0.86501006631765,-3.83845120394602));
#82727=CARTESIAN_POINT('Ctrl Pts',(36.0809089588877,-0.751331013131233,
-3.86231194935055));
#82728=CARTESIAN_POINT('Ctrl Pts',(36.0867600992662,-0.636832484538411,
-3.88109950743815));
#82729=CARTESIAN_POINT('Ctrl Pts',(36.0926117668337,-0.522323639604124,
-3.89988875828868));
#82730=CARTESIAN_POINT('Ctrl Pts',(36.0984634344012,-0.406995580413226,
-3.9136038462243));
#82731=CARTESIAN_POINT('Ctrl Pts',(36.1043151019687,-0.291333747170069,
-3.92219500379059));
#82732=CARTESIAN_POINT('Ctrl Pts',(36.1101687136529,-0.175633487255264,
-3.93078901562247));
#82733=CARTESIAN_POINT('Ctrl Pts',(36.1160223253372,-0.0595996447918956,
-3.93425568148592));
#82734=CARTESIAN_POINT('Ctrl Pts',(36.1218759370214,0.0562801840893303,
-3.93259730215018));
#82735=CARTESIAN_POINT('Ctrl Pts',(36.1277362031213,0.172291745751625,-3.93093703756034));
#82736=CARTESIAN_POINT('Ctrl Pts',(36.1335964692212,0.288148530812364,-3.92414010483423));
#82737=CARTESIAN_POINT('Ctrl Pts',(36.1394567353211,0.403365811098988,-3.91226085817861));
#82738=CARTESIAN_POINT('Ctrl Pts',(36.1453209484924,0.518660693805935,-3.90037361048105));
#82739=CARTESIAN_POINT('Ctrl Pts',(36.1511851616637,0.633314806177066,-3.88339729317651));
#82740=CARTESIAN_POINT('Ctrl Pts',(36.157049374835,0.746853112795433,-3.86143748206646));
#82741=CARTESIAN_POINT('Ctrl Pts',(36.1629222234093,0.860558611328997,-3.83944533382733));
#82742=CARTESIAN_POINT('Ctrl Pts',(36.1687950719836,0.973144624373589,-3.81245514161668));
#82743=CARTESIAN_POINT('Ctrl Pts',(36.1746679205579,1.08415069571401,-3.78062247109955));
#82744=CARTESIAN_POINT('Ctrl Pts',(36.1762626651707,1.11429387615108,-3.77197845803247));
#82745=CARTESIAN_POINT('Ctrl Pts',(36.1778574097834,1.14432066997479,-3.76297765027667));
#82746=CARTESIAN_POINT('Ctrl Pts',(36.1794521543962,1.17422212668442,-3.75362376873398));
#82747=CARTESIAN_POINT('Ctrl Pts',(36.1853246005301,1.28433047409437,-3.71917927833557));
#82748=CARTESIAN_POINT('Ctrl Pts',(36.191197046664,1.3931062966548,-3.67982815525321));
#82749=CARTESIAN_POINT('Ctrl Pts',(36.1970694927979,1.50007977488483,-3.63569108547213));
#82750=CARTESIAN_POINT('Ctrl Pts',(36.2029343317427,1.60691467926409,-3.59161119101919));
#82751=CARTESIAN_POINT('Ctrl Pts',(36.2087991706876,1.71195150374035,-3.54275783513725));
#82752=CARTESIAN_POINT('Ctrl Pts',(36.2146640096324,1.81473506447399,-3.48930159856791));
#82753=CARTESIAN_POINT('Ctrl Pts',(36.2205228197524,1.91741296773092,-3.43590031291708));
#82754=CARTESIAN_POINT('Ctrl Pts',(36.2263816298724,2.0178418499043,-3.37790574753603));
#82755=CARTESIAN_POINT('Ctrl Pts',(36.2322404399924,2.11558664467219,-3.31553647980001));
#82756=CARTESIAN_POINT('Ctrl Pts',(36.2383262288734,2.21711821387963,-3.25075093660465));
#82757=CARTESIAN_POINT('Ctrl Pts',(36.2444120177543,2.31575309863678,-3.18124504425275));
#82758=CARTESIAN_POINT('Ctrl Pts',(36.2504978066353,2.41103165901885,-3.10731642083789));
#82759=CARTESIAN_POINT('Ctrl Pts',(36.2563498367136,2.50265051272435,-3.03622744020958));
#82760=CARTESIAN_POINT('Ctrl Pts',(36.2622018667918,2.59116576601304,-2.96104949754691));
#82761=CARTESIAN_POINT('Ctrl Pts',(36.2680538968701,2.67619913160987,-2.88209077025179));
#82762=CARTESIAN_POINT('Ctrl Pts',(36.2739050372486,2.76121956935729,-2.80314404726261));
#82763=CARTESIAN_POINT('Ctrl Pts',(36.2797561776271,2.84275886913032,-2.7204179637272));
#82764=CARTESIAN_POINT('Ctrl Pts',(36.2856073180056,2.92047365725232,-2.63425940584736));
#82765=CARTESIAN_POINT('Ctrl Pts',(36.2914589855731,2.99819544749306,-2.54809308506333));
#82766=CARTESIAN_POINT('Ctrl Pts',(36.2973106531406,3.07209176419466,-2.45849398210059));
#82767=CARTESIAN_POINT('Ctrl Pts',(36.3031623207081,3.14185826004183,-2.36584354381412));
#82768=CARTESIAN_POINT('Ctrl Pts',(36.3090159323923,3.211647934617,-2.27316232400017));
#82769=CARTESIAN_POINT('Ctrl Pts',(36.3148695440765,3.27730481155736,-2.17742808310776));
#82770=CARTESIAN_POINT('Ctrl Pts',(36.3207231557607,3.33856717807005,-2.07905223539799));
#82771=CARTESIAN_POINT('Ctrl Pts',(36.3265834218606,3.39989918795403,-1.98056455352187));
#82772=CARTESIAN_POINT('Ctrl Pts',(36.3324436879605,3.45682649751959,-1.87942962204603));
#82773=CARTESIAN_POINT('Ctrl Pts',(36.3383039540603,3.50913273252388,-1.77608458850628));
#82774=CARTESIAN_POINT('Ctrl Pts',(36.3441681672316,3.56147419740369,-1.67266994887332));
#82775=CARTESIAN_POINT('Ctrl Pts',(36.3500323804029,3.60918822048394,-1.56704261891427));
#82776=CARTESIAN_POINT('Ctrl Pts',(36.3558965935742,3.65210675655598,-1.45965928857324));
#82777=CARTESIAN_POINT('Ctrl Pts',(36.3617694421485,3.69508849272728,-1.3521178298859));
#82778=CARTESIAN_POINT('Ctrl Pts',(36.3676422907228,3.73326051248998,-1.24281559881976));
#82779=CARTESIAN_POINT('Ctrl Pts',(36.3735151392971,3.76650470567798,-1.13222405119554));
#82780=CARTESIAN_POINT('Ctrl Pts',(36.37510988391,3.77553201113743,-1.10219343273561));
#82781=CARTESIAN_POINT('Ctrl Pts',(36.3767046285229,3.7841962462906,-1.07206779719081));
#82782=CARTESIAN_POINT('Ctrl Pts',(36.3782993731358,3.79249570156589,-1.04185668573188));
#82783=CARTESIAN_POINT('Ctrl Pts',(36.3841718192697,3.8230574000663,-0.930608073727307));
#82784=CARTESIAN_POINT('Ctrl Pts',(36.3900442654036,3.84877108558446,-0.817827326972223));
#82785=CARTESIAN_POINT('Ctrl Pts',(36.3959167115375,3.86948424404304,-0.703974917949945));
#82786=CARTESIAN_POINT('Ctrl Pts',(36.4017815504824,3.89017057059735,-0.59026999377152));
#82787=CARTESIAN_POINT('Ctrl Pts',(36.4076463894272,3.90586917863183,-0.475496570964712));
#82788=CARTESIAN_POINT('Ctrl Pts',(36.4135112283721,3.91647743962409,-0.36012978898659));
#82789=CARTESIAN_POINT('Ctrl Pts',(36.4193700384921,3.92707479573938,-0.244881599543646));
#82790=CARTESIAN_POINT('Ctrl Pts',(36.4252288486121,3.93259217527238,-0.129041673302607));
#82791=CARTESIAN_POINT('Ctrl Pts',(36.4310876587321,3.93297820264459,-0.0130941789565775));
#82792=CARTESIAN_POINT('Ctrl Pts',(36.4371734476131,3.93337918527441,0.107345288684975));
#82793=CARTESIAN_POINT('Ctrl Pts',(36.4432592364941,3.9282431011739,0.227900380667051));
#82794=CARTESIAN_POINT('Ctrl Pts',(36.449345025375,3.91757177732272,0.348023518637074));
#82795=CARTESIAN_POINT('Ctrl Pts',(36.4551970554533,3.90731034542402,0.463532654797463));
#82796=CARTESIAN_POINT('Ctrl Pts',(36.4610490855316,3.89193109368867,0.578641958261));
#82797=CARTESIAN_POINT('Ctrl Pts',(36.4669011156098,3.87148871989132,0.692866575723123));
#82798=CARTESIAN_POINT('Ctrl Pts',(36.4727522559883,3.85104945400259,0.807073827311895));
#82799=CARTESIAN_POINT('Ctrl Pts',(36.4786033963668,3.8255486693858,0.920396253550279));
#82800=CARTESIAN_POINT('Ctrl Pts',(36.4844545367454,3.79509250414324,1.03235744051942));
#82801=CARTESIAN_POINT('Ctrl Pts',(36.4903062043129,3.76463359479376,1.14432871521516));
#82802=CARTESIAN_POINT('Ctrl Pts',(36.4961578718804,3.72921852576281,1.25493810794196));
#82803=CARTESIAN_POINT('Ctrl Pts',(36.5020095394479,3.68900360983545,1.363723346805));
#82804=CARTESIAN_POINT('Ctrl Pts',(36.5078631511321,3.64877533318805,1.47254472770855));
#82805=CARTESIAN_POINT('Ctrl Pts',(36.5137167628164,3.6037441819966,1.57954036215897));
#82806=CARTESIAN_POINT('Ctrl Pts',(36.5195703745006,3.55411473081814,1.68426763911841));
#82807=CARTESIAN_POINT('Ctrl Pts',(36.5254306406005,3.50442886062639,1.78911397058059));
#82808=CARTESIAN_POINT('Ctrl Pts',(36.5312909067004,3.4501344339106,1.89168642383512));
#82809=CARTESIAN_POINT('Ctrl Pts',(36.5371511728003,3.39148218730608,1.99156661279144));
#82810=CARTESIAN_POINT('Ctrl Pts',(36.5430153859716,3.33279043658988,2.09151407416047));
#82811=CARTESIAN_POINT('Ctrl Pts',(36.5488795991429,3.26973524588477,2.18876531455354));
#82812=CARTESIAN_POINT('Ctrl Pts',(36.5547438123142,3.2026099230778,2.28293203591426));
#82813=CARTESIAN_POINT('Ctrl Pts',(36.5606166608885,3.13538575423729,2.37723742337755));
#82814=CARTESIAN_POINT('Ctrl Pts',(36.5664895094628,3.06407974506618,2.4684489021776));
#82815=CARTESIAN_POINT('Ctrl Pts',(36.572362358037,2.98902462502732,2.55621219600023));
#82816=CARTESIAN_POINT('Ctrl Pts',(36.5739571026498,2.96864375757753,2.58004390871256));
#82817=CARTESIAN_POINT('Ctrl Pts',(36.5755518472626,2.94798664507684,2.60362158015751));
#82818=CARTESIAN_POINT('Ctrl Pts',(36.5771465918754,2.92706038926025,2.62693861321951));
#82819=CARTESIAN_POINT('Ctrl Pts',(36.5830190380094,2.8500020884632,2.71280065003746));
#82820=CARTESIAN_POINT('Ctrl Pts',(36.5888914841433,2.76903357199705,2.79541293606631));
#82821=CARTESIAN_POINT('Ctrl Pts',(36.5947639302772,2.68445972749625,2.87439819291809));
#82822=CARTESIAN_POINT('Ctrl Pts',(36.6006287692221,2.59999544027558,2.95328113196745));
#82823=CARTESIAN_POINT('Ctrl Pts',(36.6064936081669,2.51193541201003,3.02854610588567));
#82824=CARTESIAN_POINT('Ctrl Pts',(36.6123584471118,2.42062384195347,3.09984986987538));
#82825=CARTESIAN_POINT('Ctrl Pts',(36.6182172572318,2.32940613661575,3.17108033638751));
#82826=CARTESIAN_POINT('Ctrl Pts',(36.6240760673519,2.23494386165567,3.23835743946063));
#82827=CARTESIAN_POINT('Ctrl Pts',(36.6299348774719,2.13761652479249,3.30137616653027));
#82828=CARTESIAN_POINT('Ctrl Pts',(36.6360206663529,2.03651858641248,3.36683633005071));
#82829=CARTESIAN_POINT('Ctrl Pts',(36.6421064552338,1.9323294351303,3.42770118294426));
#82830=CARTESIAN_POINT('Ctrl Pts',(36.6481922441148,1.82551068660393,3.48367618086051));
#82831=CARTESIAN_POINT('Ctrl Pts',(36.6540442741931,1.7227949103051,3.53750114551896));
#82832=CARTESIAN_POINT('Ctrl Pts',(36.6598963042713,1.61764821924696,3.58680476087673));
#82833=CARTESIAN_POINT('Ctrl Pts',(36.6657483343496,1.51050805199816,3.63137087404313));
#82834=CARTESIAN_POINT('Ctrl Pts',(36.6715994747282,1.40338417355473,3.67593021170447));
#82835=CARTESIAN_POINT('Ctrl Pts',(36.6774506151067,1.29426780308131,3.71575332056582));
#82836=CARTESIAN_POINT('Ctrl Pts',(36.6833017554852,1.18361709417196,3.75067188306094));
#82837=CARTESIAN_POINT('Ctrl Pts',(36.6891534230527,1.07295641561064,3.78559359172583));
#82838=CARTESIAN_POINT('Ctrl Pts',(36.6950050906202,0.960761518014698,3.81560975116161));
#82839=CARTESIAN_POINT('Ctrl Pts',(36.7008567581877,0.847505788546212,3.84060189792963));
#82840=CARTESIAN_POINT('Ctrl Pts',(36.706710369872,0.734212431792843,3.86560234791224));
#82841=CARTESIAN_POINT('Ctrl Pts',(36.7125639815563,0.61985794578722,3.88557537721353));
#82842=CARTESIAN_POINT('Ctrl Pts',(36.7184175932405,0.504925274437549,3.90045375145433));
#82843=CARTESIAN_POINT('Ctrl Pts',(36.7242778593404,0.389861947040513,3.9153490395069));
#82844=CARTESIAN_POINT('Ctrl Pts',(36.7301381254403,0.274219532560922,3.92513805950056));
#82845=CARTESIAN_POINT('Ctrl Pts',(36.7359983915402,0.15848555697376,3.92980550768492));
#82846=CARTESIAN_POINT('Ctrl Pts',(36.7418626047115,0.0426736309558888,
3.93447609954074));
#82847=CARTESIAN_POINT('Ctrl Pts',(36.7477268178829,-0.0732295666226823,
3.93401825249274));
#82848=CARTESIAN_POINT('Ctrl Pts',(36.7535910310542,-0.188738801397796,
3.92846874301514));
#82849=CARTESIAN_POINT('Ctrl Pts',(36.7594638796285,-0.304418130397105,
3.92291106155448));
#82850=CARTESIAN_POINT('Ctrl Pts',(36.7653367282028,-0.419701928710933,
3.91224679152824));
#82851=CARTESIAN_POINT('Ctrl Pts',(36.7712095767771,-0.534112265718246,
3.89656426709599));
#82852=CARTESIAN_POINT('Ctrl Pts',(36.7728043213897,-0.565179858602923,
3.89230575080096));
#82853=CARTESIAN_POINT('Ctrl Pts',(36.7743990660025,-0.596183118236474,
3.88767749199223));
#82854=CARTESIAN_POINT('Ctrl Pts',(36.7759938106151,-0.627112655085652,
3.88268189758464));
#82855=CARTESIAN_POINT('Ctrl Pts',(36.7818662567491,-0.741006778099209,
3.86428625051241));
#82856=CARTESIAN_POINT('Ctrl Pts',(36.787738702883,-0.854281475430034,3.84084412163663));
#82857=CARTESIAN_POINT('Ctrl Pts',(36.7936111490169,-0.966454521269314,
3.81240798686579));
#82858=CARTESIAN_POINT('Ctrl Pts',(36.7994759879617,-1.07848225771788,3.78400868837222));
#82859=CARTESIAN_POINT('Ctrl Pts',(36.8053408269066,-1.18941078364758,3.7506283496673));
#82860=CARTESIAN_POINT('Ctrl Pts',(36.8112056658514,-1.29876524641428,3.71237091825513));
#82861=CARTESIAN_POINT('Ctrl Pts',(36.8170644759715,-1.40800729707499,3.6741528139845));
#82862=CARTESIAN_POINT('Ctrl Pts',(36.8229232860915,-1.51567811518661,3.63106772473424));
#82863=CARTESIAN_POINT('Ctrl Pts',(36.8287820962115,-1.62131591775133,3.58326997236409));
#82864=CARTESIAN_POINT('Ctrl Pts',(36.8348678850925,-1.73104628126997,3.5336204660736));
#82865=CARTESIAN_POINT('Ctrl Pts',(36.8409536739735,-1.83858247899382,3.47888587242603));
#82866=CARTESIAN_POINT('Ctrl Pts',(36.8470394628544,-1.94342713727684,3.41929524348161));
#82867=CARTESIAN_POINT('Ctrl Pts',(36.8528914929327,-2.04424464932306,3.36199352635236));
#82868=CARTESIAN_POINT('Ctrl Pts',(36.858743523011,-2.14257318253464,3.30020216219617));
#82869=CARTESIAN_POINT('Ctrl Pts',(36.8645955530892,-2.23799437965998,3.23417225215515));
#82870=CARTESIAN_POINT('Ctrl Pts',(36.8704466934677,-2.33340106964617,3.16815238081751));
#82871=CARTESIAN_POINT('Ctrl Pts',(36.8762978338463,-2.42590096258857,3.09789548001554));
#82872=CARTESIAN_POINT('Ctrl Pts',(36.8821489742248,-2.51510473991064,3.02369594160508));
#82873=CARTESIAN_POINT('Ctrl Pts',(36.8880006417923,-2.60431655451206,2.9494897178004));
#82874=CARTESIAN_POINT('Ctrl Pts',(36.8938523093598,-2.6902313453144,2.87134041457043));
#82875=CARTESIAN_POINT('Ctrl Pts',(36.8997039769273,-2.77249349453142,2.78958219502149));
#82876=CARTESIAN_POINT('Ctrl Pts',(36.9055575886117,-2.85478297394511,2.70779681269794));
#82877=CARTESIAN_POINT('Ctrl Pts',(36.911411200296,-2.93341710571831,2.62240042114911));
#82878=CARTESIAN_POINT('Ctrl Pts',(36.9172648119803,-3.00807819897582,2.53376292277837));
#82879=CARTESIAN_POINT('Ctrl Pts',(36.9231250780802,-3.08282416734458,2.44502466084783));
#82880=CARTESIAN_POINT('Ctrl Pts',(36.9289853441801,-3.15358781581915,2.35303825427781));
#82881=CARTESIAN_POINT('Ctrl Pts',(36.93484561028,-3.22009266046172,2.25820553936982));
#82882=CARTESIAN_POINT('Ctrl Pts',(36.9407098234513,-3.28664229818494,2.16330895167979));
#82883=CARTESIAN_POINT('Ctrl Pts',(36.9465740366226,-3.34892719885407,2.06556258611286));
#82884=CARTESIAN_POINT('Ctrl Pts',(36.9524382497939,-3.40671592797793,1.96539451155778));
#82885=CARTESIAN_POINT('Ctrl Pts',(36.9583110983682,-3.46458975444535,1.86507893355034));
#82886=CARTESIAN_POINT('Ctrl Pts',(36.9641839469425,-3.51795400559901,1.76233489475654));
#82887=CARTESIAN_POINT('Ctrl Pts',(36.9700567955168,-3.56662456694096,1.65761219785968));
#82888=CARTESIAN_POINT('Ctrl Pts',(36.9716515401294,-3.57984083065237,1.62917523842059));
#82889=CARTESIAN_POINT('Ctrl Pts',(36.9732462847421,-3.59271127801773,1.6005924731228));
#82890=CARTESIAN_POINT('Ctrl Pts',(36.9748410293548,-3.60523285673848,1.57187310196888));
#82891=CARTESIAN_POINT('Ctrl Pts',(36.9816573132758,-3.65875279656022,1.44912028859335));
#82892=CARTESIAN_POINT('Ctrl Pts',(36.9884735971968,-3.70605617844956,1.32349986733078));
#82893=CARTESIAN_POINT('Ctrl Pts',(36.9952898811179,-3.74685935742616,1.19563119550639));
#82894=CARTESIAN_POINT('Ctrl Pts',(37.0017475223055,-3.78551565346634,1.07449040804119));
#82895=CARTESIAN_POINT('Ctrl Pts',(37.0082051634932,-3.81833803639176,0.951332193712651));
#82896=CARTESIAN_POINT('Ctrl Pts',(37.0146628046808,-3.84513250844753,0.826707319720848));
#82897=CARTESIAN_POINT('Ctrl Pts',(37.0211026152414,-3.87185299648597,0.702426555843145));
#82898=CARTESIAN_POINT('Ctrl Pts',(37.027542425802,-3.89257868793019,0.576687462732061));
#82899=CARTESIAN_POINT('Ctrl Pts',(37.0339822363626,-3.90716502540595,0.450056067889892));
#82900=CARTESIAN_POINT('Ctrl Pts',(37.0403956793402,-3.92169163962408,0.32394316094311));
#82901=CARTESIAN_POINT('Ctrl Pts',(37.0468091223177,-3.93012896942495,0.196945499472617));
#82902=CARTESIAN_POINT('Ctrl Pts',(37.0532225652953,-3.93238344128207,0.0696381413490412));
#82903=CARTESIAN_POINT('Ctrl Pts',(37.0543605223326,-3.93278345920136,0.0470496027761474));
#82904=CARTESIAN_POINT('Ctrl Pts',(37.05549847937,-3.93298895303553,0.024451349141318));
#82905=CARTESIAN_POINT('Ctrl Pts',(37.0566364364073,-3.93299956648052,0.00184663587889645));
#82906=CARTESIAN_POINT('',(38.3066365073438,-3.93243957318768,-0.00337961949426096));
#82907=CARTESIAN_POINT('Ctrl Pts',(37.0566364779651,-3.92733035500781,0.00184314972404838));
#82908=CARTESIAN_POINT('Ctrl Pts',(37.0956537346748,-3.92406703883986,-0.772091625719316));
#82909=CARTESIAN_POINT('Ctrl Pts',(37.2009533976313,-3.32801601167788,-2.86542164041253));
#82910=CARTESIAN_POINT('Ctrl Pts',(37.372535466834,0.0794706818914165,-4.65098652778712));
#82911=CARTESIAN_POINT('Ctrl Pts',(37.5713826855737,3.95542193811241,-2.44798459195364));
#82912=CARTESIAN_POINT('Ctrl Pts',(37.7702299043133,4.19800360272441,2.00368585922314));
#82913=CARTESIAN_POINT('Ctrl Pts',(37.969077123053,0.58438512629953,4.61481151241442));
#82914=CARTESIAN_POINT('Ctrl Pts',(38.1478793142703,-3.14764932441101,3.15097279315654));
#82915=CARTESIAN_POINT('Ctrl Pts',(38.2603990992409,-3.92290543832594,0.912003963472055));
#82916=CARTESIAN_POINT('Ctrl Pts',(38.3066364779651,-3.930349927301,-0.00337724190769125));
#82917=CARTESIAN_POINT('',(39.5566364779651,-3.93546570744218,-0.000396427527168986));
#82918=CARTESIAN_POINT('Ctrl Pts',(38.3066365152026,-3.93299854740284,-0.00338025549177386));
#82919=CARTESIAN_POINT('Ctrl Pts',(38.3136694315384,-3.93287880190695,-0.142706665141453));
#82920=CARTESIAN_POINT('Ctrl Pts',(38.3207023478743,-3.92535182945411,-0.281710047409065));
#82921=CARTESIAN_POINT('Ctrl Pts',(38.3277352642102,-3.9105430525726,-0.419692785232426));
#82922=CARTESIAN_POINT('Ctrl Pts',(38.3348606654883,-3.89553953586925,-0.559490037110306));
#82923=CARTESIAN_POINT('Ctrl Pts',(38.3419860667664,-3.87306150665475,-0.698239609978886));
#82924=CARTESIAN_POINT('Ctrl Pts',(38.3491114680445,-3.84328850131442,-0.835237987440902));
#82925=CARTESIAN_POINT('Ctrl Pts',(38.3549981655405,-3.81869133560515,-0.948420105061101));
#82926=CARTESIAN_POINT('Ctrl Pts',(38.3608848630364,-3.78911601011755,-1.06040738142393));
#82927=CARTESIAN_POINT('Ctrl Pts',(38.3667715605323,-3.75468813833344,-1.17081423968885));
#82928=CARTESIAN_POINT('Ctrl Pts',(38.3726440066662,-3.72034361448153,-1.28095380918857));
#82929=CARTESIAN_POINT('Ctrl Pts',(38.3785164528001,-3.68109125034966,-1.38976530845056));
#82930=CARTESIAN_POINT('Ctrl Pts',(38.384388898934,-3.6370513053883,-1.49677880863316));
#82931=CARTESIAN_POINT('Ctrl Pts',(38.3902537378789,-3.59306840993928,-1.60365368312023));
#82932=CARTESIAN_POINT('Ctrl Pts',(38.3961185768237,-3.54431042279645,-1.70873481161991));
#82933=CARTESIAN_POINT('Ctrl Pts',(38.4019834157685,-3.49094751143177,-1.81156685563309));
#82934=CARTESIAN_POINT('Ctrl Pts',(38.4078422258886,-3.43763945505075,-1.91429319233101));
#82935=CARTESIAN_POINT('Ctrl Pts',(38.4137010360086,-3.37973607925242,-2.01477467848436));
#82936=CARTESIAN_POINT('Ctrl Pts',(38.4195598461286,-3.31745556638457,-2.11257604953385));
#82937=CARTESIAN_POINT('Ctrl Pts',(38.4256456350095,-3.25276221654935,-2.21416638686929));
#82938=CARTESIAN_POINT('Ctrl Pts',(38.4317314238905,-3.18334588999762,-2.31286432590927));
#82939=CARTESIAN_POINT('Ctrl Pts',(38.4378172127715,-3.10950378745594,-2.40820995675153));
#82940=CARTESIAN_POINT('Ctrl Pts',(38.4436692428497,-3.038498004382,-2.49989330470076));
#82941=CARTESIAN_POINT('Ctrl Pts',(38.449521272928,-2.9634004436228,-2.588476765323));
#82942=CARTESIAN_POINT('Ctrl Pts',(38.4553733030063,-2.88451893905781,-2.67358177174681));
#82943=CARTESIAN_POINT('Ctrl Pts',(38.4612244433848,-2.80564942705857,-2.75867383942926));
#82944=CARTESIAN_POINT('Ctrl Pts',(38.4670755837633,-2.72299739601975,-2.84028820133775));
#82945=CARTESIAN_POINT('Ctrl Pts',(38.4729267241418,-2.63690942029811,-2.91808116904638));
#82946=CARTESIAN_POINT('Ctrl Pts',(38.4787783917093,-2.55081368803153,-2.99588114591796));
#82947=CARTESIAN_POINT('Ctrl Pts',(38.4846300592768,-2.46128170237478,-3.06985876698141));
#82948=CARTESIAN_POINT('Ctrl Pts',(38.4904817268443,-2.36869463375025,-3.13970933878325));
#82949=CARTESIAN_POINT('Ctrl Pts',(38.4963353385285,-2.27607680465157,-3.20958311724603));
#82950=CARTESIAN_POINT('Ctrl Pts',(38.5021889502127,-2.18040220412883,-3.27532687119829));
#82951=CARTESIAN_POINT('Ctrl Pts',(38.5080425618969,-2.0820820087003,-3.3366785144881));
#82952=CARTESIAN_POINT('Ctrl Pts',(38.5139028279968,-1.9836500423715,-3.39809990263931));
#82953=CARTESIAN_POINT('Ctrl Pts',(38.5197630940967,-1.88256682910686,-3.45511899536387));
#82954=CARTESIAN_POINT('Ctrl Pts',(38.5256233601966,-1.77926931984543,-3.50751902168139));
#82955=CARTESIAN_POINT('Ctrl Pts',(38.5314875733679,-1.67590223650006,-3.55995434104572));
#82956=CARTESIAN_POINT('Ctrl Pts',(38.5373517865392,-1.57031826311682,-3.6077642291169));
#82957=CARTESIAN_POINT('Ctrl Pts',(38.5432159997104,-1.46297393690635,-3.65078022618902));
#82958=CARTESIAN_POINT('Ctrl Pts',(38.5490888482847,-1.35547153978527,-3.69385956687759));
#82959=CARTESIAN_POINT('Ctrl Pts',(38.554961696859,-1.24620400492513,-3.7321307915044));
#82960=CARTESIAN_POINT('Ctrl Pts',(38.5608345454333,-1.13564268073632,-3.76547536198154));
#82961=CARTESIAN_POINT('Ctrl Pts',(38.5624292900462,-1.10562026931021,-3.77452992442493));
#82962=CARTESIAN_POINT('Ctrl Pts',(38.564024034659,-1.07550251125637,-3.78322150296472));
#82963=CARTESIAN_POINT('Ctrl Pts',(38.5656187792719,-1.04529894618971,-3.79154837936887));
#82964=CARTESIAN_POINT('Ctrl Pts',(38.5714912254058,-0.93407812282038,-3.82221105272282));
#82965=CARTESIAN_POINT('Ctrl Pts',(38.5773636715397,-0.82132076448187,-3.84802710590822));
#82966=CARTESIAN_POINT('Ctrl Pts',(38.5832361176736,-0.707487205021032,
-3.86884360691041));
#82967=CARTESIAN_POINT('Ctrl Pts',(38.5891009566184,-0.593801105986399,
-3.88963314213796));
#82968=CARTESIAN_POINT('Ctrl Pts',(38.5949657955633,-0.479041981094081,
-3.90543593084494));
#82969=CARTESIAN_POINT('Ctrl Pts',(38.6008306345081,-0.363684876442936,
-3.91614891323692));
#82970=CARTESIAN_POINT('Ctrl Pts',(38.6066894446281,-0.248446354379057,
-3.92685088310242));
#82971=CARTESIAN_POINT('Ctrl Pts',(38.6125482547481,-0.132611484342829,
-3.93247341563584));
#82972=CARTESIAN_POINT('Ctrl Pts',(38.6184070648681,-0.0166643881909874,
-3.93296469576911));
#82973=CARTESIAN_POINT('Ctrl Pts',(38.6244928537491,0.10377466582988,-3.93347500880389));
#82974=CARTESIAN_POINT('Ctrl Pts',(38.6305786426301,0.224334370491517,-3.92844836234927));
#82975=CARTESIAN_POINT('Ctrl Pts',(38.6366644315111,0.344467146008484,-3.91788608631246));
#82976=CARTESIAN_POINT('Ctrl Pts',(38.6425164615893,0.459985549531777,-3.90772951363615));
#82977=CARTESIAN_POINT('Ctrl Pts',(38.6483684916676,0.575108766293744,-3.89245476027826));
#82978=CARTESIAN_POINT('Ctrl Pts',(38.6542205217458,0.689351893536949,-3.87211608385867));
#82979=CARTESIAN_POINT('Ctrl Pts',(38.6600716621243,0.803577652092602,-3.85178049958234));
#82980=CARTESIAN_POINT('Ctrl Pts',(38.6659228025028,0.916923180325123,-3.82638259545112));
#82981=CARTESIAN_POINT('Ctrl Pts',(38.6717739428814,1.02891196816364,-3.79602807705233));
#82982=CARTESIAN_POINT('Ctrl Pts',(38.6776256104488,1.14091084621557,-3.76567082370504));
#82983=CARTESIAN_POINT('Ctrl Pts',(38.6834772780163,1.25155234188126,-3.73035617645139));
#82984=CARTESIAN_POINT('Ctrl Pts',(38.6893289455838,1.3603740415613,-3.69024002837839));
#82985=CARTESIAN_POINT('Ctrl Pts',(38.6951825572681,1.46923189539491,-3.65011055239946));
#82986=CARTESIAN_POINT('Ctrl Pts',(38.7010361689523,1.57626836340257,-3.60517654650915));
#82987=CARTESIAN_POINT('Ctrl Pts',(38.7068897806365,1.68104064902344,-3.555642183394));
#82988=CARTESIAN_POINT('Ctrl Pts',(38.7127500467364,1.78593204031363,-3.50605150936191));
#82989=CARTESIAN_POINT('Ctrl Pts',(38.7186103128363,1.88855373781312,-3.45185021656064));
#82990=CARTESIAN_POINT('Ctrl Pts',(38.7244705789361,1.98848712799414,-3.3932886617265));
#82991=CARTESIAN_POINT('Ctrl Pts',(38.7303347921074,2.08848782642049,-3.33468766386443));
#82992=CARTESIAN_POINT('Ctrl Pts',(38.7361990052788,2.18579626595397,-3.27172078027991));
#82993=CARTESIAN_POINT('Ctrl Pts',(38.7420632184501,2.28002388244395,-3.20468096625627));
#82994=CARTESIAN_POINT('Ctrl Pts',(38.7479360670243,2.37439025470839,-3.13754243211574));
#82995=CARTESIAN_POINT('Ctrl Pts',(38.7538089155986,2.46566642493059,-3.06631925078858));
#82996=CARTESIAN_POINT('Ctrl Pts',(38.7596817641729,2.55349781490262,-2.99134383000141));
#82997=CARTESIAN_POINT('Ctrl Pts',(38.7612765087858,2.57734801880756,-2.97098460451037));
#82998=CARTESIAN_POINT('Ctrl Pts',(38.7628712533987,2.60094443231498,-2.95034890347279));
#82999=CARTESIAN_POINT('Ctrl Pts',(38.7644659980115,2.62428045186533,-2.92944382263213));
#83000=CARTESIAN_POINT('Ctrl Pts',(38.7703384441454,2.71021240403054,-2.8524634960201));
#83001=CARTESIAN_POINT('Ctrl Pts',(38.7762108902794,2.79289815629724,-2.77157000534445));
#83002=CARTESIAN_POINT('Ctrl Pts',(38.7820833364133,2.87196015366701,-2.68706789563438));
#83003=CARTESIAN_POINT('Ctrl Pts',(38.7879481753581,2.95091973382448,-2.60267525027884));
#83004=CARTESIAN_POINT('Ctrl Pts',(38.793813014303,3.02626461442448,-2.51468358110271));
#83005=CARTESIAN_POINT('Ctrl Pts',(38.7996778532478,3.09765123835948,-2.42343677563289));
#83006=CARTESIAN_POINT('Ctrl Pts',(38.8055366633678,3.1689644796399,-2.33228376830675));
#83007=CARTESIAN_POINT('Ctrl Pts',(38.8113954734878,3.23632730441255,-2.23788260397548));
#83008=CARTESIAN_POINT('Ctrl Pts',(38.8172542836079,3.29943435573531,-2.14061251332266));
#83009=CARTESIAN_POINT('Ctrl Pts',(38.8233400724888,3.36498626531822,-2.03957403895337));
#83010=CARTESIAN_POINT('Ctrl Pts',(38.8294258613698,3.42594567225829,-1.9354401814996));
#83011=CARTESIAN_POINT('Ctrl Pts',(38.8355116502508,3.48201761328852,-1.82867228905251));
#83012=CARTESIAN_POINT('Ctrl Pts',(38.841363680329,3.53593579741771,-1.72600541542057));
#83013=CARTESIAN_POINT('Ctrl Pts',(38.8472157104073,3.58533484080514,-1.62090352371436));
#83014=CARTESIAN_POINT('Ctrl Pts',(38.8530677404856,3.62999819355835,-1.51380385610658));
#83015=CARTESIAN_POINT('Ctrl Pts',(38.8589188808641,3.67465475602281,-1.40672047114714));
#83016=CARTESIAN_POINT('Ctrl Pts',(38.8647700212426,3.71457690035054,-1.29764029560235));
#83017=CARTESIAN_POINT('Ctrl Pts',(38.8706211616211,3.74959589314948,-1.18702133008491));
#83018=CARTESIAN_POINT('Ctrl Pts',(38.8764728291886,3.78461804116707,-1.0763923977753));
#83019=CARTESIAN_POINT('Ctrl Pts',(38.8823244967561,3.81473603468499,-0.964224793983947));
#83020=CARTESIAN_POINT('Ctrl Pts',(38.8881761643236,3.83983098058972,-0.850991798141068));
#83021=CARTESIAN_POINT('Ctrl Pts',(38.8940297760078,3.8649342638622,-0.737721182566711));
#83022=CARTESIAN_POINT('Ctrl Pts',(38.8998833876921,3.88501109177934,-0.623384874467584));
#83023=CARTESIAN_POINT('Ctrl Pts',(38.9057369993763,3.89999379159077,-0.508465756519987));
#83024=CARTESIAN_POINT('Ctrl Pts',(38.9115972654762,3.91499352381185,-0.393415997932268));
#83025=CARTESIAN_POINT('Ctrl Pts',(38.9174575315761,3.92488751575212,-0.277782517216073));
#83026=CARTESIAN_POINT('Ctrl Pts',(38.9233177976759,3.92966002110912,-0.162052826253335));
#83027=CARTESIAN_POINT('Ctrl Pts',(38.9291820108472,3.93443574089685,-0.0462451877456786));
#83028=CARTESIAN_POINT('Ctrl Pts',(38.9350462240186,3.9340831067468,0.0696583776954723));
#83029=CARTESIAN_POINT('Ctrl Pts',(38.9409104371899,3.9286384546399,0.185172602521538));
#83030=CARTESIAN_POINT('Ctrl Pts',(38.9467832857641,3.92318578495866,0.300856928920133));
#83031=CARTESIAN_POINT('Ctrl Pts',(38.9526561343384,3.91262616976747,0.416150360371662));
#83032=CARTESIAN_POINT('Ctrl Pts',(38.9585289829127,3.89704750934145,0.530574886265481));
#83033=CARTESIAN_POINT('Ctrl Pts',(38.9601237275255,3.89281719683212,0.561646332078223));
#83034=CARTESIAN_POINT('Ctrl Pts',(38.9617184721383,3.88821708356199,0.592653780305154));
#83035=CARTESIAN_POINT('Ctrl Pts',(38.9633132167512,3.88324956792143,0.623587839231974));
#83036=CARTESIAN_POINT('Ctrl Pts',(38.9691856628851,3.86495731737279,0.737498614218898));
#83037=CARTESIAN_POINT('Ctrl Pts',(38.975058109019,3.8416180248077,0.850794544791016));
#83038=CARTESIAN_POINT('Ctrl Pts',(38.9809305551529,3.813283728366,0.962993357702474));
#83039=CARTESIAN_POINT('Ctrl Pts',(38.9867953940978,3.78498613627976,1.07504682784463));
#83040=CARTESIAN_POINT('Ctrl Pts',(38.9926602330426,3.75170650821108,1.18600560952804));
#83041=CARTESIAN_POINT('Ctrl Pts',(38.9985250719875,3.71354836056725,1.29539475594441));
#83042=CARTESIAN_POINT('Ctrl Pts',(39.0043838821075,3.67542943800527,1.40467145460097));
#83043=CARTESIAN_POINT('Ctrl Pts',(39.0102426922275,3.63244210616119,1.51238133942785));
#83044=CARTESIAN_POINT('Ctrl Pts',(39.0161015023476,3.58474026764131,1.61806248752972));
#83045=CARTESIAN_POINT('Ctrl Pts',(39.0221872912285,3.53519039104206,1.7278378758543));
#83046=CARTESIAN_POINT('Ctrl Pts',(39.0282730801095,3.48055343739693,1.83542371534555));
#83047=CARTESIAN_POINT('Ctrl Pts',(39.0343588689905,3.42105800717408,1.94032242463723));
#83048=CARTESIAN_POINT('Ctrl Pts',(39.0402108990688,3.3638478321263,2.04119191156059));
#83049=CARTESIAN_POINT('Ctrl Pts',(39.046062929147,3.30214575249688,2.13957649621314));
#83050=CARTESIAN_POINT('Ctrl Pts',(39.0519149592253,3.23620248955498,2.2350575935752));
#83051=CARTESIAN_POINT('Ctrl Pts',(39.0577660996038,3.17026925214336,2.33052417469116));
#83052=CARTESIAN_POINT('Ctrl Pts',(39.0636172399824,3.10009634832847,2.42308780618229));
#83053=CARTESIAN_POINT('Ctrl Pts',(39.0694683803609,3.02597781643561,2.51235890239423));
#83054=CARTESIAN_POINT('Ctrl Pts',(39.0753200479284,2.95185260644735,2.60163804195083));
#83055=CARTESIAN_POINT('Ctrl Pts',(39.0811717154959,2.8737813257401,2.68762373845095));
#83056=CARTESIAN_POINT('Ctrl Pts',(39.0870233830634,2.79209781446559,2.76996007091374));
#83057=CARTESIAN_POINT('Ctrl Pts',(39.0928769947477,2.71038716523769,2.85232375821863));
#83058=CARTESIAN_POINT('Ctrl Pts',(39.0987306064319,2.6250621900807,2.93103537733209));
#83059=CARTESIAN_POINT('Ctrl Pts',(39.1045842181162,2.53649250285734,3.00577690172583));
#83060=CARTESIAN_POINT('Ctrl Pts',(39.1104444842161,2.44782212916132,3.08060339266612));
#83061=CARTESIAN_POINT('Ctrl Pts',(39.116304750316,2.35589999715888,3.15145051390063));
#83062=CARTESIAN_POINT('Ctrl Pts',(39.1221650164159,2.26112769200391,3.21804141683308));
#83063=CARTESIAN_POINT('Ctrl Pts',(39.1280292295872,2.16629155475493,3.28467717080899));
#83064=CARTESIAN_POINT('Ctrl Pts',(39.1338934427585,2.06860176942996,3.34705077641272));
#83065=CARTESIAN_POINT('Ctrl Pts',(39.1397576559298,1.96848619465356,3.4049304106631));
#83066=CARTESIAN_POINT('Ctrl Pts',(39.1456305045041,1.86822319373349,3.46289527612043));
#83067=CARTESIAN_POINT('Ctrl Pts',(39.1515033530784,1.7655276393991,3.51635277259045));
#83068=CARTESIAN_POINT('Ctrl Pts',(39.1573762016527,1.66084916701591,3.56511837733652));
#83069=CARTESIAN_POINT('Ctrl Pts',(39.1589709462654,1.63242421653601,3.57836044964108));
#83070=CARTESIAN_POINT('Ctrl Pts',(39.1605656908781,1.60385314633796,3.59125683809931));
#83071=CARTESIAN_POINT('Ctrl Pts',(39.1621604354908,1.57514515364979,3.60380448206248));
#83072=CARTESIAN_POINT('Ctrl Pts',(39.1680328816248,1.46943158714517,3.65000960023234));
#83073=CARTESIAN_POINT('Ctrl Pts',(39.1739053277587,1.36150624594712,3.69163664899737));
#83074=CARTESIAN_POINT('Ctrl Pts',(39.1797777738926,1.25180296016412,3.72846863322254));
#83075=CARTESIAN_POINT('Ctrl Pts',(39.1856426128374,1.14224178443512,3.76525290515514));
#83076=CARTESIAN_POINT('Ctrl Pts',(39.1915074517823,1.03090763252803,3.7972543347504));
#83077=CARTESIAN_POINT('Ctrl Pts',(39.1973722907271,0.918256006313075,3.82430319233059));
#83078=CARTESIAN_POINT('Ctrl Pts',(39.2032311008471,0.8057201815594,3.85132424474419));
#83079=CARTESIAN_POINT('Ctrl Pts',(39.2090899109672,0.691869975818573,3.8734027555914));
#83080=CARTESIAN_POINT('Ctrl Pts',(39.2149487210872,0.57717717946286,3.89041842267735));
#83081=CARTESIAN_POINT('Ctrl Pts',(39.2210345099681,0.458041018623016,3.90809330126746));
#83082=CARTESIAN_POINT('Ctrl Pts',(39.2271202988491,0.337996091133369,3.92030497382628));
#83083=CARTESIAN_POINT('Ctrl Pts',(39.2332060877301,0.217584573488528,3.92697669376581));
#83084=CARTESIAN_POINT('Ctrl Pts',(39.2390581178084,0.101798134489563,3.93339214893908));
#83085=CARTESIAN_POINT('Ctrl Pts',(39.2449101478866,-0.0143268013692517,
3.9346853618356));
#83086=CARTESIAN_POINT('Ctrl Pts',(39.2507621779649,-0.13030254908064,3.93084090821583));
#83087=CARTESIAN_POINT('Ctrl Pts',(39.2566133183434,-0.246260664689525,
3.92699703907861));
#83088=CARTESIAN_POINT('Ctrl Pts',(39.2624644587219,-0.362069224231788,
3.91801707018397));
#83089=CARTESIAN_POINT('Ctrl Pts',(39.2683155991004,-0.477241515248946,
3.9039376962399));
#83090=CARTESIAN_POINT('Ctrl Pts',(39.2741672666679,-0.592424183313889,
3.88985705374126));
#83091=CARTESIAN_POINT('Ctrl Pts',(39.2800189342354,-0.706970058563911,
3.87067614299513));
#83092=CARTESIAN_POINT('Ctrl Pts',(39.2858706018029,-0.820399226308901,
3.84648334319437));
#83093=CARTESIAN_POINT('Ctrl Pts',(39.2917242134871,-0.933866078960063,
3.82228250574855));
#83094=CARTESIAN_POINT('Ctrl Pts',(39.2975778251714,-1.04621508233125,3.79306655444722));
#83095=CARTESIAN_POINT('Ctrl Pts',(39.3034314368556,-1.15697885567182,3.75897445156632));
#83096=CARTESIAN_POINT('Ctrl Pts',(39.3092917029555,-1.26786854583558,3.72484359260877));
#83097=CARTESIAN_POINT('Ctrl Pts',(39.3151519690554,-1.37716901374189,3.68582563963176));
#83098=CARTESIAN_POINT('Ctrl Pts',(39.3210122351553,-1.48443023067911,3.64210871477582));
#83099=CARTESIAN_POINT('Ctrl Pts',(39.3268764483266,-1.59176369138076,3.59836234521179));
#83100=CARTESIAN_POINT('Ctrl Pts',(39.3327406614979,-1.69705479161216,3.54991087418261));
#83101=CARTESIAN_POINT('Ctrl Pts',(39.3386048746692,-1.7998771722758,3.49698887111762));
#83102=CARTESIAN_POINT('Ctrl Pts',(39.3444777232435,-1.90285096501586,3.44398893725272));
#83103=CARTESIAN_POINT('Ctrl Pts',(39.3503505718177,-2.00334842532305,3.38650553720828));
#83104=CARTESIAN_POINT('Ctrl Pts',(39.356223420392,-2.10097120858039,3.32481713492882));
#83105=CARTESIAN_POINT('Ctrl Pts',(39.3578181650048,-2.12748021961938,3.30806593728376));
#83106=CARTESIAN_POINT('Ctrl Pts',(39.3594129096176,-2.15377744675309,3.291004907634));
#83107=CARTESIAN_POINT('Ctrl Pts',(39.3610076542304,-2.17985534230117,3.27364012784561));
#83108=CARTESIAN_POINT('Ctrl Pts',(39.3668637167746,-2.27561599646785,3.20987491071258));
#83109=CARTESIAN_POINT('Ctrl Pts',(39.3727197793188,-2.3687411492821,3.14179459873242));
#83110=CARTESIAN_POINT('Ctrl Pts',(39.378575841863,-2.45881502679421,3.06964455010852));
#83111=CARTESIAN_POINT('Ctrl Pts',(39.384424307879,-2.54877205979722,2.99758809506854));
#83112=CARTESIAN_POINT('Ctrl Pts',(39.390272773895,-2.63568536628193,2.92147265832977));
#83113=CARTESIAN_POINT('Ctrl Pts',(39.3961212399109,-2.71916709477171,2.8415874631464));
#83114=CARTESIAN_POINT('Ctrl Pts',(39.4019637069651,-2.80256319333762,2.76178420880572));
#83115=CARTESIAN_POINT('Ctrl Pts',(39.4078061740193,-2.88253441563955,2.67821917217045));
#83116=CARTESIAN_POINT('Ctrl Pts',(39.4136486410735,-2.95872559837939,2.5912220733651));
#83117=CARTESIAN_POINT('Ctrl Pts',(39.4196064676106,-3.03642117564412,2.5025072172758));
#83118=CARTESIAN_POINT('Ctrl Pts',(39.4255642941478,-3.11018551207959,2.41022360207101));
#83119=CARTESIAN_POINT('Ctrl Pts',(39.4315221206849,-3.17968092376429,2.31476094295922));
#83120=CARTESIAN_POINT('Ctrl Pts',(39.4373579629526,-3.2477534428941,2.22125284607863));
#83121=CARTESIAN_POINT('Ctrl Pts',(39.4431938052203,-3.31172992496697,2.1246949964004));
#83122=CARTESIAN_POINT('Ctrl Pts',(39.4490296474881,-3.37133394785222,2.02548670991917));
#83123=CARTESIAN_POINT('Ctrl Pts',(39.4548646521831,-3.43092941623973,1.92629266202487));
#83124=CARTESIAN_POINT('Ctrl Pts',(39.4606996568782,-3.48615345896569,1.82444929010516));
#83125=CARTESIAN_POINT('Ctrl Pts',(39.4665346615733,-3.53677396329765,1.72038336789792));
#83126=CARTESIAN_POINT('Ctrl Pts',(39.4723702626728,-3.58739964162599,1.61630680895937));
#83127=CARTESIAN_POINT('Ctrl Pts',(39.4782058637723,-3.63342066444593,1.51000762231545));
#83128=CARTESIAN_POINT('Ctrl Pts',(39.4840414648718,-3.67465203776792,1.40193487770584));
#83129=CARTESIAN_POINT('Ctrl Pts',(39.4900910492962,-3.71739530784309,1.28989925680764));
#83130=CARTESIAN_POINT('Ctrl Pts',(39.4961406337207,-3.75499075718299,1.17595796659253));
#83131=CARTESIAN_POINT('Ctrl Pts',(39.5021902181451,-3.78728840254579,1.06062979212455));
#83132=CARTESIAN_POINT('Ctrl Pts',(39.5080346078133,-3.81849054993651,0.949213413078005));
#83133=CARTESIAN_POINT('Ctrl Pts',(39.5138789974814,-3.8447484187838,0.83650313148381));
#83134=CARTESIAN_POINT('Ctrl Pts',(39.5197233871496,-3.86597893184856,0.722977107869293));
#83135=CARTESIAN_POINT('Ctrl Pts',(39.5258755689522,-3.88832754026671,0.603472287647107));
#83136=CARTESIAN_POINT('Ctrl Pts',(39.5320277507548,-3.90510478510686,0.483064001120986));
#83137=CARTESIAN_POINT('Ctrl Pts',(39.5381799325573,-3.91627592610257,0.3623146017337));
#83138=CARTESIAN_POINT('Ctrl Pts',(39.5443321143599,-3.92744706709828,0.241565202346451));
#83139=CARTESIAN_POINT('Ctrl Pts',(39.5504842961625,-3.93301215567005,0.120475222334223));
#83140=CARTESIAN_POINT('Ctrl Pts',(39.5566364779651,-3.93299998004603,-0.000396179149394312));
#83141=CARTESIAN_POINT('',(40.806636477965,-3.93299837325538,0.00357714558460698));
#83142=CARTESIAN_POINT('Ctrl Pts',(39.5566364779651,-3.93946210749301,-0.000396830092737622));
#83143=CARTESIAN_POINT('Ctrl Pts',(39.5577092763001,-3.93949232068474,-0.0215086434630096));
#83144=CARTESIAN_POINT('Ctrl Pts',(39.5587820746351,-3.93933734594436,-0.0426200010628439));
#83145=CARTESIAN_POINT('Ctrl Pts',(39.6261372792166,-3.91789589192311,-1.36789847410651));
#83146=CARTESIAN_POINT('Ctrl Pts',(39.7587020917098,-2.45157417157785,-3.95319811699279));
#83147=CARTESIAN_POINT('Ctrl Pts',(39.9575493104495,1.99987423861761,-4.19982074625295));
#83148=CARTESIAN_POINT('Ctrl Pts',(40.156396529189,4.61427912745781,-0.588574043643822));
#83149=CARTESIAN_POINT('Ctrl Pts',(40.3552437479286,2.99010170290171,3.56332472239632));
#83150=CARTESIAN_POINT('Ctrl Pts',(40.5540909666685,-1.38072191342157,4.44202636965956));
#83151=CARTESIAN_POINT('Ctrl Pts',(40.7045549800519,-3.72834198752477,2.01939489233835));
#83152=CARTESIAN_POINT('Ctrl Pts',(40.7887365871891,-3.93466605613737,0.357674737801762));
#83153=CARTESIAN_POINT('Ctrl Pts',(40.8066357880796,-3.9315453160497,0.00358947132840354));
#83154=CARTESIAN_POINT('',(42.0566368090547,-3.93068341693143,-0.00121071286382613));
#83155=CARTESIAN_POINT('Ctrl Pts',(40.806636477965,-3.93299837325538,0.00357714558460698));
#83156=CARTESIAN_POINT('Ctrl Pts',(40.8126843498893,-3.93310722773962,-0.116106132406968));
#83157=CARTESIAN_POINT('Ctrl Pts',(40.8187322218136,-3.92774801925936,-0.235913693313374));
#83158=CARTESIAN_POINT('Ctrl Pts',(40.8247800937378,-3.91691839487931,-0.355301685692745));
#83159=CARTESIAN_POINT('Ctrl Pts',(40.8305766403865,-3.90653880620868,-0.469728392439114));
#83160=CARTESIAN_POINT('Ctrl Pts',(40.8363731870352,-3.89113439964223,-0.583769238264932));
#83161=CARTESIAN_POINT('Ctrl Pts',(40.8421697336839,-3.87075626857845,-0.696946848232061));
#83162=CARTESIAN_POINT('Ctrl Pts',(40.8479650293874,-3.85038253529231,-0.810100033488199));
#83163=CARTESIAN_POINT('Ctrl Pts',(40.853760325091,-3.82503728550107,-0.922389937950088));
#83164=CARTESIAN_POINT('Ctrl Pts',(40.8595556207946,-3.79482309977436,-1.03334729951693));
#83165=CARTESIAN_POINT('Ctrl Pts',(40.8653511347839,-3.7646077759996,-1.14430884040567));
#83166=CARTESIAN_POINT('Ctrl Pts',(40.8711466487731,-3.72952326321698,-1.25393733151824));
#83167=CARTESIAN_POINT('Ctrl Pts',(40.8769421627624,-3.68972237107758,-1.36177745038228));
#83168=CARTESIAN_POINT('Ctrl Pts',(40.8827393641702,-3.64990989053348,-1.46964896791285));
#83169=CARTESIAN_POINT('Ctrl Pts',(40.888536565578,-3.60537844794011,-1.57573068271518));
#83170=CARTESIAN_POINT('Ctrl Pts',(40.8943337669858,-3.55632914848002,-1.67958685029127));
#83171=CARTESIAN_POINT('Ctrl Pts',(40.90013741641,-3.50722529326646,-1.7835585333087));
#83172=CARTESIAN_POINT('Ctrl Pts',(40.9059410658343,-3.45359373354725,-1.88529934734926));
#83173=CARTESIAN_POINT('Ctrl Pts',(40.9117447152585,-3.39568172111523,-1.98439780509955));
#83174=CARTESIAN_POINT('Ctrl Pts',(40.9175521771462,-3.33773166582208,-2.08356136141415));
#83175=CARTESIAN_POINT('Ctrl Pts',(40.9233596390339,-3.27549579008755,-2.18007875340368));
#83176=CARTESIAN_POINT('Ctrl Pts',(40.9291671009215,-3.20926383555447,-2.27356870004014));
#83177=CARTESIAN_POINT('Ctrl Pts',(40.9349831988458,-3.14293339021857,-2.36719767171316));
#83178=CARTESIAN_POINT('Ctrl Pts',(40.9407992967701,-3.07259526719338,-2.45778988360377));
#83179=CARTESIAN_POINT('Ctrl Pts',(40.9466153946944,-2.99857846943249,-2.54499826378249));
#83180=CARTESIAN_POINT('Ctrl Pts',(40.9483387311788,-2.97664695285533,-2.57083850671945));
#83181=CARTESIAN_POINT('Ctrl Pts',(40.9500620676632,-2.9543926983173,-2.59638191712149));
#83182=CARTESIAN_POINT('Ctrl Pts',(40.9517854041476,-2.9318248420384,-2.62162012801369));
#83183=CARTESIAN_POINT('Ctrl Pts',(40.9576578502815,-2.85492255304568,-2.70762192471537));
#83184=CARTESIAN_POINT('Ctrl Pts',(40.9635302964155,-2.77410415481936,-2.79038107508411));
#83185=CARTESIAN_POINT('Ctrl Pts',(40.9694027425494,-2.68967384953248,-2.86951974782212));
#83186=CARTESIAN_POINT('Ctrl Pts',(40.9752675814942,-2.60535291558434,-2.94855590402233));
#83187=CARTESIAN_POINT('Ctrl Pts',(40.9811324204391,-2.51742967800563,-3.02398062921735));
#83188=CARTESIAN_POINT('Ctrl Pts',(40.9869972593839,-2.42624771231289,-3.09545005427264));
#83189=CARTESIAN_POINT('Ctrl Pts',(40.992856069504,-2.33515947811122,-3.1668460115569));
#83190=CARTESIAN_POINT('Ctrl Pts',(40.998714879624,-2.24081950219823,-3.23429450251988));
#83191=CARTESIAN_POINT('Ctrl Pts',(41.004573689744,-2.14360673790931,-3.29748982609345));
#83192=CARTESIAN_POINT('Ctrl Pts',(41.010659478625,-2.04262781081007,-3.36313342772154));
#83193=CARTESIAN_POINT('Ctrl Pts',(41.0167452675059,-1.93854933299478,-3.42418733847521));
#83194=CARTESIAN_POINT('Ctrl Pts',(41.0228310563869,-1.83183238460756,-3.48035617641399));
#83195=CARTESIAN_POINT('Ctrl Pts',(41.0286830864652,-1.72921449824348,-3.53436753558338));
#83196=CARTESIAN_POINT('Ctrl Pts',(41.0345351165435,-1.62415749249673,-3.58386196629385));
#83197=CARTESIAN_POINT('Ctrl Pts',(41.0403871466217,-1.51709841278372,-3.62862252182961));
#83198=CARTESIAN_POINT('Ctrl Pts',(41.0462382870002,-1.41005560954835,-3.67337627229866));
#83199=CARTESIAN_POINT('Ctrl Pts',(41.0520894273788,-1.30101171881765,-3.71339741919552));
#83200=CARTESIAN_POINT('Ctrl Pts',(41.0579405677573,-1.19042458784561,-3.74851681344137));
#83201=CARTESIAN_POINT('Ctrl Pts',(41.0637922353248,-1.07982749294963,-3.78363937195207));
#83202=CARTESIAN_POINT('Ctrl Pts',(41.0696439028923,-0.967687275392694,
-3.81385917473373));
#83203=CARTESIAN_POINT('Ctrl Pts',(41.0754955704598,-0.854477106483174,
-3.83905689909594));
#83204=CARTESIAN_POINT('Ctrl Pts',(41.081349182144,-0.741229325426693,-3.86426299497214));
#83205=CARTESIAN_POINT('Ctrl Pts',(41.0872027938282,-0.626911289451086,
-3.88444360496097));
#83206=CARTESIAN_POINT('Ctrl Pts',(41.0930564055124,-0.512005819602848,
-3.89953061799658));
#83207=CARTESIAN_POINT('Ctrl Pts',(41.0989166716123,-0.396969724629124,
-3.91463478202574));
#83208=CARTESIAN_POINT('Ctrl Pts',(41.1047769377122,-0.281345272962014,
-3.92463373775944));
#83209=CARTESIAN_POINT('Ctrl Pts',(41.1106372038121,-0.165619961988667,
-3.92951129635619));
#83210=CARTESIAN_POINT('Ctrl Pts',(41.1165014169834,-0.049816706420237,
-3.93439214014029));
#83211=CARTESIAN_POINT('Ctrl Pts',(41.1223656301548,0.0660871313754274,
-3.93414471917854));
#83212=CARTESIAN_POINT('Ctrl Pts',(41.1282298433261,0.181606251065211,-3.92880492892865));
#83213=CARTESIAN_POINT('Ctrl Pts',(41.1341026919004,0.297295479535092,-3.92345727551976));
#83214=CARTESIAN_POINT('Ctrl Pts',(41.1399755404747,0.412598449118441,-3.91300232386485));
#83215=CARTESIAN_POINT('Ctrl Pts',(41.145848389049,0.527037069608885,-3.89752754028218));
#83216=CARTESIAN_POINT('Ctrl Pts',(41.1474431336617,0.558112342742973,-3.89332543504479));
#83217=CARTESIAN_POINT('Ctrl Pts',(41.1490378782745,0.58912395400931,-3.8887534711043));
#83218=CARTESIAN_POINT('Ctrl Pts',(41.1506326228873,0.620062509520288,-3.88381403832462));
#83219=CARTESIAN_POINT('Ctrl Pts',(41.1565050690212,0.73398984261351,-3.8656251993731));
#83220=CARTESIAN_POINT('Ctrl Pts',(41.1623775151551,0.84730691306653,-3.84238876235125));
#83221=CARTESIAN_POINT('Ctrl Pts',(41.168249961289,0.959531400593865,-3.81415632758732));
#83222=CARTESIAN_POINT('Ctrl Pts',(41.1741148002338,1.0716105120929,-3.78596046522684));
#83223=CARTESIAN_POINT('Ctrl Pts',(41.1799796391787,1.18259945809538,-3.75278157521827));
#83224=CARTESIAN_POINT('Ctrl Pts',(41.1858444781235,1.29202319802029,-3.71472274278679));
#83225=CARTESIAN_POINT('Ctrl Pts',(41.1917032882435,1.40133445462451,-3.67670303334505));
#83226=CARTESIAN_POINT('Ctrl Pts',(41.1975620983635,1.50908331740957,-3.63381349433048));
#83227=CARTESIAN_POINT('Ctrl Pts',(41.2034209084835,1.6148077239633,-3.58620760896918));
#83228=CARTESIAN_POINT('Ctrl Pts',(41.2095066973645,1.7246280466353,-3.53675740289205));
#83229=CARTESIAN_POINT('Ctrl Pts',(41.2155924862454,1.83226343923973,-3.48221813427216));
#83230=CARTESIAN_POINT('Ctrl Pts',(41.2216782751264,1.93721611310014,-3.4228179517972));
#83231=CARTESIAN_POINT('Ctrl Pts',(41.2275303052047,2.03813749178024,-3.36569936597445));
#83232=CARTESIAN_POINT('Ctrl Pts',(41.2333823352829,2.13657804680104,-3.3040866217169));
#83233=CARTESIAN_POINT('Ctrl Pts',(41.2392343653612,2.23211896571971,-3.23823006021413));
#83234=CARTESIAN_POINT('Ctrl Pts',(41.2450855057397,2.32764535929759,-3.17238351106008));
#83235=CARTESIAN_POINT('Ctrl Pts',(41.2509366461182,2.42027265306176,-3.10229466205746));
#83236=CARTESIAN_POINT('Ctrl Pts',(41.2567877864967,2.50961099460106,-3.02825719775871));
#83237=CARTESIAN_POINT('Ctrl Pts',(41.2626394540642,2.59895738554353,-2.95421306266904));
#83238=CARTESIAN_POINT('Ctrl Pts',(41.2684911216317,2.68501391688605,-2.87621986881838));
#83239=CARTESIAN_POINT('Ctrl Pts',(41.2743427891991,2.76742436474649,-2.79461113312881));
#83240=CARTESIAN_POINT('Ctrl Pts',(41.2801964008834,2.84986219207291,-2.71297528432845));
#83241=CARTESIAN_POINT('Ctrl Pts',(41.2860500125676,2.92865123366631,-2.62772179587343));
#83242=CARTESIAN_POINT('Ctrl Pts',(41.2919036242519,3.00347312760742,-2.53921999278127));
#83243=CARTESIAN_POINT('Ctrl Pts',(41.2977638903517,3.07838007945944,-2.45061758038765));
#83244=CARTESIAN_POINT('Ctrl Pts',(41.3036241564516,3.14931061507326,-2.35875979870026));
#83245=CARTESIAN_POINT('Ctrl Pts',(41.3094844225515,3.21598752142227,-2.26404798139444));
#83246=CARTESIAN_POINT('Ctrl Pts',(41.3153486357228,3.28270933674064,-2.16927237273514));
#83247=CARTESIAN_POINT('Ctrl Pts',(41.321212848894,3.34517159588094,-2.07163924815229));
#83248=CARTESIAN_POINT('Ctrl Pts',(41.3270770620653,3.403142087563,-1.97157625565368));
#83249=CARTESIAN_POINT('Ctrl Pts',(41.3329499106396,3.46119794424507,-1.8713659144418));
#83250=CARTESIAN_POINT('Ctrl Pts',(41.3388227592139,3.51474864198052,-1.76871892919217));
#83251=CARTESIAN_POINT('Ctrl Pts',(41.3446956077882,3.56360924994612,-1.664084767582));
#83252=CARTESIAN_POINT('Ctrl Pts',(41.3462903524011,3.57687711993312,-1.63567184948201));
#83253=CARTESIAN_POINT('Ctrl Pts',(41.347885097014,3.5897994388583,-1.6071124979248));
#83254=CARTESIAN_POINT('Ctrl Pts',(41.3494798416269,3.60237313772528,-1.57841590735628));
#83255=CARTESIAN_POINT('Ctrl Pts',(41.3553522877608,3.64867419979032,-1.47274432773401));
#83256=CARTESIAN_POINT('Ctrl Pts',(41.3612247338948,3.69039920210543,-1.36485681852462));
#83257=CARTESIAN_POINT('Ctrl Pts',(41.3670971800287,3.72733075580979,-1.25518701267757));
#83258=CARTESIAN_POINT('Ctrl Pts',(41.3729620189735,3.764214468239,-1.14565927351416));
#83259=CARTESIAN_POINT('Ctrl Pts',(41.3788268579184,3.79631694974478,-1.03435421721276));
#83260=CARTESIAN_POINT('Ctrl Pts',(41.3846916968632,3.82346805723129,-0.921727191381479));
#83261=CARTESIAN_POINT('Ctrl Pts',(41.3905505069833,3.85059125444227,-0.809215941723395));
#83262=CARTESIAN_POINT('Ctrl Pts',(41.3964093171033,3.87277310527054,-0.695385824960153));
#83263=CARTESIAN_POINT('Ctrl Pts',(41.4022681272233,3.88989287929663,-0.580708522063683));
#83264=CARTESIAN_POINT('Ctrl Pts',(41.4083539161043,3.90767589807999,-0.461588454922284));
#83265=CARTESIAN_POINT('Ctrl Pts',(41.4144397049853,3.91999653802832,-0.341554662205697));
#83266=CARTESIAN_POINT('Ctrl Pts',(41.4205254938662,3.92677756041714,-0.221149250517372));
#83267=CARTESIAN_POINT('Ctrl Pts',(41.4263775239445,3.93329811966705,-0.105368682941397));
#83268=CARTESIAN_POINT('Ctrl Pts',(41.4322295540228,3.9346967460258,0.0107550311402793));
#83269=CARTESIAN_POINT('Ctrl Pts',(41.438081584101,3.93095757255749,0.126734220922879));
#83270=CARTESIAN_POINT('Ctrl Pts',(41.4439327244795,3.9272189675657,0.242695778079594));
#83271=CARTESIAN_POINT('Ctrl Pts',(41.449783864858,3.91834412917111,0.358512441595939));
#83272=CARTESIAN_POINT('Ctrl Pts',(41.4556350052365,3.9043693102467,0.473697465903849));
#83273=CARTESIAN_POINT('Ctrl Pts',(41.461486672804,3.89039323218815,0.58889286840678));
#83274=CARTESIAN_POINT('Ctrl Pts',(41.4673383403715,3.87131630992616,0.703456108195251));
#83275=CARTESIAN_POINT('Ctrl Pts',(41.473190007939,3.84722648696806,0.816907190549473));
#83276=CARTESIAN_POINT('Ctrl Pts',(41.4790436196232,3.82312866057726,0.930395965090257));
#83277=CARTESIAN_POINT('Ctrl Pts',(41.4848972313074,3.79401470765438,1.04277144334969));
#83278=CARTESIAN_POINT('Ctrl Pts',(41.4907508429916,3.76002316614685,1.15356611862479));
#83279=CARTESIAN_POINT('Ctrl Pts',(41.4966111090915,3.7259929828812,1.26448674585297));
#83280=CARTESIAN_POINT('Ctrl Pts',(41.5024713751914,3.68707426497149,1.37382258780479));
#83281=CARTESIAN_POINT('Ctrl Pts',(41.5083316412913,3.64345472596101,1.48112344518355));
#83282=CARTESIAN_POINT('Ctrl Pts',(41.5141958544626,3.59980580783481,1.5884965730259));
#83283=CARTESIAN_POINT('Ctrl Pts',(41.5200600676339,3.55144993620144,1.69383161235954));
#83284=CARTESIAN_POINT('Ctrl Pts',(41.5259242808052,3.49862129336033,1.79670199132903));
#83285=CARTESIAN_POINT('Ctrl Pts',(41.5317971293795,3.44571485719775,1.8997238530554));
#83286=CARTESIAN_POINT('Ctrl Pts',(41.5376699779538,3.38832270877834,2.00027345329677));
#83287=CARTESIAN_POINT('Ctrl Pts',(41.5435428265281,3.32672295032909,2.09795219482087));
#83288=CARTESIAN_POINT('Ctrl Pts',(41.5451375711409,3.30999582350222,2.12447640106608));
#83289=CARTESIAN_POINT('Ctrl Pts',(41.5467323157537,3.29295867254856,2.1507891047475));
#83290=CARTESIAN_POINT('Ctrl Pts',(41.5483270603665,3.27561757248019,2.17688275266699));
#83291=CARTESIAN_POINT('Ctrl Pts',(41.5541995065005,3.2117611560756,2.27296932390479));
#83292=CARTESIAN_POINT('Ctrl Pts',(41.5600719526344,3.14356635758723,2.36640464870643));
#83293=CARTESIAN_POINT('Ctrl Pts',(41.5659443987683,3.07128040853467,2.45677138784852));
#83294=CARTESIAN_POINT('Ctrl Pts',(41.5718092377132,2.99908809897565,2.54702106557277));
#83295=CARTESIAN_POINT('Ctrl Pts',(41.577674076658,2.92281543388061,2.63420974279851));
#83296=CARTESIAN_POINT('Ctrl Pts',(41.5835389156029,2.8427534576025,2.71794808252274));
#83297=CARTESIAN_POINT('Ctrl Pts',(41.5893977257229,2.76277378190151,2.80160034251215));
#83298=CARTESIAN_POINT('Ctrl Pts',(41.5952565358429,2.67901282685052,2.8818090228245));
#83299=CARTESIAN_POINT('Ctrl Pts',(41.601115345963,2.59180209451376,2.95821752122357));
#83300=CARTESIAN_POINT('Ctrl Pts',(41.6072011348439,2.50121269252215,3.03758619514228));
#83301=CARTESIAN_POINT('Ctrl Pts',(41.6132869237249,2.4069010922651,3.1128539280669));
#83302=CARTESIAN_POINT('Ctrl Pts',(41.6193727126059,2.30928155488068,3.18366262350266));
#83303=CARTESIAN_POINT('Ctrl Pts',(41.6252247426841,2.21541164250376,3.25175151445801));
#83304=CARTESIAN_POINT('Ctrl Pts',(41.6310767727624,2.11848359066862,3.31571733263689));
#83305=CARTESIAN_POINT('Ctrl Pts',(41.6369288028407,2.0188990529887,3.37528304203386));
#83306=CARTESIAN_POINT('Ctrl Pts',(41.6427799432192,1.91932965541181,3.43483969549706));
#83307=CARTESIAN_POINT('Ctrl Pts',(41.6486310835977,1.81710492966494,3.48999735816178));
#83308=CARTESIAN_POINT('Ctrl Pts',(41.6544822239763,1.71265393275851,3.5405233379554));
#83309=CARTESIAN_POINT('Ctrl Pts',(41.6603338915438,1.60819352479486,3.59105387015062));
#83310=CARTESIAN_POINT('Ctrl Pts',(41.6661855591113,1.50150681905239,3.63695170987969));
#83311=CARTESIAN_POINT('Ctrl Pts',(41.6720372266788,1.39304514332302,3.67803129794516));
#83312=CARTESIAN_POINT('Ctrl Pts',(41.6778908383631,1.28454743305186,3.71912453400308));
#83313=CARTESIAN_POINT('Ctrl Pts',(41.6837444500474,1.17427396655959,3.75539618900909));
#83314=CARTESIAN_POINT('Ctrl Pts',(41.6895980617316,1.06269292353887,3.78671001665831));
#83315=CARTESIAN_POINT('Ctrl Pts',(41.6954583278315,0.950985034619151,3.81805944202657));
#83316=CARTESIAN_POINT('Ctrl Pts',(41.7013185939314,0.837967000464165,3.84443967884929));
#83317=CARTESIAN_POINT('Ctrl Pts',(41.7071788600313,0.724119031370313,3.865765206063));
#83318=CARTESIAN_POINT('Ctrl Pts',(41.7130430732026,0.610194382129835,3.88710509668228));
#83319=CARTESIAN_POINT('Ctrl Pts',(41.7189072863739,0.495439093153907,3.90338344072787));
#83320=CARTESIAN_POINT('Ctrl Pts',(41.7247714995453,0.380338625256995,3.91456658266756));
#83321=CARTESIAN_POINT('Ctrl Pts',(41.7306443481196,0.265068665068968,3.92576619244952));
#83322=CARTESIAN_POINT('Ctrl Pts',(41.7365171966939,0.149452922732807,3.93185560399583));
#83323=CARTESIAN_POINT('Ctrl Pts',(41.7423900452682,0.0339770745151441,
3.9328532337741));
#83324=CARTESIAN_POINT('Ctrl Pts',(41.7439847898808,0.00262014703646743,
3.9331241354829));
#83325=CARTESIAN_POINT('Ctrl Pts',(41.7455795344935,-0.0287264958199402,
3.93301988053087));
#83326=CARTESIAN_POINT('Ctrl Pts',(41.7471742791062,-0.0600532154152404,
3.93254149518073));
#83327=CARTESIAN_POINT('Ctrl Pts',(41.7530467252401,-0.175409913857684,
3.93077990139472));
#83328=CARTESIAN_POINT('Ctrl Pts',(41.758919171374,-0.290882167778746,3.92393526583223));
#83329=CARTESIAN_POINT('Ctrl Pts',(41.7647916175079,-0.405985227089397,
3.91198990226012));
#83330=CARTESIAN_POINT('Ctrl Pts',(41.7706564564528,-0.520939181459127,
3.90006001275743));
#83331=CARTESIAN_POINT('Ctrl Pts',(41.7765212953976,-0.635524484941258,
3.88304257749326));
#83332=CARTESIAN_POINT('Ctrl Pts',(41.7823861343425,-0.749256253116583,
3.86097190706766));
#83333=CARTESIAN_POINT('Ctrl Pts',(41.7882449444625,-0.862871109487015,
3.83892392442716));
#83334=CARTESIAN_POINT('Ctrl Pts',(41.7941037545825,-0.975633772398393,
3.8118331170997));
#83335=CARTESIAN_POINT('Ctrl Pts',(41.7999625647026,-1.08706501831039,3.7797855290963));
#83336=CARTESIAN_POINT('Ctrl Pts',(41.8060483535835,-1.20281327153411,3.74649637127466));
#83337=CARTESIAN_POINT('Ctrl Pts',(41.8121341424645,-1.31712440735174,3.70785864630608));
#83338=CARTESIAN_POINT('Ctrl Pts',(41.8182199313455,-1.42947319656069,3.66402720791134));
#83339=CARTESIAN_POINT('Ctrl Pts',(41.8240719614238,-1.53750660136114,3.62187936136642));
#83340=CARTESIAN_POINT('Ctrl Pts',(41.829923991502,-1.64372520790638,3.57492959298137));
#83341=CARTESIAN_POINT('Ctrl Pts',(41.8357760215803,-1.7476787928177,3.52336598115144));
#83342=CARTESIAN_POINT('Ctrl Pts',(41.8416271619588,-1.85161657338814,3.471810208675));
#83343=CARTESIAN_POINT('Ctrl Pts',(41.8474783023374,-1.95328964681564,3.41564217110512));
#83344=CARTESIAN_POINT('Ctrl Pts',(41.8533294427159,-2.05227027493576,3.35509697603737));
#83345=CARTESIAN_POINT('Ctrl Pts',(41.8591811102834,-2.15125982123112,3.29454632583492));
#83346=CARTESIAN_POINT('Ctrl Pts',(41.8650327778509,-2.24755608733207,3.22961794984392));
#83347=CARTESIAN_POINT('Ctrl Pts',(41.8708844454184,-2.34075894162928,3.16059117526809));
#83348=CARTESIAN_POINT('Ctrl Pts',(41.8767380571026,-2.43399276098545,3.09154146772353));
#83349=CARTESIAN_POINT('Ctrl Pts',(41.8825916687869,-2.52413079295164,3.01839089997251));
#83350=CARTESIAN_POINT('Ctrl Pts',(41.8884452804711,-2.61080527636804,2.94145963917385));
#83351=CARTESIAN_POINT('Ctrl Pts',(41.894305546571,-2.69757829177952,2.86444092252531));
#83352=CARTESIAN_POINT('Ctrl Pts',(41.9001658126709,-2.78087959043404,2.78363320889896));
#83353=CARTESIAN_POINT('Ctrl Pts',(41.9060260787708,-2.86037757662643,2.69939421336208));
#83354=CARTESIAN_POINT('Ctrl Pts',(41.9118902919421,-2.93992910718403,2.61509848024282));
#83355=CARTESIAN_POINT('Ctrl Pts',(41.9177545051134,-3.01567195505458,2.52736717551507));
#83356=CARTESIAN_POINT('Ctrl Pts',(41.9236187182847,-3.08731531527128,2.43659047525254));
#83357=CARTESIAN_POINT('Ctrl Pts',(41.9294915668589,-3.15906417460091,2.34568010089484));
#83358=CARTESIAN_POINT('Ctrl Pts',(41.9353644154332,-3.22670125756978,2.2517157150014));
#83359=CARTESIAN_POINT('Ctrl Pts',(41.9412372640075,-3.28997944614429,2.15511583074973));
#83360=CARTESIAN_POINT('Ctrl Pts',(41.9428320086203,-3.30716234283552,2.12888458316073));
#83361=CARTESIAN_POINT('Ctrl Pts',(41.9444267532331,-3.32402409339884,2.10245913603982));
#83362=CARTESIAN_POINT('Ctrl Pts',(41.9460214978459,-3.3405603494249,2.07584815240666));
#83363=CARTESIAN_POINT('Ctrl Pts',(41.9520612572671,-3.4031879371436,1.9750646552753));
#83364=CARTESIAN_POINT('Ctrl Pts',(41.9581010166883,-3.46134306028622,1.8712965097234));
#83365=CARTESIAN_POINT('Ctrl Pts',(41.9641407761096,-3.51473849071923,1.76496525230859));
#83366=CARTESIAN_POINT('Ctrl Pts',(41.9701712777305,-3.56805207613178,1.65879698045018));
#83367=CARTESIAN_POINT('Ctrl Pts',(41.9762017793514,-3.61662032103247,1.55007375489776));
#83368=CARTESIAN_POINT('Ctrl Pts',(41.9822322809723,-3.66019984270016,1.43924497966738));
#83369=CARTESIAN_POINT('Ctrl Pts',(41.9884326307217,-3.70500677473279,1.32529472943574));
#83370=CARTESIAN_POINT('Ctrl Pts',(41.9946329804711,-3.74453955918482,1.20911888860736));
#83371=CARTESIAN_POINT('Ctrl Pts',(42.0008333302205,-3.77858418078361,1.09123351704934));
#83372=CARTESIAN_POINT('Ctrl Pts',(42.006846728243,-3.81160229564376,0.976902602042955));
#83373=CARTESIAN_POINT('Ctrl Pts',(42.0128601262655,-3.83945829879576,0.860964158620311));
#83374=CARTESIAN_POINT('Ctrl Pts',(42.018873524288,-3.86200575857607,0.743908946528562));
#83375=CARTESIAN_POINT('Ctrl Pts',(42.0251673499008,-3.8856046920475,0.621395005288603));
#83376=CARTESIAN_POINT('Ctrl Pts',(42.0314611755136,-3.9033878463458,0.497658012167005));
#83377=CARTESIAN_POINT('Ctrl Pts',(42.0377550011265,-3.91524622943359,0.373277327072032));
#83378=CARTESIAN_POINT('Ctrl Pts',(42.0440488267393,-3.92710461252138,0.248896641977059));
#83379=CARTESIAN_POINT('Ctrl Pts',(42.0503426523522,-3.9330381322875,0.123872739030405));
#83380=CARTESIAN_POINT('Ctrl Pts',(42.056636477965,-3.93299981544993,-0.00120485302445938));
#83381=CARTESIAN_POINT('',(43.306636477965,-3.93597073404585,-0.00313681186104915));
#83382=CARTESIAN_POINT('Ctrl Pts',(42.0566373589272,-3.9268363506648,-0.00122044486381472));
#83383=CARTESIAN_POINT('Ctrl Pts',(42.08604781148,-3.92842785028224,-0.584780799616886));
#83384=CARTESIAN_POINT('Ctrl Pts',(42.1817406702796,-3.53244649474052,-2.48145397176705));
#83385=CARTESIAN_POINT('Ctrl Pts',(42.343715935325,-0.592762475981856,-4.61374294017385));
#83386=CARTESIAN_POINT('Ctrl Pts',(42.5425631540648,3.56060894862422,-2.99333512756587));
#83387=CARTESIAN_POINT('Ctrl Pts',(42.7414103728044,4.44327790862288,1.37668903448674));
#83388=CARTESIAN_POINT('Ctrl Pts',(42.9402575915441,1.2444427730145,4.48211484186561));
#83389=CARTESIAN_POINT('Ctrl Pts',(43.1286662932643,-2.86958038868927,3.52347388524056));
#83390=CARTESIAN_POINT('Ctrl Pts',(43.2507925887379,-3.9263799435556,1.09839315991139));
#83391=CARTESIAN_POINT('Ctrl Pts',(43.306636477965,-3.93597073404585,-0.00313681186104915));
#83392=CARTESIAN_POINT('',(44.556636477965,-3.93423236178689,0.00274293657858196));
#83393=CARTESIAN_POINT('Ctrl Pts',(43.306636477965,-3.93597073404585,-0.00313681186104915));
#83394=CARTESIAN_POINT('Ctrl Pts',(43.3170749949845,-3.93776347504488,-0.209038290373662));
#83395=CARTESIAN_POINT('Ctrl Pts',(43.39379591825,-3.82930594892105,-1.72047837853632));
#83396=CARTESIAN_POINT('Ctrl Pts',(43.5367992477632,-1.87070203706735,-4.25892770068468));
#83397=CARTESIAN_POINT('Ctrl Pts',(43.7356464665026,2.57114020051616,-3.8764970450033));
#83398=CARTESIAN_POINT('Ctrl Pts',(43.9344936852423,4.65118570275307,0.0668044115854355));
#83399=CARTESIAN_POINT('Ctrl Pts',(44.133340903982,2.4587472673275,3.94874070401929));
#83400=CARTESIAN_POINT('Ctrl Pts',(44.3321881227215,-1.99224605665835,4.20344464912718));
#83401=CARTESIAN_POINT('Ctrl Pts',(44.4732866473825,-3.8520314402992,1.64433913035412));
#83402=CARTESIAN_POINT('Ctrl Pts',(44.5481027657971,-3.93833159539374,0.170959590838341));
#83403=CARTESIAN_POINT('Ctrl Pts',(44.556636477965,-3.93699635256031,0.00274486362576644));
#83404=CARTESIAN_POINT('',(45.8066364523549,-3.93089729110193,0.00177639705978037));
#83405=CARTESIAN_POINT('Ctrl Pts',(44.556636477965,-3.93299904411574,0.00274207671270665));
#83406=CARTESIAN_POINT('Ctrl Pts',(44.5624206881413,-3.93307845537151,-0.111158599951776));
#83407=CARTESIAN_POINT('Ctrl Pts',(44.5682048983176,-3.92820579813593,-0.225252330880906));
#83408=CARTESIAN_POINT('Ctrl Pts',(44.5739891084939,-3.91835726600955,-0.339065385892148));
#83409=CARTESIAN_POINT('Ctrl Pts',(44.5797669192364,-3.90851962993069,-0.452752522396843));
#83410=CARTESIAN_POINT('Ctrl Pts',(44.5855447299789,-3.89371709785247,-0.566159178932715));
#83411=CARTESIAN_POINT('Ctrl Pts',(44.5913225407214,-3.87397789315147,-0.67881093345179));
#83412=CARTESIAN_POINT('Ctrl Pts',(44.5970958748664,-3.85425398221473,-0.791375406370457));
#83413=CARTESIAN_POINT('Ctrl Pts',(44.6028692090114,-3.82960107394074,-0.903185721844889));
#83414=CARTESIAN_POINT('Ctrl Pts',(44.6086425431563,-3.80009920536556,-1.01377267145058));
#83415=CARTESIAN_POINT('Ctrl Pts',(44.6144130463777,-3.7706118028743,-1.12430539533532));
#83416=CARTESIAN_POINT('Ctrl Pts',(44.6201835495991,-3.73628027642083,-1.23361553491909));
#83417=CARTESIAN_POINT('Ctrl Pts',(44.6259540528205,-3.69723556713716,-1.34124500412712));
#83418=CARTESIAN_POINT('Ctrl Pts',(44.6317234956459,-3.65819803276486,-1.44885469519065));
#83419=CARTESIAN_POINT('Ctrl Pts',(44.6374929384714,-3.61444918202758,-1.55478392921504));
#83420=CARTESIAN_POINT('Ctrl Pts',(44.6432623812969,-3.5661692773945,-1.65859147621335));
#83421=CARTESIAN_POINT('Ctrl Pts',(44.6490322530335,-3.51788578354319,-1.76240674045847));
#83422=CARTESIAN_POINT('Ctrl Pts',(44.6548021247701,-3.46507074697258,-1.86409961824766));
#83423=CARTESIAN_POINT('Ctrl Pts',(44.6605719965068,-3.40795148119965,-1.96325130887237));
#83424=CARTESIAN_POINT('Ctrl Pts',(44.6663478768146,-3.35077273313811,-2.0625062530911));
#83425=CARTESIAN_POINT('Ctrl Pts',(44.6721237571224,-3.28928101433859,-2.15921435327852));
#83426=CARTESIAN_POINT('Ctrl Pts',(44.6778996374303,-3.22374836692943,-2.2529836809706));
#83427=CARTESIAN_POINT('Ctrl Pts',(44.6836778400347,-3.15818937094041,-2.34679071030784));
#83428=CARTESIAN_POINT('Ctrl Pts',(44.6894560426391,-3.08858647423604,-2.4376562789466));
#83429=CARTESIAN_POINT('Ctrl Pts',(44.6952342452436,-3.01525226988168,-2.52522132673027));
#83430=CARTESIAN_POINT('Ctrl Pts',(44.7010220474629,-2.94179623177173,-2.61293185067644));
#83431=CARTESIAN_POINT('Ctrl Pts',(44.7068098496823,-2.86459678953794,-2.69733058461385));
#83432=CARTESIAN_POINT('Ctrl Pts',(44.7125976519017,-2.78400402223915,-2.77809477954879));
#83433=CARTESIAN_POINT('Ctrl Pts',(44.7183592880014,-2.70377560740306,-2.85849384701251));
#83434=CARTESIAN_POINT('Ctrl Pts',(44.7241209241011,-2.62018485274011,-2.93529096204368));
#83435=CARTESIAN_POINT('Ctrl Pts',(44.7298825602008,-2.53360749863687,-3.00820910889702));
#83436=CARTESIAN_POINT('Ctrl Pts',(44.7357550063304,-2.44536505513321,-3.082529645956));
#83437=CARTESIAN_POINT('Ctrl Pts',(44.7416274524601,-2.35370193720534,-3.15308858054237));
#83438=CARTESIAN_POINT('Ctrl Pts',(44.7474998985897,-2.25897250273774,-3.21955466359476));
#83439=CARTESIAN_POINT('Ctrl Pts',(44.7533647375302,-2.16436578114149,-3.28593464622922));
#83440=CARTESIAN_POINT('Ctrl Pts',(44.7592295764707,-2.06670097739061,-3.34823208568584));
#83441=CARTESIAN_POINT('Ctrl Pts',(44.7650944154112,-1.96636665008259,-3.40615489921451));
#83442=CARTESIAN_POINT('Ctrl Pts',(44.7709532255268,-1.86613546253602,-3.46401817035793));
#83443=CARTESIAN_POINT('Ctrl Pts',(44.7768120356424,-1.76324056556485,-3.51751555481816));
#83444=CARTESIAN_POINT('Ctrl Pts',(44.782670845758,-1.65810017070269,-3.56639773776225));
#83445=CARTESIAN_POINT('Ctrl Pts',(44.7887566346406,-1.54888648506683,-3.61717368708458));
#83446=CARTESIAN_POINT('Ctrl Pts',(44.7948424235232,-1.43725016692758,-3.66296934236462));
#83447=CARTESIAN_POINT('Ctrl Pts',(44.8009282124058,-1.32368928437454,-3.70355716554126));
#83448=CARTESIAN_POINT('Ctrl Pts',(44.8067802424795,-1.21449034357772,-3.74258598603381));
#83449=CARTESIAN_POINT('Ctrl Pts',(44.8126322725532,-1.10351238371233,-3.77679951451677));
#83450=CARTESIAN_POINT('Ctrl Pts',(44.8184843026268,-0.991218636692286,
-3.80604448401144));
#83451=CARTESIAN_POINT('Ctrl Pts',(44.8243354430007,-0.878941961991345,
-3.83528500731507));
#83452=CARTESIAN_POINT('Ctrl Pts',(44.8301865833746,-0.765350297790627,
-3.85955836943044));
#83453=CARTESIAN_POINT('Ctrl Pts',(44.8360377237485,-0.650920742602548,
-3.87876155323445));
#83454=CARTESIAN_POINT('Ctrl Pts',(44.8418893913113,-0.536480877287995,
-3.89796646724928));
#83455=CARTESIAN_POINT('Ctrl Pts',(44.8477410588741,-0.421203378591719,
-3.91210022641299));
#83456=CARTESIAN_POINT('Ctrl Pts',(44.8535927264369,-0.305573502809252,
-3.92111130094274));
#83457=CARTESIAN_POINT('Ctrl Pts',(44.8594463381164,-0.189905210974066,
-3.93012536924821));
#83458=CARTESIAN_POINT('Ctrl Pts',(44.8652999497959,-0.0738847211529398,
-3.93401333664791));
#83459=CARTESIAN_POINT('Ctrl Pts',(44.8711535614754,0.0420003653842455,
-3.93277573341115));
#83460=CARTESIAN_POINT('Ctrl Pts',(44.8770138275706,0.158017190679275,-3.9315367232607));
#83461=CARTESIAN_POINT('Ctrl Pts',(44.8828740936657,0.273897891879422,-3.9251605168428));
#83462=CARTESIAN_POINT('Ctrl Pts',(44.8887343597608,0.389157546645517,-3.91369970793479));
#83463=CARTESIAN_POINT('Ctrl Pts',(44.8945985729274,0.504494832372195,-3.90223117981569));
#83464=CARTESIAN_POINT('Ctrl Pts',(44.9004627860939,0.619209830641658,-3.88567128897828));
#83465=CARTESIAN_POINT('Ctrl Pts',(44.9063269992604,0.732827125818421,-3.86412388565179));
#83466=CARTESIAN_POINT('Ctrl Pts',(44.9121998478299,0.846611729225945,-3.8425447524912));
#83467=CARTESIAN_POINT('Ctrl Pts',(44.9180726963994,0.959295002661169,-3.81596354341015));
#83468=CARTESIAN_POINT('Ctrl Pts',(44.9239455449689,1.07041592807867,-3.78453415110968));
#83469=CARTESIAN_POINT('Ctrl Pts',(44.9255402896261,1.10059029746953,-3.77599964611486));
#83470=CARTESIAN_POINT('Ctrl Pts',(44.9271350342834,1.1306495765463,-3.76710792615816));
#83471=CARTESIAN_POINT('Ctrl Pts',(44.9287297789406,1.16058480135576,-3.7578626796175));
#83472=CARTESIAN_POINT('Ctrl Pts',(44.9346022251097,1.27081749312859,-3.72381822467294));
#83473=CARTESIAN_POINT('Ctrl Pts',(44.9404746712788,1.37973548501979,-3.68486233087554));
#83474=CARTESIAN_POINT('Ctrl Pts',(44.9463471174479,1.48686852242519,-3.64111397748287));
#83475=CARTESIAN_POINT('Ctrl Pts',(44.952211956428,1.59386277928895,-3.59742229587257));
#83476=CARTESIAN_POINT('Ctrl Pts',(44.9580767954082,1.69907630073164,-3.54895065533863));
#83477=CARTESIAN_POINT('Ctrl Pts',(44.9639416343883,1.80205328652408,-3.4958679827087));
#83478=CARTESIAN_POINT('Ctrl Pts',(44.9698004445437,1.90492441600864,-3.44283987698702));
#83479=CARTESIAN_POINT('Ctrl Pts',(44.9756592546991,2.00556321761252,-3.38521035546842));
#83480=CARTESIAN_POINT('Ctrl Pts',(44.9815180648545,2.1035338342139,-3.32319641434529));
#83481=CARTESIAN_POINT('Ctrl Pts',(44.9876038537222,2.20529997308246,-3.25877996415797));
#83482=CARTESIAN_POINT('Ctrl Pts',(44.99368964259,2.30418658640912,-3.18963267796784));
#83483=CARTESIAN_POINT('Ctrl Pts',(44.9997754314577,2.39973295664176,-3.11605050292953));
#83484=CARTESIAN_POINT('Ctrl Pts',(45.0056274615712,2.4916093342146,-3.0452946628072));
#83485=CARTESIAN_POINT('Ctrl Pts',(45.0114794916848,2.58039697900309,-2.9704386182479));
#83486=CARTESIAN_POINT('Ctrl Pts',(45.0173315217983,2.66571648721625,-2.89178917104679));
#83487=CARTESIAN_POINT('Ctrl Pts',(45.023182662212,2.75102302407562,-2.81315168113219));
#83488=CARTESIAN_POINT('Ctrl Pts',(45.0290338026257,2.83286216890139,-2.73072221537499));
#83489=CARTESIAN_POINT('Ctrl Pts',(45.0348849430394,2.91088929071739,-2.64484641088794));
#83490=CARTESIAN_POINT('Ctrl Pts',(45.040736610642,2.98892344279184,-2.55896286897464));
#83491=CARTESIAN_POINT('Ctrl Pts',(45.0465882782445,3.06314461109269,-2.46963267700669));
#83492=CARTESIAN_POINT('Ctrl Pts',(45.0524399458471,3.13324706525646,-2.37723617422875));
#83493=CARTESIAN_POINT('Ctrl Pts',(45.0582935575662,3.20337280976299,-2.28480897429129));
#83494=CARTESIAN_POINT('Ctrl Pts',(45.0641471692853,3.26937686949293,-2.1893137669915));
#83495=CARTESIAN_POINT('Ctrl Pts',(45.0700007810045,3.3309960395111,-2.09116101359062));
#83496=CARTESIAN_POINT('Ctrl Pts',(45.0758610471389,3.39268525851159,-1.99289667964614));
#83497=CARTESIAN_POINT('Ctrl Pts',(45.0817213132733,3.44997941846655,-1.8919691198558));
#83498=CARTESIAN_POINT('Ctrl Pts',(45.0875815794076,3.50266055925314,-1.78881469321238));
#83499=CARTESIAN_POINT('Ctrl Pts',(45.0934457926132,3.55537718242393,-1.6855907888594));
#83500=CARTESIAN_POINT('Ctrl Pts',(45.0993100058188,3.60347442862843,-1.5801374062886));
#83501=CARTESIAN_POINT('Ctrl Pts',(45.1051742190244,3.64678259549991,-1.47291062225748));
#83502=CARTESIAN_POINT('Ctrl Pts',(45.1110470676325,3.69015453622069,-1.36552594041497));
#83503=CARTESIAN_POINT('Ctrl Pts',(45.1169199162405,3.72872318563004,-1.25636303347945));
#83504=CARTESIAN_POINT('Ctrl Pts',(45.1227927648485,3.76236872245895,-1.14589292530437));
#83505=CARTESIAN_POINT('Ctrl Pts',(45.1243875091257,3.77150500893467,-1.11589528964697));
#83506=CARTESIAN_POINT('Ctrl Pts',(45.1259822534029,3.78027857266151,-1.08580131924658));
#83507=CARTESIAN_POINT('Ctrl Pts',(45.1275769976801,3.78868766943574,-1.05562054899741));
#83508=CARTESIAN_POINT('Ctrl Pts',(45.1334494437569,3.81965311516091,-0.944483642360871));
#83509=CARTESIAN_POINT('Ctrl Pts',(45.1393218898338,3.84577614321039,-0.831797007719057));
#83510=CARTESIAN_POINT('Ctrl Pts',(45.1451943359106,3.86690256851341,-0.718020560725395));
#83511=CARTESIAN_POINT('Ctrl Pts',(45.1510591747984,3.88800162656469,-0.604391500174129));
#83512=CARTESIAN_POINT('Ctrl Pts',(45.1569240136862,3.90411687883725,-0.489675837397397));
#83513=CARTESIAN_POINT('Ctrl Pts',(45.1627888525741,3.91514397222974,-0.374348336062974));
#83514=CARTESIAN_POINT('Ctrl Pts',(45.1686476626372,3.92615973020211,-0.259139386883065));
#83515=CARTESIAN_POINT('Ctrl Pts',(45.1745064727003,3.93209769379473,-0.143320259163626));
#83516=CARTESIAN_POINT('Ctrl Pts',(45.1803652827635,3.93290472972664,-0.0273749318511684));
#83517=CARTESIAN_POINT('Ctrl Pts',(45.1864510716658,3.93374303140654,0.0930622863947814));
#83518=CARTESIAN_POINT('Ctrl Pts',(45.1925368605682,3.92904472264376,0.213635233589722));
#83519=CARTESIAN_POINT('Ctrl Pts',(45.1986226494705,3.91880964212148,0.333796328343629));
#83520=CARTESIAN_POINT('Ctrl Pts',(45.2044746794926,3.90896769731263,0.449341961830767));
#83521=CARTESIAN_POINT('Ctrl Pts',(45.2103267095148,3.89400651467889,0.564506348318379));
#83522=CARTESIAN_POINT('Ctrl Pts',(45.2161787395369,3.87397903110801,0.678804439095266));
#83523=CARTESIAN_POINT('Ctrl Pts',(45.2220298798596,3.85395459236771,0.793085152835175));
#83524=CARTESIAN_POINT('Ctrl Pts',(45.2278810201823,3.82886545550704,0.90649942569439));
#83525=CARTESIAN_POINT('Ctrl Pts',(45.233732160505,3.79881602804613,1.01857046150957));
#83526=CARTESIAN_POINT('Ctrl Pts',(45.2395838280172,3.7687638931234,1.13065159495643));
#83527=CARTESIAN_POINT('Ctrl Pts',(45.2454354955293,3.73375068621552,1.2413888514924));
#83528=CARTESIAN_POINT('Ctrl Pts',(45.2512871630414,3.69393104054491,1.35031939469845));
#83529=CARTESIAN_POINT('Ctrl Pts',(45.2571407746707,3.65409816547271,1.45928612822909));
#83530=CARTESIAN_POINT('Ctrl Pts',(45.2629943863,3.60945581822659,1.56644456684418));
#83531=CARTESIAN_POINT('Ctrl Pts',(45.2688479979294,3.5602069648722,1.67135135961158));
#83532=CARTESIAN_POINT('Ctrl Pts',(45.2747082639753,3.51090212516121,1.77637741097504));
#83533=CARTESIAN_POINT('Ctrl Pts',(45.2805685300213,3.45698050282509,1.87914633305179));
#83534=CARTESIAN_POINT('Ctrl Pts',(45.2864287960673,3.39869131366523,1.97923883208079));
#83535=CARTESIAN_POINT('Ctrl Pts',(45.2922930091851,3.34036286491889,2.07939874652897));
#83536=CARTESIAN_POINT('Ctrl Pts',(45.298157222303,3.27766121491813,2.17687830168419));
#83537=CARTESIAN_POINT('Ctrl Pts',(45.3040214354209,3.2108782596862,2.27128813704349));
#83538=CARTESIAN_POINT('Ctrl Pts',(45.3098942839429,3.14399696256334,2.36583699652503));
#83539=CARTESIAN_POINT('Ctrl Pts',(45.3157671324649,3.07302261796205,2.45730678915368));
#83540=CARTESIAN_POINT('Ctrl Pts',(45.3216399809869,2.99828666675576,2.54534203280318));
#83541=CARTESIAN_POINT('Ctrl Pts',(45.3232347261312,2.97799246116798,2.56924760040159));
#83542=CARTESIAN_POINT('Ctrl Pts',(45.3248294712755,2.95742108973002,2.592900131298));
#83543=CARTESIAN_POINT('Ctrl Pts',(45.3264242164198,2.93657963018286,2.61629300262702));
#83544=CARTESIAN_POINT('Ctrl Pts',(45.332296662543,2.8598336066834,2.70243427544308));
#83545=CARTESIAN_POINT('Ctrl Pts',(45.3381691086663,2.779165593308,2.78534001710213));
#83546=CARTESIAN_POINT('Ctrl Pts',(45.3440415547895,2.69487910576092,2.86463184464134));
#83547=CARTESIAN_POINT('Ctrl Pts',(45.3499063937232,2.61070180325834,2.94382095723808));
#83548=CARTESIAN_POINT('Ctrl Pts',(45.3557712326568,2.52291564642326,3.0194051848909));
#83549=CARTESIAN_POINT('Ctrl Pts',(45.3616360715904,2.4318635858981,3.09104003526043));
#83550=CARTESIAN_POINT('Ctrl Pts',(45.3674948816987,2.34090512333472,3.16260124780181));
#83551=CARTESIAN_POINT('Ctrl Pts',(45.373353691807,2.24668775769553,3.23022090418208));
#83552=CARTESIAN_POINT('Ctrl Pts',(45.3792125019153,2.14958988667897,3.29359261583571));
#83553=CARTESIAN_POINT('Ctrl Pts',(45.3852982908005,2.04873030371198,3.35941943924977));
#83554=CARTESIAN_POINT('Ctrl Pts',(45.3913840796857,1.94476284241733,3.42066220667751));
#83555=CARTESIAN_POINT('Ctrl Pts',(45.3974698685708,1.8381480459053,3.47702469955773));
#83556=CARTESIAN_POINT('Ctrl Pts',(45.4033218986362,1.73562838799901,3.53122227510883));
#83557=CARTESIAN_POINT('Ctrl Pts',(45.4091739287015,1.63066141412722,3.58090735796026));
#83558=CARTESIAN_POINT('Ctrl Pts',(45.4150259587668,1.52368377511028,3.62586220828449));
#83559=CARTESIAN_POINT('Ctrl Pts',(45.420877099132,1.41672240019707,3.67081022399959));
#83560=CARTESIAN_POINT('Ctrl Pts',(45.4267282394971,1.30775134891695,3.71102927699763));
#83561=CARTESIAN_POINT('Ctrl Pts',(45.4325793798623,1.19722816067176,3.7463493872428));
#83562=CARTESIAN_POINT('Ctrl Pts',(45.438431047416,1.08669501427171,3.7816726798349));
#83563=CARTESIAN_POINT('Ctrl Pts',(45.4442827149697,0.974609846665904,3.81209602638497));
#83564=CARTESIAN_POINT('Ctrl Pts',(45.4501343825235,0.861445611746805,3.83749924534223));
#83565=CARTESIAN_POINT('Ctrl Pts',(45.4559879941936,0.748243779948002,3.86291090408409));
#83566=CARTESIAN_POINT('Ctrl Pts',(45.4618416058637,0.633962571083644,3.88329902832254));
#83567=CARTESIAN_POINT('Ctrl Pts',(45.4676952175337,0.519084681744792,3.89859463052751));
#83568=CARTESIAN_POINT('Ctrl Pts',(45.473555483619,0.404076198644307,3.91390762084989));
#83569=CARTESIAN_POINT('Ctrl Pts',(45.4794157497042,0.288470091169484,3.92411647949205));
#83570=CARTESIAN_POINT('Ctrl Pts',(45.4852760157895,0.172753826510763,3.92920413257264));
#83571=CARTESIAN_POINT('Ctrl Pts',(45.4911402289458,0.0569596233558427,
3.9342952123455));
#83572=CARTESIAN_POINT('Ctrl Pts',(45.4970044421022,-0.0589444723727581,
3.9342582184567));
#83573=CARTESIAN_POINT('Ctrl Pts',(45.5028686552585,-0.174473095974319,
3.92912816522713));
#83574=CARTESIAN_POINT('Ctrl Pts',(45.5087415038176,-0.290171842345175,
3.92399055768907));
#83575=CARTESIAN_POINT('Ctrl Pts',(45.5146143523766,-0.405493602914874,
3.91374495908021));
#83576=CARTESIAN_POINT('Ctrl Pts',(45.5204872009356,-0.519960129469059,
3.89847796758716));
#83577=CARTESIAN_POINT('Ctrl Pts',(45.5220819456768,-0.551042982949431,
3.89433228697686));
#83578=CARTESIAN_POINT('Ctrl Pts',(45.5236766904181,-0.582062846145865,
3.88981663263307));
#83579=CARTESIAN_POINT('Ctrl Pts',(45.5252714351593,-0.613010320845078,
3.8849333773615));
#83580=CARTESIAN_POINT('Ctrl Pts',(45.5311438815243,-0.726970493028684,
3.86695140574754));
#83581=CARTESIAN_POINT('Ctrl Pts',(45.5370163278893,-0.8403295674727,3.84392073604923));
#83582=CARTESIAN_POINT('Ctrl Pts',(45.5428887742542,-0.952605130974747,
3.81589209287168));
#83583=CARTESIAN_POINT('Ctrl Pts',(45.5487536134309,-1.06473525230577,3.78789975809987));
#83584=CARTESIAN_POINT('Ctrl Pts',(45.5546184526076,-1.17578425657252,3.75492242430939));
#83585=CARTESIAN_POINT('Ctrl Pts',(45.5604832917843,-1.28527691679575,3.71706231413357));
#83586=CARTESIAN_POINT('Ctrl Pts',(45.5663421021367,-1.39465702286518,3.67924112266385));
#83587=CARTESIAN_POINT('Ctrl Pts',(45.5722009124892,-1.5024835787848,3.63654727274737));
#83588=CARTESIAN_POINT('Ctrl Pts',(45.5780597228416,-1.60829424422621,3.58913340849694));
#83589=CARTESIAN_POINT('Ctrl Pts',(45.5841455116356,-1.71820416165022,3.53988266536269));
#83590=CARTESIAN_POINT('Ctrl Pts',(45.5902313004297,-1.82593839191682,3.48553890149408));
#83591=CARTESIAN_POINT('Ctrl Pts',(45.5963170892237,-1.9309987330142,3.42632936144463));
#83592=CARTESIAN_POINT('Ctrl Pts',(45.6021691195343,-2.0320236488207,3.36939409228447));
#83593=CARTESIAN_POINT('Ctrl Pts',(45.6080211498448,-2.13057590408607,3.30796016780319));
#83594=CARTESIAN_POINT('Ctrl Pts',(45.6138731801553,-2.2262362325335,3.24227716843502));
#83595=CARTESIAN_POINT('Ctrl Pts',(45.6197243207657,-2.32188201747935,3.17660415503305));
#83596=CARTESIAN_POINT('Ctrl Pts',(45.625575461376,-2.41463640914046,3.10668358511262));
#83597=CARTESIAN_POINT('Ctrl Pts',(45.6314266019864,-2.50410902253351,3.03280843497677));
#83598=CARTESIAN_POINT('Ctrl Pts',(45.637278269785,-2.59358969741732,2.95892662868305));
#83599=CARTESIAN_POINT('Ctrl Pts',(45.6431299375837,-2.67978768746533,2.88108979706325));
#83600=CARTESIAN_POINT('Ctrl Pts',(45.6489816053823,-2.76234616385116,2.79963080977774));
#83601=CARTESIAN_POINT('Ctrl Pts',(45.6548352172968,-2.84493206886839,2.71814475914715));
#83602=CARTESIAN_POINT('Ctrl Pts',(45.6606888292112,-2.9238757617867,2.63303445013365));
#83603=CARTESIAN_POINT('Ctrl Pts',(45.6665424411257,-2.99885821066938,2.54466862917372));
#83604=CARTESIAN_POINT('Ctrl Pts',(45.6724027074533,-3.07392589994712,2.45620235353938));
#83605=CARTESIAN_POINT('Ctrl Pts',(45.6782629737809,-3.14502308942954,2.36447349448886));
#83606=CARTESIAN_POINT('Ctrl Pts',(45.6841232401084,-3.2118718378919,2.26988288177098));
#83607=CARTESIAN_POINT('Ctrl Pts',(45.6899874535062,-3.2787656110491,2.17522855935663));
#83608=CARTESIAN_POINT('Ctrl Pts',(45.695851666904,-3.34140502260285,2.07770899221613));
#83609=CARTESIAN_POINT('Ctrl Pts',(45.7017158803018,-3.39955708522553,1.97775140609049));
#83610=CARTESIAN_POINT('Ctrl Pts',(45.7075887290991,-3.45779478018413,1.87764662653426));
#83611=CARTESIAN_POINT('Ctrl Pts',(45.7134615778964,-3.51153174705241,1.77509702757215));
#83612=CARTESIAN_POINT('Ctrl Pts',(45.7193344266936,-3.56058223926699,1.67055174041885));
#83613=CARTESIAN_POINT('Ctrl Pts',(45.7209291690954,-3.57390165246216,1.64216299620176));
#83614=CARTESIAN_POINT('Ctrl Pts',(45.7225239114972,-3.5868757819742,1.61362719182157));
#83615=CARTESIAN_POINT('Ctrl Pts',(45.724118653899,-3.59950154213154,1.5849535160984));
#83616=CARTESIAN_POINT('Ctrl Pts',(45.7305881397463,-3.65072121030955,1.46863131943987));
#83617=CARTESIAN_POINT('Ctrl Pts',(45.7370576255936,-3.69635132197521,1.34970412641326));
#83618=CARTESIAN_POINT('Ctrl Pts',(45.743527111441,-3.7361454474959,1.22870101943298));
#83619=CARTESIAN_POINT('Ctrl Pts',(45.7499705088804,-3.77577910193737,1.10818586133743));
#83620=CARTESIAN_POINT('Ctrl Pts',(45.7564139063199,-3.80962360872221,0.985611738784826));
#83621=CARTESIAN_POINT('Ctrl Pts',(45.7628573037594,-3.83748139162275,0.8615251412171));
#83622=CARTESIAN_POINT('Ctrl Pts',(45.7692834923951,-3.86526477291706,0.737769949856485));
#83623=CARTESIAN_POINT('Ctrl Pts',(45.7757096810308,-3.88709323586644,0.612510597555861));
#83624=CARTESIAN_POINT('Ctrl Pts',(45.7821358696666,-3.90281850505353,0.486309280820051));
#83625=CARTESIAN_POINT('Ctrl Pts',(45.7885361949728,-3.91848048512147,0.360615883540352));
#83626=CARTESIAN_POINT('Ctrl Pts',(45.794936520279,-3.92808819621711,0.233988347893363));
#83627=CARTESIAN_POINT('Ctrl Pts',(45.8013368455852,-3.93154427294153,0.106998270549759));
#83628=CARTESIAN_POINT('Ctrl Pts',(45.8031033762349,-3.932498172184,0.0719481983906104));
#83629=CARTESIAN_POINT('Ctrl Pts',(45.8048699068845,-3.93298373692229,0.0368705902930527));
#83630=CARTESIAN_POINT('Ctrl Pts',(45.8066364375341,-3.93299959826995,0.00177764125482606));
#83631=CARTESIAN_POINT('',(47.0566365067525,-3.9325046759356,-0.00340936713855836));
#83632=CARTESIAN_POINT('Ctrl Pts',(45.806636477965,-3.92726452529281,0.00177424710315623));
#83633=CARTESIAN_POINT('Ctrl Pts',(45.8454129428563,-3.92414560096597,-0.76741648345805));
#83634=CARTESIAN_POINT('Ctrl Pts',(45.9504718139941,-3.33362574617699,-2.85584174047811));
#83635=CARTESIAN_POINT('Ctrl Pts',(46.1218130913783,0.0625822105554463,
-4.65124432931964));
#83636=CARTESIAN_POINT('Ctrl Pts',(46.320660310118,3.94650710844973,-2.46233096823187));
#83637=CARTESIAN_POINT('Ctrl Pts',(46.5195075288577,4.20525141962489,1.98842986640301));
#83638=CARTESIAN_POINT('Ctrl Pts',(46.7183547475972,0.601137845897373,4.61265846243321));
#83639=CARTESIAN_POINT('Ctrl Pts',(46.897397730633,-3.14122023442404,3.16042933645599));
#83640=CARTESIAN_POINT('Ctrl Pts',(47.0101583074223,-3.92291374881594,0.916664918939353));
#83641=CARTESIAN_POINT('Ctrl Pts',(47.056636477965,-3.93047922134086,-0.00340704118923197));
#83642=CARTESIAN_POINT('',(48.3066364779243,-3.93299998520013,-0.000341197588748887));
#83643=CARTESIAN_POINT('Ctrl Pts',(47.0566365137715,-3.93299852178314,-0.00340993425095843));
#83644=CARTESIAN_POINT('Ctrl Pts',(47.063697492587,-3.93287725698335,-0.14327605577757));
#83645=CARTESIAN_POINT('Ctrl Pts',(47.0707584714024,-3.92529131289588,-0.282815375072087));
#83646=CARTESIAN_POINT('Ctrl Pts',(47.0778194502179,-3.9103676131021,-0.421324258027222));
#83647=CARTESIAN_POINT('Ctrl Pts',(47.0849765080332,-3.8952408459734,-0.561717836474329));
#83648=CARTESIAN_POINT('Ctrl Pts',(47.0921335658485,-3.87257533825972,-0.701052745607565));
#83649=CARTESIAN_POINT('Ctrl Pts',(47.0992906236638,-3.84255229214712,-0.838618436546029));
#83650=CARTESIAN_POINT('Ctrl Pts',(47.1048768108013,-3.81911887043196,-0.94599044794049));
#83651=CARTESIAN_POINT('Ctrl Pts',(47.1104629979389,-3.79120420303399,-1.05228509905202));
#83652=CARTESIAN_POINT('Ctrl Pts',(47.1160491850765,-3.75891448323585,-1.15717367223755));
#83653=CARTESIAN_POINT('Ctrl Pts',(47.1219216474124,-3.72497001294099,-1.26743746761962));
#83654=CARTESIAN_POINT('Ctrl Pts',(47.1277941097484,-3.6861128910397,-1.37639101302529));
#83655=CARTESIAN_POINT('Ctrl Pts',(47.1336665720844,-3.64246167079225,-1.48356394429405));
#83656=CARTESIAN_POINT('Ctrl Pts',(47.1395314270849,-3.59886699743339,-1.59059804105212));
#83657=CARTESIAN_POINT('Ctrl Pts',(47.1453962820855,-3.55049073048167,-1.69585573149472));
#83658=CARTESIAN_POINT('Ctrl Pts',(47.151261137086,-3.49750138385289,-1.79888106053377));
#83659=CARTESIAN_POINT('Ctrl Pts',(47.1571199630991,-3.44456650951828,-1.90180048100088));
#83660=CARTESIAN_POINT('Ctrl Pts',(47.1629787891122,-3.38702817588962,-2.00249173924161));
#83661=CARTESIAN_POINT('Ctrl Pts',(47.1688376151253,-3.32510298432286,-2.10051877964639));
#83662=CARTESIAN_POINT('Ctrl Pts',(47.1749233979874,-3.26077895955596,-2.20234315217217));
#83663=CARTESIAN_POINT('Ctrl Pts',(47.1810091808495,-3.19172150231696,-2.30129230103316));
#83664=CARTESIAN_POINT('Ctrl Pts',(47.1870949637116,-3.11822613909831,-2.39690524331773));
#83665=CARTESIAN_POINT('Ctrl Pts',(47.1929470091838,-3.04755352108066,-2.48884596789811));
#83666=CARTESIAN_POINT('Ctrl Pts',(47.1987990546561,-2.97277787900469,-2.57770166929477));
#83667=CARTESIAN_POINT('Ctrl Pts',(47.2046511001283,-2.89420567089331,-2.66309266353408));
#83668=CARTESIAN_POINT('Ctrl Pts',(47.2105022556919,-2.81564541109725,-2.74847067253917));
#83669=CARTESIAN_POINT('Ctrl Pts',(47.2163534112555,-2.73329001301056,-2.83038471788304));
#83670=CARTESIAN_POINT('Ctrl Pts',(47.2222045668191,-2.64748480158604,-2.90848985306308));
#83671=CARTESIAN_POINT('Ctrl Pts',(47.2280562493478,-2.56167186239736,-2.98660202252525));
#83672=CARTESIAN_POINT('Ctrl Pts',(47.2339079318765,-2.47240879793387,-3.06090432163304));
#83673=CARTESIAN_POINT('Ctrl Pts',(47.2397596144052,-2.38007567067358,-3.13109067289143));
#83674=CARTESIAN_POINT('Ctrl Pts',(47.2456132408115,-2.28771187115799,-3.20130033944032));
#83675=CARTESIAN_POINT('Ctrl Pts',(47.2514668672179,-2.19227630984071,-3.26739108937189));
#83676=CARTESIAN_POINT('Ctrl Pts',(47.2573204936242,-2.09417920993768,-3.32909934316547));
#83677=CARTESIAN_POINT('Ctrl Pts',(47.2631807740199,-1.99597060017408,-3.39087774254729));
#83678=CARTESIAN_POINT('Ctrl Pts',(47.2690410544157,-1.89509476322088,-3.44826348223305));
#83679=CARTESIAN_POINT('Ctrl Pts',(47.2749013348114,-1.79198786121663,-3.50103820391212));
#83680=CARTESIAN_POINT('Ctrl Pts',(47.2807655620484,-1.68881151772795,-3.55384846884721));
#83681=CARTESIAN_POINT('Ctrl Pts',(47.2866297892853,-1.58340149221702,-3.60204136069649));
#83682=CARTESIAN_POINT('Ctrl Pts',(47.2924940165223,-1.47621370860026,-3.64544676089786));
#83683=CARTESIAN_POINT('Ctrl Pts',(47.2983668787172,-1.36886809310394,-3.68891607468774));
#83684=CARTESIAN_POINT('Ctrl Pts',(47.3042397409121,-1.25973988321992,-3.72758368992329));
#83685=CARTESIAN_POINT('Ctrl Pts',(47.310112603107,-1.14929999544176,-3.7613293554909));
#83686=CARTESIAN_POINT('Ctrl Pts',(47.3117072033434,-1.1193133440762,-3.77049198258907));
#83687=CARTESIAN_POINT('Ctrl Pts',(47.3133018035798,-1.08923004604906,-3.77929203982554));
#83688=CARTESIAN_POINT('Ctrl Pts',(47.3148964038162,-1.05905963205316,-3.78772777476886));
#83689=CARTESIAN_POINT('Ctrl Pts',(47.3207689043242,-0.947949795571908,
-3.81879440614748));
#83690=CARTESIAN_POINT('Ctrl Pts',(47.3266414048322,-0.835285833085913,
-3.84501992627515));
#83691=CARTESIAN_POINT('Ctrl Pts',(47.3325139053402,-0.721527529778128,
-3.86624973634299));
#83692=CARTESIAN_POINT('Ctrl Pts',(47.3383787990124,-0.607916581201406,
-3.88745204676587));
#83693=CARTESIAN_POINT('Ctrl Pts',(47.3442436926846,-0.493214513363632,
-3.90367144072259));
#83694=CARTESIAN_POINT('Ctrl Pts',(47.3501085863568,-0.377896003926385,
-3.91480313811774));
#83695=CARTESIAN_POINT('Ctrl Pts',(47.35596745149,-0.262696030676819,-3.92592339321296));
#83696=CARTESIAN_POINT('Ctrl Pts',(47.3618263166231,-0.146881285142962,
-3.93196631434662));
#83697=CARTESIAN_POINT('Ctrl Pts',(47.3676851817563,-0.0309357060821324,
-3.93287833298835));
#83698=CARTESIAN_POINT('Ctrl Pts',(47.3737709501229,0.0895002352245635,
-3.93382567245998));
#83699=CARTESIAN_POINT('Ctrl Pts',(47.3798567184896,0.210076902211475,-3.92923656982957));
#83700=CARTESIAN_POINT('Ctrl Pts',(47.3859424868562,0.330246726315724,-3.91911037095892));
#83701=CARTESIAN_POINT('Ctrl Pts',(47.3917945723126,0.445802238383835,-3.90937300049571));
#83702=CARTESIAN_POINT('Ctrl Pts',(47.397646657769,0.560981125584535,-3.89451596011917));
#83703=CARTESIAN_POINT('Ctrl Pts',(47.4034987432254,0.675298284084939,-3.87459174978628));
#83704=CARTESIAN_POINT('Ctrl Pts',(47.4093499390223,0.789598063595361,-3.85467056841823));
#83705=CARTESIAN_POINT('Ctrl Pts',(47.4152011348193,0.903035967785185,-3.82968381972095));
#83706=CARTESIAN_POINT('Ctrl Pts',(47.4210523306163,1.01513509889997,-3.79973548171203));
#83707=CARTESIAN_POINT('Ctrl Pts',(47.4269040535837,1.12724432971841,-3.76978444547221));
#83708=CARTESIAN_POINT('Ctrl Pts',(47.4327557765511,1.23801414831716,-3.73487103798001));
#83709=CARTESIAN_POINT('Ctrl Pts',(47.4386074995184,1.3469815712235,-3.69514947556716));
#83710=CARTESIAN_POINT('Ctrl Pts',(47.444461166525,1.45598519490961,-3.65541471699444));
#83711=CARTESIAN_POINT('Ctrl Pts',(47.4503148335315,1.56318484410882,-3.61086876875883));
#83712=CARTESIAN_POINT('Ctrl Pts',(47.456168500538,1.66813697697349,-3.56171419769382));
#83713=CARTESIAN_POINT('Ctrl Pts',(47.4620288215649,1.77320841174416,-3.51250375130874));
#83714=CARTESIAN_POINT('Ctrl Pts',(47.4678891425918,1.87602685631187,-3.458674401153));
#83715=CARTESIAN_POINT('Ctrl Pts',(47.4737494636186,1.97617278397272,-3.40047498562855));
#83716=CARTESIAN_POINT('Ctrl Pts',(47.4796137315547,2.07638615962443,-3.34223637296711));
#83717=CARTESIAN_POINT('Ctrl Pts',(47.4854779994908,2.17392308734801,-3.27962205713108));
#83718=CARTESIAN_POINT('Ctrl Pts',(47.4913422674268,2.26839393475696,-3.21292358402092));
#83719=CARTESIAN_POINT('Ctrl Pts',(47.4972151701021,2.36300388412054,-3.14612690190518));
#83720=CARTESIAN_POINT('Ctrl Pts',(47.5030880727774,2.45453841736447,-3.07523431262208));
#83721=CARTESIAN_POINT('Ctrl Pts',(47.5089609754527,2.54264174438561,-3.00057693780841));
#83722=CARTESIAN_POINT('Ctrl Pts',(47.5105551911537,2.56655763658064,-2.9803109865898));
#83723=CARTESIAN_POINT('Ctrl Pts',(47.5121494068548,2.59022091086395,-2.95976782459626));
#83724=CARTESIAN_POINT('Ctrl Pts',(47.5137436225559,2.61362494454484,-2.93895451636343));
#83725=CARTESIAN_POINT('Ctrl Pts',(47.5196158969124,2.69983342105921,-2.8622889458707));
#83726=CARTESIAN_POINT('Ctrl Pts',(47.525488171269,2.78281016550265,-2.78169862677287));
#83727=CARTESIAN_POINT('Ctrl Pts',(47.5313604456256,2.86217652834462,-2.69748670443306));
#83728=CARTESIAN_POINT('Ctrl Pts',(47.5372251125981,2.94144007405476,-2.61338387652585));
#83729=CARTESIAN_POINT('Ctrl Pts',(47.5430897795706,3.01710225844809,-2.52566907353751));
#83730=CARTESIAN_POINT('Ctrl Pts',(47.5489544465431,3.08881828540358,-2.43468490769473));
#83731=CARTESIAN_POINT('Ctrl Pts',(47.5548130846949,3.16046058897979,-2.3437942726909));
#83732=CARTESIAN_POINT('Ctrl Pts',(47.5606717228466,3.22816454956605,-2.24964128248949));
#83733=CARTESIAN_POINT('Ctrl Pts',(47.5665303609984,3.29162344160212,-2.15260403202619));
#83734=CARTESIAN_POINT('Ctrl Pts',(47.5726162143441,3.35754345584558,-2.05180339199845));
#83735=CARTESIAN_POINT('Ctrl Pts',(47.5787020676899,3.41888215100117,-1.94789057282718));
#83736=CARTESIAN_POINT('Ctrl Pts',(47.5847879210356,3.47534286242914,-1.84132587788334));
#83737=CARTESIAN_POINT('Ctrl Pts',(47.5906397802171,3.52963272348791,-1.73885847469354));
#83738=CARTESIAN_POINT('Ctrl Pts',(47.5964916393985,3.57941256880411,-1.63393975254393));
#83739=CARTESIAN_POINT('Ctrl Pts',(47.60234349858,3.62446426942557,-1.52700614263904));
#83740=CARTESIAN_POINT('Ctrl Pts',(47.6081944687424,3.66950912575675,-1.42008877817344));
#83741=CARTESIAN_POINT('Ctrl Pts',(47.6140454389048,3.70982710515734,-1.31115751543514));
#83742=CARTESIAN_POINT('Ctrl Pts',(47.6198964090671,3.74524781942878,-1.20066971772589));
#83743=CARTESIAN_POINT('Ctrl Pts',(47.625747907276,3.78067173039812,-1.09017194856016));
#83744=CARTESIAN_POINT('Ctrl Pts',(47.6315994054849,3.81119737142664,-0.978117758842683));
#83745=CARTESIAN_POINT('Ctrl Pts',(47.6374509036937,3.83670413885191,-0.864979971396215));
#83746=CARTESIAN_POINT('Ctrl Pts',(47.6433043470545,3.8622193852233,-0.751804574746371));
#83747=CARTESIAN_POINT('Ctrl Pts',(47.6491577904153,3.88271234967359,-0.637545267163114));
#83748=CARTESIAN_POINT('Ctrl Pts',(47.6550112337761,3.89811361379941,-0.522684660107483));
#83749=CARTESIAN_POINT('Ctrl Pts',(47.6608713339294,3.91353239291821,-0.407693428532405));
#83750=CARTESIAN_POINT('Ctrl Pts',(47.6667314340827,3.92384785909345,-0.292099942553816));
#83751=CARTESIAN_POINT('Ctrl Pts',(47.672591534236,3.92904250328329,-0.176391630735043));
#83752=CARTESIAN_POINT('Ctrl Pts',(47.6784555826383,3.93424064737041,-0.0606053603129594));
#83753=CARTESIAN_POINT('Ctrl Pts',(47.6843196310405,3.93431109927501,0.0552954776255242));
#83754=CARTESIAN_POINT('Ctrl Pts',(47.6901836794428,3.92928844000814,0.17082551102922));
#83755=CARTESIAN_POINT('Ctrl Pts',(47.6960563662491,3.92425838179826,0.286525733189095));
#83756=CARTESIAN_POINT('Ctrl Pts',(47.7019290530553,3.91412027454157,0.401853650390887));
#83757=CARTESIAN_POINT('Ctrl Pts',(47.7078017398616,3.89896028938375,0.516330961504905));
#83758=CARTESIAN_POINT('Ctrl Pts',(47.7093981070062,3.89483936432548,0.547449225478263));
#83759=CARTESIAN_POINT('Ctrl Pts',(47.7109944741509,3.89034765612506,0.578504709157234));
#83760=CARTESIAN_POINT('Ctrl Pts',(47.7125908412955,3.88548753675185,0.60948798326632));
#83761=CARTESIAN_POINT('Ctrl Pts',(47.7184634438457,3.86760847332902,0.723467060796133));
#83762=CARTESIAN_POINT('Ctrl Pts',(47.7243360463959,3.8446799400168,0.836849554227666));
#83763=CARTESIAN_POINT('Ctrl Pts',(47.7302086489461,3.81675223316005,0.949152985913109));
#83764=CARTESIAN_POINT('Ctrl Pts',(47.7360736434181,3.78886070722584,1.06131092617733));
#83765=CARTESIAN_POINT('Ctrl Pts',(47.7419386378901,3.75598298611239,1.17239218729747));
#83766=CARTESIAN_POINT('Ctrl Pts',(47.747803632362,3.71822087056931,1.28192143193832));
#83767=CARTESIAN_POINT('Ctrl Pts',(47.7536625969548,3.68049757876209,1.3913380680984));
#83768=CARTESIAN_POINT('Ctrl Pts',(47.7595215615475,3.63790001490782,1.49920547319908));
#83769=CARTESIAN_POINT('Ctrl Pts',(47.7653805261403,3.59058041276574,1.60506115131575));
#83770=CARTESIAN_POINT('Ctrl Pts',(47.7714662567192,3.54142934773005,1.71501387881092));
#83771=CARTESIAN_POINT('Ctrl Pts',(47.7775519872982,3.48718344368452,1.82279556769424));
#83772=CARTESIAN_POINT('Ctrl Pts',(47.7836377178771,3.42806947800816,1.9279078437386));
#83773=CARTESIAN_POINT('Ctrl Pts',(47.7894898988744,3.37122410470161,2.02898626915768));
#83774=CARTESIAN_POINT('Ctrl Pts',(47.7953420798716,3.30987764434753,2.12759599818236));
#83775=CARTESIAN_POINT('Ctrl Pts',(47.8011942608689,3.24427930421203,2.22331752034241));
#83776=CARTESIAN_POINT('Ctrl Pts',(47.8070455506096,3.17869095436124,2.31902446461439));
#83777=CARTESIAN_POINT('Ctrl Pts',(47.8128968403502,3.10885224584378,2.41184373574585));
#83778=CARTESIAN_POINT('Ctrl Pts',(47.8187481300908,3.0350558082925,2.50138466465075));
#83779=CARTESIAN_POINT('Ctrl Pts',(47.8245999453131,2.96125274336959,2.59093363487894));
#83780=CARTESIAN_POINT('Ctrl Pts',(47.8304517605354,2.8834915057514,2.67720335862645));
#83781=CARTESIAN_POINT('Ctrl Pts',(47.8363035757576,2.80210464943293,2.75983668604256));
#83782=CARTESIAN_POINT('Ctrl Pts',(47.8421573332373,2.72069078026094,2.84249744002445));
#83783=CARTESIAN_POINT('Ctrl Pts',(47.8480110907171,2.63564918945304,2.92151910340916));
#83784=CARTESIAN_POINT('Ctrl Pts',(47.8538648481968,2.54734834294464,2.99658228982573));
#83785=CARTESIAN_POINT('Ctrl Pts',(47.8597252566187,2.45894717047799,3.07173076179056));
#83786=CARTESIAN_POINT('Ctrl Pts',(47.8655856650406,2.36727966612812,3.14291151194314));
#83787=CARTESIAN_POINT('Ctrl Pts',(47.8714460734626,2.27274641734158,3.20984621476809));
#83788=CARTESIAN_POINT('Ctrl Pts',(47.8773104271116,2.17814952876956,3.27682597803667));
#83789=CARTESIAN_POINT('Ctrl Pts',(47.8831747807606,2.0806834010134,3.33955377909172));
#83790=CARTESIAN_POINT('Ctrl Pts',(47.8890391344097,1.98077505993792,3.39779622136583));
#83791=CARTESIAN_POINT('Ctrl Pts',(47.8949121196797,1.88071966583925,3.45612438948748));
#83792=CARTESIAN_POINT('Ctrl Pts',(47.9007851049497,1.7782152487932,3.50995383127813));
#83793=CARTESIAN_POINT('Ctrl Pts',(47.9066580902197,1.67371078463081,3.55909837029135));
#83794=CARTESIAN_POINT('Ctrl Pts',(47.9082514134915,1.64535903724794,3.57243113618339));
#83795=CARTESIAN_POINT('Ctrl Pts',(47.9098447367633,1.61686017759492,3.58541936430235));
#83796=CARTESIAN_POINT('Ctrl Pts',(47.9114380600352,1.58822336681766,3.59805996852392));
#83797=CARTESIAN_POINT('Ctrl Pts',(47.9173108113641,1.48267236437856,3.64465134552468));
#83798=CARTESIAN_POINT('Ctrl Pts',(47.9231835626931,1.37489288537159,3.68667213053081));
#83799=CARTESIAN_POINT('Ctrl Pts',(47.9290563140221,1.26531802826798,3.72390376988182));
#83800=CARTESIAN_POINT('Ctrl Pts',(47.9349214607175,1.15588505979396,3.76108719793304));
#83801=CARTESIAN_POINT('Ctrl Pts',(47.9407866074129,1.04466172424185,3.79349368113952));
#83802=CARTESIAN_POINT('Ctrl Pts',(47.9466517541083,0.932102958880354,3.82095185445283));
#83803=CARTESIAN_POINT('Ctrl Pts',(47.9525108741465,0.819659851852007,3.84838181346806));
#83804=CARTESIAN_POINT('Ctrl Pts',(47.9583699941848,0.705884443535285,3.8708734787474));
#83805=CARTESIAN_POINT('Ctrl Pts',(47.964229114223,0.591248135025886,3.88830485466719));
#83806=CARTESIAN_POINT('Ctrl Pts',(47.970314787746,0.472179206088296,3.90641024629804));
#83807=CARTESIAN_POINT('Ctrl Pts',(47.976400461269,0.352181886539044,3.91905597209619));
#83808=CARTESIAN_POINT('Ctrl Pts',(47.982486134792,0.231798005776437,3.92616335428342));
#83809=CARTESIAN_POINT('Ctrl Pts',(47.9883384782184,0.116029749301907,3.93299823316174));
#83810=CARTESIAN_POINT('Ctrl Pts',(47.9941908216448,-9.55212978881598E-5,
3.93471161259046));
#83811=CARTESIAN_POINT('Ctrl Pts',(48.0000431650713,-0.116090136285115,
3.93128631369649));
#83812=CARTESIAN_POINT('Ctrl Pts',(48.0058946195261,-0.232067131677432,
3.92786153510579));
#83813=CARTESIAN_POINT('Ctrl Pts',(48.0117460739809,-0.34791309790432,3.91929964241296));
#83814=CARTESIAN_POINT('Ctrl Pts',(48.0175975284357,-0.463141150386326,
3.9056355788551));
#83815=CARTESIAN_POINT('Ctrl Pts',(48.0234495104708,-0.578379592089053,
3.8919702833145));
#83816=CARTESIAN_POINT('Ctrl Pts',(48.029301492506,-0.692999598839239,3.87320195109583));
#83817=CARTESIAN_POINT('Ctrl Pts',(48.0351534745411,-0.806520897288482,
3.84941723410661));
#83818=CARTESIAN_POINT('Ctrl Pts',(48.0410074007474,-0.920079910283162,
3.82562461525403));
#83819=CARTESIAN_POINT('Ctrl Pts',(48.0468613269538,-1.03253908484983,3.7968123824681));
#83820=CARTESIAN_POINT('Ctrl Pts',(48.0527152531602,-1.14343049832214,3.76311781578876));
#83821=CARTESIAN_POINT('Ctrl Pts',(48.058575832263,-1.25444793816839,3.72938495575625));
#83822=CARTESIAN_POINT('Ctrl Pts',(48.0644364113658,-1.36389366494346,3.69075880703968));
#83823=CARTESIAN_POINT('Ctrl Pts',(48.0702969904686,-1.47131692950533,3.6474258721667));
#83824=CARTESIAN_POINT('Ctrl Pts',(48.0761615161443,-1.57881253397215,3.60406375646029));
#83825=CARTESIAN_POINT('Ctrl Pts',(48.0820260418199,-1.68428258914526,3.55598871427612));
#83826=CARTESIAN_POINT('Ctrl Pts',(48.0878905674956,-1.78729984590362,3.50343378142543));
#83827=CARTESIAN_POINT('Ctrl Pts',(48.0937637254089,-1.89046873802004,3.45080149079692));
#83828=CARTESIAN_POINT('Ctrl Pts',(48.0996368833223,-1.99117726797664,3.39367635205968));
#83829=CARTESIAN_POINT('Ctrl Pts',(48.1055100412357,-2.0890260407125,3.33233539746902));
#83830=CARTESIAN_POINT('Ctrl Pts',(48.107101787082,-2.11554505822753,3.31571074491902));
#83831=CARTESIAN_POINT('Ctrl Pts',(48.1086935329284,-2.14185420489738,3.29877666346379));
#83832=CARTESIAN_POINT('Ctrl Pts',(48.1102852787747,-2.16794595377746,3.2815391726292));
#83833=CARTESIAN_POINT('Ctrl Pts',(48.1161436697141,-2.26397614954072,3.21809690868127));
#83834=CARTESIAN_POINT('Ctrl Pts',(48.1220020606534,-2.35738380061524,3.15032696055728));
#83835=CARTESIAN_POINT('Ctrl Pts',(48.1278604515928,-2.44775204026117,3.07847347713072));
#83836=CARTESIAN_POINT('Ctrl Pts',(48.1337112415304,-2.53800303113575,3.00671322040284));
#83837=CARTESIAN_POINT('Ctrl Pts',(48.1395620314681,-2.62522212975228,2.93088021971269));
#83838=CARTESIAN_POINT('Ctrl Pts',(48.1454128214058,-2.70902024659567,2.85126258060087));
#83839=CARTESIAN_POINT('Ctrl Pts',(48.1512576052132,-2.79273234045464,2.77172667300267));
#83840=CARTESIAN_POINT('Ctrl Pts',(48.1571023890205,-2.8730301375782,2.68841413843918));
#83841=CARTESIAN_POINT('Ctrl Pts',(48.1629471728279,-2.94955709858846,2.60165368989926));
#83842=CARTESIAN_POINT('Ctrl Pts',(48.1689342272069,-3.02794683756462,2.51278136536532));
#83843=CARTESIAN_POINT('Ctrl Pts',(48.1749212815859,-3.10237944058315,2.42029137357435));
#83844=CARTESIAN_POINT('Ctrl Pts',(48.1809083359649,-3.17251110960001,2.3245778669394));
#83845=CARTESIAN_POINT('Ctrl Pts',(48.1867464677607,-3.24089831654017,2.23124514754212));
#83846=CARTESIAN_POINT('Ctrl Pts',(48.1925845995565,-3.30519578873378,2.13484775451402));
#83847=CARTESIAN_POINT('Ctrl Pts',(48.1984227313523,-3.365125676473,2.03578441430868));
#83848=CARTESIAN_POINT('Ctrl Pts',(48.2042600189846,-3.42504689866194,1.93673539814745));
#83849=CARTESIAN_POINT('Ctrl Pts',(48.2100973066169,-3.48060157694486,1.83502155671701));
#83850=CARTESIAN_POINT('Ctrl Pts',(48.2159345942492,-3.53155608365004,1.7310692152639));
#83851=CARTESIAN_POINT('Ctrl Pts',(48.2217724692948,-3.58251571796839,1.62710641296191));
#83852=CARTESIAN_POINT('Ctrl Pts',(48.2276103443403,-3.62887407771079,1.52090503610112));
#83853=CARTESIAN_POINT('Ctrl Pts',(48.2334482193859,-3.67044458102268,1.41291386065862));
#83854=CARTESIAN_POINT('Ctrl Pts',(48.2395472409308,-3.71387466360447,1.30009190052059));
#83855=CARTESIAN_POINT('Ctrl Pts',(48.2456462624756,-3.75207840010692,1.18531675855074));
#83856=CARTESIAN_POINT('Ctrl Pts',(48.2517452840205,-3.78490063685083,1.06911934280799));
#83857=CARTESIAN_POINT('Ctrl Pts',(48.2575919867618,-3.81636500537843,0.957729057636036));
#83858=CARTESIAN_POINT('Ctrl Pts',(48.2634386895031,-3.84288423206317,0.845032258677021));
#83859=CARTESIAN_POINT('Ctrl Pts',(48.2692853922444,-3.86437396766523,0.731507237169474));
#83860=CARTESIAN_POINT('Ctrl Pts',(48.2751361942627,-3.88587877028598,0.617902620284232));
#83861=CARTESIAN_POINT('Ctrl Pts',(48.280986996281,-3.90234700273276,0.503469034870847));
#83862=CARTESIAN_POINT('Ctrl Pts',(48.2868377982993,-3.91374618334939,0.388689866497759));
#83863=CARTESIAN_POINT('Ctrl Pts',(48.2926969889661,-3.92516170766029,0.273746132293219));
#83864=CARTESIAN_POINT('Ctrl Pts',(48.2985561796329,-3.93149365780932,0.158456239440373));
#83865=CARTESIAN_POINT('Ctrl Pts',(48.3044153702997,-3.93276160057252,0.0433034994225827));
#83866=CARTESIAN_POINT('Ctrl Pts',(48.3051557395079,-3.93292181822595,0.0287527623332245));
#83867=CARTESIAN_POINT('Ctrl Pts',(48.3058961087161,-3.93300124705041,0.0142042075055692));
#83868=CARTESIAN_POINT('Ctrl Pts',(48.3066364779243,-3.93299998520013,-0.000341197588803423));
#83869=CARTESIAN_POINT('',(49.2909686583561,-0.918523134026603,3.82423904224853));
#83870=CARTESIAN_POINT('Ctrl Pts',(48.306636477965,-3.93299998520006,-0.000341198387843754));
#83871=CARTESIAN_POINT('Ctrl Pts',(48.3074684844815,-3.93299856716416,-0.0166869238569671));
#83872=CARTESIAN_POINT('Ctrl Pts',(48.308300490998,-3.93289524936037,-0.033032172584711));
#83873=CARTESIAN_POINT('Ctrl Pts',(48.3091324975144,-3.93269004605578,-0.0493761243297054));
#83874=CARTESIAN_POINT('Ctrl Pts',(48.315006317975,-3.93124134662219,-0.164761564550813));
#83875=CARTESIAN_POINT('Ctrl Pts',(48.3208801384356,-3.92470779553677,-0.280276028324374));
#83876=CARTESIAN_POINT('Ctrl Pts',(48.3267539588961,-3.91307046304444,-0.395434635874443));
#83877=CARTESIAN_POINT('Ctrl Pts',(48.3326201670137,-3.90144821228079,-0.510444000384883));
#83878=CARTESIAN_POINT('Ctrl Pts',(48.3384863751313,-3.88473537506585,-0.625098018529042));
#83879=CARTESIAN_POINT('Ctrl Pts',(48.3443525832488,-3.86296501795712,-0.738911544123905));
#83880=CARTESIAN_POINT('Ctrl Pts',(48.3502127558905,-3.84121705938312,-0.852607972135366));
#83881=CARTESIAN_POINT('Ctrl Pts',(48.3560729285321,-3.81442200812411,-0.965465224274634));
#83882=CARTESIAN_POINT('Ctrl Pts',(48.3619331011737,-3.78266467860207,-1.07700368117117));
#83883=CARTESIAN_POINT('Ctrl Pts',(48.3680183768021,-3.74968747550933,-1.1928265920106));
#83884=CARTESIAN_POINT('Ctrl Pts',(48.3741036524304,-3.71135916735355,-1.30722690779745));
#83885=CARTESIAN_POINT('Ctrl Pts',(48.3801889280588,-3.66783310645094,-1.4196792959054));
#83886=CARTESIAN_POINT('Ctrl Pts',(48.3860422958279,-3.62596580946009,-1.52784616036806));
#83887=CARTESIAN_POINT('Ctrl Pts',(48.391895663597,-3.57928984325164,-1.63421042976855));
#83888=CARTESIAN_POINT('Ctrl Pts',(48.3977490313661,-3.52799211720192,-1.73832120764866));
#83889=CARTESIAN_POINT('Ctrl Pts',(48.4036014980707,-3.47670228789798,-1.84241595876874));
#83890=CARTESIAN_POINT('Ctrl Pts',(48.4094539647754,-3.42079229597198,-1.9442575376294));
#83891=CARTESIAN_POINT('Ctrl Pts',(48.41530643148,-3.3604961422573,-2.04341740177425));
#83892=CARTESIAN_POINT('Ctrl Pts',(48.4211594126556,-3.30019468810806,-2.14258598273332));
#83893=CARTESIAN_POINT('Ctrl Pts',(48.4270123938311,-3.23550652036474,-2.23907202731734));
#83894=CARTESIAN_POINT('Ctrl Pts',(48.4328653750067,-3.16670993754481,-2.33247447391283));
#83895=CARTESIAN_POINT('Ctrl Pts',(48.4387202862167,-3.0978906688882,-2.42590772018707));
#83896=CARTESIAN_POINT('Ctrl Pts',(48.4445751974267,-3.02496053617689,-2.51625501408668));
#83897=CARTESIAN_POINT('Ctrl Pts',(48.4504301086367,-2.94823877130806,-2.60314754621322));
#83898=CARTESIAN_POINT('Ctrl Pts',(48.4562916469597,-2.87143016587333,-2.6901384310911));
#83899=CARTESIAN_POINT('Ctrl Pts',(48.4621531852827,-2.79082163576131,-2.77366643923067));
#83900=CARTESIAN_POINT('Ctrl Pts',(48.4680147236056,-2.70677006513171,-2.85339881799002));
#83901=CARTESIAN_POINT('Ctrl Pts',(48.4738801946845,-2.62266210072131,-2.93318469260029));
#83902=CARTESIAN_POINT('Ctrl Pts',(48.4797456657633,-2.53510680715101,-3.0091695967008));
#83903=CARTESIAN_POINT('Ctrl Pts',(48.4856111368422,-2.44449365213772,-3.08106147044462));
#83904=CARTESIAN_POINT('Ctrl Pts',(48.4914852126711,-2.35374756601887,-3.15305881084233));
#83905=CARTESIAN_POINT('Ctrl Pts',(48.4973592885,-2.25993499882691,-3.22095089561564));
#83906=CARTESIAN_POINT('Ctrl Pts',(48.503233364329,-2.16347388609934,-3.28448926686726));
#83907=CARTESIAN_POINT('Ctrl Pts',(48.5048154816374,-2.13749315304893,-3.30160262390066));
#83908=CARTESIAN_POINT('Ctrl Pts',(48.5063975989457,-2.111320418004,-3.31840040821361));
#83909=CARTESIAN_POINT('Ctrl Pts',(48.5079797162541,-2.08496412466013,-3.33487834843795));
#83910=CARTESIAN_POINT('Ctrl Pts',(48.5138537288573,-1.987109687154,-3.39605688939871));
#83911=CARTESIAN_POINT('Ctrl Pts',(48.5197277414606,-1.88639724144626,-3.45302671887418));
#83912=CARTESIAN_POINT('Ctrl Pts',(48.5256017540639,-1.7832245806399,-3.50550981955573));
#83913=CARTESIAN_POINT('Ctrl Pts',(48.5314681776143,-1.68018521590145,-3.55792511360229));
#83914=CARTESIAN_POINT('Ctrl Pts',(48.5373346011647,-1.57469232194212,-3.60586502106239));
#83915=CARTESIAN_POINT('Ctrl Pts',(48.5432010247151,-1.46717201477847,-3.64909513154301));
#83916=CARTESIAN_POINT('Ctrl Pts',(48.5490614355031,-1.35976191003179,-3.69228093353171));
#83917=CARTESIAN_POINT('Ctrl Pts',(48.5549218462911,-1.25032890636376,-3.73076638722925));
#83918=CARTESIAN_POINT('Ctrl Pts',(48.5607822570791,-1.13932243459314,-3.76436361023118));
#83919=CARTESIAN_POINT('Ctrl Pts',(48.5668674519923,-1.02405815675097,-3.79924950098197));
#83920=CARTESIAN_POINT('Ctrl Pts',(48.5729526469054,-0.907097692538037,
-3.82886445470895));
#83921=CARTESIAN_POINT('Ctrl Pts',(48.5790378418185,-0.788965889178756,
-3.85305357161205));
#83922=CARTESIAN_POINT('Ctrl Pts',(48.5848915022426,-0.675328861601405,
-3.87632232114794));
#83923=CARTESIAN_POINT('Ctrl Pts',(48.5907451626667,-0.56060844454005,-3.89457049495094));
#83924=CARTESIAN_POINT('Ctrl Pts',(48.5965988230908,-0.445285078524572,
-3.90771163199683));
#83925=CARTESIAN_POINT('Ctrl Pts',(48.6024516019306,-0.329979080662889,
-3.92085078993566));
#83926=CARTESIAN_POINT('Ctrl Pts',(48.6083043807704,-0.214070724731052,
-3.92888439368455));
#83927=CARTESIAN_POINT('Ctrl Pts',(48.6141571596102,-0.0980470935696117,
-3.93177768540422));
#83928=CARTESIAN_POINT('Ctrl Pts',(48.6200104719687,0.0179871138977239,
-3.93467124086618));
#83929=CARTESIAN_POINT('Ctrl Pts',(48.6258637843272,0.134136204493536,-3.93242354250173));
#83930=CARTESIAN_POINT('Ctrl Pts',(48.6317170966857,0.249912275789835,-3.92505195563187));
#83931=CARTESIAN_POINT('Ctrl Pts',(48.637572357708,0.36572689084317,-3.91767791463958));
#83932=CARTESIAN_POINT('Ctrl Pts',(48.6434276187304,0.481167827619029,-3.90517661938991));
#83933=CARTESIAN_POINT('Ctrl Pts',(48.6492828797528,0.595752196064166,-3.8876173063825));
#83934=CARTESIAN_POINT('Ctrl Pts',(48.6551447934754,0.710466754340802,-3.87003804262584));
#83935=CARTESIAN_POINT('Ctrl Pts',(48.6610067071979,0.824322393184345,-3.84738935310329));
#83936=CARTESIAN_POINT('Ctrl Pts',(48.6668686209204,0.936846206648068,-3.81979164158061));
#83937=CARTESIAN_POINT('Ctrl Pts',(48.6727344827349,1.04944580668567,-3.79217534256131));
#83938=CARTESIAN_POINT('Ctrl Pts',(48.6786003445494,1.16071139970324,-3.75960350004611));
#83939=CARTESIAN_POINT('Ctrl Pts',(48.6844662063638,1.27018670565374,-3.72224592588675));
#83940=CARTESIAN_POINT('Ctrl Pts',(48.6903406921989,1.37982296277079,-3.68483342842675));
#83941=CARTESIAN_POINT('Ctrl Pts',(48.6962151780341,1.48766329643573,-3.64262130679637));
#83942=CARTESIAN_POINT('Ctrl Pts',(48.7020896638692,1.59327272284702,-3.59582689108244));
#83943=CARTESIAN_POINT('Ctrl Pts',(48.7036687542441,1.62166105051042,-3.5832483244597));
#83944=CARTESIAN_POINT('Ctrl Pts',(48.7052478446189,1.64988832874966,-3.57033891094029));
#83945=CARTESIAN_POINT('Ctrl Pts',(48.7068269349938,1.6779464473734,-3.55710341707223));
#83946=CARTESIAN_POINT('Ctrl Pts',(48.7126911328813,1.78214463804094,-3.50795135053006));
#83947=CARTESIAN_POINT('Ctrl Pts',(48.7185553307689,1.8843586773044,-3.45413329509077));
#83948=CARTESIAN_POINT('Ctrl Pts',(48.7244195286564,1.98414050183357,-3.39583207314255));
#83949=CARTESIAN_POINT('Ctrl Pts',(48.7302761014818,2.08379258268181,-3.33760665873918));
#83950=CARTESIAN_POINT('Ctrl Pts',(48.7361326743071,2.18101838292689,-3.27490987674335));
#83951=CARTESIAN_POINT('Ctrl Pts',(48.7419892471324,2.27539109351899,-3.20797200292248));
#83952=CARTESIAN_POINT('Ctrl Pts',(48.7478397827625,2.3696665208539,-3.14110313140485));
#83953=CARTESIAN_POINT('Ctrl Pts',(48.7536903183926,2.46109437200237,-3.07000210183485));
#83954=CARTESIAN_POINT('Ctrl Pts',(48.7595408540227,2.54927428133677,-2.99494401258436));
#83955=CARTESIAN_POINT('Ctrl Pts',(48.7656297415106,2.64104665579661,-2.91682804348288));
#83956=CARTESIAN_POINT('Ctrl Pts',(48.7717186289986,2.7293004301247,-2.83442597610796));
#83957=CARTESIAN_POINT('Ctrl Pts',(48.7778075164865,2.81361940131041,-2.7480965893814));
#83958=CARTESIAN_POINT('Ctrl Pts',(48.7836513016526,2.89454419323814,-2.66524230926087));
#83959=CARTESIAN_POINT('Ctrl Pts',(48.7894950868186,2.97184451333193,-2.57877109368838));
#83960=CARTESIAN_POINT('Ctrl Pts',(48.7953388719847,3.04518851884893,-2.48903914888269));
#83961=CARTESIAN_POINT('Ctrl Pts',(48.8011817918658,3.11852166437307,-2.39932049061995));
#83962=CARTESIAN_POINT('Ctrl Pts',(48.8070247117469,3.18789939764433,-2.30634238397281));
#83963=CARTESIAN_POINT('Ctrl Pts',(48.812867631628,3.25302975996991,-2.21049460093213));
#83964=CARTESIAN_POINT('Ctrl Pts',(48.8187111115083,3.31816636454202,-2.11463763161534));
#83965=CARTESIAN_POINT('Ctrl Pts',(48.8245545913885,3.37905455588627,-2.01591078213367));
#83966=CARTESIAN_POINT('Ctrl Pts',(48.8303980712687,3.43544577510909,-1.91473270361298));
#83967=CARTESIAN_POINT('Ctrl Pts',(48.8362435365058,3.49185615358228,-1.81352024924149));
#83968=CARTESIAN_POINT('Ctrl Pts',(48.8420890017429,3.54376632027041,-1.70985527188832));
#83969=CARTESIAN_POINT('Ctrl Pts',(48.84793446698,3.5909740674939,-1.6041802413028));
#83970=CARTESIAN_POINT('Ctrl Pts',(48.8537866884761,3.63823637799919,-1.49838307024645));
#83971=CARTESIAN_POINT('Ctrl Pts',(48.8596389099722,3.68078525174441,-1.39057158772529));
#83972=CARTESIAN_POINT('Ctrl Pts',(48.8654911314683,3.71846693036184,-1.2812075116098));
#83973=CARTESIAN_POINT('Ctrl Pts',(48.8713473490879,3.75617433948887,-1.1717687574674));
#83974=CARTESIAN_POINT('Ctrl Pts',(48.8772035667075,3.78900781907255,-1.06077569549521));
#83975=CARTESIAN_POINT('Ctrl Pts',(48.8830597843271,3.81686417808038,-0.948702717444605));
#83976=CARTESIAN_POINT('Ctrl Pts',(48.8889247714818,3.8447622512685,-0.836461912995315));
#83977=CARTESIAN_POINT('Ctrl Pts',(48.8947897586364,3.86766824756651,-0.723138369865339));
#83978=CARTESIAN_POINT('Ctrl Pts',(48.9006547457911,3.88553047299015,-0.609214201627749));
#83979=CARTESIAN_POINT('Ctrl Pts',(48.9023278817718,3.89062612473906,-0.576714450149148));
#83980=CARTESIAN_POINT('Ctrl Pts',(48.9040010177526,3.89531162915813,-0.544165831869741));
#83981=CARTESIAN_POINT('Ctrl Pts',(48.9056741537333,3.89958656322034,-0.511579549973744));
#83982=CARTESIAN_POINT('Ctrl Pts',(48.9115580129171,3.91462007533889,-0.396984504377214));
#83983=CARTESIAN_POINT('Ctrl Pts',(48.9174418721009,3.92462275728447,-0.281537550039955));
#83984=CARTESIAN_POINT('Ctrl Pts',(48.9233257312847,3.92950719094621,-0.165717338567898));
#83985=CARTESIAN_POINT('Ctrl Pts',(48.9292019545742,3.93438528573783,-0.0500474350596651));
#83986=CARTESIAN_POINT('Ctrl Pts',(48.9350781778637,3.93415832535556,0.0659943546379723));
#83987=CARTESIAN_POINT('Ctrl Pts',(48.9409544011532,3.92879033102886,0.181921782132266));
#83988=CARTESIAN_POINT('Ctrl Pts',(48.9468245539282,3.9234278821837,0.297729449177621));
#83989=CARTESIAN_POINT('Ctrl Pts',(48.9526947067031,3.91293498308656,0.413422580262193));
#83990=CARTESIAN_POINT('Ctrl Pts',(48.958564859478,3.89732766435233,0.528513080892061));
#83991=CARTESIAN_POINT('Ctrl Pts',(48.9646463808528,3.88115836755125,0.64774768456467));
#83992=CARTESIAN_POINT('Ctrl Pts',(48.9707279022276,3.85949937841456,0.766334992409335));
#83993=CARTESIAN_POINT('Ctrl Pts',(48.9768094236024,3.83242749655273,0.883735528122851));
#83994=CARTESIAN_POINT('Ctrl Pts',(48.9826726220244,3.80632747893706,0.996921455346187));
#83995=CARTESIAN_POINT('Ctrl Pts',(48.9885358204463,3.77519662446219,1.10900391808571));
#83996=CARTESIAN_POINT('Ctrl Pts',(48.9943990188683,3.73915597887939,1.2195087394564));
#83997=CARTESIAN_POINT('Ctrl Pts',(49.000261244185,3.70312131490247,1.32999522052602));
#83998=CARTESIAN_POINT('Ctrl Pts',(49.0061234695017,3.66217860787634,1.43890418969773));
#83999=CARTESIAN_POINT('Ctrl Pts',(49.0119856948184,3.61649870358219,1.54577686843487));
#84000=CARTESIAN_POINT('Ctrl Pts',(49.0178483522195,3.57081543237963,1.65265742438907));
#84001=CARTESIAN_POINT('Ctrl Pts',(49.0237110096207,3.52039443167278,1.7575010130483));
#84002=CARTESIAN_POINT('Ctrl Pts',(49.0295736670218,3.46545432315126,1.85986970891841));
#84003=CARTESIAN_POINT('Ctrl Pts',(49.0354381616566,3.4104969975541,1.96227048498689));
#84004=CARTESIAN_POINT('Ctrl Pts',(49.0413026562914,3.35101794255593,2.06219446346489));
#84005=CARTESIAN_POINT('Ctrl Pts',(49.0471671509262,3.2872809204378,2.15922975853095));
#84006=CARTESIAN_POINT('Ctrl Pts',(49.0530380873566,3.22347388702324,2.25637164104934));
#84007=CARTESIAN_POINT('Ctrl Pts',(49.0589090237871,3.15539977696748,2.35061816239508));
#84008=CARTESIAN_POINT('Ctrl Pts',(49.0647799602175,3.08336479279709,2.44158771182593));
#84009=CARTESIAN_POINT('Ctrl Pts',(49.0706547326819,3.01128274140875,2.53261670020381));
#84010=CARTESIAN_POINT('Ctrl Pts',(49.0765295051462,2.93523493088686,2.62036414215503));
#84011=CARTESIAN_POINT('Ctrl Pts',(49.0824042776106,2.85556568354273,2.70448398534233));
#84012=CARTESIAN_POINT('Ctrl Pts',(49.0882874421249,2.77578262952704,2.78872399282997));
#84013=CARTESIAN_POINT('Ctrl Pts',(49.0941706066392,2.69236810858523,2.86932577381937));
#84014=CARTESIAN_POINT('Ctrl Pts',(49.1000537711535,2.60570090784886,2.94598231135823));
#84015=CARTESIAN_POINT('Ctrl Pts',(49.1015429715933,2.5837629128906,2.96538631563848));
#84016=CARTESIAN_POINT('Ctrl Pts',(49.1030321720331,2.56161665519144,2.98453774370936));
#84017=CARTESIAN_POINT('Ctrl Pts',(49.104521372473,2.53926857338398,3.00343205553655));
#84018=CARTESIAN_POINT('Ctrl Pts',(49.1103447293239,2.45187882260223,3.07731621329097));
#84019=CARTESIAN_POINT('Ctrl Pts',(49.1161680861748,2.3611056470291,3.14751483806536));
#84020=CARTESIAN_POINT('Ctrl Pts',(49.1219914430257,2.2672959664739,3.21369849245557));
#84021=CARTESIAN_POINT('Ctrl Pts',(49.1278073538278,2.17360623588712,3.27979752096061));
#84022=CARTESIAN_POINT('Ctrl Pts',(49.1336232646298,2.07688805952106,3.34189154446061));
#84023=CARTESIAN_POINT('Ctrl Pts',(49.1394391754318,1.97752286652601,3.39969003180684));
#84024=CARTESIAN_POINT('Ctrl Pts',(49.1452492704114,1.87825703721406,3.45743072154399));
#84025=CARTESIAN_POINT('Ctrl Pts',(49.151059365391,1.77634981625796,3.51088420597852));
#84026=CARTESIAN_POINT('Ctrl Pts',(49.1568694603706,1.67221253818103,3.55980255451762));
#84027=CARTESIAN_POINT('Ctrl Pts',(49.1626755149881,1.56814767756246,3.60868688505151));
#84028=CARTESIAN_POINT('Ctrl Pts',(49.1684815696055,1.46185622341962,3.65304217281303));
#84029=CARTESIAN_POINT('Ctrl Pts',(49.174287624223,1.35377444905346,3.69266621035398));
#84030=CARTESIAN_POINT('Ctrl Pts',(49.1800915949038,1.24573146791119,3.73227602584714));
#84031=CARTESIAN_POINT('Ctrl Pts',(49.1858955655846,1.13589983829548,3.76715782131109));
#84032=CARTESIAN_POINT('Ctrl Pts',(49.1916995362654,1.02473552523914,3.79715763477273));
#84033=CARTESIAN_POINT('Ctrl Pts',(49.1975028869562,0.913583086942417,3.82715424360365));
#84034=CARTESIAN_POINT('Ctrl Pts',(49.2033062376471,0.801098654615878,3.852269797829));
#84035=CARTESIAN_POINT('Ctrl Pts',(49.2091095883379,0.687752267144868,3.87240052409834));
#84036=CARTESIAN_POINT('Ctrl Pts',(49.2149137821895,0.574389411733869,3.89253417513308));
#84037=CARTESIAN_POINT('Ctrl Pts',(49.2207179760412,0.460164766805947,3.90768148593855));
#84038=CARTESIAN_POINT('Ctrl Pts',(49.2265221698928,0.345556637970963,3.91779014368486));
#84039=CARTESIAN_POINT('Ctrl Pts',(49.232332094217,0.230835356689904,3.92790878169488));
#84040=CARTESIAN_POINT('Ctrl Pts',(49.2381420185411,0.115730255415686,3.93297879649116));
#84041=CARTESIAN_POINT('Ctrl Pts',(49.2439519428653,0.000722841650785665,
3.93299993357487));
#84042=CARTESIAN_POINT('Ctrl Pts',(49.2497649212577,-0.114345027376021,
3.93302108176958));
#84043=CARTESIAN_POINT('Ctrl Pts',(49.2555778996502,-0.229314686452266,
3.92798808630921));
#84044=CARTESIAN_POINT('Ctrl Pts',(49.2613908780426,-0.343708406002381,
3.91795272197653));
#84045=CARTESIAN_POINT('Ctrl Pts',(49.2672127549553,-0.458277239711371,
3.90790199548594));
#84046=CARTESIAN_POINT('Ctrl Pts',(49.2730346318679,-0.572267956320908,
3.89283366289546));
#84047=CARTESIAN_POINT('Ctrl Pts',(49.2788565087805,-0.68521144197363,3.87285092403367));
#84048=CARTESIAN_POINT('Ctrl Pts',(49.2828938919724,-0.763536033415078,
3.85899319821454));
#84049=CARTESIAN_POINT('Ctrl Pts',(49.2869312751642,-0.841357213550516,
3.84277310414495));
#84050=CARTESIAN_POINT('Ctrl Pts',(49.2909686583561,-0.918523134026603,
3.82423904224853));
#84051=CARTESIAN_POINT('',(49.291,2.49116634986212,3.04344857313454));
#84052=CARTESIAN_POINT('Origin',(49.291,0.,0.));
#84053=CARTESIAN_POINT('',(48.4899635220349,-3.93640077382959,-0.000934446622206373));
#84054=CARTESIAN_POINT('Ctrl Pts',(49.291,2.49116634986212,3.04344857313454));
#84055=CARTESIAN_POINT('Ctrl Pts',(49.2247175937535,3.50515732392066,2.213462413376));
#84056=CARTESIAN_POINT('Ctrl Pts',(49.0921527812602,4.62042791627047,-0.525508407013305));
#84057=CARTESIAN_POINT('Ctrl Pts',(48.8933055625208,2.05138932172835,-4.17834256249585));
#84058=CARTESIAN_POINT('Ctrl Pts',(48.694458343781,-2.40332474549236,-3.98116326218143));
#84059=CARTESIAN_POINT('Ctrl Pts',(48.5600109969525,-3.92216493045881,-1.37922589845858));
#84060=CARTESIAN_POINT('Ctrl Pts',(48.4918460563704,-3.93942359247251,-0.0379796677341524));
#84061=CARTESIAN_POINT('Ctrl Pts',(48.4899635220349,-3.93933315937227,-0.000935142729620586));
#84062=CARTESIAN_POINT('',(47.2399635542899,-3.93231350106613,-0.00327549983485499));
#84063=CARTESIAN_POINT('Ctrl Pts',(48.4899635220349,-3.93299988918353,-0.000933639299641673));
#84064=CARTESIAN_POINT('Ctrl Pts',(48.4841266678079,-3.93302711093771,0.113739292968427));
#84065=CARTESIAN_POINT('Ctrl Pts',(48.478289813581,-3.92803487061338,0.228617479894471));
#84066=CARTESIAN_POINT('Ctrl Pts',(48.472452959354,-3.91799539673541,0.34322160648788));
#84067=CARTESIAN_POINT('Ctrl Pts',(48.4666237055437,-3.90796899568411,0.457676502165316));
#84068=CARTESIAN_POINT('Ctrl Pts',(48.4607944517333,-3.89290846354109,0.571857633777924));
#84069=CARTESIAN_POINT('Ctrl Pts',(48.4549651979229,-3.87283801159206,0.685284419761366));
#84070=CARTESIAN_POINT('Ctrl Pts',(48.4491419268033,-3.85278815838713,0.798594793351819));
#84071=CARTESIAN_POINT('Ctrl Pts',(48.4433186556837,-3.82773868257875,0.911151950930715));
#84072=CARTESIAN_POINT('Ctrl Pts',(48.4374953845641,-3.79776563490822,1.02247991780288));
#84073=CARTESIAN_POINT('Ctrl Pts',(48.4316315729698,-3.76758392074174,1.13458292820758));
#84074=CARTESIAN_POINT('Ctrl Pts',(48.4257677613755,-3.73240984801752,1.24543913760885));
#84075=CARTESIAN_POINT('Ctrl Pts',(48.4199039497813,-3.69237365308898,1.3545721855901));
#84076=CARTESIAN_POINT('Ctrl Pts',(48.4140871743393,-3.65265860568199,1.46282983050319));
#84077=CARTESIAN_POINT('Ctrl Pts',(48.4082703988973,-3.60815931243622,1.56939146215388));
#84078=CARTESIAN_POINT('Ctrl Pts',(48.4024536234553,-3.55905282173006,1.67380763892846));
#84079=CARTESIAN_POINT('Ctrl Pts',(48.396637633795,-3.50995296476548,1.7782097102371));
#84080=CARTESIAN_POINT('Ctrl Pts',(48.3908216441348,-3.45624732587386,1.88046652385039));
#84081=CARTESIAN_POINT('Ctrl Pts',(48.3850056544745,-3.39816041180273,1.98015020027692));
#84082=CARTESIAN_POINT('Ctrl Pts',(48.3791889988926,-3.34006684687096,2.07984529032817));
#84083=CARTESIAN_POINT('Ctrl Pts',(48.3733723433106,-3.27759122087877,2.17696629582394));
#84084=CARTESIAN_POINT('Ctrl Pts',(48.3675556877287,-3.21100274889135,2.27111213871359));
#84085=CARTESIAN_POINT('Ctrl Pts',(48.3616563726098,-3.14346799906705,2.36659587271112));
#84086=CARTESIAN_POINT('Ctrl Pts',(48.3557570574909,-3.07170285443242,2.45901886339764));
#84087=CARTESIAN_POINT('Ctrl Pts',(48.349857742372,-2.9960312515734,2.5479964167156));
#84088=CARTESIAN_POINT('Ctrl Pts',(48.3440322443374,-2.92130651406732,2.63586060968115));
#84089=CARTESIAN_POINT('Ctrl Pts',(48.3382067463029,-2.84277285759069,2.72036483345076));
#84090=CARTESIAN_POINT('Ctrl Pts',(48.3323812482684,-2.76077939831325,2.80117584486393));
#84091=CARTESIAN_POINT('Ctrl Pts',(48.3264450246073,-2.6772274839308,2.88352283651732));
#84092=CARTESIAN_POINT('Ctrl Pts',(48.3205088009462,-2.59008325111016,2.96203448838341));
#84093=CARTESIAN_POINT('Ctrl Pts',(48.3145725772851,-2.49975036241423,3.03640200329435));
#84094=CARTESIAN_POINT('Ctrl Pts',(48.308636353624,-2.40941747371832,3.11076951820526));
#84095=CARTESIAN_POINT('Ctrl Pts',(48.3027001299629,-2.3158963318695,3.18099267867581));
#84096=CARTESIAN_POINT('Ctrl Pts',(48.2967639063018,-2.21961939102252,3.24681055175642));
#84097=CARTESIAN_POINT('Ctrl Pts',(48.2908898279569,-2.12435035709865,3.3119393887152));
#84098=CARTESIAN_POINT('Ctrl Pts',(48.2850157496119,-2.02605343213304,3.37298018509058));
#84099=CARTESIAN_POINT('Ctrl Pts',(48.2791416712669,-1.92511465841178,3.42963883695763));
#84100=CARTESIAN_POINT('Ctrl Pts',(48.273275194168,-1.82430650270457,3.48622417071002));
#84101=CARTESIAN_POINT('Ctrl Pts',(48.267408717069,-1.72086365371022,3.53843843664275));
#84102=CARTESIAN_POINT('Ctrl Pts',(48.26154223997,-1.61520224345694,3.58602993751191));
#84103=CARTESIAN_POINT('Ctrl Pts',(48.2556817877773,-1.50964934809005,3.63357256163129));
#84104=CARTESIAN_POINT('Ctrl Pts',(48.2498213355846,-1.40188279793812,3.67650169542959));
#84105=CARTESIAN_POINT('Ctrl Pts',(48.243960883392,-1.29234393088991,3.71461117269251));
#84106=CARTESIAN_POINT('Ctrl Pts',(48.2378757085657,-1.17860472880421,3.75418198123374));
#84107=CARTESIAN_POINT('Ctrl Pts',(48.2317905337395,-1.06295496255167,3.78855588415592));
#84108=CARTESIAN_POINT('Ctrl Pts',(48.2257053589132,-0.945912664613604,
3.8175565786146));
#84109=CARTESIAN_POINT('Ctrl Pts',(48.219851687597,-0.833323106912179,3.84545397485219));
#84110=CARTESIAN_POINT('Ctrl Pts',(48.2139980162808,-0.719445474591379,
3.86837942247393));
#84111=CARTESIAN_POINT('Ctrl Pts',(48.2081443449646,-0.60475625264573,3.88622681722077));
#84112=CARTESIAN_POINT('Ctrl Pts',(48.2022915665054,-0.49008452417913,3.90407148971507));
#84113=CARTESIAN_POINT('Ctrl Pts',(48.1964387880463,-0.374601860298475,
3.91683958592564));
#84114=CARTESIAN_POINT('Ctrl Pts',(48.1905860095871,-0.258793506260321,
3.92447638814626));
#84115=CARTESIAN_POINT('Ctrl Pts',(48.1847327088812,-0.142974818578138,
3.932113871803));
#84116=CARTESIAN_POINT('Ctrl Pts',(48.1788794081753,-0.0268307951890033,
3.93461912408343));
#84117=CARTESIAN_POINT('Ctrl Pts',(48.1730261074695,0.0891503589144591,
3.9319894727104));
#84118=CARTESIAN_POINT('Ctrl Pts',(48.1671708693795,0.205169901621544,3.92935895094904));
#84119=CARTESIAN_POINT('Ctrl Pts',(48.1613156312896,0.3210260550782,3.92159015529858));
#84120=CARTESIAN_POINT('Ctrl Pts',(48.1554603931996,0.436233491927892,3.90873244678123));
#84121=CARTESIAN_POINT('Ctrl Pts',(48.1495985190088,0.551571500440835,3.89586016583321));
#84122=CARTESIAN_POINT('Ctrl Pts',(48.1437366448179,0.666258914056482,3.87788750592427));
#84123=CARTESIAN_POINT('Ctrl Pts',(48.1378747706271,0.779818280783277,3.85491536210021));
#84124=CARTESIAN_POINT('Ctrl Pts',(48.1320089580572,0.893453943896832,3.83192778413259));
#84125=CARTESIAN_POINT('Ctrl Pts',(48.1261431454874,1.0059596510704,3.80393413323241));
#84126=CARTESIAN_POINT('Ctrl Pts',(48.1202773329176,1.11687253241484,3.7710853538918));
#84127=CARTESIAN_POINT('Ctrl Pts',(48.1144029101881,1.22794821773791,3.73818835732065));
#84128=CARTESIAN_POINT('Ctrl Pts',(48.1085284874585,1.3374260218931,3.70042214311632));
#84129=CARTESIAN_POINT('Ctrl Pts',(48.102654064729,1.44486240208544,3.65798600858996));
#84130=CARTESIAN_POINT('Ctrl Pts',(48.1010749390067,1.47374278051279,3.64657859127079));
#84131=CARTESIAN_POINT('Ctrl Pts',(48.0994958132844,1.50247578059378,3.6348339790261));
#84132=CARTESIAN_POINT('Ctrl Pts',(48.0979166875621,1.53105310235788,3.62275660205876));
#84133=CARTESIAN_POINT('Ctrl Pts',(48.0920430178542,1.63734846998385,3.57783394501977));
#84134=CARTESIAN_POINT('Ctrl Pts',(48.0861693481464,1.7418421306723,3.52815426272047));
#84135=CARTESIAN_POINT('Ctrl Pts',(48.0802956784385,1.84407800639631,3.47388331789158));
#84136=CARTESIAN_POINT('Ctrl Pts',(48.074429592217,1.94618188552957,3.41968244220078));
#84137=CARTESIAN_POINT('Ctrl Pts',(48.0685635059956,2.04603341512508,3.3609022843018));
#84138=CARTESIAN_POINT('Ctrl Pts',(48.0626974197741,2.14319592845312,3.29775684553334));
#84139=CARTESIAN_POINT('Ctrl Pts',(48.056837340294,2.24025894953682,3.23467606628434));
#84140=CARTESIAN_POINT('Ctrl Pts',(48.0509772608139,2.33463808690553,3.16723912104829));
#84141=CARTESIAN_POINT('Ctrl Pts',(48.0451171813337,2.42592135437328,3.09570582943466));
#84142=CARTESIAN_POINT('Ctrl Pts',(48.0390318599791,2.52071324563104,3.0214230371108));
#84143=CARTESIAN_POINT('Ctrl Pts',(48.0329465386245,2.61216609972045,2.94272289146592));
#84144=CARTESIAN_POINT('Ctrl Pts',(48.0268612172698,2.69985149461221,2.85994596225876));
#84145=CARTESIAN_POINT('Ctrl Pts',(48.0210078704915,2.78419429161251,2.7803245185161));
#84146=CARTESIAN_POINT('Ctrl Pts',(48.0151545237132,2.86505127847718,2.6969317292472));
#84147=CARTESIAN_POINT('Ctrl Pts',(48.0093011769348,2.94207565639376,2.61011107657418));
#84148=CARTESIAN_POINT('Ctrl Pts',(48.0034487045672,3.01908852791185,2.52330339373037));
#84149=CARTESIAN_POINT('Ctrl Pts',(47.9975962321996,3.0922696547716,2.43306917464447));
#84150=CARTESIAN_POINT('Ctrl Pts',(47.991743759832,3.16131073701573,2.33978704672649));
#84151=CARTESIAN_POINT('Ctrl Pts',(47.9858907463462,3.230358202781,2.24649629396638));
#84152=CARTESIAN_POINT('Ctrl Pts',(47.9800377328605,3.29526461715692,2.15015740425872));
#84153=CARTESIAN_POINT('Ctrl Pts',(47.9741847193747,3.35576386897012,2.05117962541429));
#84154=CARTESIAN_POINT('Ctrl Pts',(47.9683297491939,3.41628334602088,1.95216875774593));
#84155=CARTESIAN_POINT('Ctrl Pts',(47.9624747790131,3.47239251545957,1.85051759905071));
#84156=CARTESIAN_POINT('Ctrl Pts',(47.9566198088323,3.52387060001388,1.7466610988849));
#84157=CARTESIAN_POINT('Ctrl Pts',(47.950758172327,3.57540729624365,1.64268635027346));
#84158=CARTESIAN_POINT('Ctrl Pts',(47.9448965358218,3.62230219956516,1.53650161880801));
#84159=CARTESIAN_POINT('Ctrl Pts',(47.9390348993165,3.66438214697297,1.42856308259236));
#84160=CARTESIAN_POINT('Ctrl Pts',(47.9331693071063,3.7064904918869,1.32055170443102));
#84161=CARTESIAN_POINT('Ctrl Pts',(47.9273037148961,3.74377727813839,1.21078455505471));
#84162=CARTESIAN_POINT('Ctrl Pts',(47.9214381226858,3.77611933416747,1.09973259209983));
#84163=CARTESIAN_POINT('Ctrl Pts',(47.9155638930086,3.80850901598256,0.988517097889588));
#84164=CARTESIAN_POINT('Ctrl Pts',(47.9096896633315,3.83593933774177,0.876013413978493));
#84165=CARTESIAN_POINT('Ctrl Pts',(47.9038154336543,3.85833825570205,0.762702369595143));
#84166=CARTESIAN_POINT('Ctrl Pts',(47.902233445377,3.86437050632624,0.732186582206608));
#84167=CARTESIAN_POINT('Ctrl Pts',(47.9006514570997,3.87003813163025,0.701612262918697));
#84168=CARTESIAN_POINT('Ctrl Pts',(47.8990694688225,3.87534036911817,0.670988840058476));
#84169=CARTESIAN_POINT('Ctrl Pts',(47.8931981591211,3.8950188198683,0.557334647856081));
#84170=CARTESIAN_POINT('Ctrl Pts',(47.8873268494198,3.909726305003,0.442623035810078));
#84171=CARTESIAN_POINT('Ctrl Pts',(47.8814555397185,3.9193553223701,0.327326835149767));
#84172=CARTESIAN_POINT('Ctrl Pts',(47.87559185214,3.92897183936552,0.212180311793679));
#84173=CARTESIAN_POINT('Ctrl Pts',(47.8697281645615,3.93352296520263,0.0964511172989043));
#84174=CARTESIAN_POINT('Ctrl Pts',(47.8638644769831,3.93295226119242,-0.019378110884881));
#84175=CARTESIAN_POINT('Ctrl Pts',(47.8580068317063,3.93238214527045,-0.13508798156012));
#84176=CARTESIAN_POINT('Ctrl Pts',(47.8521491864295,3.92670069934096,-0.250897269853491));
#84177=CARTESIAN_POINT('Ctrl Pts',(47.8462915411528,3.91590336792172,-0.366319277542559));
#84178=CARTESIAN_POINT('Ctrl Pts',(47.8402053206915,3.90468470644504,-0.486245246371798));
#84179=CARTESIAN_POINT('Ctrl Pts',(47.8341191002303,3.88794272894013,-0.605752641170845));
#84180=CARTESIAN_POINT('Ctrl Pts',(47.828032879769,3.86573198890414,-0.724296341260414));
#84181=CARTESIAN_POINT('Ctrl Pts',(47.822182040935,3.84438023847664,-0.83825542119042));
#84182=CARTESIAN_POINT('Ctrl Pts',(47.8163312021009,3.81797495370962,-0.951323518056299));
#84183=CARTESIAN_POINT('Ctrl Pts',(47.8104803632669,3.78661724024109,-1.06302345971712));
#84184=CARTESIAN_POINT('Ctrl Pts',(47.8046304218782,3.75526433665275,-1.17470626800698));
#84185=CARTESIAN_POINT('Ctrl Pts',(47.7987804804895,3.71896062650313,-1.28502094031307));
#84186=CARTESIAN_POINT('Ctrl Pts',(47.7929305391008,3.67785760393822,-1.39350365810566));
#84187=CARTESIAN_POINT('Ctrl Pts',(47.7870800770231,3.63675092289358,-1.5019960316802));
#84188=CARTESIAN_POINT('Ctrl Pts',(47.7812296149454,3.59084422679533,-1.60865573986473));
#84189=CARTESIAN_POINT('Ctrl Pts',(47.7753791528677,3.54033758856154,-1.71303787436771));
#84190=CARTESIAN_POINT('Ctrl Pts',(47.7695267519312,3.48981421229293,-1.8174546013889));
#84191=CARTESIAN_POINT('Ctrl Pts',(47.7636743509948,3.43468804270889,-1.91959188182632));
#84192=CARTESIAN_POINT('Ctrl Pts',(47.7578219500583,3.37520529466236,-2.01902902873712));
#84193=CARTESIAN_POINT('Ctrl Pts',(47.751962896438,3.31565492993703,-2.1185792102646));
#84194=CARTESIAN_POINT('Ctrl Pts',(47.7461038428178,3.25173831453506,-2.21542277683459));
#84195=CARTESIAN_POINT('Ctrl Pts',(47.7402447891975,3.18374527432843,-2.30916760504546));
#84196=CARTESIAN_POINT('Ctrl Pts',(47.7343817910201,3.11570645839669,-2.40297554614955));
#84197=CARTESIAN_POINT('Ctrl Pts',(47.7285187928428,3.04358600977531,-2.49368027200128));
#84198=CARTESIAN_POINT('Ctrl Pts',(47.7226557946655,2.96771322403652,-2.58092371446324));
#84199=CARTESIAN_POINT('Ctrl Pts',(47.7167841553799,2.89172861412003,-2.66829573960631));
#84200=CARTESIAN_POINT('Ctrl Pts',(47.7109125160944,2.81198091350175,-2.75219600145978));
#84201=CARTESIAN_POINT('Ctrl Pts',(47.7050408768089,2.72883537233496,-2.8323040992615));
#84202=CARTESIAN_POINT('Ctrl Pts',(47.7034346679002,2.70609059827031,-2.85421796932213));
#84203=CARTESIAN_POINT('Ctrl Pts',(47.7018284589915,2.68309174140948,-2.87584830433206));
#84204=CARTESIAN_POINT('Ctrl Pts',(47.7002222500828,2.65984667742076,-2.89718909507367));
#84205=CARTESIAN_POINT('Ctrl Pts',(47.6943494954793,2.5748561411265,-2.97521706913959));
#84206=CARTESIAN_POINT('Ctrl Pts',(47.6884767408758,2.4862870283832,-3.04963254301817));
#84207=CARTESIAN_POINT('Ctrl Pts',(47.6826039862723,2.39447927651606,-3.12008942088766));
#84208=CARTESIAN_POINT('Ctrl Pts',(47.6767388368527,2.3027904151666,-3.19045505750015));
#84209=CARTESIAN_POINT('Ctrl Pts',(47.670873687433,2.20787157999033,-3.25687204332534));
#84210=CARTESIAN_POINT('Ctrl Pts',(47.6650085380134,2.11009854825462,-3.31903195475032));
#84211=CARTESIAN_POINT('Ctrl Pts',(47.6591494157994,2.01242599105466,-3.38112798876318));
#84212=CARTESIAN_POINT('Ctrl Pts',(47.6532902935853,1.91190541802128,-3.43897542950064));
#84213=CARTESIAN_POINT('Ctrl Pts',(47.6474311713713,1.80894405682423,-3.49230731741642));
#84214=CARTESIAN_POINT('Ctrl Pts',(47.6413454988701,1.70200156584504,-3.5477013494691));
#84215=CARTESIAN_POINT('Ctrl Pts',(47.635259826369,1.59242608449288,-3.59822330392868));
#84216=CARTESIAN_POINT('Ctrl Pts',(47.6291741538678,1.48070545057497,-3.6436246196113));
#84217=CARTESIAN_POINT('Ctrl Pts',(47.6233218096457,1.3732682517648,-3.68728522202805));
#84218=CARTESIAN_POINT('Ctrl Pts',(47.6174694654236,1.26384778289763,-3.72621044297521));
#84219=CARTESIAN_POINT('Ctrl Pts',(47.6116171212014,1.15290034873803,-3.76022735826967));
#84220=CARTESIAN_POINT('Ctrl Pts',(47.6057656664612,1.04196977717749,-3.79423910342561));
#84221=CARTESIAN_POINT('Ctrl Pts',(47.599914211721,0.929513096818536,-3.82334390510347));
#84222=CARTESIAN_POINT('Ctrl Pts',(47.5940627569807,0.816002612318447,-3.84741845094727));
#84223=CARTESIAN_POINT('Ctrl Pts',(47.5882107751708,0.702481903362645,-3.87149516530553));
#84224=CARTESIAN_POINT('Ctrl Pts',(47.5823587933608,0.587907605908124,-3.89054063735023));
#84225=CARTESIAN_POINT('Ctrl Pts',(47.5765068115509,0.47276237440816,-3.90448264656714));
#84226=CARTESIAN_POINT('Ctrl Pts',(47.570652886081,0.3575788989112,-3.9184292864418));
#84227=CARTESIAN_POINT('Ctrl Pts',(47.5647989606111,0.241824522396646,-3.92726904332349));
#84228=CARTESIAN_POINT('Ctrl Pts',(47.5589450351412,0.125986466751967,-3.93098160898717));
#84229=CARTESIAN_POINT('Ctrl Pts',(47.5530844575288,0.0100167778548999,
-3.93469839344657));
#84230=CARTESIAN_POINT('Ctrl Pts',(47.5472238799164,-0.10603636662833,-3.9332763443045));
#84231=CARTESIAN_POINT('Ctrl Pts',(47.5413633023041,-0.221686196205895,
-3.92674728374666));
#84232=CARTESIAN_POINT('Ctrl Pts',(47.5354987785597,-0.337413896861429,
-3.92021382694383));
#84233=CARTESIAN_POINT('Ctrl Pts',(47.5296342548153,-0.45273733165556,-3.9085665529287));
#84234=CARTESIAN_POINT('Ctrl Pts',(47.5237697310709,-0.567177036468162,
-3.89188889991778));
#84235=CARTESIAN_POINT('Ctrl Pts',(47.5178965757204,-0.681785177541864,
-3.87518670016827));
#84236=CARTESIAN_POINT('Ctrl Pts',(47.51202342037,-0.795506588259925,-3.85343942207063));
#84237=CARTESIAN_POINT('Ctrl Pts',(47.5061502650195,-0.907874049112982,
-3.82678111615326));
#84238=CARTESIAN_POINT('Ctrl Pts',(47.5045585204607,-0.938327916534902,
-3.81955617302527));
#84239=CARTESIAN_POINT('Ctrl Pts',(47.502966775902,-0.968682433722741,-3.81197078341857));
#84240=CARTESIAN_POINT('Ctrl Pts',(47.5013750313433,-0.998928538987354,
-3.80402822991583));
#84241=CARTESIAN_POINT('Ctrl Pts',(47.4955024488879,-1.1105185212781,-3.77472497262171));
#84242=CARTESIAN_POINT('Ctrl Pts',(47.4896298664325,-1.22100472439362,-3.74045833527711));
#84243=CARTESIAN_POINT('Ctrl Pts',(47.4837572839771,-1.32991222295747,-3.70132712405001));
#84244=CARTESIAN_POINT('Ctrl Pts',(47.4778923057512,-1.43867870049359,-3.66224658264544));
#84245=CARTESIAN_POINT('Ctrl Pts',(47.4720273275254,-1.54587015329953,-3.61831413230468));
#84246=CARTESIAN_POINT('Ctrl Pts',(47.4661623492995,-1.65102396609546,-3.56967909809529));
#84247=CARTESIAN_POINT('Ctrl Pts',(47.4603033971205,-1.75606973726155,-3.52109403457383));
#84248=CARTESIAN_POINT('Ctrl Pts',(47.4544444449415,-1.85908165980543,-3.46781617024461));
#84249=CARTESIAN_POINT('Ctrl Pts',(47.4485854927625,-1.95961499212944,-3.41004370684915));
#84250=CARTESIAN_POINT('Ctrl Pts',(47.4424997560892,-2.06403970301986,-3.35003502467343));
#84251=CARTESIAN_POINT('Ctrl Pts',(47.4364140194159,-2.16578963941227,-3.2851769178553));
#84252=CARTESIAN_POINT('Ctrl Pts',(47.4303282827426,-2.26439189659742,-3.21574537838802));
#84253=CARTESIAN_POINT('Ctrl Pts',(47.4244761045323,-2.35920999536975,-3.14897848323712));
#84254=CARTESIAN_POINT('Ctrl Pts',(47.4186239263219,-2.45111719634862,-3.07798298423056));
#84255=CARTESIAN_POINT('Ctrl Pts',(47.4127717481116,-2.53972132550726,-3.00304921517508));
#84256=CARTESIAN_POINT('Ctrl Pts',(47.4069204576031,-2.62831201453301,-2.92812681263064));
#84257=CARTESIAN_POINT('Ctrl Pts',(47.4010691670946,-2.71360031244272,-2.84926759467338));
#84258=CARTESIAN_POINT('Ctrl Pts',(47.3952178765862,-2.79522712830017,-2.76680217963171));
#84259=CARTESIAN_POINT('Ctrl Pts',(47.3893660570423,-2.87686132432127,-2.68432930860573));
#84260=CARTESIAN_POINT('Ctrl Pts',(47.3835142374983,-2.95483308940464,-2.59824988611721));
#84261=CARTESIAN_POINT('Ctrl Pts',(47.3776624179544,-3.02882071597627,-2.50893086203525));
#84262=CARTESIAN_POINT('Ctrl Pts',(47.3718086525974,-3.10283294448411,-2.41958213810977));
#84263=CARTESIAN_POINT('Ctrl Pts',(47.3659548872403,-3.17285813669213,-2.32699198875545));
#84264=CARTESIAN_POINT('Ctrl Pts',(47.3601011218833,-3.23861578526996,-2.23155927445368));
#84265=CARTESIAN_POINT('Ctrl Pts',(47.3542407003537,-3.30444820525265,-2.13601804595969));
#84266=CARTESIAN_POINT('Ctrl Pts',(47.3483802788241,-3.36600316147584,-2.03762814169207));
#84267=CARTESIAN_POINT('Ctrl Pts',(47.3425198572944,-3.42304424395122,-1.93681622875079));
#84268=CARTESIAN_POINT('Ctrl Pts',(47.3366554874771,-3.48012375618902,-1.83593639672915));
#84269=CARTESIAN_POINT('Ctrl Pts',(47.3307911176597,-3.5326831522767,-1.73263167436644));
#84270=CARTESIAN_POINT('Ctrl Pts',(47.3249267478423,-3.5805333936393,-1.62735048991723));
#84271=CARTESIAN_POINT('Ctrl Pts',(47.3190537420387,-3.62845410020758,-1.52191426632704));
#84272=CARTESIAN_POINT('Ctrl Pts',(47.3131807362351,-3.67165165794374,-1.41449615376108));
#84273=CARTESIAN_POINT('Ctrl Pts',(47.3073077304315,-3.70998622524951,-1.30556164483295));
#84274=CARTESIAN_POINT('Ctrl Pts',(47.3057144244889,-3.72038612879807,-1.27600846435938));
#84275=CARTESIAN_POINT('Ctrl Pts',(47.3041211185462,-3.73042840543479,-1.24634374364339));
#84276=CARTESIAN_POINT('Ctrl Pts',(47.3025278126036,-3.74011091092013,-1.21657690838526));
#84277=CARTESIAN_POINT('Ctrl Pts',(47.295489133608,-3.78288489811189,-1.0850772431386));
#84278=CARTESIAN_POINT('Ctrl Pts',(47.2884504546125,-3.8187501841302,-0.951226593623726));
#84279=CARTESIAN_POINT('Ctrl Pts',(47.2814117756169,-3.8474848584014,-0.815689441130601));
#84280=CARTESIAN_POINT('Ctrl Pts',(47.2744513536712,-3.87590005641323,-0.681659210277727));
#84281=CARTESIAN_POINT('Ctrl Pts',(47.2674909317255,-3.89734228445253,-0.54597981908715));
#84282=CARTESIAN_POINT('Ctrl Pts',(47.2605305097797,-3.91164293126658,-0.40931476674097));
#84283=CARTESIAN_POINT('Ctrl Pts',(47.253674861034,-3.92572831461808,-0.274706893539193));
#84284=CARTESIAN_POINT('Ctrl Pts',(47.2468192122883,-3.93288545623893,-0.139142876403734));
#84285=CARTESIAN_POINT('Ctrl Pts',(47.2399635635426,-3.93299863541307,-0.00327625379142282));
#84286=CARTESIAN_POINT('',(45.9899634930907,-3.93107654104103,0.00207074533378259));
#84287=CARTESIAN_POINT('Ctrl Pts',(47.2399635220349,-3.92992510810637,-0.00327287152616401));
#84288=CARTESIAN_POINT('Ctrl Pts',(47.1945358793113,-3.92290211273228,0.896324194432669));
#84289=CARTESIAN_POINT('Ctrl Pts',(47.082825830341,-3.16907068698517,3.11914721721579));
#84290=CARTESIAN_POINT('Ctrl Pts',(46.9048333751243,0.527994240069298,4.62159797093886));
#84291=CARTESIAN_POINT('Ctrl Pts',(46.7059861563847,4.17322476015174,2.0547975509789));
#84292=CARTESIAN_POINT('Ctrl Pts',(46.5071389376449,3.98501756744227,-2.39950675661282));
#84293=CARTESIAN_POINT('Ctrl Pts',(46.3082917189054,0.136254273817925,-4.64966862412523));
#84294=CARTESIAN_POINT('Ctrl Pts',(46.1358999137019,-3.30896276145751,-2.89761448064259));
#84295=CARTESIAN_POINT('Ctrl Pts',(46.0297905147452,-3.9238187618561,-0.787807482198896));
#84296=CARTESIAN_POINT('Ctrl Pts',(45.9899635220349,-3.92757019263908,0.00206832399879703));
#84297=CARTESIAN_POINT('',(44.7399635220349,-3.93446379439651,0.0024830546121077));
#84298=CARTESIAN_POINT('Ctrl Pts',(45.9899634772174,-3.93299945417141,0.00207207321575638));
#84299=CARTESIAN_POINT('Ctrl Pts',(45.9833496275681,-3.9329302526653,0.133423361231383));
#84300=CARTESIAN_POINT('Ctrl Pts',(45.9767357779188,-3.92627640942975,0.26454482366088));
#84301=CARTESIAN_POINT('Ctrl Pts',(45.9701219282695,-3.91313366715487,0.394808691620507));
#84302=CARTESIAN_POINT('Ctrl Pts',(45.9636237689115,-3.90022081938343,0.522793967592652));
#84303=CARTESIAN_POINT('Ctrl Pts',(45.9571256095534,-3.88104439224054,0.64995119918622));
#84304=CARTESIAN_POINT('Ctrl Pts',(45.9506274501953,-3.85574587958801,0.775701432279254));
#84305=CARTESIAN_POINT('Ctrl Pts',(45.9439557554004,-3.82977176201388,0.904809865814193));
#84306=CARTESIAN_POINT('Ctrl Pts',(45.9372840606055,-3.79734414290077,1.03243481741227));
#84307=CARTESIAN_POINT('Ctrl Pts',(45.9306123658106,-3.75866883754653,1.15797131642222));
#84308=CARTESIAN_POINT('Ctrl Pts',(45.9239406710158,-3.7199935321923,1.28350781543213));
#84309=CARTESIAN_POINT('Ctrl Pts',(45.9172689762209,-3.67507071678868,1.40695563122873));
#84310=CARTESIAN_POINT('Ctrl Pts',(45.910597281426,-3.62415700711541,1.5277352479328));
#84311=CARTESIAN_POINT('Ctrl Pts',(45.9047248338578,-3.57934259342467,1.63404586138289));
#84312=CARTESIAN_POINT('Ctrl Pts',(45.8988523862897,-3.52977142964467,1.73856091847256));
#84313=CARTESIAN_POINT('Ctrl Pts',(45.8929799387215,-3.47560856965179,1.84082429106177));
#84314=CARTESIAN_POINT('Ctrl Pts',(45.8871150983274,-3.42151587227798,1.94295519158326));
#84315=CARTESIAN_POINT('Ctrl Pts',(45.8812502579333,-3.36284349900859,2.04283984623267));
#84316=CARTESIAN_POINT('Ctrl Pts',(45.8753854175392,-3.2998047705344,2.14004146603714));
#84317=CARTESIAN_POINT('Ctrl Pts',(45.8695266059567,-3.23683084324713,2.23714316662551));
#84318=CARTESIAN_POINT('Ctrl Pts',(45.8636677943742,-3.16949971205812,2.33156697355163));
#84319=CARTESIAN_POINT('Ctrl Pts',(45.8578089827917,-3.09807055090966,2.422900712284));
#84320=CARTESIAN_POINT('Ctrl Pts',(45.8517231944539,-3.02387414609812,2.51777281973958));
#84321=CARTESIAN_POINT('Ctrl Pts',(45.8456374061162,-2.94525597783488,2.6093101899429));
#84322=CARTESIAN_POINT('Ctrl Pts',(45.8395516177785,-2.86255624786836,2.69708374504571));
#84323=CARTESIAN_POINT('Ctrl Pts',(45.833699586214,-2.7830330368584,2.78148589419858));
#84324=CARTESIAN_POINT('Ctrl Pts',(45.8278475546495,-2.69973633784404,2.86240770440601));
#84325=CARTESIAN_POINT('Ctrl Pts',(45.8219955230849,-2.61300908549438,2.93950208693987));
#84326=CARTESIAN_POINT('Ctrl Pts',(45.8161443812139,-2.52629501842428,3.0165847486944));
#84327=CARTESIAN_POINT('Ctrl Pts',(45.8102932393429,-2.43615174389131,3.08984086521073));
#84328=CARTESIAN_POINT('Ctrl Pts',(45.8044420974718,-2.3429573898478,3.15896180245307));
#84329=CARTESIAN_POINT('Ctrl Pts',(45.7985904284071,-2.24975463890086,3.2280889675602));
#84330=CARTESIAN_POINT('Ctrl Pts',(45.7927387593424,-2.15350059398267,3.29307996647261));
#84331=CARTESIAN_POINT('Ctrl Pts',(45.7868870902777,-2.05460405395717,3.35366831715105));
#84332=CARTESIAN_POINT('Ctrl Pts',(45.7810334770931,-1.95567465719872,3.41427679730276));
#84333=CARTESIAN_POINT('Ctrl Pts',(45.7751798639086,-1.85410137191503,3.47047950489353));
#84334=CARTESIAN_POINT('Ctrl Pts',(45.769326250724,-1.75031875069544,3.52205526233816));
#84335=CARTESIAN_POINT('Ctrl Pts',(45.7634659831268,-1.64641814894475,3.57368965132615));
#84336=CARTESIAN_POINT('Ctrl Pts',(45.7576057155295,-1.54030356860845,3.62068640744339));
#84337=CARTESIAN_POINT('Ctrl Pts',(45.7517454479322,-1.43243084273132,3.6628719443617));
#84338=CARTESIAN_POINT('Ctrl Pts',(45.7458812332634,-1.32448546123561,3.70508589454439));
#84339=CARTESIAN_POINT('Ctrl Pts',(45.7400170185946,-1.2147799665808,3.74248203998889));
#84340=CARTESIAN_POINT('Ctrl Pts',(45.7341528039258,-1.10378502384003,3.77493677048324));
#84341=CARTESIAN_POINT('Ctrl Pts',(45.7282799538654,-0.992626634696376,
3.80743929242489));
#84342=CARTESIAN_POINT('Ctrl Pts',(45.722407103805,-0.880175407843266,3.83498577895984));
#84343=CARTESIAN_POINT('Ctrl Pts',(45.7165342537446,-0.766911932180097,
3.85750373794761));
#84344=CARTESIAN_POINT('Ctrl Pts',(45.7149395233919,-0.7361560469392,3.86361832836109));
#84345=CARTESIAN_POINT('Ctrl Pts',(45.7133447930392,-0.705340295015743,
3.86936243364421));
#84346=CARTESIAN_POINT('Ctrl Pts',(45.7117500626865,-0.674474337062625,
3.87473526433019));
#84347=CARTESIAN_POINT('Ctrl Pts',(45.70587761653,-0.560813318546454,3.89452021346446));
#84348=CARTESIAN_POINT('Ctrl Pts',(45.7000051703735,-0.446090714275419,
3.90933286902292));
#84349=CARTESIAN_POINT('Ctrl Pts',(45.694132724217,-0.33077946938094,3.91906544250489));
#84350=CARTESIAN_POINT('Ctrl Pts',(45.6882678852455,-0.2156175990323,3.92878540838086));
#84351=CARTESIAN_POINT('Ctrl Pts',(45.6824030462741,-0.099869012550308,
3.93343834451574));
#84352=CARTESIAN_POINT('Ctrl Pts',(45.6765382073026,0.0159835148301993,
3.93296752176441));
#84353=CARTESIAN_POINT('Ctrl Pts',(45.670679397152,0.131716950427295,3.93249718300011));
#84354=CARTESIAN_POINT('Ctrl Pts',(45.6648205870014,0.247553703526219,3.92691356341085));
#84355=CARTESIAN_POINT('Ctrl Pts',(45.6589617768508,0.363006911437183,3.91621181529406));
#84356=CARTESIAN_POINT('Ctrl Pts',(45.6528759879798,0.482932942451069,3.90509546608403));
#84357=CARTESIAN_POINT('Ctrl Pts',(45.6467901991088,0.602444656298446,3.88845636229384));
#84358=CARTESIAN_POINT('Ctrl Pts',(45.6407044102378,0.72099715796601,3.86634867778437));
#84359=CARTESIAN_POINT('Ctrl Pts',(45.6348523801191,0.834995987880806,3.84509016252104));
#84360=CARTESIAN_POINT('Ctrl Pts',(45.6290003500004,0.948107490242205,3.81877550282313));
#84361=CARTESIAN_POINT('Ctrl Pts',(45.6231483198818,1.05985426280836,3.7875055038385));
#84362=CARTESIAN_POINT('Ctrl Pts',(45.6172971794593,1.17158404628275,3.75624025889616));
#84363=CARTESIAN_POINT('Ctrl Pts',(45.6114460390368,1.28194911454815,3.72002128397307));
#84364=CARTESIAN_POINT('Ctrl Pts',(45.6055948986143,1.39048538441558,3.67899978196882));
#84365=CARTESIAN_POINT('Ctrl Pts',(45.5997432309993,1.49903143348947,3.63797458389379));
#84366=CARTESIAN_POINT('Ctrl Pts',(45.5938915633842,1.6057479699206,3.59214614469524));
#84367=CARTESIAN_POINT('Ctrl Pts',(45.5880398957692,1.71018978507401,3.54171425993522));
#84368=CARTESIAN_POINT('Ctrl Pts',(45.5821862840339,1.81466629930169,3.49126562001147));
#84369=CARTESIAN_POINT('Ctrl Pts',(45.5763326722987,1.91686621747538,3.43621067301501));
#84370=CARTESIAN_POINT('Ctrl Pts',(45.5704790605634,2.01636851616535,3.37679537535474));
#84371=CARTESIAN_POINT('Ctrl Pts',(45.5646187944075,2.11598392966051,3.31731253403057));
#84372=CARTESIAN_POINT('Ctrl Pts',(45.5587585282515,2.21289524759174,3.25345966033542));
#84373=CARTESIAN_POINT('Ctrl Pts',(45.5528982620956,2.30670997415815,3.18552634506753));
#84374=CARTESIAN_POINT('Ctrl Pts',(45.5470340488652,2.40058788790678,3.11754727456559));
#84375=CARTESIAN_POINT('Ctrl Pts',(45.5411698356349,2.49136473438587,3.04548254644141));
#84376=CARTESIAN_POINT('Ctrl Pts',(45.5353056224046,2.5786820383223,2.96966125092307));
#84377=CARTESIAN_POINT('Ctrl Pts',(45.5294327737673,2.66612792224426,2.89372830398352));
#84378=CARTESIAN_POINT('Ctrl Pts',(45.5235599251301,2.75010379755439,2.81402803281994));
#84379=CARTESIAN_POINT('Ctrl Pts',(45.5176870764928,2.83028882404551,2.73092551573328));
#84380=CARTESIAN_POINT('Ctrl Pts',(45.5160923323108,2.85206268752807,2.70835942152238));
#84381=CARTESIAN_POINT('Ctrl Pts',(45.5144975881288,2.87355726132222,2.68554263745087));
#84382=CARTESIAN_POINT('Ctrl Pts',(45.5129028439468,2.89476665755451,2.66248286347737));
#84383=CARTESIAN_POINT('Ctrl Pts',(45.5070303982175,2.97286760297757,2.57756813375818));
#84384=CARTESIAN_POINT('Ctrl Pts',(45.5011579524883,3.04735982192094,2.48907181891898));
#84385=CARTESIAN_POINT('Ctrl Pts',(45.4952855067591,3.11789691544379,2.39733348215598));
#84386=CARTESIAN_POINT('Ctrl Pts',(45.4894206682254,3.1883426348642,2.30571398369154));
#84387=CARTESIAN_POINT('Ctrl Pts',(45.4835558296916,3.25484316802578,2.21086113974441));
#84388=CARTESIAN_POINT('Ctrl Pts',(45.4776909911579,3.31708975232654,2.11315039100633));
#84389=CARTESIAN_POINT('Ctrl Pts',(45.4718321814548,3.37927234950895,2.01554008519721));
#84390=CARTESIAN_POINT('Ctrl Pts',(45.4659733717518,3.43720947500505,1.91507806460877));
#84391=CARTESIAN_POINT('Ctrl Pts',(45.4601145620487,3.49063379920915,1.81217126117228));
#84392=CARTESIAN_POINT('Ctrl Pts',(45.4540287730136,3.54612786420274,1.70527768931592));
#84393=CARTESIAN_POINT('Ctrl Pts',(45.4479429839786,3.59675211319836,1.59574643428041));
#84394=CARTESIAN_POINT('Ctrl Pts',(45.4418571949435,3.64225748729813,1.48406515902122));
#84395=CARTESIAN_POINT('Ctrl Pts',(45.4360051652942,3.68601496835745,1.37667363915109));
#84396=CARTESIAN_POINT('Ctrl Pts',(45.430153135645,3.72503938938397,1.26729463805309));
#84397=CARTESIAN_POINT('Ctrl Pts',(45.4243011059957,3.75915741224881,1.15638425704212));
#84398=CARTESIAN_POINT('Ctrl Pts',(45.4184499660499,3.79327024803743,1.04549073810435));
#84399=CARTESIAN_POINT('Ctrl Pts',(45.4125988261041,3.82247804732586,0.933066697155677));
#84400=CARTESIAN_POINT('Ctrl Pts',(45.4067476861584,3.84665706876898,0.819584281992779));
#84401=CARTESIAN_POINT('Ctrl Pts',(45.4008960190269,3.87083826873363,0.706091642103263));
#84402=CARTESIAN_POINT('Ctrl Pts',(45.3950443518954,3.88998970400641,0.591540842741068));
#84403=CARTESIAN_POINT('Ctrl Pts',(45.3891926847639,3.90403871548622,0.476414428816662));
#84404=CARTESIAN_POINT('Ctrl Pts',(45.3833390735185,3.918092394504,0.361249766157874));
#84405=CARTESIAN_POINT('Ctrl Pts',(45.3774854622732,3.92704022890058,0.245509518768089));
#84406=CARTESIAN_POINT('Ctrl Pts',(45.3716318510278,3.9308614676783,0.129680846395937));
#84407=CARTESIAN_POINT('Ctrl Pts',(45.3657715853688,3.93468705045878,0.0137204994277308));
#84408=CARTESIAN_POINT('Ctrl Pts',(45.3599113197098,3.93337439161206,-0.102328059785022));
#84409=CARTESIAN_POINT('Ctrl Pts',(45.3540510540507,3.92695487095885,-0.217978075623614));
#84410=CARTESIAN_POINT('Ctrl Pts',(45.348186841322,3.92053102656046,-0.333705985315314));
#84411=CARTESIAN_POINT('Ctrl Pts',(45.3423226285933,3.90899351240924,-0.449034406834267));
#84412=CARTESIAN_POINT('Ctrl Pts',(45.3364584158646,3.89242533084684,-0.563483845182683));
#84413=CARTESIAN_POINT('Ctrl Pts',(45.3305855677321,3.87583275164646,-0.678101817172088));
#84414=CARTESIAN_POINT('Ctrl Pts',(45.3247127195995,3.85419479718883,-0.791837818170126));
#84415=CARTESIAN_POINT('Ctrl Pts',(45.3188398714669,3.82764509296975,-0.904224553009133));
#84416=CARTESIAN_POINT('Ctrl Pts',(45.3172451227137,3.82043562547685,-0.934742727704025));
#84417=CARTESIAN_POINT('Ctrl Pts',(45.3156503739604,3.81286425855215,-0.965161511444319));
#84418=CARTESIAN_POINT('Ctrl Pts',(45.3140556252071,3.80493428586479,-0.995471787772322));
#84419=CARTESIAN_POINT('Ctrl Pts',(45.3081831788506,3.77573323515354,-1.10708527637067));
#84420=CARTESIAN_POINT('Ctrl Pts',(45.3023107324941,3.74156804667851,-1.21759967111882));
#84421=CARTESIAN_POINT('Ctrl Pts',(45.2964382861375,3.70253706269697,-1.32653997276949));
#84422=CARTESIAN_POINT('Ctrl Pts',(45.2905734469675,3.66355663958204,-1.43533915279066));
#84423=CARTESIAN_POINT('Ctrl Pts',(45.2847086077975,3.61972309385321,-1.54256790918217));
#84424=CARTESIAN_POINT('Ctrl Pts',(45.2788437686276,3.57118529858779,-1.64776350340407));
#84425=CARTESIAN_POINT('Ctrl Pts',(45.2729849582802,3.52269739825527,-1.75285096071767));
#84426=CARTESIAN_POINT('Ctrl Pts',(45.2671261479328,3.46951503916198,-1.85590903992961));
#84427=CARTESIAN_POINT('Ctrl Pts',(45.2612673375854,3.4118359883381,-1.95649282868121));
#84428=CARTESIAN_POINT('Ctrl Pts',(45.2551815487888,3.35192237098437,-2.06097337309331));
#84429=CARTESIAN_POINT('Ctrl Pts',(45.2490957599922,3.28715675230539,-2.16278360700214));
#84430=CARTESIAN_POINT('Ctrl Pts',(45.2430099711957,3.21781469002824,-2.26145033565597));
#84431=CARTESIAN_POINT('Ctrl Pts',(45.2371579408859,3.15113609440967,-2.35632722112586));
#84432=CARTESIAN_POINT('Ctrl Pts',(45.2313059105761,3.08022639715495,-2.44829726485992));
#84433=CARTESIAN_POINT('Ctrl Pts',(45.2254538802664,3.00537554915616,-2.53696803459057));
#84434=CARTESIAN_POINT('Ctrl Pts',(45.2196027396553,2.93053608091667,-2.62562532348507));
#84435=CARTESIAN_POINT('Ctrl Pts',(45.2137515990441,2.85175691986575,-2.71098401993632));
#84436=CARTESIAN_POINT('Ctrl Pts',(45.207900458433,2.76936833282354,-2.79268473644165));
#84437=CARTESIAN_POINT('Ctrl Pts',(45.2020487906319,2.68697232254,-2.87439281421092));
#84438=CARTESIAN_POINT('Ctrl Pts',(45.1961971228309,2.60096653330443,-2.95244196577199));
#84439=CARTESIAN_POINT('Ctrl Pts',(45.1903454550299,2.51171759877025,-3.02651015263915));
#84440=CARTESIAN_POINT('Ctrl Pts',(45.1844918431115,2.42243901279127,-3.10060294740515));
#84441=CARTESIAN_POINT('Ctrl Pts',(45.1786382311931,2.32991545692717,-3.17071188371098));
#84442=CARTESIAN_POINT('Ctrl Pts',(45.1727846192748,2.23454551411417,-3.23655609334247));
#84443=CARTESIAN_POINT('Ctrl Pts',(45.1669243529409,2.13906715427116,-3.30247515500219));
#84444=CARTESIAN_POINT('Ctrl Pts',(45.1610640866071,2.04073628931843,-3.36411957822822));
#84445=CARTESIAN_POINT('Ctrl Pts',(45.1552038202733,1.93997934989935,-3.4212525662342));
#84446=CARTESIAN_POINT('Ctrl Pts',(45.1493396068679,1.83915454754894,-3.47842403508392));
#84447=CARTESIAN_POINT('Ctrl Pts',(45.1434753934625,1.73590078437729,-3.53107783094257));
#84448=CARTESIAN_POINT('Ctrl Pts',(45.1376111800571,1.63066629615307,-3.5790245082411));
#84449=CARTESIAN_POINT('Ctrl Pts',(45.1317383312503,1.52527684391502,-3.62704178986041));
#84450=CARTESIAN_POINT('Ctrl Pts',(45.1258654824435,1.41790122732476,-3.67033796500544));
#84451=CARTESIAN_POINT('Ctrl Pts',(45.1199926336367,1.3090047920021,-3.7087727693289));
#84452=CARTESIAN_POINT('Ctrl Pts',(45.1183978912469,1.27943451576739,-3.71920954604711));
#84453=CARTESIAN_POINT('Ctrl Pts',(45.1168031488572,1.24975216627677,-3.7292881508894));
#84454=CARTESIAN_POINT('Ctrl Pts',(45.1152084064674,1.21996719318159,-3.73900642518312));
#84455=CARTESIAN_POINT('Ctrl Pts',(45.1093359603488,1.11028762940305,-3.77479279577373));
#84456=CARTESIAN_POINT('Ctrl Pts',(45.1034635142301,0.998848473062372,-3.80580899859355));
#84457=CARTESIAN_POINT('Ctrl Pts',(45.0975910681115,0.886102472380609,-3.83188092305084));
#84458=CARTESIAN_POINT('Ctrl Pts',(45.0917262291816,0.77350252329128,-3.85791907383934));
#84459=CARTESIAN_POINT('Ctrl Pts',(45.0858613902516,0.659599495435837,-3.87902559093735));
#84460=CARTESIAN_POINT('Ctrl Pts',(45.0799965513217,0.544863145754668,-3.89507550021798));
#84461=CARTESIAN_POINT('Ctrl Pts',(45.0741377412163,0.430244740542621,-3.91110891082112));
#84462=CARTESIAN_POINT('Ctrl Pts',(45.0682789311109,0.314795124286692,-3.9220959957818));
#84463=CARTESIAN_POINT('Ctrl Pts',(45.0624201210054,0.198995495849135,-3.92796254980006));
#84464=CARTESIAN_POINT('Ctrl Pts',(45.0563343321189,0.0787096222447494,
-3.93405638260983));
#84465=CARTESIAN_POINT('Ctrl Pts',(45.0502485432323,-0.0419534893208762,
-3.93462480424674));
#84466=CARTESIAN_POINT('Ctrl Pts',(45.0441627543457,-0.162446786266555,
-3.92964375505359));
#84467=CARTESIAN_POINT('Ctrl Pts',(45.0383107242811,-0.278311862997924,
-3.92485403096439));
#84468=CARTESIAN_POINT('Ctrl Pts',(45.0324586942165,-0.394019478645874,
-3.91493330776742));
#84469=CARTESIAN_POINT('Ctrl Pts',(45.0266066641519,-0.509082736305069,
-3.89991330257432));
#84470=CARTESIAN_POINT('Ctrl Pts',(45.0207555237866,-0.624128500597504,
-3.88489558091173));
#84471=CARTESIAN_POINT('Ctrl Pts',(45.0149043834213,-0.738529691916645,
-3.86478017220676));
#84472=CARTESIAN_POINT('Ctrl Pts',(45.0090532430561,-0.851805411671151,
-3.83965057533205));
#84473=CARTESIAN_POINT('Ctrl Pts',(45.0032015755014,-0.965091337599584,
-3.81451871427366));
#84474=CARTESIAN_POINT('Ctrl Pts',(44.9973499079468,-1.07725118680878,-3.78437185647899));
#84475=CARTESIAN_POINT('Ctrl Pts',(44.9914982403922,-1.1878158151131,-3.74934428792118));
#84476=CARTESIAN_POINT('Ctrl Pts',(44.9856446287204,-1.29841717663714,-3.7143050820487));
#84477=CARTESIAN_POINT('Ctrl Pts',(44.9797910170486,-1.40742186956713,-3.67438206586608));
#84478=CARTESIAN_POINT('Ctrl Pts',(44.9739374053768,-1.51437810721186,-3.6297586625556));
#84479=CARTESIAN_POINT('Ctrl Pts',(44.9680771392887,-1.62145593326642,-3.58508453112707));
#84480=CARTESIAN_POINT('Ctrl Pts',(44.9622168732006,-1.72648027432731,-3.53569950652833));
#84481=CARTESIAN_POINT('Ctrl Pts',(44.9563566071124,-1.82902135944053,-3.48183426755357));
#84482=CARTESIAN_POINT('Ctrl Pts',(44.9504923939525,-1.93163150916946,-3.42793274866207));
#84483=CARTESIAN_POINT('Ctrl Pts',(44.9446281807926,-2.03175471636381,-3.36954521454028));
#84484=CARTESIAN_POINT('Ctrl Pts',(44.9387639676327,-2.1289892520815,-3.306946289936));
#84485=CARTESIAN_POINT('Ctrl Pts',(44.9328911190691,-2.22636697145233,-3.24425518468169));
#84486=CARTESIAN_POINT('Ctrl Pts',(44.9270182705056,-2.32084719367175,-3.17734054994632));
#84487=CARTESIAN_POINT('Ctrl Pts',(44.921145421942,-2.41206031000855,-3.10651799622688));
#84488=CARTESIAN_POINT('Ctrl Pts',(44.919550677204,-2.43682880790952,-3.08728646085576));
#84489=CARTESIAN_POINT('Ctrl Pts',(44.9179559324659,-2.46135660688793,-3.06776698041003));
#84490=CARTESIAN_POINT('Ctrl Pts',(44.9163611877279,-2.48563678149518,-3.04796633683482));
#84491=CARTESIAN_POINT('Ctrl Pts',(44.9105671096081,-2.57385229654257,-2.9760259986984));
#84492=CARTESIAN_POINT('Ctrl Pts',(44.9047730314883,-2.65910878842539,-2.90011648010944));
#84493=CARTESIAN_POINT('Ctrl Pts',(44.8989789533686,-2.74102038004823,-2.82051347739383));
#84494=CARTESIAN_POINT('Ctrl Pts',(44.8931924170807,-2.82282535186984,-2.7410140895166));
#84495=CARTESIAN_POINT('Ctrl Pts',(44.8874058807929,-2.90129377484753,-2.65783106623817));
#84496=CARTESIAN_POINT('Ctrl Pts',(44.881619344505,-2.97607141756385,-2.5712813765824));
#84497=CARTESIAN_POINT('Ctrl Pts',(44.8757170185688,-3.0523453745741,-2.4829998118225));
#84498=CARTESIAN_POINT('Ctrl Pts',(44.8698146926325,-3.12477889579652,-2.39121565963971));
#84499=CARTESIAN_POINT('Ctrl Pts',(44.8639123666963,-3.19303385795157,-2.29630655226494));
#84500=CARTESIAN_POINT('Ctrl Pts',(44.8581359753042,-3.25983250311532,-2.20342246609502));
#84501=CARTESIAN_POINT('Ctrl Pts',(44.8523595839122,-3.32262885091409,-2.10754580369962));
#84502=CARTESIAN_POINT('Ctrl Pts',(44.8465831925201,-3.38114599827894,-2.00906464264402));
#84503=CARTESIAN_POINT('Ctrl Pts',(44.8408088880004,-3.43964200479542,-1.91061906048086));
#84504=CARTESIAN_POINT('Ctrl Pts',(44.8350345834807,-3.49386166611185,-1.80957121479011));
#84505=CARTESIAN_POINT('Ctrl Pts',(44.8292602789609,-3.54357187614594,-1.70633741053391));
#84506=CARTESIAN_POINT('Ctrl Pts',(44.8234865745486,-3.5932769199365,-1.60311433507914));
#84507=CARTESIAN_POINT('Ctrl Pts',(44.8177128701362,-3.63847326039928,-1.4977061362803));
#84508=CARTESIAN_POINT('Ctrl Pts',(44.8119391657238,-3.67897455680063,-1.39055212430661));
#84509=CARTESIAN_POINT('Ctrl Pts',(44.8059411954164,-3.72104903028886,-1.27923596812068));
#84510=CARTESIAN_POINT('Ctrl Pts',(44.799943225109,-3.75805613309071,-1.16603607841502));
#84511=CARTESIAN_POINT('Ctrl Pts',(44.7939452548016,-3.78984315864233,-1.0514646132381));
#84512=CARTESIAN_POINT('Ctrl Pts',(44.7881654491639,-3.82047399208656,-0.941060465432645));
#84513=CARTESIAN_POINT('Ctrl Pts',(44.7823856435261,-3.84625782289911,-0.829383217623024));
#84514=CARTESIAN_POINT('Ctrl Pts',(44.7766058378884,-3.86711003596097,-0.716902343258804));
#84515=CARTESIAN_POINT('Ctrl Pts',(44.7708228221345,-3.88797383038574,-0.604358996780819));
#84516=CARTESIAN_POINT('Ctrl Pts',(44.7650398063806,-3.90390049724624,-0.491011555797396));
#84517=CARTESIAN_POINT('Ctrl Pts',(44.7592567906267,-3.91485726408778,-0.377334866953882));
#84518=CARTESIAN_POINT('Ctrl Pts',(44.75346655778,-3.92582770476428,-0.26351631178214));
#84519=CARTESIAN_POINT('Ctrl Pts',(44.7476763249333,-3.93181585334791,-0.149368112098914));
#84520=CARTESIAN_POINT('Ctrl Pts',(44.7418860920866,-3.93284099725113,-0.0353651006038775));
#84521=CARTESIAN_POINT('Ctrl Pts',(44.7412452354027,-3.93295445906514,-0.0227473710867152));
#84522=CARTESIAN_POINT('Ctrl Pts',(44.7406043787188,-3.93300717721392,-0.010131414475007));
#84523=CARTESIAN_POINT('Ctrl Pts',(44.7399635220349,-3.93299921675928,0.0024821303117587));
#84524=CARTESIAN_POINT('',(43.4899635220349,-3.93339113294996,-0.0033046727686965));
#84525=CARTESIAN_POINT('Ctrl Pts',(44.7399635220349,-3.93751357002608,0.00248497933675672));
#84526=CARTESIAN_POINT('Ctrl Pts',(44.732480337686,-3.9385999113406,0.149941192123029));
#84527=CARTESIAN_POINT('Ctrl Pts',(44.6587147470908,-3.86405265430505,1.60238341515768));
#84528=CARTESIAN_POINT('Ctrl Pts',(44.5186667502484,-2.0585824653155,4.17135808064711));
#84529=CARTESIAN_POINT('Ctrl Pts',(44.3198195315091,2.39588698568534,3.98719394825372));
#84530=CARTESIAN_POINT('Ctrl Pts',(44.1209723127691,4.64954371604161,0.140475102657688));
#84531=CARTESIAN_POINT('Ctrl Pts',(43.9221250940297,2.63222480384985,-3.83528129358985));
#84532=CARTESIAN_POINT('Ctrl Pts',(43.7232778752899,-1.80300190926075,-4.2880268350132));
#84533=CARTESIAN_POINT('Ctrl Pts',(43.5792240179585,-3.81625323490381,-1.76250455766419));
#84534=CARTESIAN_POINT('Ctrl Pts',(43.5014525668734,-3.9374071917899,-0.230019437054218));
#84535=CARTESIAN_POINT('Ctrl Pts',(43.4899635220349,-3.9353688373681,-0.00330633435426386));
#84536=CARTESIAN_POINT('',(42.2399635491998,-3.93062879302141,-0.000873385175346215));
#84537=CARTESIAN_POINT('Ctrl Pts',(43.4899635220349,-3.932998611914,-0.00330434298873431));
#84538=CARTESIAN_POINT('Ctrl Pts',(43.4841873072457,-3.93309431636171,0.110608002457005));
#84539=CARTESIAN_POINT('Ctrl Pts',(43.4784110924565,-3.92823694115193,0.224695840362946));
#84540=CARTESIAN_POINT('Ctrl Pts',(43.4726348776673,-3.91840740930241,0.33848541286737));
#84541=CARTESIAN_POINT('Ctrl Pts',(43.4668642751708,-3.90858742803428,0.452164425012327));
#84542=CARTESIAN_POINT('Ctrl Pts',(43.4610936726743,-3.89380493005363,0.56554532515269));
#84543=CARTESIAN_POINT('Ctrl Pts',(43.4553230701777,-3.87409289134661,0.678154310771268));
#84544=CARTESIAN_POINT('Ctrl Pts',(43.4495561597942,-3.85439346468033,0.79069124757057));
#84545=CARTESIAN_POINT('Ctrl Pts',(43.4437892494106,-3.82977083967027,0.902456832394481));
#84546=CARTESIAN_POINT('Ctrl Pts',(43.4380223390271,-3.80030974732204,1.01298313135467));
#84547=CARTESIAN_POINT('Ctrl Pts',(43.4322572654583,-3.77085803860671,1.123474226657));
#84548=CARTESIAN_POINT('Ctrl Pts',(43.4264921918896,-3.73657103413654,1.23272640831967));
#84549=CARTESIAN_POINT('Ctrl Pts',(43.4207271183208,-3.69758424204237,1.3402834674053));
#84550=CARTESIAN_POINT('Ctrl Pts',(43.4149623885826,-3.65859977513147,1.44783411175759));
#84551=CARTESIAN_POINT('Ctrl Pts',(43.4091976588445,-3.61491622361328,1.55368943336535));
#84552=CARTESIAN_POINT('Ctrl Pts',(43.4034329291063,-3.5667181905589,1.65741073640068));
#84553=CARTESIAN_POINT('Ctrl Pts',(43.3976670507409,-3.51851055400567,1.76115270599336));
#84554=CARTESIAN_POINT('Ctrl Pts',(43.3919011723755,-3.4657868293721,1.86275942558409));
#84555=CARTESIAN_POINT('Ctrl Pts',(43.38613529401,-3.40877835683801,1.96181525989395));
#84556=CARTESIAN_POINT('Ctrl Pts',(43.3803634192129,-3.3517105963015,2.06097411086577));
#84557=CARTESIAN_POINT('Ctrl Pts',(43.3745915444158,-3.290349407056,2.15757641132062));
#84558=CARTESIAN_POINT('Ctrl Pts',(43.3688196696187,-3.22497035933261,2.2512341462909));
#84559=CARTESIAN_POINT('Ctrl Pts',(43.363044419501,-3.15955307875467,2.34494665114055));
#84560=CARTESIAN_POINT('Ctrl Pts',(43.3572691693832,-3.09011352346045,2.43571082598991));
#84561=CARTESIAN_POINT('Ctrl Pts',(43.3514939192655,-3.01696736764411,2.52317199226897));
#84562=CARTESIAN_POINT('Ctrl Pts',(43.34570992324,-2.94371044094894,2.61076560775393));
#84563=CARTESIAN_POINT('Ctrl Pts',(43.3399259272145,-2.86673599811686,2.69504591777783));
#84564=CARTESIAN_POINT('Ctrl Pts',(43.334141931189,-2.78639634865771,2.7756952981527));
#84565=CARTESIAN_POINT('Ctrl Pts',(43.3312891000629,-2.74677055160925,2.81547386328625));
#84566=CARTESIAN_POINT('Ctrl Pts',(43.3284362689368,-2.70632659616591,2.85436973667235));
#84567=CARTESIAN_POINT('Ctrl Pts',(43.3255834378107,-2.66510952229929,2.89234856719408));
#84568=CARTESIAN_POINT('Ctrl Pts',(43.319710991677,-2.58026571789122,2.97052656883632));
#84569=CARTESIAN_POINT('Ctrl Pts',(43.3138385455433,-2.49183705363632,3.0450990959405));
#84570=CARTESIAN_POINT('Ctrl Pts',(43.3079660994096,-2.4001627782383,3.11571944147085));
#84571=CARTESIAN_POINT('Ctrl Pts',(43.302101260465,-2.30860725804554,3.18624830513682));
#84572=CARTESIAN_POINT('Ctrl Pts',(43.2962364215203,-2.21381481216261,3.25283491850321));
#84573=CARTESIAN_POINT('Ctrl Pts',(43.2903715825757,-2.11616060093259,3.31517017829562));
#84574=CARTESIAN_POINT('Ctrl Pts',(43.2845127724559,-2.01860677440873,3.37744135988128));
#84575=CARTESIAN_POINT('Ctrl Pts',(43.2786539623361,-1.91819738023632,3.43546965943753));
#84576=CARTESIAN_POINT('Ctrl Pts',(43.2727951522163,-1.81533910759,3.48898737808757));
#84577=CARTESIAN_POINT('Ctrl Pts',(43.2667093633352,-1.70849595698518,3.54457845041107));
#84578=CARTESIAN_POINT('Ctrl Pts',(43.2606235744542,-1.59901070407391,3.59530210325724));
#84579=CARTESIAN_POINT('Ctrl Pts',(43.2545377855731,-1.48737078546669,3.64090883524158));
#84580=CARTESIAN_POINT('Ctrl Pts',(43.2486857554951,-1.38001902312814,3.68476378528186));
#84581=CARTESIAN_POINT('Ctrl Pts',(43.242833725417,-1.27067548382995,3.72388748066768));
#84582=CARTESIAN_POINT('Ctrl Pts',(43.236981695339,-1.15979611141858,3.75810616932762));
#84583=CARTESIAN_POINT('Ctrl Pts',(43.2311305549607,-1.04893359629425,3.79231965562897));
#84584=CARTESIAN_POINT('Ctrl Pts',(43.2252794145824,-0.936536107192468,
3.82162949608052));
#84585=CARTESIAN_POINT('Ctrl Pts',(43.2194282742041,-0.823075679452457,
3.84591152080932));
#84586=CARTESIAN_POINT('Ctrl Pts',(43.2135766066368,-0.709605028903685,
3.87019573335374));
#84587=CARTESIAN_POINT('Ctrl Pts',(43.2077249390695,-0.595071653561087,
3.88945114312864));
#84588=CARTESIAN_POINT('Ctrl Pts',(43.2018732715022,-0.479958032240053,
3.90360465304675));
#84589=CARTESIAN_POINT('Ctrl Pts',(43.1960196598182,-0.364806166382434,
3.91776286522704));
#84590=CARTESIAN_POINT('Ctrl Pts',(43.1901660481342,-0.249074081271785,
3.92681575669156));
#84591=CARTESIAN_POINT('Ctrl Pts',(43.1843124364502,-0.13324891767699,3.93074213424614));
#84592=CARTESIAN_POINT('Ctrl Pts',(43.1784521703505,-0.0172920834444121,
3.93467297532679));
#84593=CARTESIAN_POINT('Ctrl Pts',(43.1725919042509,0.0987576271060678,
3.93346565629663));
#84594=CARTESIAN_POINT('Ctrl Pts',(43.1667316381512,0.214413430015104,3.92715111512521));
#84595=CARTESIAN_POINT('Ctrl Pts',(43.1608674249801,0.330147130703012,3.92083232091399));
#84596=CARTESIAN_POINT('Ctrl Pts',(43.155003211809,0.445485985130819,3.90939949575695));
#84597=CARTESIAN_POINT('Ctrl Pts',(43.1491389986379,0.559950423097398,3.89293520671396));
#84598=CARTESIAN_POINT('Ctrl Pts',(43.1432661500639,0.674583416763201,3.87644667302519));
#84599=CARTESIAN_POINT('Ctrl Pts',(43.1373933014898,0.788339019499037,3.85491196489894));
#84600=CARTESIAN_POINT('Ctrl Pts',(43.1315204529157,0.90074981497593,3.82846428360261));
#84601=CARTESIAN_POINT('Ctrl Pts',(43.1299257083008,0.931274441735608,3.82128253920871));
#84602=CARTESIAN_POINT('Ctrl Pts',(43.128330963686,0.961700006603048,3.81373880719636));
#84603=CARTESIAN_POINT('Ctrl Pts',(43.1267362190711,0.992017390206271,3.80583637293149));
#84604=CARTESIAN_POINT('Ctrl Pts',(43.1208637729372,1.10365733585567,3.77673665432205));
#84605=CARTESIAN_POINT('Ctrl Pts',(43.1149913268034,1.21420269460918,3.74267180265341));
#84606=CARTESIAN_POINT('Ctrl Pts',(43.1091188806696,1.32317837816996,3.70373972891502));
#84607=CARTESIAN_POINT('Ctrl Pts',(43.1032540417248,1.43201289421539,3.66485808793317));
#84608=CARTESIAN_POINT('Ctrl Pts',(43.0973892027801,1.53928139303118,3.62112190110369));
#84609=CARTESIAN_POINT('Ctrl Pts',(43.0915243638353,1.64452100114867,3.572679621346));
#84610=CARTESIAN_POINT('Ctrl Pts',(43.0856655537154,1.74965242706913,3.52428713835538));
#84611=CARTESIAN_POINT('Ctrl Pts',(43.0798067435955,1.85275873747101,3.47119835664669));
#84612=CARTESIAN_POINT('Ctrl Pts',(43.0739479334756,1.95339484067194,3.41361063925519));
#84613=CARTESIAN_POINT('Ctrl Pts',(43.0678621445946,2.05792973177641,3.35379189056561));
#84614=CARTESIAN_POINT('Ctrl Pts',(43.0617763557135,2.15979871799785,3.289118718314));
#84615=CARTESIAN_POINT('Ctrl Pts',(43.0556905668325,2.25852835458129,3.21986625056886));
#84616=CARTESIAN_POINT('Ctrl Pts',(43.0498385367544,2.3534657265786,3.15327381166631));
#84617=CARTESIAN_POINT('Ctrl Pts',(43.0439865066762,2.44550009918171,3.08244763439425));
#84618=CARTESIAN_POINT('Ctrl Pts',(43.038134476598,2.53423877709297,3.00767731325658));
#84619=CARTESIAN_POINT('Ctrl Pts',(43.0322833362196,2.62296396382608,2.93291835965049));
#84620=CARTESIAN_POINT('Ctrl Pts',(43.0264321958412,2.70839413610495,2.85421672073105));
#84621=CARTESIAN_POINT('Ctrl Pts',(43.0205810554628,2.7901696067844,2.77190233691171));
#84622=CARTESIAN_POINT('Ctrl Pts',(43.0147293878954,2.87195244545116,2.68958053654886));
#84623=CARTESIAN_POINT('Ctrl Pts',(43.008877720328,2.95007963657812,2.60364563746764));
#84624=CARTESIAN_POINT('Ctrl Pts',(43.0030260527606,3.02422880900815,2.51446398080489));
#84625=CARTESIAN_POINT('Ctrl Pts',(42.9971724410765,3.0984026162358,2.42525269505807));
#84626=CARTESIAN_POINT('Ctrl Pts',(42.9913188293923,3.16859551265873,2.33279282451787));
#84627=CARTESIAN_POINT('Ctrl Pts',(42.9854652177082,3.23452626837141,2.23748269696445));
#84628=CARTESIAN_POINT('Ctrl Pts',(42.9796049516084,3.30053197450387,2.14206422037132));
#84629=CARTESIAN_POINT('Ctrl Pts',(42.9737446855086,3.36226563372475,2.04378935960896));
#84630=CARTESIAN_POINT('Ctrl Pts',(42.9678844194089,3.4194900622587,1.94308433016017));
#84631=CARTESIAN_POINT('Ctrl Pts',(42.9620202062376,3.47675303322451,1.84231147274288));
#84632=CARTESIAN_POINT('Ctrl Pts',(42.9561559930664,3.52950053835556,1.73910555462318));
#84633=CARTESIAN_POINT('Ctrl Pts',(42.9502917798952,3.57754272528043,1.63391463938392));
#84634=CARTESIAN_POINT('Ctrl Pts',(42.944418931321,3.62565565718538,1.52856882426019));
#84635=CARTESIAN_POINT('Ctrl Pts',(42.9385460827468,3.66904928791142,1.42123256002071));
#84636=CARTESIAN_POINT('Ctrl Pts',(42.9326732341727,3.70758293075699,1.31237106473719));
#84637=CARTESIAN_POINT('Ctrl Pts',(42.9310784895589,3.71804656158268,1.2828102338979));
#84638=CARTESIAN_POINT('Ctrl Pts',(42.9294837449452,3.72815212141798,1.25313700439382));
#84639=CARTESIAN_POINT('Ctrl Pts',(42.9278890003315,3.73789744300419,1.22336082395291));
#84640=CARTESIAN_POINT('Ctrl Pts',(42.9220165541974,3.77378336202907,1.11371379068472));
#84641=CARTESIAN_POINT('Ctrl Pts',(42.9161441080634,3.80490071252197,1.00230283538655));
#84642=CARTESIAN_POINT('Ctrl Pts',(42.9102716619294,3.83107497297339,0.889580548043272));
#84643=CARTESIAN_POINT('Ctrl Pts',(42.9044068229844,3.85721532718824,0.777004281579848));
#84644=CARTESIAN_POINT('Ctrl Pts',(42.8985419840394,3.87842523261075,0.663120460123252));
#84645=CARTESIAN_POINT('Ctrl Pts',(42.8926771450945,3.8945792887361,0.548398726975031));
#84646=CARTESIAN_POINT('Ctrl Pts',(42.8868183349743,3.91071673912421,0.433794923276933));
#84647=CARTESIAN_POINT('Ctrl Pts',(42.8809595248542,3.92180862047035,0.318355328002071));
#84648=CARTESIAN_POINT('Ctrl Pts',(42.875100714734,3.9277802906891,0.202561072455336));
#84649=CARTESIAN_POINT('Ctrl Pts',(42.8690149258531,3.93398331203176,0.0822807803089556));
#84650=CARTESIAN_POINT('Ctrl Pts',(42.8629291369722,3.93466126693419,-0.0383817654108247));
#84651=CARTESIAN_POINT('Ctrl Pts',(42.8568433480912,3.92978959915348,-0.15887953419208));
#84652=CARTESIAN_POINT('Ctrl Pts',(42.8509913180129,3.92510505505535,-0.274748911372842));
#84653=CARTESIAN_POINT('Ctrl Pts',(42.8451392879345,3.91528937100348,-0.390465485271834));
#84654=CARTESIAN_POINT('Ctrl Pts',(42.8392872578561,3.90037382210772,-0.505542330390647));
#84655=CARTESIAN_POINT('Ctrl Pts',(42.8334361174774,3.88546054086267,-0.620601680069629));
#84656=CARTESIAN_POINT('Ctrl Pts',(42.8275849770988,3.86544898953233,-0.735021084536224));
#84657=CARTESIAN_POINT('Ctrl Pts',(42.8217338367201,3.84042223041134,-0.848319569597698));
#84658=CARTESIAN_POINT('Ctrl Pts',(42.8158821691525,3.81539321637405,-0.961628262876645));
#84659=CARTESIAN_POINT('Ctrl Pts',(42.8100305015849,3.78534818543122,-1.07381543233026));
#84660=CARTESIAN_POINT('Ctrl Pts',(42.8041788340173,3.75042099762731,-1.18441181206375));
#84661=CARTESIAN_POINT('Ctrl Pts',(42.7983252223329,3.71548220586098,-1.29504493555809));
#84662=CARTESIAN_POINT('Ctrl Pts',(42.7924716106485,3.67565815637435,-1.4040858244576));
#84663=CARTESIAN_POINT('Ctrl Pts',(42.7866179989641,3.63113186215738,-1.5110825257495));
#84664=CARTESIAN_POINT('Ctrl Pts',(42.7807577328641,3.58655495022188,-1.61820086143755));
#84665=CARTESIAN_POINT('Ctrl Pts',(42.7748974667641,3.53726528295333,-1.72326998934912));
#84666=CARTESIAN_POINT('Ctrl Pts',(42.7690372006641,3.4834931489193,-1.82585992930244));
#84667=CARTESIAN_POINT('Ctrl Pts',(42.7631729874927,3.42968479768131,-1.92851896676967));
#84668=CARTESIAN_POINT('Ctrl Pts',(42.7573087743213,3.37138817547999,-2.02869513495938));
#84669=CARTESIAN_POINT('Ctrl Pts',(42.7514445611499,3.30887754227419,-2.12598645579729));
#84670=CARTESIAN_POINT('Ctrl Pts',(42.7455717125754,3.24627485843956,-2.22342104389715));
#84671=CARTESIAN_POINT('Ctrl Pts',(42.739698864001,3.17944601659607,-2.31796196999404));
#84672=CARTESIAN_POINT('Ctrl Pts',(42.7338260154266,3.10870629159263,-2.40923933900565));
#84673=CARTESIAN_POINT('Ctrl Pts',(42.732231270815,3.08949724953285,-2.43402528241107));
#84674=CARTESIAN_POINT('Ctrl Pts',(42.7306365262034,3.07000004406421,-2.45857078841704));
#84675=CARTESIAN_POINT('Ctrl Pts',(42.7290417815917,3.0502214508407,-2.48286892542301));
#84676=CARTESIAN_POINT('Ctrl Pts',(42.7231693354579,2.97738927290907,-2.57234375398275));
#84677=CARTESIAN_POINT('Ctrl Pts',(42.717296889324,2.90049485421054,-2.65876099088872));
#84678=CARTESIAN_POINT('Ctrl Pts',(42.7114244431901,2.81982455190766,-2.74172910705247));
#84679=CARTESIAN_POINT('Ctrl Pts',(42.7055596042453,2.73925875022137,-2.82458974600282));
#84680=CARTESIAN_POINT('Ctrl Pts',(42.6996947653005,2.65492707747333,-2.90400985585174));
#84681=CARTESIAN_POINT('Ctrl Pts',(42.6938299263556,2.56715679645829,-2.97963000763484));
#84682=CARTESIAN_POINT('Ctrl Pts',(42.6879711162357,2.47947673985589,-3.05517242486246));
#84683=CARTESIAN_POINT('Ctrl Pts',(42.6821123061157,2.38836541708526,-3.12692238549876));
#84684=CARTESIAN_POINT('Ctrl Pts',(42.6762534959957,2.29418720034906,-3.19455694733316));
#84685=CARTESIAN_POINT('Ctrl Pts',(42.6701677071147,2.1963603835543,-3.26481176972059));
#84686=CARTESIAN_POINT('Ctrl Pts',(42.6640819182337,2.09522455164948,-3.3306255453884));
#84687=CARTESIAN_POINT('Ctrl Pts',(42.6579961293527,1.99122659376556,-3.39168183240716));
#84688=CARTESIAN_POINT('Ctrl Pts',(42.6521440992745,1.89122325984881,-3.45039291080419));
#84689=CARTESIAN_POINT('Ctrl Pts',(42.6462920691963,1.78857400550308,-3.50470500623368));
#84690=CARTESIAN_POINT('Ctrl Pts',(42.640440039118,1.68370534757026,-3.5543811419941));
#84691=CARTESIAN_POINT('Ctrl Pts',(42.6345888987396,1.57885263309941,-3.60404972535902));
#84692=CARTESIAN_POINT('Ctrl Pts',(42.6287377583611,1.47178155940849,-3.64908357355293));
#84693=CARTESIAN_POINT('Ctrl Pts',(42.6228866179826,1.36294163890904,-3.68929249164768));
#84694=CARTESIAN_POINT('Ctrl Pts',(42.6170349504151,1.25409191190956,-3.72950503257452));
#84695=CARTESIAN_POINT('Ctrl Pts',(42.6111832828477,1.14347340904853,-3.76489163595134));
#84696=CARTESIAN_POINT('Ctrl Pts',(42.6053316152802,1.03155326047639,-3.79531116916657));
#84697=CARTESIAN_POINT('Ctrl Pts',(42.599478003596,0.919595928344136,-3.82574080875278));
#84698=CARTESIAN_POINT('Ctrl Pts',(42.5936243919118,0.806336489275951,-3.85119998844847));
#84699=CARTESIAN_POINT('Ctrl Pts',(42.5877707802276,0.692254087172466,-3.87159828479054));
#84700=CARTESIAN_POINT('Ctrl Pts',(42.5819105141277,0.578041995611775,-3.89201977002003));
#84701=CARTESIAN_POINT('Ctrl Pts',(42.5760502480279,0.463005480836088,-3.90736881582649));
#84702=CARTESIAN_POINT('Ctrl Pts',(42.570189981928,0.347630765393659,-3.91760664831882));
#84703=CARTESIAN_POINT('Ctrl Pts',(42.5643257687568,0.232178341493546,-3.92785137630961));
#84704=CARTESIAN_POINT('Ctrl Pts',(42.5584615555855,0.11638767529605,-3.93297801791629));
#84705=CARTESIAN_POINT('Ctrl Pts',(42.5525973424143,0.000745209508502876,
-3.9329999294003));
#84706=CARTESIAN_POINT('Ctrl Pts',(42.54672449384,-0.115067546694507,-3.93302187315028));
#84707=CARTESIAN_POINT('Ctrl Pts',(42.5408516452657,-0.230731255534072,
-3.9279241024371));
#84708=CARTESIAN_POINT('Ctrl Pts',(42.5349787966914,-0.345764285630725,
-3.91777182321562));
#84709=CARTESIAN_POINT('Ctrl Pts',(42.5333840520783,-0.377000967924689,
-3.91501501918869));
#84710=CARTESIAN_POINT('Ctrl Pts',(42.5317893074653,-0.408191205040602,
-3.91188580256903));
#84711=CARTESIAN_POINT('Ctrl Pts',(42.5301945628522,-0.439325502388764,
-3.90838612510981));
#84712=CARTESIAN_POINT('Ctrl Pts',(42.5243221167183,-0.553973630115394,
-3.89549900375098));
#84713=CARTESIAN_POINT('Ctrl Pts',(42.5184496705844,-0.668246179663863,
-3.87754141813316));
#84714=CARTESIAN_POINT('Ctrl Pts',(42.5125772244505,-0.781658957024931,
-3.85454255066703));
#84715=CARTESIAN_POINT('Ctrl Pts',(42.5067123855056,-0.894924819042929,
-3.83157347602127));
#84716=CARTESIAN_POINT('Ctrl Pts',(42.5008475465607,-1.00733272235404,-3.80357618775543));
#84717=CARTESIAN_POINT('Ctrl Pts',(42.4949827076159,-1.11840335776539,-3.77063163532837));
#84718=CARTESIAN_POINT('Ctrl Pts',(42.4891238974959,-1.22935981691158,-3.73772094861154));
#84719=CARTESIAN_POINT('Ctrl Pts',(42.4832650873759,-1.33898134851726,-3.69987323009655));
#84720=CARTESIAN_POINT('Ctrl Pts',(42.4774062772559,-1.44679927093527,-3.65722037476841));
#84721=CARTESIAN_POINT('Ctrl Pts',(42.4713204883749,-1.55879421529793,-3.61291508625743));
#84722=CARTESIAN_POINT('Ctrl Pts',(42.465234699494,-1.66884252992364,-3.5634249053048));
#84723=CARTESIAN_POINT('Ctrl Pts',(42.459148910613,-1.77643638351166,-3.50895465563977));
#84724=CARTESIAN_POINT('Ctrl Pts',(42.4532968805348,-1.87989749262114,-3.45657664094951));
#84725=CARTESIAN_POINT('Ctrl Pts',(42.4474448504565,-1.98108881431325,-3.39959427927564));
#84726=CARTESIAN_POINT('Ctrl Pts',(42.4415928203783,-2.07958037965062,-3.33823822465866));
#84727=CARTESIAN_POINT('Ctrl Pts',(42.4357416799998,-2.17805697105231,-3.27689149816649));
#84728=CARTESIAN_POINT('Ctrl Pts',(42.4298905396213,-2.273834271458,-3.21117261936068));
#84729=CARTESIAN_POINT('Ctrl Pts',(42.4240393992428,-2.36650923123514,-3.14135688174376));
#84730=CARTESIAN_POINT('Ctrl Pts',(42.4181877316753,-2.45919254104573,-3.07153485371413));
#84731=CARTESIAN_POINT('Ctrl Pts',(42.4123360641078,-2.54877262438937,-2.99761548181562));
#84732=CARTESIAN_POINT('Ctrl Pts',(42.4064843965404,-2.63487817719977,-2.91991540824669));
#84733=CARTESIAN_POINT('Ctrl Pts',(42.4006307848562,-2.72101233711132,-2.8421895201537));
#84734=CARTESIAN_POINT('Ctrl Pts',(42.394777173172,-2.80366936440841,-2.76068070954268));
#84735=CARTESIAN_POINT('Ctrl Pts',(42.3889235614878,-2.8825141160547,-2.67574314364167));
#84736=CARTESIAN_POINT('Ctrl Pts',(42.3830632953879,-2.96144849881741,-2.59070902028187));
#84737=CARTESIAN_POINT('Ctrl Pts',(42.377203029288,-3.0365616743948,-2.50223866483081));
#84738=CARTESIAN_POINT('Ctrl Pts',(42.3713427631882,-3.1075581203337,-2.41072012659041));
#84739=CARTESIAN_POINT('Ctrl Pts',(42.3654785500169,-3.1786023845863,-2.31913994776909));
#84740=CARTESIAN_POINT('Ctrl Pts',(42.3596143368456,-3.24552416002274,-2.22450783479905));
#84741=CARTESIAN_POINT('Ctrl Pts',(42.3537501236743,-3.30807165749659,-2.12724020948922));
#84742=CARTESIAN_POINT('Ctrl Pts',(42.3478772751,-3.37071125988378,-2.02982935181101));
#84743=CARTESIAN_POINT('Ctrl Pts',(42.3420044265258,-3.42896352139119,-1.92977559207154));
#84744=CARTESIAN_POINT('Ctrl Pts',(42.3361315779515,-3.48262287083093,-1.82751934040801));
#84745=CARTESIAN_POINT('Ctrl Pts',(42.3345368333385,-3.49719381666281,-1.79975213265173));
#84746=CARTESIAN_POINT('Ctrl Pts',(42.3329420887256,-3.51142637231868,-1.77182262769116));
#84747=CARTESIAN_POINT('Ctrl Pts',(42.3313473441126,-3.52531704580881,-1.74373986779274));
#84748=CARTESIAN_POINT('Ctrl Pts',(42.3250482766907,-3.5801836922543,-1.63281602672377));
#84749=CARTESIAN_POINT('Ctrl Pts',(42.3187492092687,-3.62987581658613,-1.5191699993202));
#84750=CARTESIAN_POINT('Ctrl Pts',(42.3124501418468,-3.67413461259416,-1.40329036501273));
#84751=CARTESIAN_POINT('Ctrl Pts',(42.3061711023168,-3.71825268771015,-1.28777917013381));
#84752=CARTESIAN_POINT('Ctrl Pts',(42.2998920627869,-3.7569717656237,-1.17004882670027));
#84753=CARTESIAN_POINT('Ctrl Pts',(42.2936130232569,-3.7900804902256,-1.05060881283725));
#84754=CARTESIAN_POINT('Ctrl Pts',(42.2873460973,-3.82312534121277,-0.931399223598544));
#84755=CARTESIAN_POINT('Ctrl Pts',(42.281079171343,-3.85058131694735,-0.810486841434601));
#84756=CARTESIAN_POINT('Ctrl Pts',(42.274812245386,-3.87228552257363,-0.688399470995369));
#84757=CARTESIAN_POINT('Ctrl Pts',(42.2685636294963,-3.89392631505821,-0.566668803024465));
#84758=CARTESIAN_POINT('Ctrl Pts',(42.2623150136065,-3.90984878548117,-0.443770304983643));
#84759=CARTESIAN_POINT('Ctrl Pts',(42.2560663977168,-3.91994041182175,-0.320243919172191));
#84760=CARTESIAN_POINT('Ctrl Pts',(42.2506987869713,-3.9286091991085,-0.214133771336548));
#84761=CARTESIAN_POINT('Ctrl Pts',(42.2453311762258,-3.932976188352,-0.107560690645611));
#84762=CARTESIAN_POINT('Ctrl Pts',(42.2399635654804,-3.93299990283659,-0.000874235302823624));
#84763=CARTESIAN_POINT('',(40.9899634959417,-3.93299833106861,0.00362323219413291));
#84764=CARTESIAN_POINT('Ctrl Pts',(42.2399635220349,-3.92667249913085,-0.00087196670281342));
#84765=CARTESIAN_POINT('Ctrl Pts',(42.2041423898142,-3.92526855652312,0.709962603038024));
#84766=CARTESIAN_POINT('Ctrl Pts',(42.1020388513469,-3.40040452164114,2.73803753544301));
#84767=CARTESIAN_POINT('Ctrl Pts',(41.9336529066332,-0.144695732084588,
4.64941428208763));
#84768=CARTESIAN_POINT('Ctrl Pts',(41.7348056878936,3.83289027569088,2.63570524829183));
#84769=CARTESIAN_POINT('Ctrl Pts',(41.5359584691537,4.28966176770655,-1.79910865154202));
#84770=CARTESIAN_POINT('Ctrl Pts',(41.3371112504143,0.806037805343487,-4.58129818694668));
#84771=CARTESIAN_POINT('Ctrl Pts',(41.155112934708,-3.06008131386444,-3.27603838467406));
#84772=CARTESIAN_POINT('Ctrl Pts',(41.0393970252482,-3.92331410043244,-0.973892289700984));
#84773=CARTESIAN_POINT('Ctrl Pts',(40.9899635220349,-3.93215931941742,0.00362194329329435));
#84774=CARTESIAN_POINT('',(39.7399635219896,-3.93299992292088,-0.000778655457619776));
#84775=CARTESIAN_POINT('Ctrl Pts',(40.9899634959417,-3.93299833106861,0.00362323219413291));
#84776=CARTESIAN_POINT('Ctrl Pts',(40.9824898564729,-3.93286215684296,0.151439594361313));
#84777=CARTESIAN_POINT('Ctrl Pts',(40.975016217004,-3.92438925053041,0.298883036488164));
#84778=CARTESIAN_POINT('Ctrl Pts',(40.9675425775351,-3.90772648188647,0.445154740245648));
#84779=CARTESIAN_POINT('Ctrl Pts',(40.9599054571219,-3.89069922614583,0.5946260412473));
#84780=CARTESIAN_POINT('Ctrl Pts',(40.9522683367088,-3.86511989035994,0.742874037455968));
#84781=CARTESIAN_POINT('Ctrl Pts',(40.9446312162956,-3.83119322941646,0.889071110133193));
#84782=CARTESIAN_POINT('Ctrl Pts',(40.9428930818421,-3.82347185079602,0.92234414437671));
#84783=CARTESIAN_POINT('Ctrl Pts',(40.9411549473885,-3.81531829668762,0.955511036363426));
#84784=CARTESIAN_POINT('Ctrl Pts',(40.939416812935,-3.80673532218173,0.98856218158188));
#84785=CARTESIAN_POINT('Ctrl Pts',(40.9335443668011,-3.77773695824565,1.10022849690089));
#84786=CARTESIAN_POINT('Ctrl Pts',(40.9276719206673,-3.74377246966985,1.21080473294224));
#84787=CARTESIAN_POINT('Ctrl Pts',(40.9217994745335,-3.70493933613558,1.31981571272478));
#84788=CARTESIAN_POINT('Ctrl Pts',(40.9159346355887,-3.66615650719029,1.42868547926923));
#84789=CARTESIAN_POINT('Ctrl Pts',(40.9100697966439,-3.62251771282398,1.53599363600944));
#84790=CARTESIAN_POINT('Ctrl Pts',(40.9042049576991,-3.57417098571519,1.6412771749073));
#84791=CARTESIAN_POINT('Ctrl Pts',(40.8983461475792,-3.52587395714903,1.74645248644917));
#84792=CARTESIAN_POINT('Ctrl Pts',(40.8924873374592,-3.47287879347344,1.84960694643604));
#84793=CARTESIAN_POINT('Ctrl Pts',(40.8866285273392,-3.41538245360437,1.95029528420991));
#84794=CARTESIAN_POINT('Ctrl Pts',(40.8805427384583,-3.3556586225349,2.05488443352908));
#84795=CARTESIAN_POINT('Ctrl Pts',(40.8744569495773,-3.29107794989201,2.15681208573282));
#84796=CARTESIAN_POINT('Ctrl Pts',(40.8683711606963,-3.22191513385494,2.25560454650999));
#84797=CARTESIAN_POINT('Ctrl Pts',(40.8625191306181,-3.15540890308403,2.35060232958681));
#84798=CARTESIAN_POINT('Ctrl Pts',(40.8566671005399,-3.08466630045064,2.44270095769923));
#84799=CARTESIAN_POINT('Ctrl Pts',(40.8508150704616,-3.00997656386486,2.53150747282805));
#84800=CARTESIAN_POINT('Ctrl Pts',(40.8449639300832,-2.93529818255913,2.6203004864653));
#84801=CARTESIAN_POINT('Ctrl Pts',(40.8391127897047,-2.85667412647018,2.70580206603224));
#84802=CARTESIAN_POINT('Ctrl Pts',(40.8332616493263,-2.77443400936456,2.787652225024));
#84803=CARTESIAN_POINT('Ctrl Pts',(40.8274099817588,-2.69218648240703,2.86950975873237));
#84804=CARTESIAN_POINT('Ctrl Pts',(40.8215583141914,-2.60632253975584,2.94771492624675));
#84805=CARTESIAN_POINT('Ctrl Pts',(40.815706646624,-2.5172082297601,3.02194502399167));
#84806=CARTESIAN_POINT('Ctrl Pts',(40.8098530349398,-2.42806431305464,3.09619978342063));
#84807=CARTESIAN_POINT('Ctrl Pts',(40.8039994232556,-2.33566819916816,3.16647658263216));
#84808=CARTESIAN_POINT('Ctrl Pts',(40.7981458115714,-2.2404179604264,3.23249383024915));
#84809=CARTESIAN_POINT('Ctrl Pts',(40.7922855454716,-2.14505944072703,3.29858612661021));
#84810=CARTESIAN_POINT('Ctrl Pts',(40.7864252793717,-2.04684066002644,3.36040897074151));
#84811=CARTESIAN_POINT('Ctrl Pts',(40.7805650132719,-1.94618761832499,3.41772479206247));
#84812=CARTESIAN_POINT('Ctrl Pts',(40.7747008001006,-1.84546678367061,3.47507921737108));
#84813=CARTESIAN_POINT('Ctrl Pts',(40.7688365869294,-1.74230879034057,3.52792038734939));
#84814=CARTESIAN_POINT('Ctrl Pts',(40.7629723737581,-1.63716152939203,3.57605804296837));
#84815=CARTESIAN_POINT('Ctrl Pts',(40.7570995251839,-1.53185943284241,3.62426658415084));
#84816=CARTESIAN_POINT('Ctrl Pts',(40.7512266766097,-1.42456260398709,3.66775763295613));
#84817=CARTESIAN_POINT('Ctrl Pts',(40.7453538280354,-1.31573613299586,3.70639008043259));
#84818=CARTESIAN_POINT('Ctrl Pts',(40.7437590834221,-1.28618481284678,3.71688054119201));
#84819=CARTESIAN_POINT('Ctrl Pts',(40.7421643388087,-1.25652076903543,3.72701303314016));
#84820=CARTESIAN_POINT('Ctrl Pts',(40.7405695941953,-1.22675344731855,3.73678538044294));
#84821=CARTESIAN_POINT('Ctrl Pts',(40.7346971480614,-1.11713903516171,3.77277081827219));
#84822=CARTESIAN_POINT('Ctrl Pts',(40.7288247019275,-1.0057563729685,3.80398929075869));
#84823=CARTESIAN_POINT('Ctrl Pts',(40.7229522557935,-0.893057892113009,
3.83026586562012));
#84824=CARTESIAN_POINT('Ctrl Pts',(40.7170874168487,-0.780505401298543,
3.85650840170647));
#84825=CARTESIAN_POINT('Ctrl Pts',(40.7112225779038,-0.666640880347451,
3.877821677983));
#84826=CARTESIAN_POINT('Ctrl Pts',(40.705357738959,-0.551933858533738,3.89407986767144));
#84827=CARTESIAN_POINT('Ctrl Pts',(40.6994989288389,-0.437344751047511,
3.91032134457742));
#84828=CARTESIAN_POINT('Ctrl Pts',(40.6936401187189,-0.321915272144686,
3.92151801322171));
#84829=CARTESIAN_POINT('Ctrl Pts',(40.6877813085989,-0.206126485174543,
3.92759479479612));
#84830=CARTESIAN_POINT('Ctrl Pts',(40.6816955197179,-0.085851873462126,
3.93390699966024));
#84831=CARTESIAN_POINT('Ctrl Pts',(40.6756097308369,0.0348100071207318,
3.93469448735638));
#84832=CARTESIAN_POINT('Ctrl Pts',(40.669523941956,0.155312148578736,3.92993220507732));
#84833=CARTESIAN_POINT('Ctrl Pts',(40.6636719118777,0.271185730476043,3.92535284491819));
#84834=CARTESIAN_POINT('Ctrl Pts',(40.6578198817994,0.386911167016915,3.91564220821036));
#84835=CARTESIAN_POINT('Ctrl Pts',(40.6519678517212,0.502001504513165,3.90083112803753));
#84836=CARTESIAN_POINT('Ctrl Pts',(40.6461167113426,0.617074344518227,3.88602229963274));
#84837=CARTESIAN_POINT('Ctrl Pts',(40.6402655709641,0.731511867598882,3.86611462232444));
#84838=CARTESIAN_POINT('Ctrl Pts',(40.6344144305856,0.844833024359663,3.84119072176211));
#84839=CARTESIAN_POINT('Ctrl Pts',(40.6285627630181,0.958164391380532,3.81626457555109));
#84840=CARTESIAN_POINT('Ctrl Pts',(40.6227110954506,1.07037878839605,3.78632139642283));
#84841=CARTESIAN_POINT('Ctrl Pts',(40.6168594278831,1.18100682819149,3.75149461838413));
#84842=CARTESIAN_POINT('Ctrl Pts',(40.6110058161989,1.29167162226623,3.71665626974244));
#84843=CARTESIAN_POINT('Ctrl Pts',(40.6051522045146,1.40074861706163,3.67693122002077));
#84844=CARTESIAN_POINT('Ctrl Pts',(40.5992985928304,1.50778569361863,3.63250207186713));
#84845=CARTESIAN_POINT('Ctrl Pts',(40.5934383267305,1.61494445047091,3.58802241643096));
#84846=CARTESIAN_POINT('Ctrl Pts',(40.5875780606306,1.72005827845911,3.53882814740728));
#84847=CARTESIAN_POINT('Ctrl Pts',(40.5817177945307,1.82269698853103,3.4851491629484));
#84848=CARTESIAN_POINT('Ctrl Pts',(40.5758535813594,1.92540482896517,3.43143402402463));
#84849=CARTESIAN_POINT('Ctrl Pts',(40.5699893681881,2.02563387543411,3.37322836212841));
#84850=CARTESIAN_POINT('Ctrl Pts',(40.5641251550168,2.12298190106599,3.31080607220451));
#84851=CARTESIAN_POINT('Ctrl Pts',(40.5582523064425,2.22047327746065,3.24829186174274));
#84852=CARTESIAN_POINT('Ctrl Pts',(40.5523794578682,2.31507482939733,3.18154886825232));
#84853=CARTESIAN_POINT('Ctrl Pts',(40.5465066092939,2.4064163757511,3.11089203067495));
#84854=CARTESIAN_POINT('Ctrl Pts',(40.5449118646811,2.43121974623194,3.09170549629499));
#84855=CARTESIAN_POINT('Ctrl Pts',(40.5433171200684,2.45578294099633,3.07223058036415));
#84856=CARTESIAN_POINT('Ctrl Pts',(40.5417223754557,2.48009902229586,3.05247405224141));
#84857=CARTESIAN_POINT('Ctrl Pts',(40.5358499293217,2.56963992839446,2.97972312631378));
#84858=CARTESIAN_POINT('Ctrl Pts',(40.5299774831878,2.65612693165349,2.90290718572238));
#84859=CARTESIAN_POINT('Ctrl Pts',(40.5241050370539,2.73916824320118,2.8223122320959));
#84860=CARTESIAN_POINT('Ctrl Pts',(40.518240198109,2.82210198271784,2.74182168147909));
#84861=CARTESIAN_POINT('Ctrl Pts',(40.5123753591642,2.90159861307141,2.65756213816487));
#84862=CARTESIAN_POINT('Ctrl Pts',(40.5065105202193,2.97729840836829,2.56986053853661));
#84863=CARTESIAN_POINT('Ctrl Pts',(40.5006517100993,3.05292038723931,2.48224909271918));
#84864=CARTESIAN_POINT('Ctrl Pts',(40.4947928999793,3.12475302586017,2.39120293949301));
#84865=CARTESIAN_POINT('Ctrl Pts',(40.4889340898592,3.19247305138952,2.29708615775545));
#84866=CARTESIAN_POINT('Ctrl Pts',(40.4828483009783,3.26281664845811,2.19932315604083));
#84867=CARTESIAN_POINT('Ctrl Pts',(40.4767625120973,3.32872220444049,2.0982471091588));
#84868=CARTESIAN_POINT('Ctrl Pts',(40.4706767232163,3.38987287186793,1.99430461880173));
#84869=CARTESIAN_POINT('Ctrl Pts',(40.464824693138,3.44867470546611,1.89435462186979));
#84870=CARTESIAN_POINT('Ctrl Pts',(40.4589726630598,3.50307995977951,1.79175471236219));
#84871=CARTESIAN_POINT('Ctrl Pts',(40.4531206329815,3.55285127102775,1.68693119182629));
#84872=CARTESIAN_POINT('Ctrl Pts',(40.4472694926029,3.60261501541071,1.58212360788999));
#84873=CARTESIAN_POINT('Ctrl Pts',(40.4414183522244,3.64774604027802,1.47509345840352));
#84874=CARTESIAN_POINT('Ctrl Pts',(40.4355672118459,3.68805374272889,1.36629008294119));
#84875=CARTESIAN_POINT('Ctrl Pts',(40.4297155442784,3.72836507691226,1.25747690427175));
#84876=CARTESIAN_POINT('Ctrl Pts',(40.4238638767109,3.76385208116434,1.14689056965885));
#84877=CARTESIAN_POINT('Ctrl Pts',(40.4180122091434,3.79437319888796,1.03499808094545));
#84878=CARTESIAN_POINT('Ctrl Pts',(40.4121585974591,3.82490445673235,0.923068417861169));
#84879=CARTESIAN_POINT('Ctrl Pts',(40.4063049857749,3.8504664387394,0.809832136374644));
#84880=CARTESIAN_POINT('Ctrl Pts',(40.4004513740906,3.87096828653383,0.695768298105991));
#84881=CARTESIAN_POINT('Ctrl Pts',(40.3945911079907,3.89149344093353,0.581574791483559));
#84882=CARTESIAN_POINT('Ctrl Pts',(40.3887308418908,3.90694690638146,0.466552257409715));
#84883=CARTESIAN_POINT('Ctrl Pts',(40.3828705757909,3.91728946762736,0.351186883034859));
#84884=CARTESIAN_POINT('Ctrl Pts',(40.3770063626196,3.92763899490981,0.235743806493633));
#84885=CARTESIAN_POINT('Ctrl Pts',(40.3711421494482,3.93287074496085,0.119957841781663));
#84886=CARTESIAN_POINT('Ctrl Pts',(40.3652779362769,3.93299763246142,0.00431544353016689));
#84887=CARTESIAN_POINT('Ctrl Pts',(40.3594050877026,3.93312470681139,-0.111497245036857));
#84888=CARTESIAN_POINT('Ctrl Pts',(40.3535322391283,3.92813193350777,-0.227165533792494));
#84889=CARTESIAN_POINT('Ctrl Pts',(40.347659390554,3.91808408127113,-0.342207732364104));
#84890=CARTESIAN_POINT('Ctrl Pts',(40.3460646459413,3.91535563390519,-0.373446904305652));
#84891=CARTESIAN_POINT('Ctrl Pts',(40.3444699013287,3.91225473193894,-0.404639969150923));
#84892=CARTESIAN_POINT('Ctrl Pts',(40.342875156716,3.90878331850588,-0.435777430542405));
#84893=CARTESIAN_POINT('Ctrl Pts',(40.3370027105821,3.89600027585911,-0.550437209492545));
#84894=CARTESIAN_POINT('Ctrl Pts',(40.3311302644482,3.87814643010622,-0.66472601320237));
#84895=CARTESIAN_POINT('Ctrl Pts',(40.3252578183143,3.85525052411216,-0.778159621371421));
#84896=CARTESIAN_POINT('Ctrl Pts',(40.3193929793694,3.83238427756186,-0.891446287212729));
#84897=CARTESIAN_POINT('Ctrl Pts',(40.3135281404246,3.80448904063948,-1.00387955913017));
#84898=CARTESIAN_POINT('Ctrl Pts',(40.3076633014797,3.77164532767107,-1.11498005464538));
#84899=CARTESIAN_POINT('Ctrl Pts',(40.3018044913597,3.73883537675374,-1.22596634320083));
#84900=CARTESIAN_POINT('Ctrl Pts',(40.2959456812397,3.70108718427368,-1.33562218642375));
#84901=CARTESIAN_POINT('Ctrl Pts',(40.2900868711197,3.65853221970939,-1.44347878313062));
#84902=CARTESIAN_POINT('Ctrl Pts',(40.2840010822387,3.61432861439189,-1.55551390007959));
#84903=CARTESIAN_POINT('Ctrl Pts',(40.2779152933577,3.5649383516893,-1.66560709475051));
#84904=CARTESIAN_POINT('Ctrl Pts',(40.2718295044768,3.51056579425569,-1.77325035012035));
#84905=CARTESIAN_POINT('Ctrl Pts',(40.2659774743985,3.45828171937946,-1.87675896345987));
#84906=CARTESIAN_POINT('Ctrl Pts',(40.2601254443202,3.40139123898617,-1.97800196997601));
#84907=CARTESIAN_POINT('Ctrl Pts',(40.254273414242,3.34012461671111,-2.07654919152918));
#84908=CARTESIAN_POINT('Ctrl Pts',(40.2484222738635,3.27886730896415,-2.17508143068523));
#84909=CARTESIAN_POINT('Ctrl Pts',(40.2425711334849,3.21323540038668,-2.27091834883834));
#84910=CARTESIAN_POINT('Ctrl Pts',(40.2367199931064,3.143503818494,-2.36365664662058));
#84911=CARTESIAN_POINT('Ctrl Pts',(40.2308683255389,3.07376595377106,-2.45640330014304));
#84912=CARTESIAN_POINT('Ctrl Pts',(40.2250166579714,2.99992792987121,-2.54605044789692));
#84913=CARTESIAN_POINT('Ctrl Pts',(40.2191649904039,2.92230605180612,-2.63222649853262));
#84914=CARTESIAN_POINT('Ctrl Pts',(40.2133113787197,2.84465838519605,-2.71843117969123));
#84915=CARTESIAN_POINT('Ctrl Pts',(40.2074577670355,2.76322464121197,-2.80116216366751));
#84916=CARTESIAN_POINT('Ctrl Pts',(40.2016041553512,2.67835868270532,-2.88008398606308));
#84917=CARTESIAN_POINT('Ctrl Pts',(40.1957438892513,2.59339624814367,-2.95909552718937));
#84918=CARTESIAN_POINT('Ctrl Pts',(40.1898836231515,2.50499411415356,-3.03428898199129));
#84919=CARTESIAN_POINT('Ctrl Pts',(40.1840233570516,2.41354006161249,-3.10536847588037));
#84920=CARTESIAN_POINT('Ctrl Pts',(40.1781591438803,2.32202441192372,-3.17649584401845));
#84921=CARTESIAN_POINT('Ctrl Pts',(40.172294930709,2.22745308709818,-3.24350349547377));
#84922=CARTESIAN_POINT('Ctrl Pts',(40.1664307175377,2.1302422802082,-3.30613926319104));
#84923=CARTESIAN_POINT('Ctrl Pts',(40.1605578689634,2.03288832461819,-3.36886726580493));
#84924=CARTESIAN_POINT('Ctrl Pts',(40.1546850203891,1.93288748538726,-3.42721032847708));
#84925=CARTESIAN_POINT('Ctrl Pts',(40.1488121718148,1.83067998586112,-3.48096248031597));
#84926=CARTESIAN_POINT('Ctrl Pts',(40.147217427202,1.80292601652283,-3.49555862620468));
#84927=CARTESIAN_POINT('Ctrl Pts',(40.1456226825891,1.77500944286886,-3.50981652938437));
#84928=CARTESIAN_POINT('Ctrl Pts',(40.1440279379763,1.746939303992,-3.5237326896585));
#84929=CARTESIAN_POINT('Ctrl Pts',(40.1381554918424,1.64357455379922,-3.57497719673732));
#84930=CARTESIAN_POINT('Ctrl Pts',(40.1322830457085,1.53778003612507,-3.62175550893053));
#84931=CARTESIAN_POINT('Ctrl Pts',(40.1264105995746,1.42997862296408,-3.66382998211786));
#84932=CARTESIAN_POINT('Ctrl Pts',(40.1205457606298,1.32231685616405,-3.70584995187246));
#84933=CARTESIAN_POINT('Ctrl Pts',(40.114680921685,1.212653745353,-3.74317805126427));
#84934=CARTESIAN_POINT('Ctrl Pts',(40.1088160827401,1.10143608626553,-3.77562280264754));
#84935=CARTESIAN_POINT('Ctrl Pts',(40.1029572726201,0.990332754577357,-3.80803420209663));
#84936=CARTESIAN_POINT('Ctrl Pts',(40.0970984625001,0.877678447586047,-3.83557212330901));
#84937=CARTESIAN_POINT('Ctrl Pts',(40.0912396523801,0.763938611919312,-3.85809367398185));
#84938=CARTESIAN_POINT('Ctrl Pts',(40.0851538634991,0.645792330840744,-3.88148774203657));
#84939=CARTESIAN_POINT('Ctrl Pts',(40.0790680746182,0.526475133337671,-3.8994687304049));
#84940=CARTESIAN_POINT('Ctrl Pts',(40.0729822857372,0.406524868837962,-3.91193386076711));
#84941=CARTESIAN_POINT('Ctrl Pts',(40.0671302556589,0.291181965974274,-3.92392019799237));
#84942=CARTESIAN_POINT('Ctrl Pts',(40.0612782255807,0.175254181137358,-3.93080654902714));
#84943=CARTESIAN_POINT('Ctrl Pts',(40.0554261955024,0.0592278899181963,
-3.9325540119693));
#84944=CARTESIAN_POINT('Ctrl Pts',(40.0495750551239,-0.0567807615142353,
-3.93430120924));
#84945=CARTESIAN_POINT('Ctrl Pts',(40.0437239147454,-0.172887476354015,
-3.93091106563208));
#84946=CARTESIAN_POINT('Ctrl Pts',(40.0378727743669,-0.288604339455222,
-3.92239678452443));
#84947=CARTESIAN_POINT('Ctrl Pts',(40.0320211067994,-0.404331628670237,
-3.91388173627826));
#84948=CARTESIAN_POINT('Ctrl Pts',(40.0261694392319,-0.519668584052631,
-3.90024166307759));
#84949=CARTESIAN_POINT('Ctrl Pts',(40.0203177716645,-0.634131590288176,
-3.88154172027026));
#84950=CARTESIAN_POINT('Ctrl Pts',(40.0144641599802,-0.748632624905172,
-3.86283556472589));
#84951=CARTESIAN_POINT('Ctrl Pts',(40.008610548296,-0.862258725289931,-3.83906626351055));
#84952=CARTESIAN_POINT('Ctrl Pts',(40.0027569366118,-0.974536358533108,
-3.81035010017413));
#84953=CARTESIAN_POINT('Ctrl Pts',(39.9968966705119,-1.08694162956307,-3.78160129215661));
#84954=CARTESIAN_POINT('Ctrl Pts',(39.991036404412,-1.1979949730428,-3.74789449994818));
#84955=CARTESIAN_POINT('Ctrl Pts',(39.9851761383122,-1.30723781953995,-3.70939594586025));
#84956=CARTESIAN_POINT('Ctrl Pts',(39.9793119251409,-1.41655424449064,-3.67087146179919));
#84957=CARTESIAN_POINT('Ctrl Pts',(39.9734477119696,-1.52405736187819,-3.62754894358141));
#84958=CARTESIAN_POINT('Ctrl Pts',(39.9675834987983,-1.62931000667219,-3.57964214722057));
#84959=CARTESIAN_POINT('Ctrl Pts',(39.961710650224,-1.73471764225125,-3.53166480525024));
#84960=CARTESIAN_POINT('Ctrl Pts',(39.9558378016497,-1.83786782434999,-3.47908989924171));
#84961=CARTESIAN_POINT('Ctrl Pts',(39.9499649530754,-1.93834925514787,-3.42217637842758));
#84962=CARTESIAN_POINT('Ctrl Pts',(39.9483702084626,-1.96563451858214,-3.40672177755203));
#84963=CARTESIAN_POINT('Ctrl Pts',(39.9467754638497,-1.99272317105285,-3.39094750118053));
#84964=CARTESIAN_POINT('Ctrl Pts',(39.9451807192368,-2.01960738063346,-3.3748592604864));
#84965=CARTESIAN_POINT('Ctrl Pts',(39.9393082731029,-2.11860509559063,-3.31561634089736));
#84966=CARTESIAN_POINT('Ctrl Pts',(39.933435826969,-2.21515960775382,-3.25191456193877));
#84967=CARTESIAN_POINT('Ctrl Pts',(39.9275633808351,-2.30884235755335,-3.18398115069287));
#84968=CARTESIAN_POINT('Ctrl Pts',(39.9216985418903,-2.40240375036212,-3.11613574064653));
#84969=CARTESIAN_POINT('Ctrl Pts',(39.9158337029454,-2.49310044719666,-3.0440698398317));
#84970=CARTESIAN_POINT('Ctrl Pts',(39.9099688640006,-2.580529788326,-2.96805576287949));
#84971=CARTESIAN_POINT('Ctrl Pts',(39.9041100538806,-2.66786925551552,-2.89211982542243));
#84972=CARTESIAN_POINT('Ctrl Pts',(39.8982512437606,-2.75194773759665,-2.81224405413166));
#84973=CARTESIAN_POINT('Ctrl Pts',(39.8923924336406,-2.83239336053307,-2.72874272352822));
#84974=CARTESIAN_POINT('Ctrl Pts',(39.8863066447596,-2.91595556302168,-2.64200643084679));
#84975=CARTESIAN_POINT('Ctrl Pts',(39.8802208558787,-2.99559736112515,-2.55135824521931));
#84976=CARTESIAN_POINT('Ctrl Pts',(39.8741350669977,-3.07094147611195,-2.45719503708911));
#84977=CARTESIAN_POINT('Ctrl Pts',(39.8682830369194,-3.14339157843153,-2.36664869428625));
#84978=CARTESIAN_POINT('Ctrl Pts',(39.8624310068412,-3.21186777857737,-2.2728527288008));
#84979=CARTESIAN_POINT('Ctrl Pts',(39.8565789767629,-3.27607436366046,-2.17619524945872));
#84980=CARTESIAN_POINT('Ctrl Pts',(39.8507278363844,-3.34027118724505,-2.0795524652112));
#84981=CARTESIAN_POINT('Ctrl Pts',(39.8448766960059,-3.40019945777604,-1.98004937633592));
#84982=CARTESIAN_POINT('Ctrl Pts',(39.8390255556274,-3.4556064613382,-1.87810356060514));
#84983=CARTESIAN_POINT('Ctrl Pts',(39.8331738880599,-3.51101845708308,-1.77614855953483));
#84984=CARTESIAN_POINT('Ctrl Pts',(39.8273222204924,-3.56190817865106,-1.67175075729493));
#84985=CARTESIAN_POINT('Ctrl Pts',(39.8214705529249,-3.60806893954932,-1.56535220556252));
#84986=CARTESIAN_POINT('Ctrl Pts',(39.8156169412407,-3.65424503657302,-1.45891830472615));
#84987=CARTESIAN_POINT('Ctrl Pts',(39.8097633295565,-3.69568888442674,-1.35048271165834));
#84988=CARTESIAN_POINT('Ctrl Pts',(39.8039097178723,-3.73224225777654,-1.24050664216967));
#84989=CARTESIAN_POINT('Ctrl Pts',(39.7980494517724,-3.76883718518785,-1.13040555132353));
#84990=CARTESIAN_POINT('Ctrl Pts',(39.7921891856725,-3.80053041103256,-1.0187608811661));
#84991=CARTESIAN_POINT('Ctrl Pts',(39.7863289195726,-3.82721380981329,-0.906048262497335));
#84992=CARTESIAN_POINT('Ctrl Pts',(39.7804647064014,-3.85391518069266,-0.793259728375754));
#84993=CARTESIAN_POINT('Ctrl Pts',(39.7746004932301,-3.87559992850287,-0.679402218543763));
#84994=CARTESIAN_POINT('Ctrl Pts',(39.7687362800588,-3.8922114870999,-0.56495906018719));
#84995=CARTESIAN_POINT('Ctrl Pts',(39.7628634314845,-3.90884750720583,-0.450347377467224));
#84996=CARTESIAN_POINT('Ctrl Pts',(39.7569905829102,-3.92039538724821,-0.335148734787296));
#84997=CARTESIAN_POINT('Ctrl Pts',(39.7511177343359,-3.92685056468687,-0.219849136041925));
#84998=CARTESIAN_POINT('Ctrl Pts',(39.749522989723,-3.92860343798432,-0.188540068279316));
#84999=CARTESIAN_POINT('Ctrl Pts',(39.7479282451101,-3.92998108784378,-0.157223539597995));
#85000=CARTESIAN_POINT('Ctrl Pts',(39.7463335004972,-3.93098408375229,-0.125909226374263));
#85001=CARTESIAN_POINT('Ctrl Pts',(39.7442101743431,-3.93231952481774,-0.0842157165003056));
#85002=CARTESIAN_POINT('Ctrl Pts',(39.742086848189,-3.93299166275049,-0.0425008473423755));
#85003=CARTESIAN_POINT('Ctrl Pts',(39.7399635220349,-3.93299992292071,-0.000778656347341876));
#85004=CARTESIAN_POINT('',(38.4899635541443,-3.93221249083461,-0.00323415915035297));
#85005=CARTESIAN_POINT('Ctrl Pts',(39.7399635219896,-3.93299992292088,-0.000778655457617156));
#85006=CARTESIAN_POINT('Ctrl Pts',(39.7341222016867,-3.93302264681791,0.114000075487013));
#85007=CARTESIAN_POINT('Ctrl Pts',(39.7282808813837,-3.92801663955931,0.228980042591623));
#85008=CARTESIAN_POINT('Ctrl Pts',(39.7224395610808,-3.91795511212009,0.343681159524406));
#85009=CARTESIAN_POINT('Ctrl Pts',(39.7166057401983,-3.90790650224411,0.458235016616241));
#85010=CARTESIAN_POINT('Ctrl Pts',(39.7107719193158,-3.8928153129585,0.572510322663808));
#85011=CARTESIAN_POINT('Ctrl Pts',(39.7049380984333,-3.87270674435775,0.686025853890374));
#85012=CARTESIAN_POINT('Ctrl Pts',(39.6991101642807,-3.85261846669758,0.799426840071701));
#85013=CARTESIAN_POINT('Ctrl Pts',(39.6932822301281,-3.82752295049738,0.912069166749725));
#85014=CARTESIAN_POINT('Ctrl Pts',(39.6874542959755,-3.79749722697163,1.02347633638633));
#85015=CARTESIAN_POINT('Ctrl Pts',(39.6816222953831,-3.7674505530035,1.13496124035252));
#85016=CARTESIAN_POINT('Ctrl Pts',(39.6757902947907,-3.7324668492666,1.24520884713989));
#85017=CARTESIAN_POINT('Ctrl Pts',(39.6699582941983,-3.69267473507464,1.35375119609972));
#85018=CARTESIAN_POINT('Ctrl Pts',(39.6641366491117,-3.6529532771636,1.46210081343785));
#85019=CARTESIAN_POINT('Ctrl Pts',(39.6583150040252,-3.60844060355128,1.56875082642146));
#85020=CARTESIAN_POINT('Ctrl Pts',(39.6524933589386,-3.55931438831396,1.67325135145357));
#85021=CARTESIAN_POINT('Ctrl Pts',(39.6466724354933,-3.5101942626788,1.77773892277819));
#85022=CARTESIAN_POINT('Ctrl Pts',(39.640851512048,-3.45646191029779,1.88007715749181));
#85023=CARTESIAN_POINT('Ctrl Pts',(39.6350305886027,-3.39834244097618,1.97983778473391));
#85024=CARTESIAN_POINT('Ctrl Pts',(39.6292089391354,-3.34021572263118,2.07961085474481));
#85025=CARTESIAN_POINT('Ctrl Pts',(39.6233872896681,-3.27770101050125,2.17680531706256));
#85026=CARTESIAN_POINT('Ctrl Pts',(39.6175656402009,-3.21106809880611,2.2710197411801));
#85027=CARTESIAN_POINT('Ctrl Pts',(39.6117256936639,-3.14422576415691,2.36553027517054));
#85028=CARTESIAN_POINT('Ctrl Pts',(39.605885747127,-3.07323954689038,2.45704166411266));
#85029=CARTESIAN_POINT('Ctrl Pts',(39.60004580059,-2.9984232303731,2.54518115888809));
#85030=CARTESIAN_POINT('Ctrl Pts',(39.5942152834158,-2.92372771465095,2.63317834084265));
#85031=CARTESIAN_POINT('Ctrl Pts',(39.5883847662415,-2.84521477321636,2.71781422872262));
#85032=CARTESIAN_POINT('Ctrl Pts',(39.5825542490673,-2.76323366118692,2.79875485415988));
#85033=CARTESIAN_POINT('Ctrl Pts',(39.576709587849,-2.68105367409605,2.87989183057919));
#85034=CARTESIAN_POINT('Ctrl Pts',(39.5708649266307,-2.59538899735307,2.95731532969188));
#85035=CARTESIAN_POINT('Ctrl Pts',(39.5650202654124,-2.5066238357333,3.03073026614604));
#85036=CARTESIAN_POINT('Ctrl Pts',(39.5591756041941,-2.41785867411354,3.10414520260021));
#85037=CARTESIAN_POINT('Ctrl Pts',(39.5533309429757,-2.32599339744468,3.17355137528231));
#85038=CARTESIAN_POINT('Ctrl Pts',(39.5474862817574,-2.231439307828,3.23869844466571));
#85039=CARTESIAN_POINT('Ctrl Pts',(39.5416138356235,-2.13643571783778,3.30415521648654));
#85040=CARTESIAN_POINT('Ctrl Pts',(39.5357413894896,-2.03839047734439,3.36553779771454));
#85041=CARTESIAN_POINT('Ctrl Pts',(39.5298689433557,-1.93768826068458,3.4225506869008));
#85042=CARTESIAN_POINT('Ctrl Pts',(39.5240041044108,-1.83711649405956,3.47948972137339));
#85043=CARTESIAN_POINT('Ctrl Pts',(39.518139265466,-1.73389495229055,3.53207011878397));
#85044=CARTESIAN_POINT('Ctrl Pts',(39.5122744265212,-1.6284385705889,3.58003866205637));
#85045=CARTESIAN_POINT('Ctrl Pts',(39.5064156164011,-1.52309059391863,3.62795789554443));
#85046=CARTESIAN_POINT('Ctrl Pts',(39.5005568062811,-1.41551272082882,3.67127453449536));
#85047=CARTESIAN_POINT('Ctrl Pts',(39.4946979961611,-1.30614527324796,3.70978079206468));
#85048=CARTESIAN_POINT('Ctrl Pts',(39.4886122072801,-1.19254077288174,3.74977883763395));
#85049=CARTESIAN_POINT('Ctrl Pts',(39.4825264183991,-1.07700562759994,3.78458601745905));
#85050=CARTESIAN_POINT('Ctrl Pts',(39.4764406295182,-0.960057541266778,
3.81402392722657));
#85051=CARTESIAN_POINT('Ctrl Pts',(39.4705885994399,-0.847601501104463,
3.84233110921568));
#85052=CARTESIAN_POINT('Ctrl Pts',(39.4647365693616,-0.73383949939955,3.86567377607085));
#85053=CARTESIAN_POINT('Ctrl Pts',(39.4588845392834,-0.619247398138756,
3.88394408557826));
#85054=CARTESIAN_POINT('Ctrl Pts',(39.4530333989049,-0.504672718621039,
3.90221161740175));
#85055=CARTESIAN_POINT('Ctrl Pts',(39.4471822585263,-0.389268598568526,
3.91540826013805));
#85056=CARTESIAN_POINT('Ctrl Pts',(39.4413311181478,-0.273519851921076,
3.92347752518159));
#85057=CARTESIAN_POINT('Ctrl Pts',(39.4354794505803,-0.157760676287066,
3.93154751726762));
#85058=CARTESIAN_POINT('Ctrl Pts',(39.4296277830128,-0.0416572247126819,
3.93448918454312));
#85059=CARTESIAN_POINT('Ctrl Pts',(39.4237761154453,0.074302538509432,3.93229807272682));
#85060=CARTESIAN_POINT('Ctrl Pts',(39.4179225037611,0.190300827385199,3.93010623295099));
#85061=CARTESIAN_POINT('Ctrl Pts',(39.4120688920769,0.306154919920153,3.92277823104649));
#85062=CARTESIAN_POINT('Ctrl Pts',(39.4062152803926,0.421379542415999,3.91036165606626));
#85063=CARTESIAN_POINT('Ctrl Pts',(39.4003550142927,0.536735152850913,3.89793096586021));
#85064=CARTESIAN_POINT('Ctrl Pts',(39.3944947481928,0.651459453743064,3.88040020079199));
#85065=CARTESIAN_POINT('Ctrl Pts',(39.3886344820929,0.765074862772757,3.85786851180198));
#85066=CARTESIAN_POINT('Ctrl Pts',(39.3827702689216,0.878766795312571,3.83532164701896));
#85067=CARTESIAN_POINT('Ctrl Pts',(39.3769060557504,0.991347948291256,3.80776724942484));
#85068=CARTESIAN_POINT('Ctrl Pts',(39.3710418425791,1.10235514877109,3.77535456957063));
#85069=CARTESIAN_POINT('Ctrl Pts',(39.3651689940048,1.21352581396196,3.7428941601158));
#85070=CARTESIAN_POINT('Ctrl Pts',(39.3592961454305,1.32311751110444,3.70556132301106));
#85071=CARTESIAN_POINT('Ctrl Pts',(39.3534232968562,1.43068622752751,3.66355372805738));
#85072=CARTESIAN_POINT('Ctrl Pts',(39.3518285522434,1.45989601028432,3.65214676176146));
#85073=CARTESIAN_POINT('Ctrl Pts',(39.3502338076306,1.48895676312913,3.64039535624159));
#85074=CARTESIAN_POINT('Ctrl Pts',(39.3486390630179,1.51785991994509,3.62830404781963));
#85075=CARTESIAN_POINT('Ctrl Pts',(39.3427666168839,1.62429215376019,3.58377932779368));
#85076=CARTESIAN_POINT('Ctrl Pts',(39.33689417075,1.72894179370186,3.53449298768078));
#85077=CARTESIAN_POINT('Ctrl Pts',(39.3310217246161,1.83135226396449,3.48060883830288));
#85078=CARTESIAN_POINT('Ctrl Pts',(39.3251568856712,1.93363007131431,3.4267944906571));
#85079=CARTESIAN_POINT('Ctrl Pts',(39.3192920467263,2.03367411486602,3.36839436885132));
#85080=CARTESIAN_POINT('Ctrl Pts',(39.3134272077815,2.13104702644055,3.30562060301828));
#85081=CARTESIAN_POINT('Ctrl Pts',(39.3075683976614,2.2283198424741,3.24291136615893));
#85082=CARTESIAN_POINT('Ctrl Pts',(39.3017095875414,2.32292664278129,3.17583765056074));
#85083=CARTESIAN_POINT('Ctrl Pts',(39.2958507774214,2.41445454864099,3.10465750648068));
#85084=CARTESIAN_POINT('Ctrl Pts',(39.2897649885404,2.50952837768939,3.03071974087418));
#85085=CARTESIAN_POINT('Ctrl Pts',(39.2836791996594,2.60127952367582,2.95235114529647));
#85086=CARTESIAN_POINT('Ctrl Pts',(39.2775934107785,2.68927798352129,2.86989075181402));
#85087=CARTESIAN_POINT('Ctrl Pts',(39.2717413807002,2.77389636972064,2.79059771152558));
#85088=CARTESIAN_POINT('Ctrl Pts',(39.2658893506219,2.85504470831304,2.70752172058038));
#85089=CARTESIAN_POINT('Ctrl Pts',(39.2600373205436,2.93237497801825,2.62100476693433));
#85090=CARTESIAN_POINT('Ctrl Pts',(39.2541861801651,3.00969349099628,2.53450096669151));
#85091=CARTESIAN_POINT('Ctrl Pts',(39.2483350397866,3.08319481386154,2.44455755202576));
#85092=CARTESIAN_POINT('Ctrl Pts',(39.2424838994081,3.15256928403407,2.35155180877754));
#85093=CARTESIAN_POINT('Ctrl Pts',(39.2366322318405,3.22195000486086,2.25853768569241));
#85094=CARTESIAN_POINT('Ctrl Pts',(39.230780564273,3.28720288666852,2.16246101688231));
#85095=CARTESIAN_POINT('Ctrl Pts',(39.2249288967055,3.34806033518655,2.06372987378448));
#85096=CARTESIAN_POINT('Ctrl Pts',(39.2190752850213,3.4089380025537,1.96496592894859));
#85097=CARTESIAN_POINT('Ctrl Pts',(39.2132216733371,3.46541711611587,1.86354610790681));
#85098=CARTESIAN_POINT('Ctrl Pts',(39.2073680616529,3.51727531575113,1.75990435910813));
#85099=CARTESIAN_POINT('Ctrl Pts',(39.2015077955529,3.56919246805268,1.65614478983991));
#85100=CARTESIAN_POINT('Ctrl Pts',(39.1956475294531,3.61647803638353,1.55015862108794));
#85101=CARTESIAN_POINT('Ctrl Pts',(39.1897872633532,3.65895719374826,1.4424012112855));
#85102=CARTESIAN_POINT('Ctrl Pts',(39.1839230501818,3.70146496214628,1.33457122351704));
#85103=CARTESIAN_POINT('Ctrl Pts',(39.1780588370105,3.73915973942352,1.22496800915292));
#85104=CARTESIAN_POINT('Ctrl Pts',(39.1721946238392,3.771916634124,1.11406189469826));
#85105=CARTESIAN_POINT('Ctrl Pts',(39.1663217752649,3.80472176530183,1.00299246438819));
#85106=CARTESIAN_POINT('Ctrl Pts',(39.1604489266906,3.83257440271595,0.890616704555471));
#85107=CARTESIAN_POINT('Ctrl Pts',(39.1545760781162,3.85540074576738,0.777415004702317));
#85108=CARTESIAN_POINT('Ctrl Pts',(39.1529813335035,3.86159913265726,0.746675611594062));
#85109=CARTESIAN_POINT('Ctrl Pts',(39.1513865888908,3.86742719220224,0.715875341961086));
#85110=CARTESIAN_POINT('Ctrl Pts',(39.1497918442781,3.87288410860961,0.68502385453292));
#85111=CARTESIAN_POINT('Ctrl Pts',(39.1439193981442,3.89297851582945,0.571417138681087));
#85112=CARTESIAN_POINT('Ctrl Pts',(39.1380469520103,3.90810353902675,0.45673529994965));
#85113=CARTESIAN_POINT('Ctrl Pts',(39.1321745058764,3.91815010211211,0.341450988164994));
#85114=CARTESIAN_POINT('Ctrl Pts',(39.1263096669316,3.92818365084143,0.226316016116477));
#85115=CARTESIAN_POINT('Ctrl Pts',(39.1204448279867,3.93315178651159,0.110580531044016));
#85116=CARTESIAN_POINT('Ctrl Pts',(39.1145799890419,3.93299646542847,-0.00527284810658881));
#85117=CARTESIAN_POINT('Ctrl Pts',(39.1087211789219,3.93284130400935,-0.121007134518799));
#85118=CARTESIAN_POINT('Ctrl Pts',(39.1028623688019,3.9275731621685,-0.23685866307964));
#85119=CARTESIAN_POINT('Ctrl Pts',(39.0970035586819,3.91718586633032,-0.352340586112312));
#85120=CARTESIAN_POINT('Ctrl Pts',(39.0909177698009,3.90639615165778,-0.472296445536227));
#85121=CARTESIAN_POINT('Ctrl Pts',(39.08483198092,3.89008257456317,-0.591853029483201));
#85122=CARTESIAN_POINT('Ctrl Pts',(39.078746192039,3.86829782477532,-0.710465297420283));
#85123=CARTESIAN_POINT('Ctrl Pts',(39.0728941619607,3.84734984029886,-0.824521596972113));
#85124=CARTESIAN_POINT('Ctrl Pts',(39.0670421318825,3.82134331373662,-0.937704341699031));
#85125=CARTESIAN_POINT('Ctrl Pts',(39.0611901018042,3.79037774973595,-1.04953585660834));
#85126=CARTESIAN_POINT('Ctrl Pts',(39.0553389614257,3.75941689351263,-1.16135036947396));
#85127=CARTESIAN_POINT('Ctrl Pts',(39.0494878210472,3.72349860919663,-1.27181366272718));
#85128=CARTESIAN_POINT('Ctrl Pts',(39.0436366806687,3.68277283527244,-1.38046124312832));
#85129=CARTESIAN_POINT('Ctrl Pts',(39.0377850131013,3.64204339194754,-1.48911861269909));
#85130=CARTESIAN_POINT('Ctrl Pts',(39.0319333455338,3.59650574303546,-1.59595955712241));
#85131=CARTESIAN_POINT('Ctrl Pts',(39.0260816779663,3.54635847090481,-1.7005383253081));
#85132=CARTESIAN_POINT('Ctrl Pts',(39.0202280662821,3.49619453819819,-1.80515183800608));
#85133=CARTESIAN_POINT('Ctrl Pts',(39.0143744545979,3.44141811567231,-1.90750130749258));
#85134=CARTESIAN_POINT('Ctrl Pts',(39.0085208429137,3.382274012236,-2.00716504208125));
#85135=CARTESIAN_POINT('Ctrl Pts',(39.0026605768138,3.32306267348093,-2.10694207491223));
#85136=CARTESIAN_POINT('Ctrl Pts',(38.9968003107139,3.25947395451529,-2.20402692315999));
#85137=CARTESIAN_POINT('Ctrl Pts',(38.9909400446141,3.19179637616573,-2.29802630383016));
#85138=CARTESIAN_POINT('Ctrl Pts',(38.9850758314428,3.12407321486295,-2.3920889960058));
#85139=CARTESIAN_POINT('Ctrl Pts',(38.9792116182715,3.05225596596096,-2.48306175892373));
#85140=CARTESIAN_POINT('Ctrl Pts',(38.9733474051002,2.97667274221939,-2.57058522242078));
#85141=CARTESIAN_POINT('Ctrl Pts',(38.9674745565259,2.90097821768147,-2.65823756942801));
#85142=CARTESIAN_POINT('Ctrl Pts',(38.9616017079516,2.82150693301668,-2.7424301802827));
#85143=CARTESIAN_POINT('Ctrl Pts',(38.9557288593774,2.73862309141705,-2.82284122174049));
#85144=CARTESIAN_POINT('Ctrl Pts',(38.9541341147644,2.71611637117436,-2.84467646464894));
#85145=CARTESIAN_POINT('Ctrl Pts',(38.9525393701515,2.69335820126911,-2.86623310145387));
#85146=CARTESIAN_POINT('Ctrl Pts',(38.9509446255386,2.6703562656032,-2.88750522332926));
#85147=CARTESIAN_POINT('Ctrl Pts',(38.9450721794047,2.58565453525737,-2.9658371323104));
#85148=CARTESIAN_POINT('Ctrl Pts',(38.9391997332708,2.4973614051379,-3.04057008110341));
#85149=CARTESIAN_POINT('Ctrl Pts',(38.9333272871369,2.40581549393361,-3.11135674732889));
#85150=CARTESIAN_POINT('Ctrl Pts',(38.927462448192,2.31438817165108,-3.18205171623755));
#85151=CARTESIAN_POINT('Ctrl Pts',(38.9215976092472,2.21971677175287,-3.24881031806787));
#85152=CARTESIAN_POINT('Ctrl Pts',(38.9157327703023,2.12217589277859,-3.31132276894135));
#85153=CARTESIAN_POINT('Ctrl Pts',(38.9098739601823,2.02473528200919,-3.37377095946267));
#85154=CARTESIAN_POINT('Ctrl Pts',(38.9040151500623,1.92443140523235,-3.43198145930564));
#85155=CARTESIAN_POINT('Ctrl Pts',(38.8981563399423,1.8216704649381,-3.48568583167964));
#85156=CARTESIAN_POINT('Ctrl Pts',(38.8920705510613,1.71492841748643,-3.54147078895906));
#85157=CARTESIAN_POINT('Ctrl Pts',(38.8859847621803,1.60553543515362,-3.59239313158994));
#85158=CARTESIAN_POINT('Ctrl Pts',(38.8798989732994,1.49397850077039,-3.6382024736449));
#85159=CARTESIAN_POINT('Ctrl Pts',(38.8740469432211,1.38670653517688,-3.6822522513835));
#85160=CARTESIAN_POINT('Ctrl Pts',(38.8681949131429,1.27743420618785,-3.72157439838867));
#85161=CARTESIAN_POINT('Ctrl Pts',(38.8623428830646,1.16661714144689,-3.7559943350972));
#85162=CARTESIAN_POINT('Ctrl Pts',(38.8564917426861,1.05581692451981,-3.79040903885096));
#85163=CARTESIAN_POINT('Ctrl Pts',(38.8506406023076,0.9434728334458,-3.81992289162211));
#85164=CARTESIAN_POINT('Ctrl Pts',(38.844789461929,0.830056677352447,-3.84441086674963));
#85165=CARTESIAN_POINT('Ctrl Pts',(38.8389377943615,0.716630302439545,-3.86890104824886));
#85166=CARTESIAN_POINT('Ctrl Pts',(38.833086126794,0.602132074559348,-3.88836436467114));
#85167=CARTESIAN_POINT('Ctrl Pts',(38.8272344592265,0.487044339022436,-3.90272684309653));
#85168=CARTESIAN_POINT('Ctrl Pts',(38.8213808475423,0.371918367548383,-3.9170940932104));
#85169=CARTESIAN_POINT('Ctrl Pts',(38.8155272358581,0.256202908932304,-3.92635708442548));
#85170=CARTESIAN_POINT('Ctrl Pts',(38.8096736241738,0.140385064663461,-3.93049373916553));
#85171=CARTESIAN_POINT('Ctrl Pts',(38.8038133580739,0.0244355580779736,
-3.93463509647581));
#85172=CARTESIAN_POINT('Ctrl Pts',(38.797953091974,-0.0916161531383416,
-3.93363847076239));
#85173=CARTESIAN_POINT('Ctrl Pts',(38.7920928258741,-0.20728322965967,-3.92753391617461));
#85174=CARTESIAN_POINT('Ctrl Pts',(38.7862286127029,-0.3230282115524,-3.92142524997956));
#85175=CARTESIAN_POINT('Ctrl Pts',(38.7803643995316,-0.438387632494599,
-3.91020184441281));
#85176=CARTESIAN_POINT('Ctrl Pts',(38.7745001863604,-0.552881773172785,
-3.89394539572569));
#85177=CARTESIAN_POINT('Ctrl Pts',(38.7686273377861,-0.667544513289531,
-3.87766500845006));
#85178=CARTESIAN_POINT('Ctrl Pts',(38.7627544892118,-0.781339025385813,
-3.85633686212652));
#85179=CARTESIAN_POINT('Ctrl Pts',(38.7568816406375,-0.893797652072539,
-3.83009330919622));
#85180=CARTESIAN_POINT('Ctrl Pts',(38.7552868960246,-0.924335267134304,
-3.82296699491646));
#85181=CARTESIAN_POINT('Ctrl Pts',(38.7536921514118,-0.954774477665476,
-3.81547851376626));
#85182=CARTESIAN_POINT('Ctrl Pts',(38.7520974067989,-0.98510615834445,-3.80763113454965));
#85183=CARTESIAN_POINT('Ctrl Pts',(38.746224960665,-1.09679875131735,-3.77873414918237));
#85184=CARTESIAN_POINT('Ctrl Pts',(38.7403525145311,-1.20740577352903,-3.74487005168703));
#85185=CARTESIAN_POINT('Ctrl Pts',(38.7344800683971,-1.31645195970563,-3.70613589035632));
#85186=CARTESIAN_POINT('Ctrl Pts',(38.7286152294523,-1.42535688703736,-3.66745190540571));
#85187=CARTESIAN_POINT('Ctrl Pts',(38.7227503905074,-1.53270461327704,-3.62391053946211));
#85188=CARTESIAN_POINT('Ctrl Pts',(38.7168855515626,-1.63803199619866,-3.57565940484122));
#85189=CARTESIAN_POINT('Ctrl Pts',(38.7110267414425,-1.74325110669441,-3.52745787049758));
#85190=CARTESIAN_POINT('Ctrl Pts',(38.7051679313225,-1.84645363126394,-3.47455636852455));
#85191=CARTESIAN_POINT('Ctrl Pts',(38.6993091212024,-1.94719412064057,-3.41715145355642));
#85192=CARTESIAN_POINT('Ctrl Pts',(38.6932233323215,-2.05183744198914,-3.35752258932152));
#85193=CARTESIAN_POINT('Ctrl Pts',(38.6871375434405,-2.15382367618305,-3.29303446950404));
#85194=CARTESIAN_POINT('Ctrl Pts',(38.6810517545595,-2.25267887974533,-3.22396136216756));
#85195=CARTESIAN_POINT('Ctrl Pts',(38.6751997244813,-2.34773699562076,-3.15754139433116));
#85196=CARTESIAN_POINT('Ctrl Pts',(38.669347694403,-2.43989980335057,-3.08688242463019));
#85197=CARTESIAN_POINT('Ctrl Pts',(38.6634956643247,-2.52877408251778,-3.01227333414256));
#85198=CARTESIAN_POINT('Ctrl Pts',(38.6576445239462,-2.61763484989107,-2.93767558667415));
#85199=CARTESIAN_POINT('Ctrl Pts',(38.6517933835677,-2.70320776629022,-2.85912917820392));
#85200=CARTESIAN_POINT('Ctrl Pts',(38.6459422431892,-2.78513254614726,-2.77696339558001));
#85201=CARTESIAN_POINT('Ctrl Pts',(38.6400905756216,-2.86706470744469,-2.69479020980131));
#85202=CARTESIAN_POINT('Ctrl Pts',(38.6342389080541,-2.9453477869035,-2.60899729433365));
#85203=CARTESIAN_POINT('Ctrl Pts',(38.6283872404865,-3.01965874879582,-2.51995040443673));
#85204=CARTESIAN_POINT('Ctrl Pts',(38.6225336288023,-3.09399439923746,-2.43087393022981));
#85205=CARTESIAN_POINT('Ctrl Pts',(38.616680017118,-3.16435504332694,-2.33854164913412));
#85206=CARTESIAN_POINT('Ctrl Pts',(38.6108264054338,-3.23045872844755,-2.24335137769299));
#85207=CARTESIAN_POINT('Ctrl Pts',(38.6049661393339,-3.29663756057493,-2.14805289346525));
#85208=CARTESIAN_POINT('Ctrl Pts',(38.599105873234,-3.35854953867246,-2.04989027376121));
#85209=CARTESIAN_POINT('Ctrl Pts',(38.5932456071341,-3.41595670555015,-1.94928930274778));
#85210=CARTESIAN_POINT('Ctrl Pts',(38.5873813939628,-3.47340253793976,-1.84862057385229));
#85211=CARTESIAN_POINT('Ctrl Pts',(38.5815171807914,-3.52633732922251,-1.74551059031613));
#85212=CARTESIAN_POINT('Ctrl Pts',(38.5756529676201,-3.57457041386852,-1.64040707030171));
#85213=CARTESIAN_POINT('Ctrl Pts',(38.5697801190458,-3.62287452460275,-1.53514877909776));
#85214=CARTESIAN_POINT('Ctrl Pts',(38.5639072704715,-3.66646295564883,-1.4278914740419));
#85215=CARTESIAN_POINT('Ctrl Pts',(38.5580344218972,-3.70519417592132,-1.31910011701869));
#85216=CARTESIAN_POINT('Ctrl Pts',(38.5564396772845,-3.71571145796756,-1.28955833191726));
#85217=CARTESIAN_POINT('Ctrl Pts',(38.5548449326719,-3.72587087367678,-1.25990349824903));
#85218=CARTESIAN_POINT('Ctrl Pts',(38.5532501880592,-3.73567023864127,-1.23014505979169));
#85219=CARTESIAN_POINT('Ctrl Pts',(38.5462392868433,-3.77875072889645,-1.0993194274556));
#85220=CARTESIAN_POINT('Ctrl Pts',(38.5392283856274,-3.81498593538232,-0.966134731394327));
#85221=CARTESIAN_POINT('Ctrl Pts',(38.5322174844115,-3.84415332338129,-0.831248594787745));
#85222=CARTESIAN_POINT('Ctrl Pts',(38.5251751644464,-3.87345142251401,-0.695757977593311));
#85223=CARTESIAN_POINT('Ctrl Pts',(38.5181328444814,-3.89561804847248,-0.558550643918599));
#85224=CARTESIAN_POINT('Ctrl Pts',(38.5110905245163,-3.91047620229872,-0.420315204644498));
#85225=CARTESIAN_POINT('Ctrl Pts',(38.5040482045513,-3.92533435612497,-0.282079765370396));
#85226=CARTESIAN_POINT('Ctrl Pts',(38.4970058845862,-3.93288385965473,-0.142816253941332));
#85227=CARTESIAN_POINT('Ctrl Pts',(38.4899635646211,-3.93299866955088,-0.00323501329192832));
#85228=CARTESIAN_POINT('',(37.2399634924685,-3.93111579142054,0.00213576531572005));
#85229=CARTESIAN_POINT('Ctrl Pts',(38.4899635220349,-3.92980300012612,-0.00323154136619402));
#85230=CARTESIAN_POINT('Ctrl Pts',(38.4447766711298,-3.92290905173679,0.891666188285667));
#85231=CARTESIAN_POINT('Ctrl Pts',(38.3333074139783,-3.17538053464665,3.10966251113421));
#85232=CARTESIAN_POINT('Ctrl Pts',(38.1555557505799,0.511208908507071,4.62348953424194));
#85233=CARTESIAN_POINT('Ctrl Pts',(37.9567085318404,4.16573650181501,2.06993464119223));
#85234=CARTESIAN_POINT('Ctrl Pts',(37.7578613131006,3.99370385220429,-2.38501982428893));
#85235=CARTESIAN_POINT('Ctrl Pts',(37.5590140943612,0.153136628653335,-4.64914392058655));
#85236=CARTESIAN_POINT('Ctrl Pts',(37.386381497339,-3.30324063369252,-2.90718042645609));
#85237=CARTESIAN_POINT('Ctrl Pts',(37.2800313065638,-3.92374991679303,-0.792479136698486));
#85238=CARTESIAN_POINT('Ctrl Pts',(37.2399635220349,-3.92764697970144,0.00213329408759316));
#85239=CARTESIAN_POINT('',(35.9899635220349,-3.93452019141862,0.00241941282782897));
#85240=CARTESIAN_POINT('Ctrl Pts',(37.2399634764134,-3.932999419371,0.00213710723760822));
#85241=CARTESIAN_POINT('Ctrl Pts',(37.2334098247858,-3.93292870039597,0.132283916372161));
#85242=CARTESIAN_POINT('Ctrl Pts',(37.2268561731581,-3.92639368087127,0.262202170396104));
#85243=CARTESIAN_POINT('Ctrl Pts',(37.2203025215305,-3.91348782244965,0.391282587829128));
#85244=CARTESIAN_POINT('Ctrl Pts',(37.2137879833111,-3.90065898858428,0.519592629395078));
#85245=CARTESIAN_POINT('Ctrl Pts',(37.2072734450916,-3.88153532829353,0.64707459334773));
#85246=CARTESIAN_POINT('Ctrl Pts',(37.2007589068722,-3.85625898977929,0.7731465603276));
#85247=CARTESIAN_POINT('Ctrl Pts',(37.1941856985404,-3.83075501185786,0.900353934946174));
#85248=CARTESIAN_POINT('Ctrl Pts',(37.1876124902087,-3.79898711375405,1.02612555331995));
#85249=CARTESIAN_POINT('Ctrl Pts',(37.181039281877,-3.76115085212069,1.14988402353968));
#85250=CARTESIAN_POINT('Ctrl Pts',(37.1744660735452,-3.72331459048733,1.27364249375941));
#85251=CARTESIAN_POINT('Ctrl Pts',(37.1678928652135,-3.67941012507819,1.39538760983665));
#85252=CARTESIAN_POINT('Ctrl Pts',(37.1613196568818,-3.62968041094891,1.51456565205135));
#85253=CARTESIAN_POINT('Ctrl Pts',(37.1554472107479,-3.58525232458046,1.62103825993672));
#85254=CARTESIAN_POINT('Ctrl Pts',(37.149574764614,-3.536061001913,1.72573259710872));
#85255=CARTESIAN_POINT('Ctrl Pts',(37.14370231848,-3.4822698392381,1.82819193924835));
#85256=CARTESIAN_POINT('Ctrl Pts',(37.1378374795352,-3.42854835784009,1.93051855516616));
#85257=CARTESIAN_POINT('Ctrl Pts',(37.1319726405903,-3.37023907644195,2.03061557100527));
#85258=CARTESIAN_POINT('Ctrl Pts',(37.1261078016455,-3.30755372806207,2.12804542620281));
#85259=CARTESIAN_POINT('Ctrl Pts',(37.1202489915254,-3.24493281776612,2.22537512732371));
#85260=CARTESIAN_POINT('Ctrl Pts',(37.1143901814054,-3.17794501041741,2.32004277573182));
#85261=CARTESIAN_POINT('Ctrl Pts',(37.1085313712854,-3.1068479813703,2.41163525862749));
#85262=CARTESIAN_POINT('Ctrl Pts',(37.1024455824044,-3.03299655079306,2.5067761665195));
#85263=CARTESIAN_POINT('Ctrl Pts',(37.0963597935234,-2.95471127585929,2.59859841486491));
#85264=CARTESIAN_POINT('Ctrl Pts',(37.0902740046425,-2.87233079815463,2.68667169300091));
#85265=CARTESIAN_POINT('Ctrl Pts',(37.0844219745642,-2.79311460403095,2.7713620236754));
#85266=CARTESIAN_POINT('Ctrl Pts',(37.0785699444859,-2.71011231082609,2.85258574219773));
#85267=CARTESIAN_POINT('Ctrl Pts',(37.0727179144076,-2.62366559043396,2.92999451698681));
#85268=CARTESIAN_POINT('Ctrl Pts',(37.0668667740291,-2.5372320127675,3.00739152311324));
#85269=CARTESIAN_POINT('Ctrl Pts',(37.0610156336506,-2.44735535698887,3.08097446305657));
#85270=CARTESIAN_POINT('Ctrl Pts',(37.0551644932721,-2.35441262768268,3.15043333187807));
#85271=CARTESIAN_POINT('Ctrl Pts',(37.0493128257046,-2.26146152421694,3.21989845895832));
#85272=CARTESIAN_POINT('Ctrl Pts',(37.043461158137,-2.16544412918584,3.28523852878785));
#85273=CARTESIAN_POINT('Ctrl Pts',(37.0376094905695,-2.06676827094617,3.34618557677398));
#85274=CARTESIAN_POINT('Ctrl Pts',(37.0317558788853,-1.96805962933559,3.4071528733773));
#85275=CARTESIAN_POINT('Ctrl Pts',(37.025902267201,-1.86669111976615,3.46372402889574));
#85276=CARTESIAN_POINT('Ctrl Pts',(37.0200486555168,-1.7630964886576,3.51567628937638));
#85277=CARTESIAN_POINT('Ctrl Pts',(37.0141883894169,-1.6593840906435,3.56768760945197));
#85278=CARTESIAN_POINT('Ctrl Pts',(37.008328123317,-1.55344088967951,3.61506936869121));
#85279=CARTESIAN_POINT('Ctrl Pts',(37.0024678572171,-1.44572208530969,3.65764632681289));
#85280=CARTESIAN_POINT('Ctrl Pts',(36.9966036440458,-1.33793072897609,3.70025196183959));
#85281=CARTESIAN_POINT('Ctrl Pts',(36.9907394308744,-1.22836177771908,3.73804621739922));
#85282=CARTESIAN_POINT('Ctrl Pts',(36.9848752177031,-1.11748544447807,3.77090377514193));
#85283=CARTESIAN_POINT('Ctrl Pts',(36.9790023691288,-1.00644583923602,3.80380971759439));
#85284=CARTESIAN_POINT('Ctrl Pts',(36.9731295205545,-0.894095409315755,
3.83176435416209));
#85285=CARTESIAN_POINT('Ctrl Pts',(36.9672566719802,-0.780914477028074,
3.85469344819636));
#85286=CARTESIAN_POINT('Ctrl Pts',(36.9656619273675,-0.75018072325557,3.86091973663587));
#85287=CARTESIAN_POINT('Ctrl Pts',(36.9640671827548,-0.719385756813729,
3.86677575314457));
#85288=CARTESIAN_POINT('Ctrl Pts',(36.9624724381421,-0.688539235687553,
3.87226067316223));
#85289=CARTESIAN_POINT('Ctrl Pts',(36.9565999920082,-0.574950807615644,
3.89245820014941));
#85290=CARTESIAN_POINT('Ctrl Pts',(36.9507275458743,-0.460282746080942,
3.90768732111895));
#85291=CARTESIAN_POINT('Ctrl Pts',(36.9448550997404,-0.345007601699793,
3.91783853097207));
#85292=CARTESIAN_POINT('Ctrl Pts',(36.9389902607955,-0.229881785179329,
3.92797659090931));
#85293=CARTESIAN_POINT('Ctrl Pts',(36.9331254218507,-0.114150857684523,
3.93304978499831));
#85294=CARTESIAN_POINT('Ctrl Pts',(36.9272605829058,0.00170261472762606,
3.93299963146491));
#85295=CARTESIAN_POINT('Ctrl Pts',(36.9214017727858,0.117436994305847,3.93294952948738));
#85296=CARTESIAN_POINT('Ctrl Pts',(36.9155429626657,0.233293257362139,3.92778655562286));
#85297=CARTESIAN_POINT('Ctrl Pts',(36.9096841525457,0.348784562024424,3.91750409435567));
#85298=CARTESIAN_POINT('Ctrl Pts',(36.9035983636647,0.468750166535014,3.90682327569679));
#85299=CARTESIAN_POINT('Ctrl Pts',(36.8975125747838,0.58832151009465,3.89061823444403));
#85300=CARTESIAN_POINT('Ctrl Pts',(36.8914267859028,0.70695350456514,3.86894116553652));
#85301=CARTESIAN_POINT('Ctrl Pts',(36.8855747558245,0.821028772942941,3.84809672585305));
#85302=CARTESIAN_POINT('Ctrl Pts',(36.8797227257462,0.934235078816343,3.82219295318668));
#85303=CARTESIAN_POINT('Ctrl Pts',(36.873870695668,1.04609465706276,3.79132891852774));
#85304=CARTESIAN_POINT('Ctrl Pts',(36.8680195552894,1.15793722899886,3.76046957621039));
#85305=CARTESIAN_POINT('Ctrl Pts',(36.8621684149109,1.26843308205228,3.72465158125484));
#85306=CARTESIAN_POINT('Ctrl Pts',(36.8563172745324,1.377117587066,3.68402445043373));
#85307=CARTESIAN_POINT('Ctrl Pts',(36.8504656069649,1.48581188457658,3.64339365909954));
#85308=CARTESIAN_POINT('Ctrl Pts',(36.8446139393974,1.5926941224023,3.59795301527448));
#85309=CARTESIAN_POINT('Ctrl Pts',(36.8387622718299,1.69731836937081,3.54790069660869));
#85310=CARTESIAN_POINT('Ctrl Pts',(36.8329086601456,1.80197737596095,3.49783174891369));
#85311=CARTESIAN_POINT('Ctrl Pts',(36.8270550484614,1.90437652732299,3.44314825808369));
#85312=CARTESIAN_POINT('Ctrl Pts',(36.8212014367771,2.00409390971568,3.3840946501303));
#85313=CARTESIAN_POINT('Ctrl Pts',(36.8153411706772,2.10392465133778,3.32497390973388));
#85314=CARTESIAN_POINT('Ctrl Pts',(36.8094809045773,2.20106718311247,3.26147334706311));
#85315=CARTESIAN_POINT('Ctrl Pts',(36.8036206384774,2.29512796029872,3.19388112581778));
#85316=CARTESIAN_POINT('Ctrl Pts',(36.7977564253061,2.38925209034279,3.12624337910996));
#85317=CARTESIAN_POINT('Ctrl Pts',(36.7918922121348,2.48029000886613,3.05450874156429));
#85318=CARTESIAN_POINT('Ctrl Pts',(36.7860279989635,2.56788204800477,2.97900499958204));
#85319=CARTESIAN_POINT('Ctrl Pts',(36.7801551503892,2.65560307163525,2.90339007384512));
#85320=CARTESIAN_POINT('Ctrl Pts',(36.7742823018149,2.73986778894419,2.8239952489147));
#85321=CARTESIAN_POINT('Ctrl Pts',(36.7684094532406,2.82035403620938,2.74118443568422));
#85322=CARTESIAN_POINT('Ctrl Pts',(36.7668147086279,2.84220970090093,2.71869754595714));
#85323=CARTESIAN_POINT('Ctrl Pts',(36.7652199640151,2.86378698786068,2.69595895376266));
#85324=CARTESIAN_POINT('Ctrl Pts',(36.7636252194024,2.88507998128988,2.67297633763571));
#85325=CARTESIAN_POINT('Ctrl Pts',(36.7577527732685,2.96348874714819,2.58834574904788));
#85326=CARTESIAN_POINT('Ctrl Pts',(36.7518803271346,3.03830181444336,2.50012049516091));
#85327=CARTESIAN_POINT('Ctrl Pts',(36.7460078810007,3.10917155355338,2.4086388792375));
#85328=CARTESIAN_POINT('Ctrl Pts',(36.7401430420559,3.17994948773362,2.31727576894753));
#85329=CARTESIAN_POINT('Ctrl Pts',(36.7342782031111,3.24679400131313,2.22266500908758));
#85330=CARTESIAN_POINT('Ctrl Pts',(36.7284133641662,3.30939497049408,2.12518091683237));
#85331=CARTESIAN_POINT('Ctrl Pts',(36.7225545540462,3.37193158832961,2.02779703440739));
#85332=CARTESIAN_POINT('Ctrl Pts',(36.7166957439262,3.43023311640159,1.92754604033316));
#85333=CARTESIAN_POINT('Ctrl Pts',(36.7108369338062,3.48403074929415,1.82483389325517));
#85334=CARTESIAN_POINT('Ctrl Pts',(36.7047511449252,3.53991258013931,1.71814252933926));
#85335=CARTESIAN_POINT('Ctrl Pts',(36.6986653560443,3.59093420476172,1.60879581752963));
#85336=CARTESIAN_POINT('Ctrl Pts',(36.6925795671633,3.63684479527185,1.49728051316513));
#85337=CARTESIAN_POINT('Ctrl Pts',(36.686727537085,3.68099193245167,1.39004857855646));
#85338=CARTESIAN_POINT('Ctrl Pts',(36.6808755070068,3.7204132567031,1.28081198980515));
#85339=CARTESIAN_POINT('Ctrl Pts',(36.6750234769285,3.75493377493265,1.17002621589008));
#85340=CARTESIAN_POINT('Ctrl Pts',(36.66917233655,3.78944904491566,1.05925728503194));
#85341=CARTESIAN_POINT('Ctrl Pts',(36.6633211961715,3.81906486740816,0.946940031848625));
#85342=CARTESIAN_POINT('Ctrl Pts',(36.657470055793,3.84365578750946,0.83354615177868));
#85343=CARTESIAN_POINT('Ctrl Pts',(36.6516183882256,3.86824892325786,0.720142054896152));
#85344=CARTESIAN_POINT('Ctrl Pts',(36.6457667206581,3.88781616898965,0.605661542282593));
#85345=CARTESIAN_POINT('Ctrl Pts',(36.6399150530906,3.90228311395982,0.490586891899909));
#85346=CARTESIAN_POINT('Ctrl Pts',(36.6340614414064,3.91675486532571,0.375474009927441));
#85347=CARTESIAN_POINT('Ctrl Pts',(36.6282078297221,3.92612289501087,0.25976700759516));
#85348=CARTESIAN_POINT('Ctrl Pts',(36.6223542180379,3.93036468327514,0.143952966150416));
#85349=CARTESIAN_POINT('Ctrl Pts',(36.616493951938,3.93461129362597,0.0280072667119841));
#85350=CARTESIAN_POINT('Ctrl Pts',(36.6106336858382,3.93372001584771,-0.0880453013893719));
#85351=CARTESIAN_POINT('Ctrl Pts',(36.6047734197383,3.92772046214228,-0.203717871746349));
#85352=CARTESIAN_POINT('Ctrl Pts',(36.598909206567,3.9217168675509,-0.31946835117574));
#85353=CARTESIAN_POINT('Ctrl Pts',(36.5930449933957,3.9105981856969,-0.43483791278791));
#85354=CARTESIAN_POINT('Ctrl Pts',(36.5871807802244,3.89444567732624,-0.549346763306142));
#85355=CARTESIAN_POINT('Ctrl Pts',(36.5813079316501,3.87826938342547,-0.664024234923348));
#85356=CARTESIAN_POINT('Ctrl Pts',(36.5754350830758,3.85704454441074,-0.777838061049976));
#85357=CARTESIAN_POINT('Ctrl Pts',(36.5695622345016,3.83090308814628,-0.890320464344874));
#85358=CARTESIAN_POINT('Ctrl Pts',(36.5679674898887,3.8238044977393,-0.920864535834475));
#85359=CARTESIAN_POINT('Ctrl Pts',(36.5663727452758,3.81634365128301,-0.95131053159593));
#85360=CARTESIAN_POINT('Ctrl Pts',(36.5647780006629,3.80852380929646,-0.981649323344114));
#85361=CARTESIAN_POINT('Ctrl Pts',(36.558905554529,3.77972822631074,-1.09336810193003));
#85362=CARTESIAN_POINT('Ctrl Pts',(36.553033108395,3.74596454780185,-1.20400581916583));
#85363=CARTESIAN_POINT('Ctrl Pts',(36.5471606622611,3.70732939059398,-1.31308712187657));
#85364=CARTESIAN_POINT('Ctrl Pts',(36.5412958233163,3.66874428151579,-1.42202712025262));
#85365=CARTESIAN_POINT('Ctrl Pts',(36.5354309843714,3.62530037987541,-1.52941432753211));
#85366=CARTESIAN_POINT('Ctrl Pts',(36.5295661454266,3.57714487750403,-1.63478546768274));
#85367=CARTESIAN_POINT('Ctrl Pts',(36.5237073353066,3.52903887710375,-1.74004829042668));
#85368=CARTESIAN_POINT('Ctrl Pts',(36.5178485251865,3.47623108042718,-1.84329879453504));
#85369=CARTESIAN_POINT('Ctrl Pts',(36.5119897150665,3.41891763766497,-1.94409135249952));
#85370=CARTESIAN_POINT('Ctrl Pts',(36.5059039261855,3.35938378940106,-2.04878875964854));
#85371=CARTESIAN_POINT('Ctrl Pts',(36.4998181373046,3.29498827554955,-2.15083349179325));
#85372=CARTESIAN_POINT('Ctrl Pts',(36.4937323484236,3.22600493383233,-2.24975135668133));
#85373=CARTESIAN_POINT('Ctrl Pts',(36.4878803183453,3.15967128366404,-2.34486972702322));
#85374=CARTESIAN_POINT('Ctrl Pts',(36.482028288267,3.08909600512226,-2.4370966384242));
#85375=CARTESIAN_POINT('Ctrl Pts',(36.4761762581888,3.01456762221467,-2.52603860839359));
#85376=CARTESIAN_POINT('Ctrl Pts',(36.4703251178103,2.94005057005607,-2.61496705627786));
#85377=CARTESIAN_POINT('Ctrl Pts',(36.4644739774317,2.86158187393101,-2.70061123899355));
#85378=CARTESIAN_POINT('Ctrl Pts',(36.4586228370532,2.77949049349779,-2.78261057220651));
#85379=CARTESIAN_POINT('Ctrl Pts',(36.4527711694857,2.69739171661382,-2.86461729357673));
#85380=CARTESIAN_POINT('Ctrl Pts',(36.4469195019182,2.61166989902848,-2.94297822047091));
#85381=CARTESIAN_POINT('Ctrl Pts',(36.4410678343507,2.5226905026107,-3.01736998527489));
#85382=CARTESIAN_POINT('Ctrl Pts',(36.4352142226665,2.43368154430616,-3.09178646547384));
#85383=CARTESIAN_POINT('Ctrl Pts',(36.4293606109823,2.34141317208805,-3.16223089646156));
#85384=CARTESIAN_POINT('Ctrl Pts',(36.423506999298,2.24628294638947,-3.2284209646141));
#85385=CARTESIAN_POINT('Ctrl Pts',(36.4176467331981,2.15104457616456,-3.2946862779741));
#85386=CARTESIAN_POINT('Ctrl Pts',(36.4117864670982,2.05293819834845,-3.35668733902035));
#85387=CARTESIAN_POINT('Ctrl Pts',(36.4059262009983,1.95238938092377,-3.41418580414952));
#85388=CARTESIAN_POINT('Ctrl Pts',(36.400061987827,1.85177284074446,-3.47172299628259));
#85389=CARTESIAN_POINT('Ctrl Pts',(36.3941977746557,1.74871095197124,-3.52475136524969));
#85390=CARTESIAN_POINT('Ctrl Pts',(36.3883335614844,1.64365125950279,-3.57307983917725));
#85391=CARTESIAN_POINT('Ctrl Pts',(36.3824607129101,1.53843686038308,-3.6214794796596));
#85392=CARTESIAN_POINT('Ctrl Pts',(36.3765878643359,1.43121916751251,-3.66516525702887));
#85393=CARTESIAN_POINT('Ctrl Pts',(36.3707150157616,1.32246301410729,-3.70399521818242));
#85394=CARTESIAN_POINT('Ctrl Pts',(36.3691202711488,1.29293078838095,-3.71453931285502));
#85395=CARTESIAN_POINT('Ctrl Pts',(36.367525526536,1.26328518927632,-3.72472564395935));
#85396=CARTESIAN_POINT('Ctrl Pts',(36.3659307819232,1.23353565858427,-3.73455201851588));
#85397=CARTESIAN_POINT('Ctrl Pts',(36.3600583357892,1.12398675959701,-3.77073640491336));
#85398=CARTESIAN_POINT('Ctrl Pts',(36.3541858896553,1.01266095893547,-3.80215704412923));
#85399=CARTESIAN_POINT('Ctrl Pts',(36.3483134435214,0.900010369633905,-3.82863818276831));
#85400=CARTESIAN_POINT('Ctrl Pts',(36.3424486045765,0.78750570833446,-3.85508501763962));
#85401=CARTESIAN_POINT('Ctrl Pts',(36.3365837656316,0.673680069858687,-3.8766049828504));
#85402=CARTESIAN_POINT('Ctrl Pts',(36.3307189266868,0.559002754264918,-3.8930713993869));
#85403=CARTESIAN_POINT('Ctrl Pts',(36.3248601165668,0.444443322461914,-3.90952088909186));
#85404=CARTESIAN_POINT('Ctrl Pts',(36.3190013064467,0.329034361644007,-3.92092710456594));
#85405=CARTESIAN_POINT('Ctrl Pts',(36.3131424963267,0.213256798060077,-3.92721409374141));
#85406=CARTESIAN_POINT('Ctrl Pts',(36.3070567074457,0.0929938445441312,
-3.93374464995247));
#85407=CARTESIAN_POINT('Ctrl Pts',(36.3009709185648,-0.0276664074746646,
-3.93475120119759));
#85408=CARTESIAN_POINT('Ctrl Pts',(36.2948851296838,-0.14817699638656,-3.9302077016033));
#85409=CARTESIAN_POINT('Ctrl Pts',(36.2890330996055,-0.264058701266171,
-3.92583872055473));
#85410=CARTESIAN_POINT('Ctrl Pts',(36.2831810695272,-0.37980157700227,-3.91633820245232));
#85411=CARTESIAN_POINT('Ctrl Pts',(36.277329039449,-0.49491861473092,-3.90173609625162));
#85412=CARTESIAN_POINT('Ctrl Pts',(36.2714778990704,-0.610018150909,-3.8871362100481));
#85413=CARTESIAN_POINT('Ctrl Pts',(36.2656267586919,-0.724491628305239,
-3.86743632990958));
#85414=CARTESIAN_POINT('Ctrl Pts',(36.2597756183134,-0.837857848307911,
-3.84271820799143));
#85415=CARTESIAN_POINT('Ctrl Pts',(36.2539239507459,-0.951234282630988,
-3.81799785896526));
#85416=CARTESIAN_POINT('Ctrl Pts',(36.2480722831784,-1.06350285734598,-3.78825845740157));
#85417=CARTESIAN_POINT('Ctrl Pts',(36.2422206156109,-1.17419394375876,-3.75363258490229));
#85418=CARTESIAN_POINT('Ctrl Pts',(36.2363670039266,-1.28492180539675,-3.71899520854755));
#85419=CARTESIAN_POINT('Ctrl Pts',(36.2305133922424,-1.39407074230773,-3.67946825647472));
#85420=CARTESIAN_POINT('Ctrl Pts',(36.2246597805581,-1.50118830475779,-3.63523351019689));
#85421=CARTESIAN_POINT('Ctrl Pts',(36.2187995144582,-1.60842763900001,-3.59094847763355));
#85422=CARTESIAN_POINT('Ctrl Pts',(36.2129392483583,-1.71363060725445,-3.54194512663007));
#85423=CARTESIAN_POINT('Ctrl Pts',(36.2070789822584,-1.81636660379168,-3.48845257394024));
#85424=CARTESIAN_POINT('Ctrl Pts',(36.2012147690871,-1.91917179621669,-3.43492399235306));
#85425=CARTESIAN_POINT('Ctrl Pts',(36.1953505559158,-2.01950635142536,-3.37690039487789));
#85426=CARTESIAN_POINT('Ctrl Pts',(36.1894863427445,-2.11696754594518,-3.31465494575451));
#85427=CARTESIAN_POINT('Ctrl Pts',(36.1836134941702,-2.21457225787572,-3.25231783650188));
#85428=CARTESIAN_POINT('Ctrl Pts',(36.1777406455959,-2.30929482757873,-3.1857467046369));
#85429=CARTESIAN_POINT('Ctrl Pts',(36.1718677970216,-2.40076450275936,-3.11525581650859));
#85430=CARTESIAN_POINT('Ctrl Pts',(36.1702730524089,-2.42560266602413,-3.09611434492741));
#85431=CARTESIAN_POINT('Ctrl Pts',(36.1686783077962,-2.45020117753265,-3.07668405622527));
#85432=CARTESIAN_POINT('Ctrl Pts',(36.1670835631835,-2.47455308725801,-3.0569717071543));
#85433=CARTESIAN_POINT('Ctrl Pts',(36.1612882209238,-2.5630485431541,-2.9853365320287));
#85434=CARTESIAN_POINT('Ctrl Pts',(36.155492878664,-2.64859779005247,-2.90971999295362));
#85435=CARTESIAN_POINT('Ctrl Pts',(36.1496975364043,-2.73081386313657,-2.83039655258784));
#85436=CARTESIAN_POINT('Ctrl Pts',(36.1439097363987,-2.81292293744588,-2.75117634642691));
#85437=CARTESIAN_POINT('Ctrl Pts',(36.1381219363931,-2.89170715676281,-2.66825911971025));
#85438=CARTESIAN_POINT('Ctrl Pts',(36.1323341363876,-2.96681105847508,-2.58196071684098));
#85439=CARTESIAN_POINT('Ctrl Pts',(36.1264020274562,-3.04378754793543,-2.49351061042225));
#85440=CARTESIAN_POINT('Ctrl Pts',(36.1204699185248,-3.1168973971269,-2.40150874837553));
#85441=CARTESIAN_POINT('Ctrl Pts',(36.1145378095935,-3.18579619034485,-2.30633727663243));
#85442=CARTESIAN_POINT('Ctrl Pts',(36.1087601655715,-3.25290094269537,-2.21364395438578));
#85443=CARTESIAN_POINT('Ctrl Pts',(36.1029825215496,-3.31601096819452,-2.1179444200756));
#85444=CARTESIAN_POINT('Ctrl Pts',(36.0972048775276,-3.37484808622337,-2.0196260532372));
#85445=CARTESIAN_POINT('Ctrl Pts',(36.0914293147106,-3.43366401012889,-1.92134310233455));
#85446=CARTESIAN_POINT('Ctrl Pts',(36.0856537518936,-3.48820986723053,-1.82044355797122));
#85447=CARTESIAN_POINT('Ctrl Pts',(36.0798781890765,-3.53825118769959,-1.71734316103173));
#85448=CARTESIAN_POINT('Ctrl Pts',(36.0741032215919,-3.58828735001918,-1.61425339145483));
#85449=CARTESIAN_POINT('Ctrl Pts',(36.0683282541072,-3.63381971388977,-1.508963603127));
#85450=CARTESIAN_POINT('Ctrl Pts',(36.0625532866225,-3.67466050355064,-1.40191268759684));
#85451=CARTESIAN_POINT('Ctrl Pts',(36.0565041395735,-3.71744030151651,-1.28977928918629));
#85452=CARTESIAN_POINT('Ctrl Pts',(36.0504549925246,-3.75507186446882,-1.17571388591425));
#85453=CARTESIAN_POINT('Ctrl Pts',(36.0444058454756,-3.78739718369451,-1.06024128053141));
#85454=CARTESIAN_POINT('Ctrl Pts',(36.0386247027133,-3.81829034660931,-0.949884628354775));
#85455=CARTESIAN_POINT('Ctrl Pts',(36.0328435599511,-3.84433734512878,-0.838243238474594));
#85456=CARTESIAN_POINT('Ctrl Pts',(36.0270624171888,-3.8654524764882,-0.725786574697586));
#85457=CARTESIAN_POINT('Ctrl Pts',(36.0212780528597,-3.88657937434611,-0.613267243957136));
#85458=CARTESIAN_POINT('Ctrl Pts',(36.0154936885306,-3.90276887576901,-0.499932155174765));
#85459=CARTESIAN_POINT('Ctrl Pts',(36.0097093242014,-3.91398711034839,-0.38625626211963));
#85460=CARTESIAN_POINT('Ctrl Pts',(36.0039176492429,-3.9252195232109,-0.272436698597958));
#85461=CARTESIAN_POINT('Ctrl Pts',(35.9981259742844,-3.93146811458794,-0.158275894357944));
#85462=CARTESIAN_POINT('Ctrl Pts',(35.992334299326,-3.93275107682362,-0.0442489292822916));
#85463=CARTESIAN_POINT('Ctrl Pts',(35.9915440402289,-3.93292613370875,-0.0286902442554935));
#85464=CARTESIAN_POINT('Ctrl Pts',(35.9907537811319,-3.93300881996226,-0.0131340427485895));
#85465=CARTESIAN_POINT('Ctrl Pts',(35.9899635220349,-3.93299925641567,0.00241847757537678));
#85466=CARTESIAN_POINT('',(34.739963522035,-3.93332081374984,-0.00333872239636136));
#85467=CARTESIAN_POINT('Ctrl Pts',(35.9899635220349,-3.93762631029128,0.0024213228406085));
#85468=CARTESIAN_POINT('Ctrl Pts',(35.9827211295046,-3.9386567952212,0.145122008460187));
#85469=CARTESIAN_POINT('Ctrl Pts',(35.9091963307278,-3.86675733052379,1.59277050702035));
#85470=CARTESIAN_POINT('Ctrl Pts',(35.7693891257042,-2.07371529249546,4.1638557740525));
#85471=CARTESIAN_POINT('Ctrl Pts',(35.5705419069645,2.38139350245334,3.99586724101343));
#85472=CARTESIAN_POINT('Ctrl Pts',(35.371694688225,4.6490029931939,0.157356889391723));
#85473=CARTESIAN_POINT('Ctrl Pts',(35.1728474694854,2.64613353856358,-3.82569827841376));
#85474=CARTESIAN_POINT('Ctrl Pts',(34.9740002507456,-1.78741999599338,-4.29454535187287));
#85475=CARTESIAN_POINT('Ctrl Pts',(34.8297056015956,-3.81320887697328,-1.77214066905022));
#85476=CARTESIAN_POINT('Ctrl Pts',(34.751693358692,-3.93732144507338,-0.234826367187542));
#85477=CARTESIAN_POINT('Ctrl Pts',(34.739963522035,-3.93522822798615,-0.00334034146760698));
#85478=CARTESIAN_POINT('',(33.4899635468833,-3.93061375975798,-0.000796215185199833));
#85479=CARTESIAN_POINT('Ctrl Pts',(34.739963522035,-3.93299858311176,-0.00333844887719042));
#85480=CARTESIAN_POINT('Ctrl Pts',(34.7341874476538,-3.93309528539993,0.110585704628955));
#85481=CARTESIAN_POINT('Ctrl Pts',(34.7284113732727,-3.92823788115257,0.224683591804017));
#85482=CARTESIAN_POINT('Ctrl Pts',(34.7226352988915,-3.91840775789089,0.338481377479638));
#85483=CARTESIAN_POINT('Ctrl Pts',(34.7168647659296,-3.90858706540015,0.452169988445717));
#85484=CARTESIAN_POINT('Ctrl Pts',(34.7110942329677,-3.89380317397632,0.565558647516841));
#85485=CARTESIAN_POINT('Ctrl Pts',(34.7053237000058,-3.87408952563053,0.678173537820377));
#85486=CARTESIAN_POINT('Ctrl Pts',(34.6995567654491,-3.85438817037686,0.790718203414797));
#85487=CARTESIAN_POINT('Ctrl Pts',(34.6937898308923,-3.82976324162912,0.902489640128141));
#85488=CARTESIAN_POINT('Ctrl Pts',(34.6880228963355,-3.8002999313102,1.0130199564094));
#85489=CARTESIAN_POINT('Ctrl Pts',(34.6822577349691,-3.77084568023356,1.12351628734061));
#85490=CARTESIAN_POINT('Ctrl Pts',(34.6764925736027,-3.73655611310215,1.23277184402113));
#85491=CARTESIAN_POINT('Ctrl Pts',(34.6707274122363,-3.69756718542943,1.34033052238448));
#85492=CARTESIAN_POINT('Ctrl Pts',(34.6649625312168,-3.65858015370136,1.44788397040904));
#85493=CARTESIAN_POINT('Ctrl Pts',(34.6591976501973,-3.6148943615961,1.55374030305034));
#85494=CARTESIAN_POINT('Ctrl Pts',(34.6534327691778,-3.56669483819284,1.65746098934742));
#85495=CARTESIAN_POINT('Ctrl Pts',(34.6476666761293,-3.51848518115074,1.76120348224966));
#85496=CARTESIAN_POINT('Ctrl Pts',(34.6419005830808,-3.4657600879619,1.86280905011959));
#85497=CARTESIAN_POINT('Ctrl Pts',(34.6361344900323,-3.40875129601817,1.96186227903348));
#85498=CARTESIAN_POINT('Ctrl Pts',(34.6303623658268,-3.3516828746216,2.06101911459542));
#85499=CARTESIAN_POINT('Ctrl Pts',(34.6245902416213,-3.29032202516318,2.15761791282369));
#85500=CARTESIAN_POINT('Ctrl Pts',(34.6188181174158,-3.22494467578866,2.25127093840399));
#85501=CARTESIAN_POINT('Ctrl Pts',(34.6130425610421,-3.15952845232737,2.3449796510973));
#85502=CARTESIAN_POINT('Ctrl Pts',(34.6072670046685,-3.09009123587556,2.43573876783277));
#85503=CARTESIAN_POINT('Ctrl Pts',(34.6014914482948,-3.01694901452852,2.52319393700432));
#85504=CARTESIAN_POINT('Ctrl Pts',(34.5957072109202,-2.94369685612108,2.61078055643865));
#85505=CARTESIAN_POINT('Ctrl Pts',(34.5899229735457,-2.86672886659721,2.69505300422099));
#85506=CARTESIAN_POINT('Ctrl Pts',(34.5841387361711,-2.7863975975899,2.77569404440497));
#85507=CARTESIAN_POINT('Ctrl Pts',(34.5815277618695,-2.75013648563879,2.81209498543454));
#85508=CARTESIAN_POINT('Ctrl Pts',(34.5789167875679,-2.71319052644958,2.84775655000578));
#85509=CARTESIAN_POINT('Ctrl Pts',(34.5763058132664,-2.6755942070439,2.88265236184197));
#85510=CARTESIAN_POINT('Ctrl Pts',(34.5704333671324,-2.59103482995219,2.96113791996639));
#85511=CARTESIAN_POINT('Ctrl Pts',(34.5645609209985,-2.50287752499796,3.0360310441156));
#85512=CARTESIAN_POINT('Ctrl Pts',(34.5586884748646,-2.41146027973897,3.10698379771142));
#85513=CARTESIAN_POINT('Ctrl Pts',(34.5528236359197,-2.32016145672751,3.17784463884011));
#85514=CARTESIAN_POINT('Ctrl Pts',(34.5469587969749,-2.22561141486791,3.2447750090869));
#85515=CARTESIAN_POINT('Ctrl Pts',(34.5410939580301,-2.12818418966159,3.30746444499022));
#85516=CARTESIAN_POINT('Ctrl Pts',(34.53523514791,-2.03085711582818,3.37008943860792));
#85517=CARTESIAN_POINT('Ctrl Pts',(34.52937633779,-1.93065908706628,3.42848194686668));
#85518=CARTESIAN_POINT('Ctrl Pts',(34.52351752767,-1.82799581784233,3.48237279594689));
#85519=CARTESIAN_POINT('Ctrl Pts',(34.517431738789,-1.72135522537966,3.53835145430905));
#85520=CARTESIAN_POINT('Ctrl Pts',(34.511345949908,-1.61205487419881,3.58947231887924));
#85521=CARTESIAN_POINT('Ctrl Pts',(34.5052601610271,-1.50058129174565,3.63548412001249));
#85522=CARTESIAN_POINT('Ctrl Pts',(34.4994081309488,-1.39338947648432,3.67972858025478));
#85523=CARTESIAN_POINT('Ctrl Pts',(34.4935561008705,-1.28418871798513,3.71924904926795));
#85524=CARTESIAN_POINT('Ctrl Pts',(34.4877040707923,-1.17343432618692,3.7538701205724));
#85525=CARTESIAN_POINT('Ctrl Pts',(34.4818529304137,-1.06269677267447,3.78848592834298));
#85526=CARTESIAN_POINT('Ctrl Pts',(34.4760017900352,-0.950406449934469,
3.81820369615239));
#85527=CARTESIAN_POINT('Ctrl Pts',(34.4701506496567,-0.837034939327708,
3.84289754096367));
#85528=CARTESIAN_POINT('Ctrl Pts',(34.4642989820892,-0.723653213923857,
3.8675936106956));
#85529=CARTESIAN_POINT('Ctrl Pts',(34.4584473145217,-0.609190510912237,
3.88726476961269));
#85530=CARTESIAN_POINT('Ctrl Pts',(34.4525956469542,-0.494129040508674,
3.90183616920623));
#85531=CARTESIAN_POINT('Ctrl Pts',(34.44674203527,-0.379029342894668,3.91641240989868));
#85532=CARTESIAN_POINT('Ctrl Pts',(34.4408884235858,-0.263330892192644,
3.9258854703341));
#85533=CARTESIAN_POINT('Ctrl Pts',(34.4350348119016,-0.147520749006666,
3.93023238862698));
#85534=CARTESIAN_POINT('Ctrl Pts',(34.4291745458017,-0.0315789522580382,
3.93458424851878));
#85535=CARTESIAN_POINT('Ctrl Pts',(34.4233142797018,0.0844743770975343,
3.93379831940984));
#85536=CARTESIAN_POINT('Ctrl Pts',(34.4174540136019,0.200152345972468,3.92790377153027));
#85537=CARTESIAN_POINT('Ctrl Pts',(34.4115898004306,0.315908227555552,3.92200525348945));
#85538=CARTESIAN_POINT('Ctrl Pts',(34.4057255872593,0.431287834768613,3.91099130451018));
#85539=CARTESIAN_POINT('Ctrl Pts',(34.399861374088,0.545811300767073,3.89494274976603));
#85540=CARTESIAN_POINT('Ctrl Pts',(34.3939885255137,0.660503409386893,3.87887056256963));
#85541=CARTESIAN_POINT('Ctrl Pts',(34.3881156769395,0.774336455757687,3.85774904835337));
#85542=CARTESIAN_POINT('Ctrl Pts',(34.3822428283652,0.886842542971706,3.83170971029585));
#85543=CARTESIAN_POINT('Ctrl Pts',(34.3806480837524,0.917393045717129,3.82463884961164));
#85544=CARTESIAN_POINT('Ctrl Pts',(34.3790533391396,0.947845801617697,3.81720564399785));
#85545=CARTESIAN_POINT('Ctrl Pts',(34.3774585945268,0.978191679432268,3.80941334568585));
#85546=CARTESIAN_POINT('Ctrl Pts',(34.3715861483928,1.08993655157172,3.78071918881001));
#85547=CARTESIAN_POINT('Ctrl Pts',(34.3657137022589,1.20060487266298,3.74705595710973));
#85548=CARTESIAN_POINT('Ctrl Pts',(34.359841256125,1.30972120202169,3.70851983586105));
#85549=CARTESIAN_POINT('Ctrl Pts',(34.3539764171801,1.41869618167212,3.67003363445047));
#85550=CARTESIAN_POINT('Ctrl Pts',(34.3481115782352,1.52612278150101,3.62668723291229));
#85551=CARTESIAN_POINT('Ctrl Pts',(34.3422467392904,1.63153759205154,3.57862740247188));
#85552=CARTESIAN_POINT('Ctrl Pts',(34.3363879291703,1.73684404030358,3.53061697565574));
#85553=CARTESIAN_POINT('Ctrl Pts',(34.3305291190503,1.84014243886888,3.47790292779082));
#85554=CARTESIAN_POINT('Ctrl Pts',(34.3246703089303,1.94098698236471,3.42068100446252));
#85555=CARTESIAN_POINT('Ctrl Pts',(34.3185845200493,2.04573838903953,3.36124222122756));
#85556=CARTESIAN_POINT('Ctrl Pts',(34.3124987311684,2.14784153504624,3.29693936640616));
#85557=CARTESIAN_POINT('Ctrl Pts',(34.3064129422874,2.24682197974801,3.22804584715292));
#85558=CARTESIAN_POINT('Ctrl Pts',(34.3005609122091,2.34200052617568,3.16179856931368));
#85559=CARTESIAN_POINT('Ctrl Pts',(34.2947088821308,2.43429146524979,3.09130704008724));
#85560=CARTESIAN_POINT('Ctrl Pts',(34.2888568520526,2.52330105273017,3.01685942617332));
#85561=CARTESIAN_POINT('Ctrl Pts',(34.283005711674,2.61229710784553,2.94242313072873));
#85562=CARTESIAN_POINT('Ctrl Pts',(34.2771545712955,2.6980124863042,2.86403221160928));
#85563=CARTESIAN_POINT('Ctrl Pts',(34.2713034309169,2.78008630530296,2.78201530101237));
#85564=CARTESIAN_POINT('Ctrl Pts',(34.2654517633494,2.86216751916993,2.6999910006747));
#85565=CARTESIAN_POINT('Ctrl Pts',(34.2596000957819,2.94060622892761,2.61434035160873));
#85566=CARTESIAN_POINT('Ctrl Pts',(34.2537484282144,3.0150787353421,2.52542852199145));
#85567=CARTESIAN_POINT('Ctrl Pts',(34.2478948165302,3.08957598397633,2.43648715293561));
#85568=CARTESIAN_POINT('Ctrl Pts',(34.242041204846,3.16010414381335,2.34428276562728));
#85569=CARTESIAN_POINT('Ctrl Pts',(34.2361875931617,3.22638054045464,2.24921266406171));
#85570=CARTESIAN_POINT('Ctrl Pts',(34.2303273270618,3.29273228044229,2.1540344863189));
#85571=CARTESIAN_POINT('Ctrl Pts',(34.2244670609619,3.35482237334615,2.05598443123333));
#85572=CARTESIAN_POINT('Ctrl Pts',(34.218606794862,3.41241208934595,1.95548785025261));
#85573=CARTESIAN_POINT('Ctrl Pts',(34.2127425816907,3.47004059381008,1.85492358169993));
#85574=CARTESIAN_POINT('Ctrl Pts',(34.2068783685194,3.52316249676447,1.75190987261508));
#85575=CARTESIAN_POINT('Ctrl Pts',(34.2010141553481,3.57158632014928,1.64689409426426));
#85576=CARTESIAN_POINT('Ctrl Pts',(34.1951413067738,3.6200814504965,1.54172367392868));
#85577=CARTESIAN_POINT('Ctrl Pts',(34.1892684581995,3.66386453819004,1.43454568159406));
#85578=CARTESIAN_POINT('Ctrl Pts',(34.1833956096252,3.7027932082271,1.32582482142524));
#85579=CARTESIAN_POINT('Ctrl Pts',(34.1818008650125,3.71336410683561,1.29630217941409));
#85580=CARTESIAN_POINT('Ctrl Pts',(34.1802061203997,3.72357734493953,1.26666583930661));
#85581=CARTESIAN_POINT('Ctrl Pts',(34.178611375787,3.73343072098931,1.23692524089908));
#85582=CARTESIAN_POINT('Ctrl Pts',(34.1727389296531,3.76971453698585,1.12740923391896));
#85583=CARTESIAN_POINT('Ctrl Pts',(34.1668664835192,3.80123622077032,1.01611200164018));
#85584=CARTESIAN_POINT('Ctrl Pts',(34.1609940373853,3.82781960860819,0.903485497368166));
#85585=CARTESIAN_POINT('Ctrl Pts',(34.1551291984405,3.85436856022431,0.791004889898326));
#85586=CARTESIAN_POINT('Ctrl Pts',(34.1492643594956,3.87599184334496,0.677198833363267));
#85587=CARTESIAN_POINT('Ctrl Pts',(34.1433995205508,3.89256235299504,0.562536512633344));
#85588=CARTESIAN_POINT('Ctrl Pts',(34.1375407104308,3.90911582880992,0.447992060280275));
#85589=CARTESIAN_POINT('Ctrl Pts',(34.1316819003108,3.92062680364344,0.332593501161323));
#85590=CARTESIAN_POINT('Ctrl Pts',(34.1258230901908,3.92701888889182,0.216821692380688));
#85591=CARTESIAN_POINT('Ctrl Pts',(34.1197373013099,3.93365861274941,0.0965647166165378));
#85592=CARTESIAN_POINT('Ctrl Pts',(34.1136515124289,3.93477469457016,-0.0240945719776713));
#85593=CARTESIAN_POINT('Ctrl Pts',(34.1075657235479,3.93034059197947,-0.144609235661027));
#85594=CARTESIAN_POINT('Ctrl Pts',(34.1017136934697,3.92607680592999,-0.260494858796975));
#85595=CARTESIAN_POINT('Ctrl Pts',(34.0958616633914,3.91668135891694,-0.376246311069399));
#85596=CARTESIAN_POINT('Ctrl Pts',(34.0900096333132,3.9021837577946,-0.491376556628453));
#85597=CARTESIAN_POINT('Ctrl Pts',(34.0841584929347,3.88768836078124,-0.606489298629065));
#85598=CARTESIAN_POINT('Ctrl Pts',(34.0783073525562,3.86809240362079,-0.720980611694875));
#85599=CARTESIAN_POINT('Ctrl Pts',(34.0724562121776,3.84347720162034,-0.834369223200796));
#85600=CARTESIAN_POINT('Ctrl Pts',(34.0666045446102,3.81885978178503,-0.947768051044381));
#85601=CARTESIAN_POINT('Ctrl Pts',(34.0607528770427,3.78922230580551,-1.06006357584979));
#85602=CARTESIAN_POINT('Ctrl Pts',(34.0549012094752,3.75469692891723,-1.17078604876362));
#85603=CARTESIAN_POINT('Ctrl Pts',(34.049047597791,3.72016008156113,-1.2815453073313));
#85604=CARTESIAN_POINT('Ctrl Pts',(34.0431939861067,3.68073222721102,-1.39073008040158));
#85605=CARTESIAN_POINT('Ctrl Pts',(34.0373403744225,3.63659473658771,-1.49788775341231));
#85606=CARTESIAN_POINT('Ctrl Pts',(34.0314801083226,3.5924070702399,-1.60516724381235));
#85607=CARTESIAN_POINT('Ctrl Pts',(34.0256198422227,3.54349923885702,-1.71041465218157));
#85608=CARTESIAN_POINT('Ctrl Pts',(34.0197595761228,3.4900999682102,-1.81319916498413));
#85609=CARTESIAN_POINT('Ctrl Pts',(34.0138953629515,3.43666473149438,-1.91605290635171));
#85610=CARTESIAN_POINT('Ctrl Pts',(34.0080311497802,3.37873223798797,-2.01644009193294));
#85611=CARTESIAN_POINT('Ctrl Pts',(34.0021669366089,3.31657528624049,-2.11395775045265));
#85612=CARTESIAN_POINT('Ctrl Pts',(33.9962940880347,3.25432680468145,-2.21161900952961));
#85613=CARTESIAN_POINT('Ctrl Pts',(33.9904212394604,3.18784168595066,-2.30640197105836));
#85614=CARTESIAN_POINT('Ctrl Pts',(33.9845483908861,3.11743385971219,-2.39793559761724));
#85615=CARTESIAN_POINT('Ctrl Pts',(33.9829536462732,3.09831494319716,-2.42279112658315));
#85616=CARTESIAN_POINT('Ctrl Pts',(33.9813589016604,3.07890699213294,-2.44740726606919));
#85617=CARTESIAN_POINT('Ctrl Pts',(33.9797641570475,3.05921675695992,-2.47177705991775));
#85618=CARTESIAN_POINT('Ctrl Pts',(33.9738917109136,2.98670994647429,-2.56151575570399));
#85619=CARTESIAN_POINT('Ctrl Pts',(33.9680192647797,2.91012981974181,-2.64821163018046));
#85620=CARTESIAN_POINT('Ctrl Pts',(33.9621468186458,2.82976131037675,-2.73147211706341));
#85621=CARTESIAN_POINT('Ctrl Pts',(33.9562819797009,2.74949691068483,-2.81462474799453));
#85622=CARTESIAN_POINT('Ctrl Pts',(33.9504171407561,2.66545417203359,-2.8943505465603));
#85623=CARTESIAN_POINT('Ctrl Pts',(33.9445523018113,2.57795904995689,-2.97028889785916));
#85624=CARTESIAN_POINT('Ctrl Pts',(33.9386934916913,2.49055386944009,-3.046149187506));
#85625=CARTESIAN_POINT('Ctrl Pts',(33.9328346815713,2.3997036747864,-3.11822950465146));
#85626=CARTESIAN_POINT('Ctrl Pts',(33.9269758714512,2.30577166317804,-3.18620558616125));
#85627=CARTESIAN_POINT('Ctrl Pts',(33.9208900825703,2.20820058985354,-3.25681515918901));
#85628=CARTESIAN_POINT('Ctrl Pts',(33.9148042936893,2.10730439758311,-3.32299572996346));
#85629=CARTESIAN_POINT('Ctrl Pts',(33.9087185048083,2.00352882353616,-3.38442923596577));
#85630=CARTESIAN_POINT('Ctrl Pts',(33.90286647473,1.90373933155899,-3.44350304413928));
#85631=CARTESIAN_POINT('Ctrl Pts',(33.8970144446518,1.8012879636811,-3.49818750580618));
#85632=CARTESIAN_POINT('Ctrl Pts',(33.8911624145735,1.69660037345911,-3.54824409712444));
#85633=CARTESIAN_POINT('Ctrl Pts',(33.885311274195,1.59192869917097,-3.59829307820546));
#85634=CARTESIAN_POINT('Ctrl Pts',(33.8794601338165,1.48502185134508,-3.64371540963567));
#85635=CARTESIAN_POINT('Ctrl Pts',(33.873608993438,1.37632864882293,-3.68431926554));
#85636=CARTESIAN_POINT('Ctrl Pts',(33.8677573258705,1.2676256530206,-3.72492677986021));
#85637=CARTESIAN_POINT('Ctrl Pts',(33.861905658303,1.15713636981042,-3.76071481095275));
#85638=CARTESIAN_POINT('Ctrl Pts',(33.8560539907355,1.04532741380425,-3.79154053096486));
#85639=CARTESIAN_POINT('Ctrl Pts',(33.8502003790513,0.933481311179146,-3.82237649229677));
#85640=CARTESIAN_POINT('Ctrl Pts',(33.844346767367,0.820315062227955,-3.84824675451633));
#85641=CARTESIAN_POINT('Ctrl Pts',(33.8384931556828,0.706307479360857,-3.86905915496247));
#85642=CARTESIAN_POINT('Ctrl Pts',(33.8326328895829,0.592170292091333,-3.88989521505172));
#85643=CARTESIAN_POINT('Ctrl Pts',(33.826772623483,0.477190268775185,-3.90566186267629));
#85644=CARTESIAN_POINT('Ctrl Pts',(33.8209123573831,0.361853487965521,-3.91631855870372));
#85645=CARTESIAN_POINT('Ctrl Pts',(33.8150481442118,0.246439024248364,-3.92698243234722));
#85646=CARTESIAN_POINT('Ctrl Pts',(33.8091839310405,0.130667736450913,-3.93252948152007));
#85647=CARTESIAN_POINT('Ctrl Pts',(33.8033197178692,0.0150261125709177,
-3.9329712960993));
#85648=CARTESIAN_POINT('Ctrl Pts',(33.7974468692949,-0.100785800484037,
-3.9334137612768));
#85649=CARTESIAN_POINT('Ctrl Pts',(33.7915740207206,-0.216467257082468,
-3.92873600454368));
#85650=CARTESIAN_POINT('Ctrl Pts',(33.7857011721463,-0.33153639225403,-3.91900148259875));
#85651=CARTESIAN_POINT('Ctrl Pts',(33.7841064275335,-0.362782878707366,
-3.91635811861041));
#85652=CARTESIAN_POINT('Ctrl Pts',(33.7825116829207,-0.393984272536504,
-3.91334217583988));
#85653=CARTESIAN_POINT('Ctrl Pts',(33.7809169383078,-0.425131072127442,
-3.90995557155216));
#85654=CARTESIAN_POINT('Ctrl Pts',(33.7750444921739,-0.539825237807404,
-3.89748482790048));
#85655=CARTESIAN_POINT('Ctrl Pts',(33.76917204604,-0.65416223887964,-3.87994228967359));
#85656=CARTESIAN_POINT('Ctrl Pts',(33.7632995999061,-0.767657778564146,
-3.85735538095856));
#85657=CARTESIAN_POINT('Ctrl Pts',(33.7574347609612,-0.881006295694552,
-3.83479773141105));
#85658=CARTESIAN_POINT('Ctrl Pts',(33.7515699220164,-0.993515117454448,
-3.80720878610233));
#85659=CARTESIAN_POINT('Ctrl Pts',(33.7457050830715,-1.10470464387939,-3.77466775356339));
#85660=CARTESIAN_POINT('Ctrl Pts',(33.7398462729515,-1.21577987182446,-3.74216017193186));
#85661=CARTESIAN_POINT('Ctrl Pts',(33.7339874628314,-1.32553810762419,-3.7047107438636));
#85662=CARTESIAN_POINT('Ctrl Pts',(33.7281286527114,-1.4335101938042,-3.66244966166901));
#85663=CARTESIAN_POINT('Ctrl Pts',(33.7220428638304,-1.54566527445485,-3.61855132414855));
#85664=CARTESIAN_POINT('Ctrl Pts',(33.7159570749495,-1.65589256478992,-3.56946106006242));
#85665=CARTESIAN_POINT('Ctrl Pts',(33.7098712860685,-1.76368349313182,-3.51538184783024));
#85666=CARTESIAN_POINT('Ctrl Pts',(33.7040192559902,-1.86733410723615,-3.46337985059013));
#85667=CARTESIAN_POINT('Ctrl Pts',(33.698167225912,-1.96873166748688,-3.40676529501449));
#85668=CARTESIAN_POINT('Ctrl Pts',(33.6923151958337,-2.06744537026547,-3.3457672723858));
#85669=CARTESIAN_POINT('Ctrl Pts',(33.6864640554552,-2.16614406533622,-3.28477852344936));
#85670=CARTESIAN_POINT('Ctrl Pts',(33.6806129150767,-2.2621593626964,-3.21940784976893));
#85671=CARTESIAN_POINT('Ctrl Pts',(33.6747617746981,-2.35508721576678,-3.14992907954003));
#85672=CARTESIAN_POINT('Ctrl Pts',(33.6689101071306,-2.44802344165643,-3.08044404925919));
#85673=CARTESIAN_POINT('Ctrl Pts',(33.6630584395631,-2.53787133918501,-3.00685043415877));
#85674=CARTESIAN_POINT('Ctrl Pts',(33.6572067719956,-2.62425845699118,-2.92946352612731));
#85675=CARTESIAN_POINT('Ctrl Pts',(33.6513531603114,-2.71067427544373,-2.85205090761565));
#85676=CARTESIAN_POINT('Ctrl Pts',(33.6454995486272,-2.79362672017384,-2.77084276589168));
#85677=CARTESIAN_POINT('Ctrl Pts',(33.6396459369429,-2.8727793643566,-2.68619204892854));
#85678=CARTESIAN_POINT('Ctrl Pts',(33.633785670843,-2.95202198966969,-2.60144510059783));
#85679=CARTESIAN_POINT('Ctrl Pts',(33.6279254047431,-3.02745591010843,-2.51324806784514));
#85680=CARTESIAN_POINT('Ctrl Pts',(33.6220651386432,-3.0987841961425,-2.42198792435831));
#85681=CARTESIAN_POINT('Ctrl Pts',(33.6162009254719,-3.17016052399471,-2.33066631432769));
#85682=CARTESIAN_POINT('Ctrl Pts',(33.6103367123006,-3.23742547192394,-2.23627782131645));
#85683=CARTESIAN_POINT('Ctrl Pts',(33.6044724991293,-3.30032574039641,-2.13923795013011));
#85684=CARTESIAN_POINT('Ctrl Pts',(33.598599650555,-3.36331863325876,-2.04205518195652));
#85685=CARTESIAN_POINT('Ctrl Pts',(33.5927268019806,-3.42193381066567,-1.94221359850298));
#85686=CARTESIAN_POINT('Ctrl Pts',(33.5868539534063,-3.47596410363447,-1.84015286056474));
#85687=CARTESIAN_POINT('Ctrl Pts',(33.5852592087936,-3.49063577744745,-1.81243874365247));
#85688=CARTESIAN_POINT('Ctrl Pts',(33.5836644641809,-3.50496965262407,-1.78456110189523));
#85689=CARTESIAN_POINT('Ctrl Pts',(33.5820697195682,-3.51896220436475,-1.75652896482021));
#85690=CARTESIAN_POINT('Ctrl Pts',(33.5757828686536,-3.57412406915894,-1.64601981796256));
#85691=CARTESIAN_POINT('Ctrl Pts',(33.5694960177391,-3.62414209049564,-1.53277880180385));
#85692=CARTESIAN_POINT('Ctrl Pts',(33.5632091668245,-3.66875642446101,-1.41729153598547));
#85693=CARTESIAN_POINT('Ctrl Pts',(33.5569419548774,-3.71323139144215,-1.30216503117198));
#85694=CARTESIAN_POINT('Ctrl Pts',(33.5506747429303,-3.75233621169791,-1.18480656813154));
#85695=CARTESIAN_POINT('Ctrl Pts',(33.5444075309832,-3.78585837643043,-1.06572292534765));
#85696=CARTESIAN_POINT('Ctrl Pts',(33.5381521325137,-3.81931735304266,-0.946863751108828));
#85697=CARTESIAN_POINT('Ctrl Pts',(33.5318967340443,-3.84721455081169,-0.82628618464541));
#85698=CARTESIAN_POINT('Ctrl Pts',(33.5256413355748,-3.86938585152948,-0.704515529980335));
#85699=CARTESIAN_POINT('Ctrl Pts',(33.5194037340276,-3.89149407378478,-0.58309131893491));
#85700=CARTESIAN_POINT('Ctrl Pts',(33.5131661324805,-3.9079088197401,-0.460481103916105));
#85701=CARTESIAN_POINT('Ctrl Pts',(33.5069285309334,-3.91851629497949,-0.337222546666419));
#85702=CARTESIAN_POINT('Ctrl Pts',(33.5012735412267,-3.92813299826519,-0.225476731027766));
#85703=CARTESIAN_POINT('Ctrl Pts',(33.4956185515199,-3.93297714188587,-0.113198403560563));
#85704=CARTESIAN_POINT('Ctrl Pts',(33.4899635618132,-3.93299991924726,-0.00079699499911527));
#85705=CARTESIAN_POINT('',(32.2399635002821,-3.93299832602929,0.00362869822633291));
#85706=CARTESIAN_POINT('Ctrl Pts',(33.489963522035,-3.92664241618237,-0.000794917321835231));
#85707=CARTESIAN_POINT('Ctrl Pts',(33.4543831816328,-3.92537167507928,0.70527486915122));
#85708=CARTESIAN_POINT('Ctrl Pts',(33.3525204349843,-3.40567834183995,2.72842261129244));
#85709=CARTESIAN_POINT('Ctrl Pts',(33.1843752820887,-0.161577020458298,
4.64885823486118));
#85710=CARTESIAN_POINT('Ctrl Pts',(32.9855280633493,3.82329463833261,2.64960527812334));
#85711=CARTESIAN_POINT('Ctrl Pts',(32.7866808446095,4.29616613733598,-1.78352082740046));
#85712=CARTESIAN_POINT('Ctrl Pts',(32.5878336258701,0.822667401222829,-4.5783412245405));
#85713=CARTESIAN_POINT('Ctrl Pts',(32.4055945183451,-3.05328697462271,-3.28541975544593));
#85714=CARTESIAN_POINT('Ctrl Pts',(32.2896378170668,-3.92337245183106,-0.978557300575992));
#85715=CARTESIAN_POINT('Ctrl Pts',(32.239963522035,-3.93230204247149,0.00362762571011338));
#85716=CARTESIAN_POINT('',(30.9899635219853,-3.93299990487155,-0.000865032002295244));
#85717=CARTESIAN_POINT('Ctrl Pts',(32.2399635002821,-3.93299832602929,0.00362869822633291));
#85718=CARTESIAN_POINT('Ctrl Pts',(32.2324495091862,-3.93286122768884,0.152224009785864));
#85719=CARTESIAN_POINT('Ctrl Pts',(32.2249355180902,-3.92429936199548,0.300442608336801));
#85720=CARTESIAN_POINT('Ctrl Pts',(32.2174215269942,-3.90746138941711,0.447475686730029));
#85721=CARTESIAN_POINT('Ctrl Pts',(32.2097357398829,-3.89023844212168,0.597870453562282));
#85722=CARTESIAN_POINT('Ctrl Pts',(32.2020499527715,-3.86435660804196,0.747025156214954));
#85723=CARTESIAN_POINT('Ctrl Pts',(32.1943641656602,-3.83002292530235,0.894099206832475));
#85724=CARTESIAN_POINT('Ctrl Pts',(32.1929558399037,-3.82373170112221,0.921048713837953));
#85725=CARTESIAN_POINT('Ctrl Pts',(32.1915475141471,-3.81715682519089,0.947928419918569));
#85726=CARTESIAN_POINT('Ctrl Pts',(32.1901391883906,-3.81029974298554,0.974733229455291));
#85727=CARTESIAN_POINT('Ctrl Pts',(32.1842667422567,-3.78170703586469,1.08650410306624));
#85728=CARTESIAN_POINT('Ctrl Pts',(32.1783942961228,-3.74814427871285,1.19720293681802));
#85729=CARTESIAN_POINT('Ctrl Pts',(32.1725218499888,-3.70970722517867,1.30635420290868));
#85730=CARTESIAN_POINT('Ctrl Pts',(32.166657011044,-3.67131996314989,1.41536407403392));
#85731=CARTESIAN_POINT('Ctrl Pts',(32.1607921720991,-3.62807109743308,1.52282997788857));
#85732=CARTESIAN_POINT('Ctrl Pts',(32.1549273331542,-3.58010697852691,1.62828837197314));
#85733=CARTESIAN_POINT('Ctrl Pts',(32.1490685230342,-3.5321921648571,1.73363835895746));
#85734=CARTESIAN_POINT('Ctrl Pts',(32.1432097129142,-3.47957190924197,1.83698456685857));
#85735=CARTESIAN_POINT('Ctrl Pts',(32.1373509027941,-3.42244155250033,1.93788101278668));
#85736=CARTESIAN_POINT('Ctrl Pts',(32.1312651139132,-3.36309788327394,2.04268633266862));
#85737=CARTESIAN_POINT('Ctrl Pts',(32.1251793250322,-3.29888774047044,2.14484780840094));
#85738=CARTESIAN_POINT('Ctrl Pts',(32.1190935361512,-3.23008410045181,2.2438907513532));
#85739=CARTESIAN_POINT('Ctrl Pts',(32.113241506073,-3.16392324953187,2.33912939543602));
#85740=CARTESIAN_POINT('Ctrl Pts',(32.1073894759947,-3.09351552770848,2.43148428613212));
#85741=CARTESIAN_POINT('Ctrl Pts',(32.1015374459164,-3.0191487441359,2.52056141777633));
#85742=CARTESIAN_POINT('Ctrl Pts',(32.0956863055379,-2.94479326674391,2.60962500678647));
#85743=CARTESIAN_POINT('Ctrl Pts',(32.0898351651594,-2.86648018922745,2.69541151035522));
#85744=CARTESIAN_POINT('Ctrl Pts',(32.0839840247809,-2.78453781605224,2.7775597475077));
#85745=CARTESIAN_POINT('Ctrl Pts',(32.0781323572134,-2.70258805985182,2.85971538623378));
#85746=CARTESIAN_POINT('Ctrl Pts',(32.0722806896459,-2.61700864988439,2.93823181421886));
#85747=CARTESIAN_POINT('Ctrl Pts',(32.0664290220784,-2.52816446033411,3.01278500087602));
#85748=CARTESIAN_POINT('Ctrl Pts',(32.0605754103941,-2.43929075381722,3.08736295655783));
#85749=CARTESIAN_POINT('Ctrl Pts',(32.0547217987099,-2.34715042739772,3.15797478712707));
#85750=CARTESIAN_POINT('Ctrl Pts',(32.0488681870256,-2.25214052830562,3.22433745764355));
#85751=CARTESIAN_POINT('Ctrl Pts',(32.0430079209257,-2.15702262147515,3.29077556958269));
#85752=CARTESIAN_POINT('Ctrl Pts',(32.0371476548258,-2.0590289699169,3.35295464317976));
#85753=CARTESIAN_POINT('Ctrl Pts',(32.0312873887259,-1.95858470819298,3.41063556259425));
#85754=CARTESIAN_POINT('Ctrl Pts',(32.0254231755546,-1.85807279413596,3.46835533190128));
#85755=CARTESIAN_POINT('Ctrl Pts',(32.0195589623833,-1.75510734962699,3.52157072506845));
#85756=CARTESIAN_POINT('Ctrl Pts',(32.013694749212,-1.65013557193111,3.57008985800744));
#85757=CARTESIAN_POINT('Ctrl Pts',(32.0078219006377,-1.54500921704376,3.61868043825796));
#85758=CARTESIAN_POINT('Ctrl Pts',(32.0019490520634,-1.4378710135635,3.66256080019713));
#85759=CARTESIAN_POINT('Ctrl Pts',(31.9960762034891,-1.32918553622086,3.70158814703922));
#85760=CARTESIAN_POINT('Ctrl Pts',(31.9944814588765,-1.29967250225172,3.71218584087319));
#85761=CARTESIAN_POINT('Ctrl Pts',(31.9928867142638,-1.2700454455619,3.72242597756096));
#85762=CARTESIAN_POINT('Ctrl Pts',(31.9912919696511,-1.2403138039453,3.73230634698476));
#85763=CARTESIAN_POINT('Ctrl Pts',(31.9854195235172,-1.13083077921645,3.76868956268156));
#85764=CARTESIAN_POINT('Ctrl Pts',(31.9795470773833,-1.01956220703233,3.80031226505993));
#85765=CARTESIAN_POINT('Ctrl Pts',(31.9736746312493,-0.906959880597128,
3.82699788019111));
#85766=CARTESIAN_POINT('Ctrl Pts',(31.9678097923045,-0.794503419644181,
3.85364892667488));
#85767=CARTESIAN_POINT('Ctrl Pts',(31.9619449533597,-0.680717038829331,
3.8753755098871));
#85768=CARTESIAN_POINT('Ctrl Pts',(31.9560801144148,-0.566069807448353,
3.89205009899608));
#85769=CARTESIAN_POINT('Ctrl Pts',(31.9502213042948,-0.451540428932859,
3.90870754728025));
#85770=CARTESIAN_POINT('Ctrl Pts',(31.9443624941748,-0.336152366604314,
3.92032327198773));
#85771=CARTESIAN_POINT('Ctrl Pts',(31.9385036840548,-0.220386408026008,
3.92682044804157));
#85772=CARTESIAN_POINT('Ctrl Pts',(31.9324178951738,-0.100135509109817,
3.9335693340741));
#85773=CARTESIAN_POINT('Ctrl Pts',(31.9263321062928,0.0205227166320908,
3.9347949455506));
#85774=CARTESIAN_POINT('Ctrl Pts',(31.9202463174118,0.141041355778371,3.93047024361719));
#85775=CARTESIAN_POINT('Ctrl Pts',(31.9143942873336,0.256930801677664,3.92631165608009));
#85776=CARTESIAN_POINT('Ctrl Pts',(31.9085422572553,0.372690735103975,3.91702128789831));
#85777=CARTESIAN_POINT('Ctrl Pts',(31.902690227177,0.487834093622869,3.9026282038005));
#85778=CARTESIAN_POINT('Ctrl Pts',(31.8968390867985,0.602959946589611,3.8882373079217));
#85779=CARTESIAN_POINT('Ctrl Pts',(31.89098794642,0.717469000980662,3.86874528988671));
#85780=CARTESIAN_POINT('Ctrl Pts',(31.8851368060415,0.830879910554138,3.84423302808734));
#85781=CARTESIAN_POINT('Ctrl Pts',(31.879285138474,0.944301038474486,3.81971855772801));
#85782=CARTESIAN_POINT('Ctrl Pts',(31.8734334709065,1.05662342083569,3.7901830317544));
#85783=CARTESIAN_POINT('Ctrl Pts',(31.867581803339,1.16737718901218,3.7557581789266));
#85784=CARTESIAN_POINT('Ctrl Pts',(31.8617281916547,1.27816775323912,3.72132188902859));
#85785=CARTESIAN_POINT('Ctrl Pts',(31.8558745799705,1.38738827249572,3.68199316489111));
#85786=CARTESIAN_POINT('Ctrl Pts',(31.8500209682862,1.49458596776459,3.63795296629316));
#85787=CARTESIAN_POINT('Ctrl Pts',(31.8441607021864,1.60190552592078,3.59386270257257));
#85788=CARTESIAN_POINT('Ctrl Pts',(31.8383004360865,1.70719728767763,3.5450504311115));
#85789=CARTESIAN_POINT('Ctrl Pts',(31.8324401699866,1.81003023204784,3.49174448650998));
#85790=CARTESIAN_POINT('Ctrl Pts',(31.8265759568153,1.91293243760318,3.43840263869747));
#85791=CARTESIAN_POINT('Ctrl Pts',(31.8207117436439,2.01337217083464,3.38056129689765));
#85792=CARTESIAN_POINT('Ctrl Pts',(31.8148475304726,2.11094621299648,3.31849289374496));
#85793=CARTESIAN_POINT('Ctrl Pts',(31.8089746818983,2.20866393874395,3.25633309117372));
#85794=CARTESIAN_POINT('Ctrl Pts',(31.8031018333241,2.3035072139943,3.18993404036242));
#85795=CARTESIAN_POINT('Ctrl Pts',(31.7972289847498,2.39510471650483,3.11960933403148));
#85796=CARTESIAN_POINT('Ctrl Pts',(31.795634240137,2.41997759068629,3.10051298833999));
#85797=CARTESIAN_POINT('Ctrl Pts',(31.7940394955241,2.44461133786158,3.08112739090936));
#85798=CARTESIAN_POINT('Ctrl Pts',(31.7924447509113,2.46899899574816,3.06145928586263));
#85799=CARTESIAN_POINT('Ctrl Pts',(31.7865723047774,2.55880347360716,2.98903396677659));
#85800=CARTESIAN_POINT('Ctrl Pts',(31.7806998586435,2.64556882901847,2.91253257095941));
#85801=CARTESIAN_POINT('Ctrl Pts',(31.7748274125096,2.72890223720773,2.83223967555055));
#85802=CARTESIAN_POINT('Ctrl Pts',(31.7689625735647,2.81212769498282,2.75205079186402));
#85803=CARTESIAN_POINT('Ctrl Pts',(31.7630977346199,2.89192975164321,2.66808046002105));
#85804=CARTESIAN_POINT('Ctrl Pts',(31.757232895675,2.96794749654531,2.58065430806809));
#85805=CARTESIAN_POINT('Ctrl Pts',(31.751374085555,3.04388709818183,2.49331802677652));
#85806=CARTESIAN_POINT('Ctrl Pts',(31.745515275435,3.11604985613295,2.40253330144581));
#85807=CARTESIAN_POINT('Ctrl Pts',(31.7396564653149,3.18411117770079,2.30866303475429));
#85808=CARTESIAN_POINT('Ctrl Pts',(31.733570676434,3.25480929310917,2.21115609843426));
#85809=CARTESIAN_POINT('Ctrl Pts',(31.727484887553,3.32108142651117,2.11032002405109));
#85810=CARTESIAN_POINT('Ctrl Pts',(31.721399098672,3.38260911089501,2.00660025986494));
#85811=CARTESIAN_POINT('Ctrl Pts',(31.7155470685938,3.44177348000197,1.90686443405825));
#85812=CARTESIAN_POINT('Ctrl Pts',(31.7096950385155,3.49655092076498,1.80446274895838));
#85813=CARTESIAN_POINT('Ctrl Pts',(31.7038430084372,3.54670252304745,1.69982064142333));
#85814=CARTESIAN_POINT('Ctrl Pts',(31.6979918680587,3.59684650064796,1.59519444290721));
#85815=CARTESIAN_POINT('Ctrl Pts',(31.6921407276802,3.64236585951319,1.48832887186991));
#85816=CARTESIAN_POINT('Ctrl Pts',(31.6862895873017,3.68306836642569,1.37967257283546));
#85817=CARTESIAN_POINT('Ctrl Pts',(31.6804379197342,3.72377454064267,1.27100648384548));
#85818=CARTESIAN_POINT('Ctrl Pts',(31.6745862521667,3.75966285514443,1.16054973323197));
#85819=CARTESIAN_POINT('Ctrl Pts',(31.6687345845992,3.79059005856127,1.04876880576058));
#85820=CARTESIAN_POINT('Ctrl Pts',(31.662880972915,3.82152753701391,0.936950740982704));
#85821=CARTESIAN_POINT('Ctrl Pts',(31.6570273612307,3.84750051678102,0.823808022741547));
#85822=CARTESIAN_POINT('Ctrl Pts',(31.6511737495465,3.86841640059097,0.709819379588075));
#85823=CARTESIAN_POINT('Ctrl Pts',(31.6453134834466,3.88935606168445,0.595701153562978));
#85824=CARTESIAN_POINT('Ctrl Pts',(31.6394532173467,3.90522707749785,0.480735490010174));
#85825=CARTESIAN_POINT('Ctrl Pts',(31.6335929512468,3.915988467671,0.365408430482562));
#85826=CARTESIAN_POINT('Ctrl Pts',(31.6277287380755,3.926757105975,0.250003694594859));
#85827=CARTESIAN_POINT('Ctrl Pts',(31.6218645249042,3.93240924582848,0.13423748990664));
#85828=CARTESIAN_POINT('Ctrl Pts',(31.6160003117329,3.93295603548759,0.0185963147360922));
#85829=CARTESIAN_POINT('Ctrl Pts',(31.6101274631586,3.93350363032702,-0.0972151489489237));
#85830=CARTESIAN_POINT('Ctrl Pts',(31.6042546145843,3.92893088694179,-0.212900804182463));
#85831=CARTESIAN_POINT('Ctrl Pts',(31.59838176601,3.91930082458506,-0.327978728589047));
#85832=CARTESIAN_POINT('Ctrl Pts',(31.5967870213972,3.91668582611037,-0.359227601716395));
#85833=CARTESIAN_POINT('Ctrl Pts',(31.5951922767845,3.91369820807359,-0.390431720451608));
#85834=CARTESIAN_POINT('Ctrl Pts',(31.5935975321717,3.91033987911371,-0.421581581444166));
#85835=CARTESIAN_POINT('Ctrl Pts',(31.5877250860378,3.89797325579415,-0.536287020355445));
#85836=CARTESIAN_POINT('Ctrl Pts',(31.5818526399039,3.88053451576804,-0.650639898796893));
#85837=CARTESIAN_POINT('Ctrl Pts',(31.57598019377,3.85805064348412,-0.764155895293471));
#85838=CARTESIAN_POINT('Ctrl Pts',(31.5701153548252,3.83559589689393,-0.877524842736153));
#85839=CARTESIAN_POINT('Ctrl Pts',(31.5642505158803,3.80810909437062,-0.990058662381687));
#85840=CARTESIAN_POINT('Ctrl Pts',(31.5583856769355,3.77566900904911,-1.10127768256061));
#85841=CARTESIAN_POINT('Ctrl Pts',(31.5525268668155,3.74326227086528,-1.21238237394107));
#85842=CARTESIAN_POINT('Ctrl Pts',(31.5466680566955,3.7059124927633,-1.32217455974736));
#85843=CARTESIAN_POINT('Ctrl Pts',(31.5408092465755,3.66374944111582,-1.43018496451457));
#85844=CARTESIAN_POINT('Ctrl Pts',(31.5347234576945,3.61995293198713,-1.54237984827041));
#85845=CARTESIAN_POINT('Ctrl Pts',(31.5286376688135,3.57096274845395,-1.65265165554713));
#85846=CARTESIAN_POINT('Ctrl Pts',(31.5225518799326,3.5169814071894,-1.76049163062028));
#85847=CARTESIAN_POINT('Ctrl Pts',(31.5166998498543,3.46507352163452,-1.8641894075411));
#85848=CARTESIAN_POINT('Ctrl Pts',(31.510847819776,3.40855103440419,-1.96563831864943));
#85849=CARTESIAN_POINT('Ctrl Pts',(31.5049957896978,3.34764264561864,-2.06440735254344));
#85850=CARTESIAN_POINT('Ctrl Pts',(31.4991446493193,3.28674351689803,-2.16316137031758));
#85851=CARTESIAN_POINT('Ctrl Pts',(31.4932935089408,3.22146002934798,-2.25923596923873));
#85852=CARTESIAN_POINT('Ctrl Pts',(31.4874423685623,3.15206564427238,-2.35222685432289));
#85853=CARTESIAN_POINT('Ctrl Pts',(31.4815907009948,3.08266500674803,-2.44522611790543));
#85854=CARTESIAN_POINT('Ctrl Pts',(31.4757390334273,3.00915298262472,-2.53514078402328));
#85855=CARTESIAN_POINT('Ctrl Pts',(31.4698873658598,2.93184452556327,-2.62159811525808));
#85856=CARTESIAN_POINT('Ctrl Pts',(31.4640337541756,2.85451038408561,-2.70808417046646));
#85857=CARTESIAN_POINT('Ctrl Pts',(31.4581801424913,2.77337757703474,-2.79111029881737));
#85858=CARTESIAN_POINT('Ctrl Pts',(31.4523265308071,2.68879874684229,-2.87033975323119));
#85859=CARTESIAN_POINT('Ctrl Pts',(31.4464662647072,2.60412376700378,-2.94965927609339));
#85860=CARTESIAN_POINT('Ctrl Pts',(31.4406059986074,2.51599524676099,-3.02517322751174));
#85861=CARTESIAN_POINT('Ctrl Pts',(31.4347457325075,2.42479989010049,-3.09658432679762));
#85862=CARTESIAN_POINT('Ctrl Pts',(31.4288815193362,2.33354311053194,-3.1680435236791));
#85863=CARTESIAN_POINT('Ctrl Pts',(31.4230173061649,2.23921571708517,-3.23539412633645));
#85864=CARTESIAN_POINT('Ctrl Pts',(31.4171530929936,2.14223298445839,-3.29838245816014));
#85865=CARTESIAN_POINT('Ctrl Pts',(31.4112802444193,2.04510743898454,-3.36146354405205));
#85866=CARTESIAN_POINT('Ctrl Pts',(31.405407395845,1.9453191053953,-3.42016932986814));
#85867=CARTESIAN_POINT('Ctrl Pts',(31.3995345472707,1.8433074562443,-3.47429224760298));
#85868=CARTESIAN_POINT('Ctrl Pts',(31.3979398026579,1.81560666915988,-3.48898907324042));
#85869=CARTESIAN_POINT('Ctrl Pts',(31.396345058045,1.7877420506565,-3.50334824882253));
#85870=CARTESIAN_POINT('Ctrl Pts',(31.3947503134321,1.75972262705796,-3.51736624135449));
#85871=CARTESIAN_POINT('Ctrl Pts',(31.3888778672982,1.65654462949257,-3.56898573289212));
#85872=CARTESIAN_POINT('Ctrl Pts',(31.3830054211642,1.5509206634995,-3.61614788158668));
#85873=CARTESIAN_POINT('Ctrl Pts',(31.3771329750303,1.44327273538859,-3.65861350941636));
#85874=CARTESIAN_POINT('Ctrl Pts',(31.3712681360855,1.33576425481336,-3.70102412711018));
#85875=CARTESIAN_POINT('Ctrl Pts',(31.3654032971406,1.22623740701823,-3.73875017234563));
#85876=CARTESIAN_POINT('Ctrl Pts',(31.3595384581958,1.11513828952806,-3.77159854640289));
#85877=CARTESIAN_POINT('Ctrl Pts',(31.3536796480758,1.00415337758109,-3.80441315361765));
#85878=CARTESIAN_POINT('Ctrl Pts',(31.3478208379557,0.891599804726413,-3.83235994638736));
#85879=CARTESIAN_POINT('Ctrl Pts',(31.3419620278357,0.777942495674706,-3.85529434329253));
#85880=CARTESIAN_POINT('Ctrl Pts',(31.3358762389548,0.659881938411699,-3.87911725183847));
#85881=CARTESIAN_POINT('Ctrl Pts',(31.3297904500738,0.540630817295887,-3.89753136803522));
#85882=CARTESIAN_POINT('Ctrl Pts',(31.3237046611928,0.420726605016576,-3.91043196128397));
#85883=CARTESIAN_POINT('Ctrl Pts',(31.3178526311145,0.305427985479641,-3.92283703500502));
#85884=CARTESIAN_POINT('Ctrl Pts',(31.3120006010363,0.189525969535115,-3.93014427989007));
#85885=CARTESIAN_POINT('Ctrl Pts',(31.306148570958,0.0735067883130117,-3.93231302824075));
#85886=CARTESIAN_POINT('Ctrl Pts',(31.3002974305795,-0.0424947542032381,
-3.93448144687082));
#85887=CARTESIAN_POINT('Ctrl Pts',(31.294446290201,-0.158613013407076,-3.93151291456186));
#85888=CARTESIAN_POINT('Ctrl Pts',(31.2885951498225,-0.274360029426959,
-3.92341886296287));
#85889=CARTESIAN_POINT('Ctrl Pts',(31.282743482255,-0.390117474277434,-3.91532408208811));
#85890=CARTESIAN_POINT('Ctrl Pts',(31.2768918146875,-0.505503197075474,
-3.90210289272387));
#85891=CARTESIAN_POINT('Ctrl Pts',(31.27104014712,-0.620033349112839,-3.88381869375849));
#85892=CARTESIAN_POINT('Ctrl Pts',(31.2651865354358,-0.734601551839591,
-3.8655284201799));
#85893=CARTESIAN_POINT('Ctrl Pts',(31.2593329237516,-0.84831321062232,-3.84217185738055));
#85894=CARTESIAN_POINT('Ctrl Pts',(31.2534793120673,-0.96069437344229,-3.8138635687235));
#85895=CARTESIAN_POINT('Ctrl Pts',(31.2476190459675,-1.07320329174214,-3.78552309905931));
#85896=CARTESIAN_POINT('Ctrl Pts',(31.2417587798676,-1.18437829407815,-3.75221976897599));
#85897=CARTESIAN_POINT('Ctrl Pts',(31.2358985137677,-1.29376021047995,-3.71411813460192));
#85898=CARTESIAN_POINT('Ctrl Pts',(31.2300343005964,-1.40321579900311,-3.67599083759253));
#85899=CARTESIAN_POINT('Ctrl Pts',(31.2241700874251,-1.51087551380498,-3.63305895385118));
#85900=CARTESIAN_POINT('Ctrl Pts',(31.2183058742538,-1.61630141657886,-3.5855346506156));
#85901=CARTESIAN_POINT('Ctrl Pts',(31.2124330256795,-1.72188256527054,-3.53794036501441));
#85902=CARTESIAN_POINT('Ctrl Pts',(31.2065601771052,-1.82522296933522,-3.48574034876349));
#85903=CARTESIAN_POINT('Ctrl Pts',(31.2006873285309,-1.92591039340687,-3.42919205594662));
#85904=CARTESIAN_POINT('Ctrl Pts',(31.1990925839181,-1.95325159335207,-3.41383663102915));
#85905=CARTESIAN_POINT('Ctrl Pts',(31.1974978393053,-1.98039734438661,-3.39816081881947));
#85906=CARTESIAN_POINT('Ctrl Pts',(31.1959030946925,-2.00733979389806,-3.38217030201516));
#85907=CARTESIAN_POINT('Ctrl Pts',(31.1900306485585,-2.10655197006687,-3.32328723833731));
#85908=CARTESIAN_POINT('Ctrl Pts',(31.1841582024246,-2.20333714987633,-3.25993647329951));
#85909=CARTESIAN_POINT('Ctrl Pts',(31.1782857562907,-2.2972659515097,-3.19234367636604));
#85910=CARTESIAN_POINT('Ctrl Pts',(31.1724209173458,-2.39107307741595,-3.12483843939897));
#85911=CARTESIAN_POINT('Ctrl Pts',(31.166556078401,-2.48203085103357,-3.05310233764));
#85912=CARTESIAN_POINT('Ctrl Pts',(31.1606912394561,-2.56973562649878,-2.97740622184863));
#85913=CARTESIAN_POINT('Ctrl Pts',(31.1548324293361,-2.65735024488843,-2.9017879187008));
#85914=CARTESIAN_POINT('Ctrl Pts',(31.1489736192161,-2.74171820538918,-2.82221796690118));
#85915=CARTESIAN_POINT('Ctrl Pts',(31.1431148090961,-2.82246649527063,-2.73900928860688));
#85916=CARTESIAN_POINT('Ctrl Pts',(31.1370290202151,-2.9063430904582,-2.65257698600789));
#85917=CARTESIAN_POINT('Ctrl Pts',(31.1309432313341,-2.98631351137256,-2.56221858107816));
#85918=CARTESIAN_POINT('Ctrl Pts',(31.1248574424532,-3.06199904071403,-2.46832957172789));
#85919=CARTESIAN_POINT('Ctrl Pts',(31.1190054123749,-3.13477744345842,-2.37804689556482));
#85920=CARTESIAN_POINT('Ctrl Pts',(31.1131533822966,-3.2035937697591,-2.28450018871559));
#85921=CARTESIAN_POINT('Ctrl Pts',(31.1073013522183,-3.26815089943506,-2.18807648370019));
#85922=CARTESIAN_POINT('Ctrl Pts',(31.1014502118398,-3.33269821431826,-2.09166743823808));
#85923=CARTESIAN_POINT('Ctrl Pts',(31.0955990714613,-3.39298739018811,-1.99238260768692));
#85924=CARTESIAN_POINT('Ctrl Pts',(31.0897479310828,-3.4487641985508,-1.89063864945004));
#85925=CARTESIAN_POINT('Ctrl Pts',(31.0838962635153,-3.50454603241568,-1.78888552406107));
#85926=CARTESIAN_POINT('Ctrl Pts',(31.0780445959478,-3.55581449184181,-1.68467319301558));
#85927=CARTESIAN_POINT('Ctrl Pts',(31.0721929283803,-3.60236128658844,-1.57844295458813));
#85928=CARTESIAN_POINT('Ctrl Pts',(31.066339316696,-3.64892354571373,-1.4721774229758));
#85929=CARTESIAN_POINT('Ctrl Pts',(31.0604857050118,-3.69076085510404,-1.3638930293081));
#85930=CARTESIAN_POINT('Ctrl Pts',(31.0546320933275,-3.72771331577219,-1.25405041183149));
#85931=CARTESIAN_POINT('Ctrl Pts',(31.0487718272276,-3.76470778418629,-1.1440829247065));
#85932=CARTESIAN_POINT('Ctrl Pts',(31.0429115611277,-3.79680618815631,-1.03255407013663));
#85933=CARTESIAN_POINT('Ctrl Pts',(31.0370512950278,-3.8238986758598,-0.919939083177609));
#85934=CARTESIAN_POINT('Ctrl Pts',(31.0311870818565,-3.85100941119605,-0.807248246523758));
#85935=CARTESIAN_POINT('Ctrl Pts',(31.0253228686852,-3.87310743803521,-0.693470225611817));
#85936=CARTESIAN_POINT('Ctrl Pts',(31.0194586555139,-3.89013443562237,-0.579088139047071));
#85937=CARTESIAN_POINT('Ctrl Pts',(31.0135858069396,-3.90718650647712,-0.46453761805056));
#85938=CARTESIAN_POINT('Ctrl Pts',(31.0077129583653,-3.91915260208994,-0.349381665687266));
#85939=CARTESIAN_POINT('Ctrl Pts',(31.001840109791,-3.92602639524769,-0.234106266081031));
#85940=CARTESIAN_POINT('Ctrl Pts',(31.0002453651783,-3.92789294168911,-0.202803769485678));
#85941=CARTESIAN_POINT('Ctrl Pts',(30.9986506205656,-3.92938429425715,-0.171492449566823));
#85942=CARTESIAN_POINT('Ctrl Pts',(30.9970558759528,-3.93050098729974,-0.140181984704809));
#85943=CARTESIAN_POINT('Ctrl Pts',(30.9946917579802,-3.93215642107315,-0.093766005543916));
#85944=CARTESIAN_POINT('Ctrl Pts',(30.9923276400076,-3.9329896873435,-0.0473205289319825));
#85945=CARTESIAN_POINT('Ctrl Pts',(30.9899635220349,-3.93299990487134,-0.000865032977774666));
#85946=CARTESIAN_POINT('',(29.7399635545323,-3.9321542581735,-0.00319654787924418));
#85947=CARTESIAN_POINT('Ctrl Pts',(30.9899635219853,-3.93299990487155,-0.000865032002347642));
#85948=CARTESIAN_POINT('Ctrl Pts',(30.9841253417436,-3.93302513698879,0.113856636603515));
#85949=CARTESIAN_POINT('Ctrl Pts',(30.9782871615019,-3.92802663704679,0.228780085806603));
#85950=CARTESIAN_POINT('Ctrl Pts',(30.9724489812603,-3.91797751735153,0.343425644831478));
#85951=CARTESIAN_POINT('Ctrl Pts',(30.9666182781553,-3.90794126787233,0.457924373769877));
#85952=CARTESIAN_POINT('Ctrl Pts',(30.9607875750502,-3.89286729525467,0.572145506995858));
#85953=CARTESIAN_POINT('Ctrl Pts',(30.9549568719452,-3.87278070147756,0.685608225054937));
#85954=CARTESIAN_POINT('Ctrl Pts',(30.9491320302226,-3.85271429998339,0.798956883391825));
#85955=CARTESIAN_POINT('Ctrl Pts',(30.9433071884999,-3.82764537044766,0.911548232901897));
#85956=CARTESIAN_POINT('Ctrl Pts',(30.9374823467773,-3.79765084705022,1.02290617551112));
#85957=CARTESIAN_POINT('Ctrl Pts',(30.9316615817414,-3.76767731620202,1.13418618098947));
#85958=CARTESIAN_POINT('Ctrl Pts',(30.9258408167055,-3.73278515561282,1.24423409336451));
#85959=CARTESIAN_POINT('Ctrl Pts',(30.9200200516697,-3.69310231239223,1.35258430798347));
#85960=CARTESIAN_POINT('Ctrl Pts',(30.9142014303861,-3.65343408412109,1.46089461787837));
#85961=CARTESIAN_POINT('Ctrl Pts',(30.9083828091025,-3.60897882362711,1.56750808008232));
#85962=CARTESIAN_POINT('Ctrl Pts',(30.902564187819,-3.55991403820347,1.67197519138348));
#85963=CARTESIAN_POINT('Ctrl Pts',(30.8967462590075,-3.51085509196278,1.77642987009029));
#85964=CARTESIAN_POINT('Ctrl Pts',(30.890928330196,-3.45718788940113,1.87873832685015));
#85965=CARTESIAN_POINT('Ctrl Pts',(30.8851104013845,-3.39913737069582,1.97847267737998));
#85966=CARTESIAN_POINT('Ctrl Pts',(30.879291714612,-3.34107928915678,2.07822002132187));
#85967=CARTESIAN_POINT('Ctrl Pts',(30.8734730278396,-3.27863696731716,2.17539223080068));
#85968=CARTESIAN_POINT('Ctrl Pts',(30.8676543410671,-3.21208002246922,2.2695882730694));
#85969=CARTESIAN_POINT('Ctrl Pts',(30.8618296959027,-3.14545492266097,2.36388077300362));
#85970=CARTESIAN_POINT('Ctrl Pts',(30.8560050507382,-3.07470702598918,2.45519067578944));
#85971=CARTESIAN_POINT('Ctrl Pts',(30.8501804055738,-3.00014789455701,2.5431479726483));
#85972=CARTESIAN_POINT('Ctrl Pts',(30.8443528158915,-2.92555107143917,2.63114973433288));
#85973=CARTESIAN_POINT('Ctrl Pts',(30.8385252262092,-2.84713946084802,2.7157952074665));
#85974=CARTESIAN_POINT('Ctrl Pts',(30.8326976365269,-2.76526202818392,2.79675077822178));
#85975=CARTESIAN_POINT('Ctrl Pts',(30.8268603130383,-2.68324783587989,2.87784156883371));
#85976=CARTESIAN_POINT('Ctrl Pts',(30.8210229895497,-2.59775656565234,2.95522986146392));
#85977=CARTESIAN_POINT('Ctrl Pts',(30.8151856660612,-2.50917122701455,3.02862159298951));
#85978=CARTESIAN_POINT('Ctrl Pts',(30.8095266631118,-2.42329202336917,3.09977132898978));
#85979=CARTESIAN_POINT('Ctrl Pts',(30.8038676601625,-2.33450535955606,3.16716498088228));
#85980=CARTESIAN_POINT('Ctrl Pts',(30.7982086572131,-2.24318446416675,3.23057463305229));
#85981=CARTESIAN_POINT('Ctrl Pts',(30.7923362110792,-2.14841917708794,3.29637593587396));
#85982=CARTESIAN_POINT('Ctrl Pts',(30.7864637649453,-2.05059746597944,3.35811411933725));
#85983=CARTESIAN_POINT('Ctrl Pts',(30.7805913188114,-1.9501029296624,3.41549228717064));
#85984=CARTESIAN_POINT('Ctrl Pts',(30.7747264798666,-1.84973857435013,3.47279612710707));
#85985=CARTESIAN_POINT('Ctrl Pts',(30.7688616409218,-1.74670863494545,3.5257509801732));
#85986=CARTESIAN_POINT('Ctrl Pts',(30.7629968019769,-1.6414271244812,3.57410212431282));
#85987=CARTESIAN_POINT('Ctrl Pts',(30.7571379918569,-1.53625383928816,3.62240356536911));
#85988=CARTESIAN_POINT('Ctrl Pts',(30.7512791817369,-1.42883396013813,3.66611053908882));
#85989=CARTESIAN_POINT('Ctrl Pts',(30.745420371617,-1.31960705157309,3.70501366116761));
#85990=CARTESIAN_POINT('Ctrl Pts',(30.739334582736,-1.2061485349061,3.74542394635063));
#85991=CARTESIAN_POINT('Ctrl Pts',(30.733248793855,-1.09074053777285,3.78065041027169));
#85992=CARTESIAN_POINT('Ctrl Pts',(30.727163004974,-0.973900112830244,3.81051276998638));
#85993=CARTESIAN_POINT('Ctrl Pts',(30.7213109748958,-0.861547598720272,
3.83922809854539));
#85994=CARTESIAN_POINT('Ctrl Pts',(30.7154589448175,-0.747871105288671,
3.86298368670579));
#85995=CARTESIAN_POINT('Ctrl Pts',(30.7096069147393,-0.633346099804996,
3.88166996508742));
#85996=CARTESIAN_POINT('Ctrl Pts',(30.7037557743608,-0.518838505863574,
3.90035340254428));
#85997=CARTESIAN_POINT('Ctrl Pts',(30.6979046339823,-0.40348306421814,3.91396899608031));
#85998=CARTESIAN_POINT('Ctrl Pts',(30.6920534936038,-0.287764380499728,
3.92245849708007));
#85999=CARTESIAN_POINT('Ctrl Pts',(30.6862018260363,-0.172035270503619,
3.93094876298565));
#86000=CARTESIAN_POINT('Ctrl Pts',(30.6803501584688,-0.055943265647758,
3.93431198797021));
#86001=CARTESIAN_POINT('Ctrl Pts',(30.6744984909013,0.0600236891657086,
3.93254194596052));
#86002=CARTESIAN_POINT('Ctrl Pts',(30.6686448792171,0.176029172022672,3.93077131588455));
#86003=CARTESIAN_POINT('Ctrl Pts',(30.6627912675328,0.291909109136011,3.92386403395518));
#86004=CARTESIAN_POINT('Ctrl Pts',(30.6569376558486,0.407178057208399,3.91186592685997));
#86005=CARTESIAN_POINT('Ctrl Pts',(30.6510773897487,0.522578043609061,3.8998541802554));
#86006=CARTESIAN_POINT('Ctrl Pts',(30.6452171236488,0.637365243240775,3.88274010009507));
#86007=CARTESIAN_POINT('Ctrl Pts',(30.6393568575489,0.75106171691046,3.86062110254186));
#86008=CARTESIAN_POINT('Ctrl Pts',(30.6334926443776,0.864834768690114,3.83848720715608));
#86009=CARTESIAN_POINT('Ctrl Pts',(30.6276284312063,0.9775152308187,3.81134177867732));
#86010=CARTESIAN_POINT('Ctrl Pts',(30.621764218035,1.08863939147607,3.77933238486993));
#86011=CARTESIAN_POINT('Ctrl Pts',(30.6158913694607,1.19992718907508,3.74727585532468));
#86012=CARTESIAN_POINT('Ctrl Pts',(30.6100185208864,1.309653721049,3.71034119694256));
#86013=CARTESIAN_POINT('Ctrl Pts',(30.6041456723121,1.41737425990548,3.66872446599052));
#86014=CARTESIAN_POINT('Ctrl Pts',(30.6025509276993,1.44662526933686,3.65742363698888));
#86015=CARTESIAN_POINT('Ctrl Pts',(30.6009561830864,1.47572850051372,3.64577782989925));
#86016=CARTESIAN_POINT('Ctrl Pts',(30.5993614384736,1.50467537090407,3.63379154990964));
#86017=CARTESIAN_POINT('Ctrl Pts',(30.5934889923397,1.61126857444412,3.58965358385694));
#86018=CARTESIAN_POINT('Ctrl Pts',(30.5876165462057,1.71609648552891,3.54074755642489));
#86019=CARTESIAN_POINT('Ctrl Pts',(30.5817441000718,1.81870193655789,3.48723561950731));
#86020=CARTESIAN_POINT('Ctrl Pts',(30.575879261127,1.92117447209504,3.43379300215652));
#86021=CARTESIAN_POINT('Ctrl Pts',(30.5700144221821,2.02142990972165,3.37575652997487));
#86022=CARTESIAN_POINT('Ctrl Pts',(30.5641495832373,2.1190301138874,3.31333674359223));
#86023=CARTESIAN_POINT('Ctrl Pts',(30.5582907731173,2.21652998886429,3.25098112230627));
#86024=CARTESIAN_POINT('Ctrl Pts',(30.5524319629973,2.31137971331781,3.18425137062467));
#86025=CARTESIAN_POINT('Ctrl Pts',(30.5465731528773,2.40316547425604,3.11340403792116));
#86026=CARTESIAN_POINT('Ctrl Pts',(30.5404873639963,2.49850714806143,3.03981197728392));
#86027=CARTESIAN_POINT('Ctrl Pts',(30.5344015751153,2.59054224926123,2.96177705106598));
#86028=CARTESIAN_POINT('Ctrl Pts',(30.5283157862343,2.6788395465697,2.87963672773742));
#86029=CARTESIAN_POINT('Ctrl Pts',(30.5224637561561,2.76374529170566,2.80065146351629));
#86030=CARTESIAN_POINT('Ctrl Pts',(30.5166117260778,2.8451947481822,2.71787067367035));
#86031=CARTESIAN_POINT('Ctrl Pts',(30.5107596959995,2.92283865523893,2.63163508021934));
#86032=CARTESIAN_POINT('Ctrl Pts',(30.504908555621,3.00047075788517,2.54541259739586));
#86033=CARTESIAN_POINT('Ctrl Pts',(30.4990574152425,3.07429818498459,2.45573666242723));
#86034=CARTESIAN_POINT('Ctrl Pts',(30.493206274864,3.14400990605597,2.36298343426735));
#86035=CARTESIAN_POINT('Ctrl Pts',(30.4873546072965,3.21372790816818,2.27022184902196));
#86036=CARTESIAN_POINT('Ctrl Pts',(30.481502939729,3.27932921872088,2.17438274986283));
#86037=CARTESIAN_POINT('Ctrl Pts',(30.4756512721615,3.34054476348101,2.07587323388969));
#86038=CARTESIAN_POINT('Ctrl Pts',(30.4697976604772,3.40178064606174,1.97733098981012));
#86039=CARTESIAN_POINT('Ctrl Pts',(30.463944048793,3.45862764744553,1.87611691567687));
#86040=CARTESIAN_POINT('Ctrl Pts',(30.4580904371087,3.51086183328906,1.77266414967816));
#86041=CARTESIAN_POINT('Ctrl Pts',(30.4522301710089,3.56315539922169,1.66909377804698));
#86042=CARTESIAN_POINT('Ctrl Pts',(30.446369904909,3.6108254966039,1.56328000411087));
#86043=CARTESIAN_POINT('Ctrl Pts',(30.4405096388091,3.65369564616487,1.45567754849619));
#86044=CARTESIAN_POINT('Ctrl Pts',(30.4346454256378,3.69659467010448,1.3480026192821));
#86045=CARTESIAN_POINT('Ctrl Pts',(30.4287812124665,3.73468717332118,1.23853699896449));
#86046=CARTESIAN_POINT('Ctrl Pts',(30.4229169992952,3.76784655740463,1.12775055746123));
#86047=CARTESIAN_POINT('Ctrl Pts',(30.4170441507209,3.80105477065506,1.01680097632789));
#86048=CARTESIAN_POINT('Ctrl Pts',(30.4111713021466,3.82931526613401,0.904527091545456));
#86049=CARTESIAN_POINT('Ctrl Pts',(30.4052984535723,3.85255249941213,0.791409021475846));
#86050=CARTESIAN_POINT('Ctrl Pts',(30.4037037089595,3.85886246162522,0.760692337642873));
#86051=CARTESIAN_POINT('Ctrl Pts',(30.4021089643467,3.86480231998018,0.72991343301046));
#86052=CARTESIAN_POINT('Ctrl Pts',(30.4005142197339,3.8703712236184,0.699081963282273));
#86053=CARTESIAN_POINT('Ctrl Pts',(30.3946417735999,3.89087800970672,0.585548960095529));
#86054=CARTESIAN_POINT('Ctrl Pts',(30.388769327466,3.9064193483538,0.470922797049242));
#86055=CARTESIAN_POINT('Ctrl Pts',(30.3828968813321,3.91688444797553,0.355675724793542));
#86056=CARTESIAN_POINT('Ctrl Pts',(30.3770320423872,3.92733599106737,0.240577944034012));
#86057=CARTESIAN_POINT('Ctrl Pts',(30.3711672034424,3.9327243349837,0.12486126145588));
#86058=CARTESIAN_POINT('Ctrl Pts',(30.3653023644975,3.9329896840009,0.00900808206402624));
#86059=CARTESIAN_POINT('Ctrl Pts',(30.3594435543775,3.93325476024971,-0.106726004795038));
#86060=CARTESIAN_POINT('Ctrl Pts',(30.3535847442575,3.92840731549468,-0.222595898502569));
#86061=CARTESIAN_POINT('Ctrl Pts',(30.3477259341375,3.91843940843405,-0.338114777007737));
#86062=CARTESIAN_POINT('Ctrl Pts',(30.3416401452565,3.90808533026572,-0.458109023611916));
#86063=CARTESIAN_POINT('Ctrl Pts',(30.3355543563755,3.8922059763021,-0.577724054775901));
#86064=CARTESIAN_POINT('Ctrl Pts',(30.3294685674946,3.87085205685679,-0.696414642240932));
#86065=CARTESIAN_POINT('Ctrl Pts',(30.3236165374163,3.85031835427077,-0.81054625302127));
#86066=CARTESIAN_POINT('Ctrl Pts',(30.317764507338,3.82472297102752,-0.923822682539965));
#86067=CARTESIAN_POINT('Ctrl Pts',(30.3119124772597,3.79416367665801,-1.03576589764723));
#86068=CARTESIAN_POINT('Ctrl Pts',(30.3060613368812,3.76360902829963,-1.14769209372857));
#86069=CARTESIAN_POINT('Ctrl Pts',(30.3002101965027,3.7280920781872,-1.25828507976001));
#86070=CARTESIAN_POINT('Ctrl Pts',(30.2943590561242,3.68776107721996,-1.36707982113023));
#86071=CARTESIAN_POINT('Ctrl Pts',(30.2885073885567,3.647426442421,-1.47588436492967));
#86072=CARTESIAN_POINT('Ctrl Pts',(30.2826557209892,3.60227703820654,-1.58288995437695));
#86073=CARTESIAN_POINT('Ctrl Pts',(30.2768040534217,3.55250982709289,-1.68765012025847));
#86074=CARTESIAN_POINT('Ctrl Pts',(30.2709504417374,3.50272608167206,-1.79244509091858));
#86075=CARTESIAN_POINT('Ctrl Pts',(30.2650968300531,3.44832165599115,-1.89499278146015));
#86076=CARTESIAN_POINT('Ctrl Pts',(30.2592432183689,3.3895398261628,-1.99487061406404));
#86077=CARTESIAN_POINT('Ctrl Pts',(30.253382952269,3.33069117285034,-2.09486198829771));
#86078=CARTESIAN_POINT('Ctrl Pts',(30.2475226861691,3.26745539273513,-2.19217709016946));
#86079=CARTESIAN_POINT('Ctrl Pts',(30.2416624200692,3.20011957671275,-2.28642159164486));
#86080=CARTESIAN_POINT('Ctrl Pts',(30.2357982068979,3.13273840792464,-2.38072956972229));
#86081=CARTESIAN_POINT('Ctrl Pts',(30.2299339937265,3.06125195884796,-2.47196250473654));
#86082=CARTESIAN_POINT('Ctrl Pts',(30.2240697805552,2.98598703518934,-2.55975983750062));
#86083=CARTESIAN_POINT('Ctrl Pts',(30.2181969319809,2.91061127945028,-2.64768645706356));
#86084=CARTESIAN_POINT('Ctrl Pts',(30.2123240834066,2.83144622601685,-2.73216707687537));
#86085=CARTESIAN_POINT('Ctrl Pts',(30.2064512348323,2.74885490708845,-2.81287854337434));
#86086=CARTESIAN_POINT('Ctrl Pts',(30.2048564902196,2.72642762001491,-2.83479536529685));
#86087=CARTESIAN_POINT('Ctrl Pts',(30.2032617456069,2.70374787330462,-2.85643449597814));
#86088=CARTESIAN_POINT('Ctrl Pts',(30.2016670009942,2.68082332935361,-2.87778999873053));
#86089=CARTESIAN_POINT('Ctrl Pts',(30.1957945548603,2.59640658423568,-2.95642894729872));
#86090=CARTESIAN_POINT('Ctrl Pts',(30.1899221087264,2.50838539502564,-3.03148199994583));
#86091=CARTESIAN_POINT('Ctrl Pts',(30.1840496625925,2.41709711703613,-3.10260060704172));
#86092=CARTESIAN_POINT('Ctrl Pts',(30.1781848236476,2.3259270942293,-3.17362708682334));
#86093=CARTESIAN_POINT('Ctrl Pts',(30.1723199847028,2.23149872205837,-3.24072900487486));
#86094=CARTESIAN_POINT('Ctrl Pts',(30.1664551457579,2.13418547175362,-3.30359521917498));
#86095=CARTESIAN_POINT('Ctrl Pts',(30.1605963356379,2.03697225566015,-3.36639680946816));
#86096=CARTESIAN_POINT('Ctrl Pts',(30.1547375255179,1.93688040518021,-3.42497113367271));
#86097=CARTESIAN_POINT('Ctrl Pts',(30.1488787153978,1.83431514541938,-3.47904828182724));
#86098=CARTESIAN_POINT('Ctrl Pts',(30.1427929265169,1.72777635944791,-3.53522045675878));
#86099=CARTESIAN_POINT('Ctrl Pts',(30.1367071376359,1.61856899968815,-3.58653967476689));
#86100=CARTESIAN_POINT('Ctrl Pts',(30.1306213487549,1.50717913659744,-3.6327537833172));
#86101=CARTESIAN_POINT('Ctrl Pts',(30.1247693186766,1.40006782498762,-3.67719278022727));
#86102=CARTESIAN_POINT('Ctrl Pts',(30.1189172885984,1.29093899691935,-3.71691144098346));
#86103=CARTESIAN_POINT('Ctrl Pts',(30.1130652585201,1.18024764312597,-3.75173353276797));
#86104=CARTESIAN_POINT('Ctrl Pts',(30.1072141181416,1.06957311803465,-3.78655033045688));
#86105=CARTESIAN_POINT('Ctrl Pts',(30.1013629777631,0.957336933753299,-3.8164719153507));
#86106=CARTESIAN_POINT('Ctrl Pts',(30.0955118373846,0.84401044232151,-3.84137154845144));
#86107=CARTESIAN_POINT('Ctrl Pts',(30.0896601698171,0.73067374014865,-3.86627342501445));
#86108=CARTESIAN_POINT('Ctrl Pts',(30.0838085022495,0.616246939290572,-3.88615236158756));
#86109=CARTESIAN_POINT('Ctrl Pts',(30.077956834682,0.501212113278957,-3.90093263431996));
#86110=CARTESIAN_POINT('Ctrl Pts',(30.0721032229978,0.386139068907821,-3.91571781754596));
#86111=CARTESIAN_POINT('Ctrl Pts',(30.0662496113135,0.27045800747624,-3.92540091597733));
#86112=CARTESIAN_POINT('Ctrl Pts',(30.0603959996292,0.154655947097649,-3.92995808349495));
#86113=CARTESIAN_POINT('Ctrl Pts',(30.0545357335293,0.0387222423464035,
-3.93452043162384));
#86114=CARTESIAN_POINT('Ctrl Pts',(30.0486754674294,-0.0773323226202726,
-3.93394520170984));
#86115=CARTESIAN_POINT('Ctrl Pts',(30.0428152013295,-0.193020802557902,
-3.92826067996765));
#86116=CARTESIAN_POINT('Ctrl Pts',(30.0369509881582,-0.308787202283246,
-3.92257232952335));
#86117=CARTESIAN_POINT('Ctrl Pts',(30.0310867749869,-0.424186615459352,
-3.91176787343508));
#86118=CARTESIAN_POINT('Ctrl Pts',(30.0252225618156,-0.538739029292221,
-3.89592726553221));
#86119=CARTESIAN_POINT('Ctrl Pts',(30.0193497132413,-0.653460128374264,
-3.88006333139114));
#86120=CARTESIAN_POINT('Ctrl Pts',(30.013476864667,-0.767331333810295,-3.85914851890151));
#86121=CARTESIAN_POINT('Ctrl Pts',(30.0076040160927,-0.879884510716179,
-3.83331348154593));
#86122=CARTESIAN_POINT('Ctrl Pts',(30.00600927148,-0.91044780044609,-3.82629809776389));
#86123=CARTESIAN_POINT('Ctrl Pts',(30.0044145268673,-0.940914001339077,
-3.81892019218749));
#86124=CARTESIAN_POINT('Ctrl Pts',(30.0028197822545,-0.971273976264554,
-3.81118300046472));
#86125=CARTESIAN_POINT('Ctrl Pts',(29.9969473361206,-1.08307075924357,-3.78269176666031));
#86126=CARTESIAN_POINT('Ctrl Pts',(29.9910748899867,-1.19380001443587,-3.74922951171389));
#86127=CARTESIAN_POINT('Ctrl Pts',(29.9852024438528,-1.30298612731375,-3.71089155756779));
#86128=CARTESIAN_POINT('Ctrl Pts',(29.979337604908,-1.41203080008544,-3.67260326655341));
#86129=CARTESIAN_POINT('Ctrl Pts',(29.9734727659631,-1.51953591940979,-3.62945197229674));
#86130=CARTESIAN_POINT('Ctrl Pts',(29.9676079270183,-1.62503781012665,-3.58158360444913));
#86131=CARTESIAN_POINT('Ctrl Pts',(29.9617491168983,-1.73043124903029,-3.5337644434096));
#86132=CARTESIAN_POINT('Ctrl Pts',(29.9558903067783,-1.83382518110547,-3.48123802340571));
#86133=CARTESIAN_POINT('Ctrl Pts',(29.9500314966583,-1.93477344632288,-3.42419928032874));
#86134=CARTESIAN_POINT('Ctrl Pts',(29.9439457077773,-2.03963259304888,-3.36495077401223));
#86135=CARTESIAN_POINT('Ctrl Pts',(29.9378599188964,-2.14185231432237,-3.30083339613807));
#86136=CARTESIAN_POINT('Ctrl Pts',(29.9317741300154,-2.24095767391047,-3.23211969205068));
#86137=CARTESIAN_POINT('Ctrl Pts',(29.9259220999371,-2.33625633716823,-3.16604532256921));
#86138=CARTESIAN_POINT('Ctrl Pts',(29.9200700698589,-2.42867510338249,-3.0957214661676));
#86139=CARTESIAN_POINT('Ctrl Pts',(29.9142180397806,-2.51781970578769,-3.02143557421753));
#86140=CARTESIAN_POINT('Ctrl Pts',(29.9083668994021,-2.60695075530109,-2.94716097614985));
#86141=CARTESIAN_POINT('Ctrl Pts',(29.9025157590236,-2.69280831328885,-2.8689258047693));
#86142=CARTESIAN_POINT('Ctrl Pts',(29.8966646186451,-2.77503090090207,-2.78705803653936));
#86143=CARTESIAN_POINT('Ctrl Pts',(29.8908129510777,-2.85726089678748,-2.70518289200653));
#86144=CARTESIAN_POINT('Ctrl Pts',(29.8849612835102,-2.93585497829912,-2.61967479165901));
#86145=CARTESIAN_POINT('Ctrl Pts',(29.8791096159427,-3.01048878376404,-2.53089831538743));
#86146=CARTESIAN_POINT('Ctrl Pts',(29.8732560042585,-3.08514738503834,-2.44209234464522));
#86147=CARTESIAN_POINT('Ctrl Pts',(29.8674023925742,-3.15584282815298,-2.35001615504212));
#86148=CARTESIAN_POINT('Ctrl Pts',(29.86154878089,-3.22229171785936,-2.25506653671571));
#86149=CARTESIAN_POINT('Ctrl Pts',(29.8556885147901,-3.28881614700269,-2.16000897917859));
#86150=CARTESIAN_POINT('Ctrl Pts',(29.8498282486902,-3.35108415005529,-2.06207181189839));
#86151=CARTESIAN_POINT('Ctrl Pts',(29.8439679825904,-3.40885622535348,-1.96167995220138));
#86152=CARTESIAN_POINT('Ctrl Pts',(29.8381037694191,-3.46666721194057,-1.8612204754656));
#86153=CARTESIAN_POINT('Ctrl Pts',(29.8322395562478,-3.51997605146945,-1.75830338037986));
#86154=CARTESIAN_POINT('Ctrl Pts',(29.8263753430765,-3.56859045398145,-1.65337568983956));
#86155=CARTESIAN_POINT('Ctrl Pts',(29.8205024945022,-3.61727644409519,-1.54829348702854));
#86156=CARTESIAN_POINT('Ctrl Pts',(29.8146296459279,-3.66125404412129,-1.44119516068858));
#86157=CARTESIAN_POINT('Ctrl Pts',(29.8087567973536,-3.70038003560882,-1.33254515573307));
#86158=CARTESIAN_POINT('Ctrl Pts',(29.8071620527407,-3.71100451593692,-1.30304175412173));
#86159=CARTESIAN_POINT('Ctrl Pts',(29.8055673081279,-3.72127154277174,-1.2734240052593));
#86160=CARTESIAN_POINT('Ctrl Pts',(29.803972563515,-3.73117889742914,-1.2437013449295));
#86161=CARTESIAN_POINT('Ctrl Pts',(29.7969890545378,-3.77456396337151,-1.11354353560678));
#86162=CARTESIAN_POINT('Ctrl Pts',(29.7900055455606,-3.8111662578302,-0.981018558808337));
#86163=CARTESIAN_POINT('Ctrl Pts',(29.7830220365834,-3.84076258079052,-0.846777301301432));
#86164=CARTESIAN_POINT('Ctrl Pts',(29.7758456247582,-3.87117643187473,-0.708827947908951));
#86165=CARTESIAN_POINT('Ctrl Pts',(29.7686692129329,-3.89419154278163,-0.569066121117047));
#86166=CARTESIAN_POINT('Ctrl Pts',(29.7614928011076,-3.90961824669457,-0.428222097880171));
#86167=CARTESIAN_POINT('Ctrl Pts',(29.7543163892823,-3.9250449506075,-0.287378074643332));
#86168=CARTESIAN_POINT('Ctrl Pts',(29.747139977457,-3.93288305006062,-0.145451907656713));
#86169=CARTESIAN_POINT('Ctrl Pts',(29.7399635656318,-3.93299870026503,-0.00319745422851603));
#86170=CARTESIAN_POINT('',(28.489963522035,-3.92772619981674,0.00219722477549311));
#86171=CARTESIAN_POINT('Ctrl Pts',(29.739963522035,-3.92968187761009,-0.00319389424515149));
#86172=CARTESIAN_POINT('Ctrl Pts',(29.6950174629484,-3.92291879964284,0.887004282061398));
#86173=CARTESIAN_POINT('Ctrl Pts',(29.5837889976154,-3.18166436252796,3.10018088548878));
#86174=CARTESIAN_POINT('Ctrl Pts',(29.4062781260356,0.494417430209507,4.62531527855905));
#86175=CARTESIAN_POINT('Ctrl Pts',(29.2074309072962,4.15819300996308,2.08504698106617));
#86176=CARTESIAN_POINT('Ctrl Pts',(29.0085836885562,4.00233764393561,-2.37050277479532));
#86177=CARTESIAN_POINT('Ctrl Pts',(28.8097364698168,0.170016879685549,-4.64855722584818));
#86178=CARTESIAN_POINT('Ctrl Pts',(28.6368630809762,-3.29749257198293,-2.91674327551318));
#86179=CARTESIAN_POINT('Ctrl Pts',(28.5302720983823,-3.92368339933592,-0.797150168107896));
#86180=CARTESIAN_POINT('Ctrl Pts',(28.489963522035,-3.92772619981674,0.00219722477549311));
#86181=CARTESIAN_POINT('',(27.239963522035,-3.93773669167115,0.00235620308681454));
#86182=CARTESIAN_POINT('Ctrl Pts',(28.489963522035,-3.92772619981674,0.00219722477549311));
#86183=CARTESIAN_POINT('Ctrl Pts',(28.4639896921358,-3.93033127847545,0.51727652289259));
#86184=CARTESIAN_POINT('Ctrl Pts',(28.3717334559901,-3.59630940642058,2.34353714429184));
#86185=CARTESIAN_POINT('Ctrl Pts',(28.2131948135979,-0.830978145420823,
4.57684010461503));
#86186=CARTESIAN_POINT('Ctrl Pts',(28.0143475948581,3.4007603027884,3.17377053114104));
#86187=CARTESIAN_POINT('Ctrl Pts',(27.8155003761186,4.50862997901059,-1.14465965847099));
#86188=CARTESIAN_POINT('Ctrl Pts',(27.6166531573788,1.474964486074,-4.41162892661981));
#86189=CARTESIAN_POINT('Ctrl Pts',(27.4248075393512,-2.759048571294,-3.6538230993727));
#86190=CARTESIAN_POINT('Ctrl Pts',(27.2992443275697,-3.92947964173005,-1.16559882579688));
#86191=CARTESIAN_POINT('Ctrl Pts',(27.239963522035,-3.93773669167115,0.00235620308681454));
#86192=CARTESIAN_POINT('',(25.989963522035,-3.93325007891365,-0.00337094196644616));
#86193=CARTESIAN_POINT('Ctrl Pts',(27.239963522035,-3.93773669167115,0.00235620308681454));
#86194=CARTESIAN_POINT('Ctrl Pts',(27.2329619213232,-3.93871192414688,0.140302283404259));
#86195=CARTESIAN_POINT('Ctrl Pts',(27.1596779143649,-3.86944318367108,1.5831590277253));
#86196=CARTESIAN_POINT('Ctrl Pts',(27.0201115011599,-2.08882077843383,4.15629856686949));
#86197=CARTESIAN_POINT('Ctrl Pts',(26.8212642824203,2.36686862149651,4.004487851141));
#86198=CARTESIAN_POINT('Ctrl Pts',(26.6224170636807,4.64840097541825,0.174236600890457));
#86199=CARTESIAN_POINT('Ctrl Pts',(26.423569844941,2.66000738516909,-3.81606482285398));
#86200=CARTESIAN_POINT('Ctrl Pts',(26.2247226262013,-1.77181451638399,-4.30100724724962));
#86201=CARTESIAN_POINT('Ctrl Pts',(26.0801871852327,-3.81014481169265,-1.78177796532842));
#86202=CARTESIAN_POINT('Ctrl Pts',(26.0019341505106,-3.9372342010039,-0.239632457677508));
#86203=CARTESIAN_POINT('Ctrl Pts',(25.989963522035,-3.93508678583485,-0.00337251609275779));
#86204=CARTESIAN_POINT('',(24.7399635445061,-3.9306001245949,-0.000718677470833023));
#86205=CARTESIAN_POINT('Ctrl Pts',(25.989963522035,-3.93299855558116,-0.00337072640157237));
#86206=CARTESIAN_POINT('Ctrl Pts',(25.9841875105398,-3.93309620432813,0.110566845214765));
#86207=CARTESIAN_POINT('Ctrl Pts',(25.9784114990446,-3.92823857947925,0.224676345046821));
#86208=CARTESIAN_POINT('Ctrl Pts',(25.9726354875494,-3.9184075443469,0.338483849548717));
#86209=CARTESIAN_POINT('Ctrl Pts',(25.9665685167649,-3.90808128322736,0.458024263455157));
#86210=CARTESIAN_POINT('Ctrl Pts',(25.9605015459804,-3.89226740998787,0.577230993667277));
#86211=CARTESIAN_POINT('Ctrl Pts',(25.9544345751959,-3.87100689880111,0.695553441105879));
#86212=CARTESIAN_POINT('Ctrl Pts',(25.9486676611254,-3.85079787761639,0.808023965728239));
#86213=CARTESIAN_POINT('Ctrl Pts',(25.9429007470548,-3.82566814695001,0.919695102139139));
#86214=CARTESIAN_POINT('Ctrl Pts',(25.9371338329842,-3.79570600900335,1.03009945792426));
#86215=CARTESIAN_POINT('Ctrl Pts',(25.9313685509217,-3.76575235019257,1.14047256982631));
#86216=CARTESIAN_POINT('Ctrl Pts',(25.9256032688591,-3.73096911289362,1.24957920184213));
#86217=CARTESIAN_POINT('Ctrl Pts',(25.9198379867965,-3.69149527863074,1.35696411442859));
#86218=CARTESIAN_POINT('Ctrl Pts',(25.9140728441454,-3.65202239889297,1.46434643031783));
#86219=CARTESIAN_POINT('Ctrl Pts',(25.9083077014943,-3.60785929551641,1.5700067091801));
#86220=CARTESIAN_POINT('Ctrl Pts',(25.9025425588432,-3.55919389605387,1.67350763675965));
#86221=CARTESIAN_POINT('Ctrl Pts',(25.8967760633438,-3.51051707676943,1.7770328518653));
#86222=CARTESIAN_POINT('Ctrl Pts',(25.8910095678444,-3.45733604460149,1.87839732321322));
#86223=CARTESIAN_POINT('Ctrl Pts',(25.8852430723451,-3.39988526660132,1.97718718738192));
#86224=CARTESIAN_POINT('Ctrl Pts',(25.8794704699136,-3.34237364610159,2.07608167367198));
#86225=CARTESIAN_POINT('Ctrl Pts',(25.8736978674821,-3.28058347096434,2.17239574252534));
#86226=CARTESIAN_POINT('Ctrl Pts',(25.8679252650506,-3.21479318612327,2.2657435358962));
#86227=CARTESIAN_POINT('Ctrl Pts',(25.8621491040677,-3.14896234451134,2.35914887401055));
#86228=CARTESIAN_POINT('Ctrl Pts',(25.8563729430848,-3.0791267473614,2.44958396172238));
#86229=CARTESIAN_POINT('Ctrl Pts',(25.8505967821018,-3.0056046509437,2.53669660823395));
#86230=CARTESIAN_POINT('Ctrl Pts',(25.8448120833999,-2.93197388182711,2.62393801557886));
#86231=CARTESIAN_POINT('Ctrl Pts',(25.8390273846979,-2.85464602973347,2.70784687121573));
#86232=CARTESIAN_POINT('Ctrl Pts',(25.8332426859959,-2.77397558729295,2.78810839837742));
#86233=CARTESIAN_POINT('Ctrl Pts',(25.8311711869046,-2.74508752296738,2.81685003024867));
#86234=CARTESIAN_POINT('Ctrl Pts',(25.8290996878134,-2.71577112039666,2.84512432816432));
#86235=CARTESIAN_POINT('Ctrl Pts',(25.8270281887221,-2.6860436152956,2.87291815002268));
#86236=CARTESIAN_POINT('Ctrl Pts',(25.8211557425882,-2.60176978040093,2.95171022982959));
#86237=CARTESIAN_POINT('Ctrl Pts',(25.8152832964543,-2.5138849970653,3.02692296358918));
#86238=CARTESIAN_POINT('Ctrl Pts',(25.8094108503204,-2.42272598724428,3.09820718976818));
#86239=CARTESIAN_POINT('Ctrl Pts',(25.8035460113756,-2.33168506515144,3.16939907408935));
#86240=CARTESIAN_POINT('Ctrl Pts',(25.7976811724307,-2.23737867391849,3.23667231876815));
#86241=CARTESIAN_POINT('Ctrl Pts',(25.7918163334859,-2.14017971927364,3.29971510424912));
#86242=CARTESIAN_POINT('Ctrl Pts',(25.7859575233659,-2.0430806813487,3.36269308421483));
#86243=CARTESIAN_POINT('Ctrl Pts',(25.7800987132459,-1.9430953390677,3.4214490312959));
#86244=CARTESIAN_POINT('Ctrl Pts',(25.7742399031258,-1.84062842683969,3.47571230027884));
#86245=CARTESIAN_POINT('Ctrl Pts',(25.7681541142449,-1.73419179852608,3.53207780662852));
#86246=CARTESIAN_POINT('Ctrl Pts',(25.7620683253639,-1.62507779015006,3.58359520891931));
#86247=CARTESIAN_POINT('Ctrl Pts',(25.7559825364829,-1.51377201357829,3.63001147255861));
#86248=CARTESIAN_POINT('Ctrl Pts',(25.7501305064047,-1.40674155867399,3.67464485965931));
#86249=CARTESIAN_POINT('Ctrl Pts',(25.7442784763264,-1.29768502074069,3.71456158124025));
#86250=CARTESIAN_POINT('Ctrl Pts',(25.7384264462481,-1.1870570698065,3.74958457872634));
#86251=CARTESIAN_POINT('Ctrl Pts',(25.7325753058696,-1.07644593793511,3.78460225157261));
#86252=CARTESIAN_POINT('Ctrl Pts',(25.7267241654911,-0.964264262058645,
3.81472755492515));
#86253=CARTESIAN_POINT('Ctrl Pts',(25.7208730251126,-0.85098316334188,3.83983289424275));
#86254=CARTESIAN_POINT('Ctrl Pts',(25.7150213575452,-0.737691857974338,
3.86494049555669));
#86255=CARTESIAN_POINT('Ctrl Pts',(25.7091696899777,-0.623301336437284,
3.88502714426204));
#86256=CARTESIAN_POINT('Ctrl Pts',(25.7033180224102,-0.508293533989227,
3.90001624141551));
#86257=CARTESIAN_POINT('Ctrl Pts',(25.697464410726,-0.393247522160508,3.91501031844083));
#86258=CARTESIAN_POINT('Ctrl Pts',(25.6916107990418,-0.277584231303043,
3.92490342295136));
#86259=CARTESIAN_POINT('Ctrl Pts',(25.6857571873576,-0.161790635434357,
3.92967082467295));
#86260=CARTESIAN_POINT('Ctrl Pts',(25.6798969212577,-0.045865404814469,
3.93444364600116));
#86261=CARTESIAN_POINT('Ctrl Pts',(25.6740366551578,0.0701900132309724,
3.93407911717854));
#86262=CARTESIAN_POINT('Ctrl Pts',(25.6681763890579,0.185888622905629,3.92860464031114));
#86263=CARTESIAN_POINT('Ctrl Pts',(25.6623121758866,0.301665159191289,3.92312647621336));
#86264=CARTESIAN_POINT('Ctrl Pts',(25.6564479627153,0.417083997958116,3.91253154862948));
#86265=CARTESIAN_POINT('Ctrl Pts',(25.650583749544,0.531664982044918,3.89689893978111));
#86266=CARTESIAN_POINT('Ctrl Pts',(25.6447109009698,0.64641469345154,3.88124331098565));
#86267=CARTESIAN_POINT('Ctrl Pts',(25.6388380523955,0.760323682616542,3.8605352691614));
#86268=CARTESIAN_POINT('Ctrl Pts',(25.6329652038212,0.872923578222459,3.83490461766434));
#86269=CARTESIAN_POINT('Ctrl Pts',(25.6313704592083,0.903499554200888,3.82794473390718));
#86270=CARTESIAN_POINT('Ctrl Pts',(25.6297757145954,0.933979099670331,3.82062215268567));
#86271=CARTESIAN_POINT('Ctrl Pts',(25.6281809699825,0.96435307164083,3.81294009305377));
#86272=CARTESIAN_POINT('Ctrl Pts',(25.6223085238485,1.07620139696237,3.78465187623174));
#86273=CARTESIAN_POINT('Ctrl Pts',(25.6164360777146,1.18699122127737,3.75139070833524));
#86274=CARTESIAN_POINT('Ctrl Pts',(25.6105636315807,1.29624675778246,3.7132510476587));
#86275=CARTESIAN_POINT('Ctrl Pts',(25.6046987926359,1.40536076424958,3.67516079324382));
#86276=CARTESIAN_POINT('Ctrl Pts',(25.598833953691,1.5129440487181,3.63220474850107));
#86277=CARTESIAN_POINT('Ctrl Pts',(25.5929691147462,1.61853267185289,3.58452800102674));
#86278=CARTESIAN_POINT('Ctrl Pts',(25.5871103046262,1.72401275401673,3.53690026338234));
#86279=CARTESIAN_POINT('Ctrl Pts',(25.5812514945062,1.82750187880104,3.48456164437377));
#86280=CARTESIAN_POINT('Ctrl Pts',(25.5753926843862,1.92855353300051,3.42770626955567));
#86281=CARTESIAN_POINT('Ctrl Pts',(25.5693068955052,2.03352007414724,3.36864823544891));
#86282=CARTESIAN_POINT('Ctrl Pts',(25.5632211066242,2.13585603375695,3.30471654586177));
#86283=CARTESIAN_POINT('Ctrl Pts',(25.5571353177433,2.23508598156619,3.23618288343016));
#86284=CARTESIAN_POINT('Ctrl Pts',(25.551283287665,2.33050444753691,3.17028164009632));
#86285=CARTESIAN_POINT('Ctrl Pts',(25.5454312575867,2.42305073626668,3.10012568831626));
#86286=CARTESIAN_POINT('Ctrl Pts',(25.5395792275085,2.51233005976414,3.02600176318612));
#86287=CARTESIAN_POINT('Ctrl Pts',(25.5337280871299,2.60159580988775,2.95188910731417));
#86288=CARTESIAN_POINT('Ctrl Pts',(25.5278769467514,2.68759526440664,2.87380994154586));
#86289=CARTESIAN_POINT('Ctrl Pts',(25.5220258063729,2.76996634961764,2.79209158552974));
#86290=CARTESIAN_POINT('Ctrl Pts',(25.5161741388054,2.85234485648086,2.71036586667242));
#86291=CARTESIAN_POINT('Ctrl Pts',(25.5103224712379,2.93109405069021,2.62500059688869));
#86292=CARTESIAN_POINT('Ctrl Pts',(25.5044708036704,3.00588890920285,2.53635976658109));
#86293=CARTESIAN_POINT('Ctrl Pts',(25.4986171919862,3.08070861703143,2.44768948686959));
#86294=CARTESIAN_POINT('Ctrl Pts',(25.4927635803019,3.15157111040107,2.35574179846793));
#86295=CARTESIAN_POINT('Ctrl Pts',(25.4869099686177,3.21819227414718,2.26091297634814));
#86296=CARTESIAN_POINT('Ctrl Pts',(25.4810497025178,3.28488917317232,2.1659763523393));
#86297=CARTESIAN_POINT('Ctrl Pts',(25.4751894364179,3.34733488112954,2.06815239567862));
#86298=CARTESIAN_POINT('Ctrl Pts',(25.469329170318,3.40528912530119,1.96786558817046));
#86299=CARTESIAN_POINT('Ctrl Pts',(25.4634649571468,3.46328240345805,1.8675112343796));
#86300=CARTESIAN_POINT('Ctrl Pts',(25.4576007439755,3.51677800384791,1.76469109252163));
#86301=CARTESIAN_POINT('Ctrl Pts',(25.4517365308042,3.56558282524708,1.6598518356477));
#86302=CARTESIAN_POINT('Ctrl Pts',(25.4458636822299,3.6144595146511,1.55485819672696));
#86303=CARTESIAN_POINT('Ctrl Pts',(25.4399908336556,3.65863148205304,1.44783988939282));
#86304=CARTESIAN_POINT('Ctrl Pts',(25.4341179850813,3.69795466602593,1.33926109777634));
#86305=CARTESIAN_POINT('Ctrl Pts',(25.4325232404685,3.70863269305282,1.30977703381479));
#86306=CARTESIAN_POINT('Ctrl Pts',(25.4309284958556,3.718953474776,1.28017797382429));
#86307=CARTESIAN_POINT('Ctrl Pts',(25.4293337512428,3.7289147753841,1.25047334954495));
#86308=CARTESIAN_POINT('Ctrl Pts',(25.4234613051088,3.76559600996759,1.14108981276867));
#86309=CARTESIAN_POINT('Ctrl Pts',(25.4175888589749,3.79752161144521,1.02990777090968));
#86310=CARTESIAN_POINT('Ctrl Pts',(25.411716412841,3.82451377617999,0.917378534635202));
#86311=CARTESIAN_POINT('Ctrl Pts',(25.4058515738961,3.85147097516186,0.804995069161654));
#86312=CARTESIAN_POINT('Ctrl Pts',(25.3999867349513,3.87350735088755,0.691268278026297));
#86313=CARTESIAN_POINT('Ctrl Pts',(25.3941218960064,3.89049409558753,0.576666881482352));
#86314=CARTESIAN_POINT('Ctrl Pts',(25.3882630858864,3.90746337857897,0.462183290687546));
#86315=CARTESIAN_POINT('Ctrl Pts',(25.3824042757664,3.91939329513246,0.346827289198799));
#86316=CARTESIAN_POINT('Ctrl Pts',(25.3765454656464,3.92620571113299,0.231079453579754));
#86317=CARTESIAN_POINT('Ctrl Pts',(25.3704596767654,3.93328204996276,0.110847379732617));
#86318=CARTESIAN_POINT('Ctrl Pts',(25.3643738878845,3.9348362439859,-0.00980706089680983));
#86319=CARTESIAN_POINT('Ctrl Pts',(25.3582880990035,3.93083976504607,-0.130337030549801));
#86320=CARTESIAN_POINT('Ctrl Pts',(25.3524360689252,3.92699679326041,-0.246237371744446));
#86321=CARTESIAN_POINT('Ctrl Pts',(25.3465840388469,3.91802170715974,-0.362022176262712));
#86322=CARTESIAN_POINT('Ctrl Pts',(25.3407320087687,3.90394224495369,-0.477204304324647));
#86323=CARTESIAN_POINT('Ctrl Pts',(25.3348808683901,3.88986492328586,-0.592368920940156));
#86324=CARTESIAN_POINT('Ctrl Pts',(25.3290297280116,3.87068481865748,-0.706930633091622));
#86325=CARTESIAN_POINT('Ctrl Pts',(25.3231785876331,3.84648149831601,-0.820407876066914));
#86326=CARTESIAN_POINT('Ctrl Pts',(25.3173269200656,3.8222759972503,-0.933895343365568));
#86327=CARTESIAN_POINT('Ctrl Pts',(25.3114752524981,3.79304646698865,-1.04629774295961));
#86328=CARTESIAN_POINT('Ctrl Pts',(25.3056235849306,3.7589233562151,-1.15714484923049));
#86329=CARTESIAN_POINT('Ctrl Pts',(25.2997699732464,3.72478890861983,-1.26802878256231));
#86330=CARTESIAN_POINT('Ctrl Pts',(25.2939163615621,3.68575776924242,-1.37735600025294));
#86331=CARTESIAN_POINT('Ctrl Pts',(25.2880627498779,3.6420096641432,-1.48467323215835));
#86332=CARTESIAN_POINT('Ctrl Pts',(25.282202483778,3.59821182597481,-1.59211246284075));
#86333=CARTESIAN_POINT('Ctrl Pts',(25.2763422176781,3.54968647530237,-1.69753676402993));
#86334=CARTESIAN_POINT('Ctrl Pts',(25.2704819515782,3.49666077208495,-1.80051449451602));
#86335=CARTESIAN_POINT('Ctrl Pts',(25.2646177384068,3.44359935440785,-1.90356158370516));
#86336=CARTESIAN_POINT('Ctrl Pts',(25.2587535252355,3.38603175340706,-2.00415846311935));
#86337=CARTESIAN_POINT('Ctrl Pts',(25.2528893120642,3.32422930262604,-2.10190117359557));
#86338=CARTESIAN_POINT('Ctrl Pts',(25.2470164634899,3.26233584405733,-2.19978781603129));
#86339=CARTESIAN_POINT('Ctrl Pts',(25.2411436149156,3.19619532501196,-2.29481156332244));
#86340=CARTESIAN_POINT('Ctrl Pts',(25.2352707663413,3.12612032583015,-2.38660024059992));
#86341=CARTESIAN_POINT('Ctrl Pts',(25.2336760217286,3.1070917869502,-2.4115250273956));
#86342=CARTESIAN_POINT('Ctrl Pts',(25.2320812771159,3.08777334619203,-2.43621147578762));
#86343=CARTESIAN_POINT('Ctrl Pts',(25.2304865325032,3.06817172869338,-2.46065260515309));
#86344=CARTESIAN_POINT('Ctrl Pts',(25.2246140863693,2.99599124162355,-2.55065398500134));
#86345=CARTESIAN_POINT('Ctrl Pts',(25.2187416402353,2.91972641653179,-2.63762735400208));
#86346=CARTESIAN_POINT('Ctrl Pts',(25.2128691941014,2.83966075972733,-2.72117911385208));
#86347=CARTESIAN_POINT('Ctrl Pts',(25.2070043551566,2.75969882027951,-2.80462264043429));
#86348=CARTESIAN_POINT('Ctrl Pts',(25.2011395162117,2.67594612379049,-2.88465307656847));
#86349=CARTESIAN_POINT('Ctrl Pts',(25.1952746772669,2.58872731423561,-2.96090862617043));
#86350=CARTESIAN_POINT('Ctrl Pts',(25.1894158671469,2.50159816220215,-3.03708578805298));
#86351=CARTESIAN_POINT('Ctrl Pts',(25.1835570570268,2.41101029348404,-3.10949551136133));
#86352=CARTESIAN_POINT('Ctrl Pts',(25.1776982469068,2.31732572545454,-3.17781221631276));
#86353=CARTESIAN_POINT('Ctrl Pts',(25.1716124580258,2.22001168203069,-3.24877560902566));
#86354=CARTESIAN_POINT('Ctrl Pts',(25.1655266691449,2.11935645966524,-3.31532210234597));
#86355=CARTESIAN_POINT('Ctrl Pts',(25.1594408802639,2.01580463768916,-3.37713201735894));
#86356=CARTESIAN_POINT('Ctrl Pts',(25.1535888501856,1.91623030333138,-3.43656777644727));
#86357=CARTESIAN_POINT('Ctrl Pts',(25.1477368201074,1.8139781726968,-3.49162388336151));
#86358=CARTESIAN_POINT('Ctrl Pts',(25.1418847900291,1.70947303044468,-3.54206027026394));
#86359=CARTESIAN_POINT('Ctrl Pts',(25.1360336496506,1.60498377638853,-3.59248898918773));
#86360=CARTESIAN_POINT('Ctrl Pts',(25.1301825092721,1.4982425639467,-3.63829920498125));
#86361=CARTESIAN_POINT('Ctrl Pts',(25.1243313688935,1.38969751247317,-3.67929746335165));
#86362=CARTESIAN_POINT('Ctrl Pts',(25.118479701326,1.28114268106726,-3.7202994156739));
#86363=CARTESIAN_POINT('Ctrl Pts',(25.1126280337585,1.17078407425861,-3.7564884026335));
#86364=CARTESIAN_POINT('Ctrl Pts',(25.106776366191,1.05908778496831,-3.78771990301961));
#86365=CARTESIAN_POINT('Ctrl Pts',(25.1009227545068,0.947354386491927,-3.81896177953878));
#86366=CARTESIAN_POINT('Ctrl Pts',(25.0950691428226,0.83428281970488,-3.8452427831944));
#86367=CARTESIAN_POINT('Ctrl Pts',(25.0892155311384,0.720351559213901,-3.86646901334255));
#86368=CARTESIAN_POINT('Ctrl Pts',(25.0833552650385,0.606290781083612,-3.88771937357763));
#86369=CARTESIAN_POINT('Ctrl Pts',(25.0774949989386,0.491368765187452,-3.90390341514437));
#86370=CARTESIAN_POINT('Ctrl Pts',(25.0716347328387,0.376071439674704,-3.91497883420345));
#86371=CARTESIAN_POINT('Ctrl Pts',(25.0657705196674,0.260696457828296,-3.92606171290163));
#86372=CARTESIAN_POINT('Ctrl Pts',(25.0599063064961,0.14494607482321,-3.93202909650567));
#86373=CARTESIAN_POINT('Ctrl Pts',(25.0540420933247,0.0293068175335294,
-3.93289080835536));
#86374=CARTESIAN_POINT('Ctrl Pts',(25.0481692447504,-0.086502725446165,
-3.93375378912704));
#86375=CARTESIAN_POINT('Ctrl Pts',(25.0422963961761,-0.202200404596252,
-3.92949610804844));
#86376=CARTESIAN_POINT('Ctrl Pts',(25.0364235476018,-0.317304127708729,
-3.92017947172563));
#86377=CARTESIAN_POINT('Ctrl Pts',(25.0348288029891,-0.348560006354695,
-3.91764958262716));
#86378=CARTESIAN_POINT('Ctrl Pts',(25.0332340583763,-0.379772145524845,
-3.91474695346925));
#86379=CARTESIAN_POINT('Ctrl Pts',(25.0316393137635,-0.410931036706119,
-3.9114734670034));
#86380=CARTESIAN_POINT('Ctrl Pts',(25.0257668676296,-0.525669728147831,
-3.89941926548007));
#86381=CARTESIAN_POINT('Ctrl Pts',(25.0198944214957,-0.640069673261343,
-3.88229200593471));
#86382=CARTESIAN_POINT('Ctrl Pts',(25.0140219753618,-0.753646478881124,
-3.86011735376919));
#86383=CARTESIAN_POINT('Ctrl Pts',(25.008157136417,-0.867076156674893,-3.83797142673244));
#86384=CARTESIAN_POINT('Ctrl Pts',(25.0022922974721,-0.979684413505547,
-3.81079118812873));
#86385=CARTESIAN_POINT('Ctrl Pts',(24.9964274585273,-1.0909913649604,-3.77865410451682));
#86386=CARTESIAN_POINT('Ctrl Pts',(24.9905686484073,-1.20218389722635,-3.74655005656884));
#86387=CARTESIAN_POINT('Ctrl Pts',(24.9847098382873,-1.31207739010615,-3.70949941270171));
#86388=CARTESIAN_POINT('Ctrl Pts',(24.9788510281673,-1.42020221648381,-3.66763066083466));
#86389=CARTESIAN_POINT('Ctrl Pts',(24.9727652392864,-1.5325159547089,-3.62413985308453));
#86390=CARTESIAN_POINT('Ctrl Pts',(24.9666794504054,-1.64292076745683,-3.57545015309787));
#86391=CARTESIAN_POINT('Ctrl Pts',(24.9605936615244,-1.75090734937847,-3.52176269130849));
#86392=CARTESIAN_POINT('Ctrl Pts',(24.9547416314462,-1.85474610189072,-3.47013739714183));
#86393=CARTESIAN_POINT('Ctrl Pts',(24.9488896013679,-1.95634856381872,-3.41389139410223));
#86394=CARTESIAN_POINT('Ctrl Pts',(24.9430375712896,-2.05528310254263,-3.35325220769371));
#86395=CARTESIAN_POINT('Ctrl Pts',(24.9371864309111,-2.15420259998476,-3.29262224042243));
#86396=CARTESIAN_POINT('Ctrl Pts',(24.9313352905326,-2.25045462838112,-3.22760063375053));
#86397=CARTESIAN_POINT('Ctrl Pts',(24.9254841501541,-2.34363414953303,-3.15845974695619));
#86398=CARTESIAN_POINT('Ctrl Pts',(24.9196324825866,-2.43682206617908,-3.08931263055365));
#86399=CARTESIAN_POINT('Ctrl Pts',(24.9137808150191,-2.52693659328818,-3.01604574255075));
#86400=CARTESIAN_POINT('Ctrl Pts',(24.9079291474517,-2.61360413711462,-2.93897302036908));
#86401=CARTESIAN_POINT('Ctrl Pts',(24.9020755357674,-2.70030047475459,-2.86187469208975));
#86402=CARTESIAN_POINT('Ctrl Pts',(24.8962219240832,-2.78354724322715,-2.78096828994615));
#86403=CARTESIAN_POINT('Ctrl Pts',(24.890368312399,-2.86300673635456,-2.69660553800299));
#86404=CARTESIAN_POINT('Ctrl Pts',(24.8845080462991,-2.94255655943915,-2.61214688205301));
#86405=CARTESIAN_POINT('Ctrl Pts',(24.8786477801992,-3.01831023017652,-2.5242243348382));
#86406=CARTESIAN_POINT('Ctrl Pts',(24.8727875140994,-3.08996941587409,-2.43322378933027));
#86407=CARTESIAN_POINT('Ctrl Pts',(24.8669233009281,-3.16167686626099,-2.34216195212588));
#86408=CARTESIAN_POINT('Ctrl Pts',(24.8610590877568,-3.22928409982488,-2.24801832354449));
#86409=CARTESIAN_POINT('Ctrl Pts',(24.8551948745856,-3.29253630998429,-2.15120748590996));
#86410=CARTESIAN_POINT('Ctrl Pts',(24.8493220260113,-3.3558816627889,-2.05425408855334));
#86411=CARTESIAN_POINT('Ctrl Pts',(24.843449177437,-3.41485898328074,-1.95462599775342));
#86412=CARTESIAN_POINT('Ctrl Pts',(24.8375763288627,-3.46925950741377,-1.85276211916672));
#86413=CARTESIAN_POINT('Ctrl Pts',(24.8359815842498,-3.484031715773,-1.82510145848849));
#86414=CARTESIAN_POINT('Ctrl Pts',(24.8343868396368,-3.49846672148907,-1.79727604748046));
#86415=CARTESIAN_POINT('Ctrl Pts',(24.8327920950239,-3.51256096699897,-1.76929490281164));
#86416=CARTESIAN_POINT('Ctrl Pts',(24.8265172351429,-3.5680177561215,-1.65919717262696));
#86417=CARTESIAN_POINT('Ctrl Pts',(24.8202423752619,-3.61836096930805,-1.54635787322841));
#86418=CARTESIAN_POINT('Ctrl Pts',(24.8139675153808,-3.66332972147213,-1.43125970801211));
#86419=CARTESIAN_POINT('Ctrl Pts',(24.8077119179017,-3.70816042972878,-1.31651486815399));
#86420=CARTESIAN_POINT('Ctrl Pts',(24.8014563204226,-3.74764945383605,-1.1995252913079));
#86421=CARTESIAN_POINT('Ctrl Pts',(24.7952007229434,-3.78158312857588,-1.08079509698659));
#86422=CARTESIAN_POINT('Ctrl Pts',(24.7889566520863,-3.81545427681164,-0.962283676023485));
#86423=CARTESIAN_POINT('Ctrl Pts',(24.7827125812291,-3.84379037820219,-0.842038338564769));
#86424=CARTESIAN_POINT('Ctrl Pts',(24.776468510372,-3.86642608699356,-0.720581927205831));
#86425=CARTESIAN_POINT('Ctrl Pts',(24.7702417352015,-3.88899909628404,-0.599461942527479));
#86426=CARTESIAN_POINT('Ctrl Pts',(24.764014960031,-3.90590313373206,-0.477137891634039));
#86427=CARTESIAN_POINT('Ctrl Pts',(24.7577881848605,-3.91702312745135,-0.354145194815961));
#86428=CARTESIAN_POINT('Ctrl Pts',(24.7518466425865,-3.92763374224968,-0.236786483841156));
#86429=CARTESIAN_POINT('Ctrl Pts',(24.7459051003125,-3.93297833254885,-0.118819332281221));
#86430=CARTESIAN_POINT('Ctrl Pts',(24.7399635580385,-3.93299993420865,-0.000719384965967845));
#86431=CARTESIAN_POINT('',(23.4899635046889,-3.93299832268712,0.00363231885978147));
#86432=CARTESIAN_POINT('Ctrl Pts',(24.739963522035,-3.92661513087914,-0.000717502642775814));
#86433=CARTESIAN_POINT('Ctrl Pts',(24.7046239734514,-3.92547634547242,0.700586071088623));
#86434=CARTESIAN_POINT('Ctrl Pts',(24.6030020186211,-3.41092723159537,2.71880545169115));
#86435=CARTESIAN_POINT('Ctrl Pts',(24.4350976575446,-0.178456178513938,
4.64824089454367));
#86436=CARTESIAN_POINT('Ctrl Pts',(24.236250438805,3.81364859256515,2.66347037411458));
#86437=CARTESIAN_POINT('Ctrl Pts',(24.0374032200652,4.30261386396493,-1.76790948834883));
#86438=CARTESIAN_POINT('Ctrl Pts',(23.8385560013257,0.839286150601286,-4.57532389878272));
#86439=CARTESIAN_POINT('Ctrl Pts',(23.6560761019823,-3.0464647852414,-3.29479500069049));
#86440=CARTESIAN_POINT('Ctrl Pts',(23.5398786088853,-3.9234348859021,-0.983222851819869));
#86441=CARTESIAN_POINT('Ctrl Pts',(23.489963522035,-3.93244535509981,0.00363146522480512));
#86442=CARTESIAN_POINT('',(22.2399631348525,-3.93532363914096,-0.000943749275237955));
#86443=CARTESIAN_POINT('Ctrl Pts',(23.4899635046889,-3.93299832268712,0.00363231885978147));
#86444=CARTESIAN_POINT('Ctrl Pts',(23.4824079195757,-3.93286034573355,0.15303085679816));
#86445=CARTESIAN_POINT('Ctrl Pts',(23.4748523344626,-3.9242063378758,0.30204887539334));
#86446=CARTESIAN_POINT('Ctrl Pts',(23.4672967493495,-3.90718678259729,0.449867142495451));
#86447=CARTESIAN_POINT('Ctrl Pts',(23.4595604189944,-3.88976008431239,0.601221528649032));
#86448=CARTESIAN_POINT('Ctrl Pts',(23.4518240886393,-3.86356278656303,0.751318393200962));
#86449=CARTESIAN_POINT('Ctrl Pts',(23.4440877582841,-3.82880428901931,0.899303461789901));
#86450=CARTESIAN_POINT('Ctrl Pts',(23.4430123601382,-3.82397264118408,0.919874308829396));
#86451=CARTESIAN_POINT('Ctrl Pts',(23.4419369619923,-3.81897564221488,0.940404384476784));
#86452=CARTESIAN_POINT('Ctrl Pts',(23.4408615638464,-3.81381392671508,0.960891425913532));
#86453=CARTESIAN_POINT('Ctrl Pts',(23.4349891177125,-3.78562725339186,1.07276538416606));
#86454=CARTESIAN_POINT('Ctrl Pts',(23.4291166715786,-3.7524666701744,1.18358535611239));
#86455=CARTESIAN_POINT('Ctrl Pts',(23.4232442254447,-3.71442620341627,1.29287546939936));
#86456=CARTESIAN_POINT('Ctrl Pts',(23.4173793864999,-3.67643501442353,1.40202400785769));
#86457=CARTESIAN_POINT('Ctrl Pts',(23.4115145475551,-3.63357664757394,1.50964624193568));
#86458=CARTESIAN_POINT('Ctrl Pts',(23.4056497086102,-3.58599576925675,1.61527810078411));
#86459=CARTESIAN_POINT('Ctrl Pts',(23.3997908984902,-3.53846380221969,1.72080137421707));
#86460=CARTESIAN_POINT('Ctrl Pts',(23.3939320883702,-3.48621914844071,1.82433796745765));
#86461=CARTESIAN_POINT('Ctrl Pts',(23.3880732782502,-3.42945552806597,1.92544119126442));
#86462=CARTESIAN_POINT('Ctrl Pts',(23.3819874893693,-3.3704928031022,2.03046129989939));
#86463=CARTESIAN_POINT('Ctrl Pts',(23.3759017004883,-3.30665403671978,2.13285525220847));
#86464=CARTESIAN_POINT('Ctrl Pts',(23.3698159116073,-3.23821047986439,2.23214737150046));
#86465=CARTESIAN_POINT('Ctrl Pts',(23.3639638815291,-3.1723958810977,2.32762562090973));
#86466=CARTESIAN_POINT('Ctrl Pts',(23.3581118514508,-3.10232396837973,2.42023555653111));
#86467=CARTESIAN_POINT('Ctrl Pts',(23.3522598213725,-3.02828111831431,2.50958213024819));
#86468=CARTESIAN_POINT('Ctrl Pts',(23.346408680994,-2.95424952518105,2.59891512036715));
#86469=CARTESIAN_POINT('Ctrl Pts',(23.3405575406155,-2.87624845876133,2.68498541688066));
#86470=CARTESIAN_POINT('Ctrl Pts',(23.334706400237,-2.79460490989147,2.76743064910587));
#86471=CARTESIAN_POINT('Ctrl Pts',(23.3288547326696,-2.71295400492076,2.84988330966375));
#86472=CARTESIAN_POINT('Ctrl Pts',(23.3230030651021,-2.62766025596515,2.92870996291517));
#86473=CARTESIAN_POINT('Ctrl Pts',(23.3171513975346,-2.53908735823309,3.00358525553394));
#86474=CARTESIAN_POINT('Ctrl Pts',(23.3112977858504,-2.45048503366638,3.07848542419168));
#86475=CARTESIAN_POINT('Ctrl Pts',(23.3054441741662,-2.35860170954444,3.14943135513341));
#86476=CARTESIAN_POINT('Ctrl Pts',(23.299590562482,-2.26383340276663,3.2161385735876));
#86477=CARTESIAN_POINT('Ctrl Pts',(23.2937302963821,-2.16895736289373,3.28292162514837));
#86478=CARTESIAN_POINT('Ctrl Pts',(23.2878700302822,-2.07119013248194,3.3454561084084));
#86479=CARTESIAN_POINT('Ctrl Pts',(23.2820097641823,-1.97095597504987,3.40350136541992));
#86480=CARTESIAN_POINT('Ctrl Pts',(23.276145551011,-1.87065430679648,3.46158571771665));
#86481=CARTESIAN_POINT('Ctrl Pts',(23.2702813378397,-1.76788276866357,3.51517463245229));
#86482=CARTESIAN_POINT('Ctrl Pts',(23.2644171246684,-1.66308785822796,3.56407460300914));
#86483=CARTESIAN_POINT('Ctrl Pts',(23.2585442760942,-1.55813863104833,3.61304658168363));
#86484=CARTESIAN_POINT('Ctrl Pts',(23.2526714275199,-1.4511604655139,3.65731567821485));
#86485=CARTESIAN_POINT('Ctrl Pts',(23.2467985789456,-1.34261741479074,3.69673740986571));
#86486=CARTESIAN_POINT('Ctrl Pts',(23.2452038343326,-1.31314305609978,3.70744219705526));
#86487=CARTESIAN_POINT('Ctrl Pts',(23.2436090897197,-1.28355337713294,3.71778984347746));
#86488=CARTESIAN_POINT('Ctrl Pts',(23.2420143451067,-1.25385780759683,3.72777810476005));
#86489=CARTESIAN_POINT('Ctrl Pts',(23.2361418989728,-1.14450761378008,3.76455861862816));
#86490=CARTESIAN_POINT('Ctrl Pts',(23.2302694528389,-1.03335459863079,3.79658513396738));
#86491=CARTESIAN_POINT('Ctrl Pts',(23.224397006705,-0.920849911226558,3.82367943753056));
#86492=CARTESIAN_POINT('Ctrl Pts',(23.2185321677601,-0.808490962822574,
3.85073864302979));
#86493=CARTESIAN_POINT('Ctrl Pts',(23.2126673288153,-0.694784222365801,
3.87287824672256));
#86494=CARTESIAN_POINT('Ctrl Pts',(23.2068024898704,-0.58019829298932,3.88996901540517));
#86495=CARTESIAN_POINT('Ctrl Pts',(23.2009436797504,-0.465730153462115,
3.9070422154467));
#86496=CARTESIAN_POINT('Ctrl Pts',(23.1950848696304,-0.350385029046763,
3.91907684306931));
#86497=CARTESIAN_POINT('Ctrl Pts',(23.1892260595104,-0.234643425181591,
3.92599432794025));
#86498=CARTESIAN_POINT('Ctrl Pts',(23.1831402706294,-0.114417824515235,
3.93317980616016));
#86499=CARTESIAN_POINT('Ctrl Pts',(23.1770544817485,0.00623515556169527,
3.93484352525785));
#86500=CARTESIAN_POINT('Ctrl Pts',(23.1709686928675,0.126768703412605,3.93095646068932));
#86501=CARTESIAN_POINT('Ctrl Pts',(23.1651166627892,0.242672485364009,3.92721870060331));
#86502=CARTESIAN_POINT('Ctrl Pts',(23.159264632711,0.358465389433446,3.91834872343684));
#86503=CARTESIAN_POINT('Ctrl Pts',(23.1534126026327,0.473660250861932,3.90437382518035));
#86504=CARTESIAN_POINT('Ctrl Pts',(23.1475614622542,0.588837598908159,3.89040105156493));
#86505=CARTESIAN_POINT('Ctrl Pts',(23.1417103218757,0.703416674859619,3.87132494979667));
#86506=CARTESIAN_POINT('Ctrl Pts',(23.1358591814972,0.816915841974344,3.8472246499433));
#86507=CARTESIAN_POINT('Ctrl Pts',(23.1300075139297,0.930425235387965,3.82312217864783));
#86508=CARTESIAN_POINT('Ctrl Pts',(23.1241558463622,1.0428541221751,3.7939946952414));
#86509=CARTESIAN_POINT('Ctrl Pts',(23.1183041787948,1.15373215849437,3.75997222150057));
#86510=CARTESIAN_POINT('Ctrl Pts',(23.1124505671105,1.26464703215,3.72593844437315));
#86511=CARTESIAN_POINT('Ctrl Pts',(23.1065969554263,1.37400963584463,3.68700656435129));
#86512=CARTESIAN_POINT('Ctrl Pts',(23.1007433437421,1.48136653647223,3.64335589595915));
#86513=CARTESIAN_POINT('Ctrl Pts',(23.0948830776422,1.58884548097268,3.59965560526427));
#86514=CARTESIAN_POINT('Ctrl Pts',(23.0890228115423,1.6943137882741,3.55122597493344));
#86515=CARTESIAN_POINT('Ctrl Pts',(23.0831625454425,1.79733961113691,3.49829377300395));
#86516=CARTESIAN_POINT('Ctrl Pts',(23.0772983322712,1.90043482509449,3.4453259195908));
#86517=CARTESIAN_POINT('Ctrl Pts',(23.0714341190999,2.00108392083609,3.38784966049926));
#86518=CARTESIAN_POINT('Ctrl Pts',(23.0655699059286,2.09888269305838,3.32613596246155));
#86519=CARTESIAN_POINT('Ctrl Pts',(23.0596970573543,2.19682547979467,3.2643313873297));
#86520=CARTESIAN_POINT('Ctrl Pts',(23.05382420878,2.29190922789305,3.19827715463894));
#86521=CARTESIAN_POINT('Ctrl Pts',(23.0479513602057,2.38376147888872,3.12828550675386));
#86522=CARTESIAN_POINT('Ctrl Pts',(23.0463566155929,2.40870352883323,3.10927960152754));
#86523=CARTESIAN_POINT('Ctrl Pts',(23.04476187098,2.43340750363462,3.08998357818745));
#86524=CARTESIAN_POINT('Ctrl Pts',(23.0431671263671,2.45786641656803,3.07040415553181));
#86525=CARTESIAN_POINT('Ctrl Pts',(23.0372946802332,2.54793328215618,2.99830539818229));
#86526=CARTESIAN_POINT('Ctrl Pts',(23.0314222340993,2.63497584575797,2.9221195557755));
#86527=CARTESIAN_POINT('Ctrl Pts',(23.0255497879654,2.71860025187564,2.84212977720964));
#86528=CARTESIAN_POINT('Ctrl Pts',(23.0196849490205,2.80211633061937,2.76224361770735));
#86529=CARTESIAN_POINT('Ctrl Pts',(23.0138201100757,2.88222276143276,2.67856360444628));
#86530=CARTESIAN_POINT('Ctrl Pts',(23.0079552711308,2.95855745368066,2.59141405284269));
#86531=CARTESIAN_POINT('Ctrl Pts',(23.0020964610108,3.03481367685349,2.5043540875662));
#86532=CARTESIAN_POINT('Ctrl Pts',(22.9962376508908,3.10730560270164,2.41383198708636));
#86533=CARTESIAN_POINT('Ctrl Pts',(22.9903788407708,3.17570732295032,2.32020947307775));
#86534=CARTESIAN_POINT('Ctrl Pts',(22.9842930518898,3.24675902457591,2.222959887737));
#86535=CARTESIAN_POINT('Ctrl Pts',(22.9782072630088,3.31339686162952,2.12236511533057));
#86536=CARTESIAN_POINT('Ctrl Pts',(22.9721214741278,3.37530075175515,2.01886944481338));
#86537=CARTESIAN_POINT('Ctrl Pts',(22.9662694440496,3.43482687631556,1.91934910510346));
#86538=CARTESIAN_POINT('Ctrl Pts',(22.9604174139713,3.4899757813125,1.817146994531));
#86539=CARTESIAN_POINT('Ctrl Pts',(22.954565383893,3.5405070134031,1.71268767965543));
#86540=CARTESIAN_POINT('Ctrl Pts',(22.9487142435145,3.59103056309559,1.60824424600833));
#86541=CARTESIAN_POINT('Ctrl Pts',(22.942863103136,3.63693765580665,1.50154466239417));
#86542=CARTESIAN_POINT('Ctrl Pts',(22.9370119627575,3.6780344305367,1.39303687237151));
#86543=CARTESIAN_POINT('Ctrl Pts',(22.93116029519,3.71913490809483,1.28451930577405));
#86544=CARTESIAN_POINT('Ctrl Pts',(22.9253086276225,3.75542405967508,1.17419359548204));
#86545=CARTESIAN_POINT('Ctrl Pts',(22.919456960055,3.78675694102397,1.06252570303348));
#86546=CARTESIAN_POINT('Ctrl Pts',(22.9136033483708,3.81810023218825,0.950820710832328));
#86547=CARTESIAN_POINT('Ctrl Pts',(22.9077497366865,3.84448386727344,0.837773047571822));
#86548=CARTESIAN_POINT('Ctrl Pts',(22.9018961250023,3.86581351133244,0.72386110242196));
#86549=CARTESIAN_POINT('Ctrl Pts',(22.8960358589024,3.88716740303973,0.609819661591173));
#86550=CARTESIAN_POINT('Ctrl Pts',(22.8901755928025,3.90345575996642,0.494912384329474));
#86551=CARTESIAN_POINT('Ctrl Pts',(22.8843153267026,3.91463583718272,0.379625160184026));
#86552=CARTESIAN_POINT('Ctrl Pts',(22.8784511135313,3.92582344452861,0.264260286508817));
#86553=CARTESIAN_POINT('Ctrl Pts',(22.87258690036,3.93189589966359,0.148515368169132));
#86554=CARTESIAN_POINT('Ctrl Pts',(22.8667226871887,3.93286258427199,0.0328769407558719));
#86555=CARTESIAN_POINT('Ctrl Pts',(22.8608498386144,3.93383069238102,-0.0829317711256017));
#86556=CARTESIAN_POINT('Ctrl Pts',(22.8549769900401,3.92967803920366,-0.198633267574225));
#86557=CARTESIAN_POINT('Ctrl Pts',(22.8491041414658,3.92046589369477,-0.313745400565606));
#86558=CARTESIAN_POINT('Ctrl Pts',(22.847509396853,3.91796437858899,-0.345003562875146));
#86559=CARTESIAN_POINT('Ctrl Pts',(22.8459146522402,3.91509008387223,-0.376218324086762));
#86560=CARTESIAN_POINT('Ctrl Pts',(22.8443199076274,3.91184488366374,-0.407380173982224));
#86561=CARTESIAN_POINT('Ctrl Pts',(22.8384474614935,3.8998948427197,-0.522129760516045));
#86562=CARTESIAN_POINT('Ctrl Pts',(22.8325750153596,3.88287143834218,-0.636545205998862));
#86563=CARTESIAN_POINT('Ctrl Pts',(22.8267025692257,3.86079989620795,-0.750142094166606));
#86564=CARTESIAN_POINT('Ctrl Pts',(22.8208377302808,3.83875694563342,-0.863591828493058));
#86565=CARTESIAN_POINT('Ctrl Pts',(22.814972891336,3.81167893991004,-0.976224712159847));
#86566=CARTESIAN_POINT('Ctrl Pts',(22.8091080523911,3.77964290994305,-1.08756079063067));
#86567=CARTESIAN_POINT('Ctrl Pts',(22.8032492422711,3.74763981176064,-1.19878241997172));
#86568=CARTESIAN_POINT('Ctrl Pts',(22.7973904321511,3.71068894047635,-1.30870950080175));
#86569=CARTESIAN_POINT('Ctrl Pts',(22.791531622031,3.66891835764608,-1.41687228956162));
#86570=CARTESIAN_POINT('Ctrl Pts',(22.7854458331501,3.62552952214327,-1.52922546088548));
#86571=CARTESIAN_POINT('Ctrl Pts',(22.7793600442691,3.57694006369284,-1.63967442688406));
#86572=CARTESIAN_POINT('Ctrl Pts',(22.7732742553881,3.52335065031684,-1.74770969983917));
#86573=CARTESIAN_POINT('Ctrl Pts',(22.7674222253098,3.47181963846494,-1.8515952731335));
#86574=CARTESIAN_POINT('Ctrl Pts',(22.7615701952316,3.4156658896206,-1.95324875127649));
#86575=CARTESIAN_POINT('Ctrl Pts',(22.7557181651533,3.3551165373737,-2.05223829528676));
#86576=CARTESIAN_POINT('Ctrl Pts',(22.7498670247748,3.29457639060643,-2.15121278965245));
#86577=CARTESIAN_POINT('Ctrl Pts',(22.7440158843962,3.22964218481652,-2.24752380264201));
#86578=CARTESIAN_POINT('Ctrl Pts',(22.7381647440177,3.16058591149103,-2.34076604898577));
#86579=CARTESIAN_POINT('Ctrl Pts',(22.7323130764502,3.09152341618074,-2.43401669647558));
#86580=CARTESIAN_POINT('Ctrl Pts',(22.7264614088827,3.01833836105618,-2.5241976954736));
#86581=CARTESIAN_POINT('Ctrl Pts',(22.7206097413152,2.94134434427477,-2.61093516740704));
#86582=CARTESIAN_POINT('Ctrl Pts',(22.714756129631,2.86432474754457,-2.69770145638605));
#86583=CARTESIAN_POINT('Ctrl Pts',(22.7089025179467,2.78349394712559,-2.78102163444996));
#86584=CARTESIAN_POINT('Ctrl Pts',(22.7030489062625,2.69920336038026,-2.86055767627781));
#86585=CARTESIAN_POINT('Ctrl Pts',(22.6971886401626,2.61481695166547,-2.94018413508418));
#86586=CARTESIAN_POINT('Ctrl Pts',(22.6913283740627,2.52696320710391,-3.01601758750192));
#86587=CARTESIAN_POINT('Ctrl Pts',(22.6854681079628,2.4360277486927,-3.08775935066176));
#86588=CARTESIAN_POINT('Ctrl Pts',(22.6796038947915,2.34503104242302,-3.1595494341296));
#86589=CARTESIAN_POINT('Ctrl Pts',(22.6737396816202,2.25094882401828,-3.22724210000187));
#86590=CARTESIAN_POINT('Ctrl Pts',(22.6678754684489,2.15419544432737,-3.29058216545936));
#86591=CARTESIAN_POINT('Ctrl Pts',(22.6620026198746,2.05729958952528,-3.35401550293377));
#86592=CARTESIAN_POINT('Ctrl Pts',(22.6561297713003,1.95772507724096,-3.41308323788457));
#86593=CARTESIAN_POINT('Ctrl Pts',(22.650256922726,1.85591062344171,-3.46757620792913));
#86594=CARTESIAN_POINT('Ctrl Pts',(22.6486621781132,1.82826338383714,-3.48237351954225));
#86595=CARTESIAN_POINT('Ctrl Pts',(22.6470674335005,1.80045108787041,-3.49683377820558));
#86596=CARTESIAN_POINT('Ctrl Pts',(22.6454726888878,1.77248274897734,-3.51095341817258));
#86597=CARTESIAN_POINT('Ctrl Pts',(22.6396002427538,1.66949286439449,-3.56294721358935));
#86598=CARTESIAN_POINT('Ctrl Pts',(22.6337277966199,1.56404084268664,-3.61049257697362));
#86599=CARTESIAN_POINT('Ctrl Pts',(22.627855350486,1.456547818915,-3.65334879955555));
#86600=CARTESIAN_POINT('Ctrl Pts',(22.6219905115412,1.34919404201552,-3.69614950602361));
#86601=CARTESIAN_POINT('Ctrl Pts',(22.6161256725963,1.23980490129853,-3.73427299970174));
#86602=CARTESIAN_POINT('Ctrl Pts',(22.6102608336515,1.12882579019753,-3.76752456334194));
#86603=CARTESIAN_POINT('Ctrl Pts',(22.6044020235314,1.01796076127777,-3.80074194567657));
#86604=CARTESIAN_POINT('Ctrl Pts',(22.5985432134114,0.905509406527807,-3.82909724153774));
#86605=CARTESIAN_POINT('Ctrl Pts',(22.5926844032914,0.791936122611474,-3.85244418229559));
#86606=CARTESIAN_POINT('Ctrl Pts',(22.5865986144104,0.673962845738983,-3.87669561723851));
#86607=CARTESIAN_POINT('Ctrl Pts',(22.5805128255295,0.554779373282434,-3.8955426184819));
#86608=CARTESIAN_POINT('Ctrl Pts',(22.5744270366485,0.434922794106225,-3.90887850452874));
#86609=CARTESIAN_POINT('Ctrl Pts',(22.5685750065702,0.319669978056154,-3.92170215119032));
#86610=CARTESIAN_POINT('Ctrl Pts',(22.5627229764919,0.20379525911963,-3.92943019358294));
#86611=CARTESIAN_POINT('Ctrl Pts',(22.5568709464137,0.0877847175549696,
-3.93202019874819));
#86612=CARTESIAN_POINT('Ctrl Pts',(22.5510198060352,-0.0282081866174044,
-3.93460981014805));
#86613=CARTESIAN_POINT('Ctrl Pts',(22.5451686656566,-0.144336459218755,
-3.93206292827684));
#86614=CARTESIAN_POINT('Ctrl Pts',(22.5393175252781,-0.260112102085443,
-3.92438921290291));
#86615=CARTESIAN_POINT('Ctrl Pts',(22.5334658577106,-0.375898176362008,
-3.9167148061256));
#86616=CARTESIAN_POINT('Ctrl Pts',(22.5276141901431,-0.491331145267315,
-3.90391267491319));
#86617=CARTESIAN_POINT('Ctrl Pts',(22.5217625225756,-0.605926933078434,
-3.88604446085865));
#86618=CARTESIAN_POINT('Ctrl Pts',(22.5159089108914,-0.720560793385398,
-3.86817031039476));
#86619=CARTESIAN_POINT('Ctrl Pts',(22.5100552992071,-0.834356511329692,
-3.84522679395706));
#86620=CARTESIAN_POINT('Ctrl Pts',(22.5042016875229,-0.946839722032035,
-3.81732675321124));
#86621=CARTESIAN_POINT('Ctrl Pts',(22.498341421423,-1.05945080422265,-3.78939499555665));
#86622=CARTESIAN_POINT('Ctrl Pts',(22.4924811553231,-1.17074599962289,-3.75649556668775));
#86623=CARTESIAN_POINT('Ctrl Pts',(22.4866208892232,-1.28026554377832,-3.71879135438034));
#86624=CARTESIAN_POINT('Ctrl Pts',(22.4807566760519,-1.38985885275179,-3.68106174711369));
#86625=CARTESIAN_POINT('Ctrl Pts',(22.4748924628806,-1.49767374552357,-3.63852106388615));
#86626=CARTESIAN_POINT('Ctrl Pts',(22.4690282497093,-1.60327151628474,-3.59137988036215));
#86627=CARTESIAN_POINT('Ctrl Pts',(22.463155401135,-1.7090247860494,-3.54416927863918));
#86628=CARTESIAN_POINT('Ctrl Pts',(22.4572825525607,-1.81255404958358,-3.49234484037944));
#86629=CARTESIAN_POINT('Ctrl Pts',(22.4514097039864,-1.91344613941091,-3.43616252112345));
#86630=CARTESIAN_POINT('Ctrl Pts',(22.4498149593737,-1.94084291538542,-3.42090647461853));
#86631=CARTESIAN_POINT('Ctrl Pts',(22.4482202147609,-1.96804540707908,-3.40532933324931));
#86632=CARTESIAN_POINT('Ctrl Pts',(22.4466254701481,-1.9950457412971,-3.38943675116269));
#86633=CARTESIAN_POINT('Ctrl Pts',(22.4407530240142,-2.09447107060941,-3.33091431974292));
#86634=CARTESIAN_POINT('Ctrl Pts',(22.4348805778803,-2.19148564199589,-3.26791540387743));
#86635=CARTESIAN_POINT('Ctrl Pts',(22.4290081317464,-2.28565925705394,-3.20066411243723));
#86636=CARTESIAN_POINT('Ctrl Pts',(22.4231432928016,-2.37971087925262,-3.13349993857594));
#86637=CARTESIAN_POINT('Ctrl Pts',(22.4172784538568,-2.47092853041574,-3.06209458168142));
#86638=CARTESIAN_POINT('Ctrl Pts',(22.411413614912,-2.5589075838686,-2.9867174250705));
#86639=CARTESIAN_POINT('Ctrl Pts',(22.405554804792,-2.64679619829897,-2.91141775322549));
#86640=CARTESIAN_POINT('Ctrl Pts',(22.399695994672,-2.73145252486569,-2.83215467001134));
#86641=CARTESIAN_POINT('Ctrl Pts',(22.3938371845519,-2.81250241706229,-2.74923974109549));
#86642=CARTESIAN_POINT('Ctrl Pts',(22.387751395671,-2.89669229907429,-2.66311256814963));
#86643=CARTESIAN_POINT('Ctrl Pts',(22.38166560679,-2.97699028842615,-2.57304513525218));
#86644=CARTESIAN_POINT('Ctrl Pts',(22.375579817909,-3.05301623424322,-2.47943156256577));
#86645=CARTESIAN_POINT('Ctrl Pts',(22.3697277878308,-3.12612197786177,-2.38941374337947));
#86646=CARTESIAN_POINT('Ctrl Pts',(22.3638757577525,-3.1952775230049,-2.29611752853822));
#86647=CARTESIAN_POINT('Ctrl Pts',(22.3580237276743,-3.26018434611698,-2.19992886915322));
#86648=CARTESIAN_POINT('Ctrl Pts',(22.3521725872958,-3.32508130127155,-2.10375483358679));
#86649=CARTESIAN_POINT('Ctrl Pts',(22.3463214469173,-3.38573058759472,-2.00468957038597));
#86650=CARTESIAN_POINT('Ctrl Pts',(22.3404703065388,-3.44187646536597,-1.90314881109173));
#86651=CARTESIAN_POINT('Ctrl Pts',(22.3346186389713,-3.49802740189262,-1.80159890295372));
#86652=CARTESIAN_POINT('Ctrl Pts',(22.3287669714038,-3.54967392322551,-1.69757341709578));
#86653=CARTESIAN_POINT('Ctrl Pts',(22.3229153038363,-3.59660613812219,-1.59151289257164));
#86654=CARTESIAN_POINT('Ctrl Pts',(22.3170616921521,-3.64355394544678,-1.48541713124725));
#86655=CARTESIAN_POINT('Ctrl Pts',(22.3112080804679,-3.6857841647678,-1.37728536466135));
#86656=CARTESIAN_POINT('Ctrl Pts',(22.3053544687837,-3.723135225553,-1.267577647423));
#86657=CARTESIAN_POINT('Ctrl Pts',(22.2994942026838,-3.76052874721483,-1.15774521389146));
#86658=CARTESIAN_POINT('Ctrl Pts',(22.2936339365839,-3.79303190610754,-1.04633364536741));
#86659=CARTESIAN_POINT('Ctrl Pts',(22.287773670484,-3.820533125532,-0.933817774896539));
#86660=CARTESIAN_POINT('Ctrl Pts',(22.2819094573127,-3.84805286788273,-0.821226121488842));
#86661=CARTESIAN_POINT('Ctrl Pts',(22.2760452441415,-3.8705638823988,-0.707529089609426));
#86662=CARTESIAN_POINT('Ctrl Pts',(22.2701810309702,-3.88800609448337,-0.593209582913304));
#86663=CARTESIAN_POINT('Ctrl Pts',(22.2643081823959,-3.90547399126356,-0.478721733938183));
#86664=CARTESIAN_POINT('Ctrl Pts',(22.2584353338216,-3.9178581446798,-0.363609990171793));
#86665=CARTESIAN_POINT('Ctrl Pts',(22.2525624852473,-3.92515046292946,-0.248360309559825));
#86666=CARTESIAN_POINT('Ctrl Pts',(22.2509677406344,-3.92713065790591,-0.217064796833616));
#86667=CARTESIAN_POINT('Ctrl Pts',(22.2493729960215,-3.9287356935202,-0.185759098495439));
#86668=CARTESIAN_POINT('Ctrl Pts',(22.2477782514086,-3.92996606897404,-0.154452894802086));
#86669=CARTESIAN_POINT('Ctrl Pts',(22.2451733416174,-3.93197580585645,-0.103316282791359));
#86670=CARTESIAN_POINT('Ctrl Pts',(22.2425684318262,-3.93298750996713,-0.052140189329702));
#86671=CARTESIAN_POINT('Ctrl Pts',(22.239963522035,-3.93299988507042,-0.000950808129968768));
#86672=CARTESIAN_POINT('',(20.9899638959796,-3.93207325480824,-0.00316412887844202));
#86673=CARTESIAN_POINT('Ctrl Pts',(22.2399624835488,-3.93923257004676,-0.000931875137709155));
#86674=CARTESIAN_POINT('Ctrl Pts',(22.1762853332555,-3.93515111789854,1.25237922762071));
#86675=CARTESIAN_POINT('Ctrl Pts',(22.0463257767155,-2.60887796690492,3.81768824482034));
#86676=CARTESIAN_POINT('Ctrl Pts',(21.8500838139293,1.76400300349318,4.3042169351731));
#86677=CARTESIAN_POINT('Ctrl Pts',(21.6512365951896,4.57456014021278,0.843439117503365));
#86678=CARTESIAN_POINT('Ctrl Pts',(21.4523893764499,3.18302001183926,-3.39210460121854));
#86679=CARTESIAN_POINT('Ctrl Pts',(21.2535421577102,-1.13237711623261,-4.51173049815657));
#86680=CARTESIAN_POINT('Ctrl Pts',(21.0994006690304,-3.67124635021135,-2.1670127640921));
#86681=CARTESIAN_POINT('Ctrl Pts',(21.0115415865969,-3.93275998093503,-0.430560889368484));
#86682=CARTESIAN_POINT('Ctrl Pts',(20.9899649104101,-3.92956263409438,-0.00318220646910175));
#86683=CARTESIAN_POINT('',(19.7399630144492,-3.93119624677767,0.0022721441981891));
#86684=CARTESIAN_POINT('Ctrl Pts',(20.989963522035,-3.93299873257221,-0.00315746502512106));
#86685=CARTESIAN_POINT('Ctrl Pts',(20.9841232485646,-3.93309168334435,0.112623791810322));
#86686=CARTESIAN_POINT('Ctrl Pts',(20.9782829750942,-3.92806771476633,0.228472972992468));
#86687=CARTESIAN_POINT('Ctrl Pts',(20.9724427016238,-3.91793560031064,0.343903521090631));
#86688=CARTESIAN_POINT('Ctrl Pts',(20.9666036388637,-3.90780558627987,0.459310140007778));
#86689=CARTESIAN_POINT('Ctrl Pts',(20.9607645761037,-3.89256956762769,0.574297885362371));
#86690=CARTESIAN_POINT('Ctrl Pts',(20.9549255133436,-3.8722883276806,0.688383691925197));
#86691=CARTESIAN_POINT('Ctrl Pts',(20.9490862357527,-3.8520063415458,0.802473695934891));
#86692=CARTESIAN_POINT('Ctrl Pts',(20.9432469581617,-3.82667883766087,0.915661286759442));
#86693=CARTESIAN_POINT('Ctrl Pts',(20.9374076805708,-3.79641789498912,1.02747270844844));
#86694=CARTESIAN_POINT('Ctrl Pts',(20.9315667627835,-3.76614845231261,1.13931553687937));
#86695=CARTESIAN_POINT('Ctrl Pts',(20.9257258449962,-3.73094292380567,1.24978102730664));
#86696=CARTESIAN_POINT('Ctrl Pts',(20.919884927209,-3.69096330339389,1.35841042877315));
#86697=CARTESIAN_POINT('Ctrl Pts',(20.914037239955,-3.65093734767691,1.46716572879546));
#86698=CARTESIAN_POINT('Ctrl Pts',(20.908189552701,-3.60612639588913,1.57408030124601));
#86699=CARTESIAN_POINT('Ctrl Pts',(20.9023418654471,-3.55674074244052,1.67871507143518));
#86700=CARTESIAN_POINT('Ctrl Pts',(20.8964904987089,-3.50732401453099,1.78341567995696));
#86701=CARTESIAN_POINT('Ctrl Pts',(20.8906391319708,-3.45332704621566,1.88583326332586));
#86702=CARTESIAN_POINT('Ctrl Pts',(20.8847877652327,-3.39500537267214,1.98555471330491));
#86703=CARTESIAN_POINT('Ctrl Pts',(20.8789267994929,-3.33658802407192,2.08543975350351));
#86704=CARTESIAN_POINT('Ctrl Pts',(20.8730658337531,-3.27383202684813,2.18261947962998));
#86705=CARTESIAN_POINT('Ctrl Pts',(20.8672048680132,-3.20703557374272,2.2767107477123));
#86706=CARTESIAN_POINT('Ctrl Pts',(20.8634191520858,-3.16389039807688,2.33748619463052));
#86707=CARTESIAN_POINT('Ctrl Pts',(20.8596334361584,-3.11906032460714,2.39697376210787));
#86708=CARTESIAN_POINT('Ctrl Pts',(20.855847720231,-3.07263405224841,2.45507820261667));
#86709=CARTESIAN_POINT('Ctrl Pts',(20.8499752740971,-3.00061708403131,2.54521047972609));
#86710=CARTESIAN_POINT('Ctrl Pts',(20.8441028279632,-2.92451028708953,2.63232216620249));
#86711=CARTESIAN_POINT('Ctrl Pts',(20.8382303818293,-2.84459645267688,2.7160191496781));
#86712=CARTESIAN_POINT('Ctrl Pts',(20.8323655428845,-2.76478613894951,2.79960771176272));
#86713=CARTESIAN_POINT('Ctrl Pts',(20.8265007039396,-2.68117887787208,2.87979007124439));
#86714=CARTESIAN_POINT('Ctrl Pts',(20.8206358649948,-2.59409865603453,2.95620384323542));
#86715=CARTESIAN_POINT('Ctrl Pts',(20.8147770548748,-2.50710794925554,3.03253906486069));
#86716=CARTESIAN_POINT('Ctrl Pts',(20.8089182447548,-2.41665169160741,3.10511313351274));
#86717=CARTESIAN_POINT('Ctrl Pts',(20.8030594346348,-2.32309130876799,3.17359981269325));
#86718=CARTESIAN_POINT('Ctrl Pts',(20.7969736457538,-2.22590626164745,3.24473976468245));
#86719=CARTESIAN_POINT('Ctrl Pts',(20.7908878568728,-2.1253720220937,3.31146889055746));
#86720=CARTESIAN_POINT('Ctrl Pts',(20.7848020679919,-2.02193258831947,3.37346670478481));
#86721=CARTESIAN_POINT('Ctrl Pts',(20.7789500379136,-1.92246632526592,3.43308314576557));
#86722=CARTESIAN_POINT('Ctrl Pts',(20.7730980078354,-1.82031431897399,3.48832480340048));
#86723=CARTESIAN_POINT('Ctrl Pts',(20.7672459777571,-1.71590091755337,3.53895083903966));
#86724=CARTESIAN_POINT('Ctrl Pts',(20.7613948373786,-1.61150339038099,3.58956917786744));
#86725=CARTESIAN_POINT('Ctrl Pts',(20.7555436970001,-1.50484552351931,3.63557310966683));
#86726=CARTESIAN_POINT('Ctrl Pts',(20.7496925566217,-1.39637508436237,3.67676836689123));
#86727=CARTESIAN_POINT('Ctrl Pts',(20.7438408890542,-1.28789487199603,3.71796733581697));
#86728=CARTESIAN_POINT('Ctrl Pts',(20.7379892214867,-1.17760214913332,3.75435662211436));
#86729=CARTESIAN_POINT('Ctrl Pts',(20.7321375539193,-1.06596274554514,3.78579085860667));
#86730=CARTESIAN_POINT('Ctrl Pts',(20.726283942235,-0.95428625166892,3.81723553858801));
#86731=CARTESIAN_POINT('Ctrl Pts',(20.7204303305508,-0.841262585091059,
3.84372178336171));
#86732=CARTESIAN_POINT('Ctrl Pts',(20.7145767188666,-0.727370049150624,
3.86515482375527));
#86733=CARTESIAN_POINT('Ctrl Pts',(20.7087164527667,-0.613348039593898,
3.88661222933856));
#86734=CARTESIAN_POINT('Ctrl Pts',(20.7028561866668,-0.498455595654684,
3.90300488820321));
#86735=CARTESIAN_POINT('Ctrl Pts',(20.696995920567,-0.38317856787765,3.91428961436417));
#86736=CARTESIAN_POINT('Ctrl Pts',(20.6911317073957,-0.267823897438149,
3.92558194113908));
#86737=CARTESIAN_POINT('Ctrl Pts',(20.6852674942244,-0.152084539141536,
3.93175946280133));
#86738=CARTESIAN_POINT('Ctrl Pts',(20.6794032810531,-0.0364470368946023,
3.9328311193721));
#86739=CARTESIAN_POINT('Ctrl Pts',(20.6735304324788,0.0793607484578857,
3.93390435402096));
#86740=CARTESIAN_POINT('Ctrl Pts',(20.6676575839045,0.195065966862631,3.92985673216703));
#86741=CARTESIAN_POINT('Ctrl Pts',(20.6617847353302,0.310186414876173,3.9207490850635));
#86742=CARTESIAN_POINT('Ctrl Pts',(20.6601899907173,0.34144683509439,3.91827594601159));
#86743=CARTESIAN_POINT('Ctrl Pts',(20.6585952461043,0.372664192628336,3.91542998810426));
#86744=CARTESIAN_POINT('Ctrl Pts',(20.6570005014914,0.403828975562439,3.912213076827));
#86745=CARTESIAN_POINT('Ctrl Pts',(20.6511280553575,0.518589362630107,3.90036720630957));
#86746=CARTESIAN_POINT('Ctrl Pts',(20.6452556092236,0.633020214199333,3.88344767112789));
#86747=CARTESIAN_POINT('Ctrl Pts',(20.6393831630896,0.746637091306685,3.86147925721285));
#86748=CARTESIAN_POINT('Ctrl Pts',(20.6335183241448,0.860106788678741,3.83953930126486));
#86749=CARTESIAN_POINT('Ctrl Pts',(20.6276534852,0.972764206367716,3.81256355073526));
#86750=CARTESIAN_POINT('Ctrl Pts',(20.6217886462551,1.08412932010921,3.78062860081224));
#86751=CARTESIAN_POINT('Ctrl Pts',(20.6159298361351,1.19537995487396,3.74872647876743));
#86752=CARTESIAN_POINT('Ctrl Pts',(20.6100710260151,1.30534053306963,3.71187541051525));
#86753=CARTESIAN_POINT('Ctrl Pts',(20.6042122158951,1.41354119508099,3.67020303114269));
#86754=CARTESIAN_POINT('Ctrl Pts',(20.5981264270141,1.52593370692096,3.62691620364123));
#86755=CARTESIAN_POINT('Ctrl Pts',(20.5920406381331,1.63642673515667,3.57842702676651));
#86756=CARTESIAN_POINT('Ctrl Pts',(20.5859548492521,1.7445106101207,3.52493570596349));
#86757=CARTESIAN_POINT('Ctrl Pts',(20.5801028191739,1.84844291859143,3.47349901889008));
#86758=CARTESIAN_POINT('Ctrl Pts',(20.5742507890956,1.95014732918308,3.41743757051405));
#86759=CARTESIAN_POINT('Ctrl Pts',(20.5683987590174,2.04919179690856,3.35697810232397));
#86760=CARTESIAN_POINT('Ctrl Pts',(20.5625476186388,2.14822120663928,3.2965278259482));
#86761=CARTESIAN_POINT('Ctrl Pts',(20.5566964782603,2.24459112485832,3.23168107454867));
#86762=CARTESIAN_POINT('Ctrl Pts',(20.5508453378818,2.33789601955901,3.16270947159712));
#86763=CARTESIAN_POINT('Ctrl Pts',(20.5449936703143,2.43120932105043,3.09373165428957));
#86764=CARTESIAN_POINT('Ctrl Pts',(20.5391420027468,2.52145671762473,3.020628492351));
#86765=CARTESIAN_POINT('Ctrl Pts',(20.5332903351793,2.60826404619016,2.94371324441626));
#86766=CARTESIAN_POINT('Ctrl Pts',(20.5274367234951,2.69510021501009,2.86677244270213));
#86767=CARTESIAN_POINT('Ctrl Pts',(20.5215831118108,2.7784937340069,2.78601731061528));
#86768=CARTESIAN_POINT('Ctrl Pts',(20.5157295001266,2.85810625899502,2.70179895852624));
#86769=CARTESIAN_POINT('Ctrl Pts',(20.5098692340267,2.93780928790779,2.61748486658481));
#86770=CARTESIAN_POINT('Ctrl Pts',(20.5040089679268,3.01372245951614,2.52969999707192));
#86771=CARTESIAN_POINT('Ctrl Pts',(20.4981487018269,3.08554674102027,2.43882970069236));
#86772=CARTESIAN_POINT('Ctrl Pts',(20.4922844886556,3.15741939841086,2.34789820034322));
#86773=CARTESIAN_POINT('Ctrl Pts',(20.4864202754844,3.22519744080989,2.25387746964359));
#86774=CARTESIAN_POINT('Ctrl Pts',(20.4805560623131,3.28862530937061,2.15718162762597));
#86775=CARTESIAN_POINT('Ctrl Pts',(20.4746832137388,3.35214657924372,2.06034339522458));
#86776=CARTESIAN_POINT('Ctrl Pts',(20.4688103651645,3.4113046799798,1.96082254350937));
#86777=CARTESIAN_POINT('Ctrl Pts',(20.4629375165902,3.46589005103204,1.85905759839686));
#86778=CARTESIAN_POINT('Ctrl Pts',(20.4613427719774,3.48071245370826,1.83142380264347));
#86779=CARTESIAN_POINT('Ctrl Pts',(20.4597480273646,3.49519795340568,1.80362464463149));
#86780=CARTESIAN_POINT('Ctrl Pts',(20.4581532827518,3.50934297619718,1.77566913455619));
#86781=CARTESIAN_POINT('Ctrl Pts',(20.4522808366178,3.56143024066478,1.67272649048393));
#86782=CARTESIAN_POINT('Ctrl Pts',(20.4464083904839,3.60907130997126,1.56731767217624));
#86783=CARTESIAN_POINT('Ctrl Pts',(20.4405359443499,3.65202509315485,1.45986359601413));
#86784=CARTESIAN_POINT('Ctrl Pts',(20.4346711054051,3.69492323384417,1.35254871627138));
#86785=CARTESIAN_POINT('Ctrl Pts',(20.4288062664602,3.7331460112999,1.243194227746));
#86786=CARTESIAN_POINT('Ctrl Pts',(20.4229414275154,3.76649830404232,1.13224534693074));
#86787=CARTESIAN_POINT('Ctrl Pts',(20.4170826173953,3.79981631193363,1.02141051722102));
#86788=CARTESIAN_POINT('Ctrl Pts',(20.4112238072753,3.82827367536364,0.908984948709361));
#86789=CARTESIAN_POINT('Ctrl Pts',(20.4053649971552,3.85172370420032,0.795432905090898));
#86790=CARTESIAN_POINT('Ctrl Pts',(20.3992792082743,3.87608222100296,0.677481691396547));
#86791=CARTESIAN_POINT('Ctrl Pts',(20.3931934193933,3.89503740490437,0.558315376668335));
#86792=CARTESIAN_POINT('Ctrl Pts',(20.3871076305123,3.90848208690171,0.438470952707787));
#86793=CARTESIAN_POINT('Ctrl Pts',(20.3812556004341,3.92141035059607,0.323229824983995));
#86794=CARTESIAN_POINT('Ctrl Pts',(20.3754035703558,3.92924357666178,0.207362169025676));
#86795=CARTESIAN_POINT('Ctrl Pts',(20.3695515402775,3.93193889091192,0.0913540263717977));
#86796=CARTESIAN_POINT('Ctrl Pts',(20.363700399899,3.93463379538624,-0.0246364792546189));
#86797=CARTESIAN_POINT('Ctrl Pts',(20.3578492595204,3.93219233158833,-0.140767015976084));
#86798=CARTESIAN_POINT('Ctrl Pts',(20.3519981191419,3.92462371629558,-0.256549577061237));
#86799=CARTESIAN_POINT('Ctrl Pts',(20.3461464515744,3.91705441906898,-0.3723425701796));
#86800=CARTESIAN_POINT('Ctrl Pts',(20.3402947840069,3.90435707898377,-0.487787112834));
#86801=CARTESIAN_POINT('Ctrl Pts',(20.3344431164393,3.88659289818115,-0.602399073544966));
#86802=CARTESIAN_POINT('Ctrl Pts',(20.3285895047551,3.86882281553248,-0.717049112124836));
#86803=CARTESIAN_POINT('Ctrl Pts',(20.3227358930708,3.84598260816349,-0.830865610473498));
#86804=CARTESIAN_POINT('Ctrl Pts',(20.3168822813866,3.8181846870822,-0.94337410147354));
#86805=CARTESIAN_POINT('Ctrl Pts',(20.3110220152867,3.79035516518226,-1.05601049270072));
#86806=CARTESIAN_POINT('Ctrl Pts',(20.3051617491868,3.75755677960058,-1.167335507151));
#86807=CARTESIAN_POINT('Ctrl Pts',(20.2993014830869,3.71995200068839,-1.27688923269579));
#86808=CARTESIAN_POINT('Ctrl Pts',(20.2934372699155,3.68232189378844,-1.38651674608085));
#86809=CARTESIAN_POINT('Ctrl Pts',(20.2875730567442,3.63987909852825,-1.49437021131679));
#86810=CARTESIAN_POINT('Ctrl Pts',(20.2817088435729,3.59283379224433,-1.60001073162253));
#86811=CARTESIAN_POINT('Ctrl Pts',(20.2758359949986,3.54571920894637,-1.70580681388301));
#86812=CARTESIAN_POINT('Ctrl Pts',(20.2699631464243,3.49398877214061,-1.8093830791024));
#86813=CARTESIAN_POINT('Ctrl Pts',(20.26409029785,3.4378980622037,-1.91032612762743));
#86814=CARTESIAN_POINT('Ctrl Pts',(20.2624955532373,3.42266689178285,-1.93773674119633));
#86815=CARTESIAN_POINT('Ctrl Pts',(20.2609008086247,3.40711445026582,-1.9649533620427));
#86816=CARTESIAN_POINT('Ctrl Pts',(20.259306064012,3.39124638465022,-1.99196811184236));
#86817=CARTESIAN_POINT('Ctrl Pts',(20.2534336178781,3.33281423204201,-2.09144652472551));
#86818=CARTESIAN_POINT('Ctrl Pts',(20.2475611717442,3.26990340843406,-2.18851824426593));
#86819=CARTESIAN_POINT('Ctrl Pts',(20.2416887256103,3.20273763208658,-2.28275286880039));
#86820=CARTESIAN_POINT('Ctrl Pts',(20.2358238866655,3.13565886254135,-2.37686542144368));
#86821=CARTESIAN_POINT('Ctrl Pts',(20.2299590477206,3.06433633913443,-2.46814785421082));
#86822=CARTESIAN_POINT('Ctrl Pts',(20.2240942087758,2.98903907776629,-2.55619529605742));
#86823=CARTESIAN_POINT('Ctrl Pts',(20.2182353986558,2.91381921903475,-2.64415222858108));
#86824=CARTESIAN_POINT('Ctrl Pts',(20.2123765885357,2.83463301641362,-2.72888047241358));
#86825=CARTESIAN_POINT('Ctrl Pts',(20.2065177784157,2.75179169580537,-2.8100055983746));
#86826=CARTESIAN_POINT('Ctrl Pts',(20.2004319895347,2.6657409828596,-2.89427362881527));
#86827=CARTESIAN_POINT('Ctrl Pts',(20.1943462006538,2.57574647866703,-2.97465334502407));
#86828=CARTESIAN_POINT('Ctrl Pts',(20.1882604117728,2.48220195814077,-3.05076423851502));
#86829=CARTESIAN_POINT('Ctrl Pts',(20.1824083816945,2.39225053877939,-3.12395166691658));
#86830=CARTESIAN_POINT('Ctrl Pts',(20.1765563516163,2.29901713926724,-3.19319187447863));
#86831=CARTESIAN_POINT('Ctrl Pts',(20.170704321538,2.20288743956765,-3.25818598741617));
#86832=CARTESIAN_POINT('Ctrl Pts',(20.1648531811595,2.10677235472292,-3.32317021912522));
#86833=CARTESIAN_POINT('Ctrl Pts',(20.159002040781,2.00776218755567,-3.38390940830432));
#86834=CARTESIAN_POINT('Ctrl Pts',(20.1531509004025,1.90627243728438,-3.44014743795231));
#86835=CARTESIAN_POINT('Ctrl Pts',(20.147299232835,1.80477354276511,-3.49639053465868));
#86836=CARTESIAN_POINT('Ctrl Pts',(20.1414475652675,1.70079498260152,-3.54813146526662));
#86837=CARTESIAN_POINT('Ctrl Pts',(20.1355958977,1.59477710513419,-3.5951599387148));
#86838=CARTESIAN_POINT('Ctrl Pts',(20.1297422860157,1.48872400503487,-3.64220403657137));
#86839=CARTESIAN_POINT('Ctrl Pts',(20.1238886743314,1.38063061805801,-3.68453239657957));
#86840=CARTESIAN_POINT('Ctrl Pts',(20.1180350626471,1.27095685195525,-3.72198303065288));
#86841=CARTESIAN_POINT('Ctrl Pts',(20.1121747965473,1.16115840815582,-3.75947623879801));
#86842=CARTESIAN_POINT('Ctrl Pts',(20.1063145304474,1.04977639072099,-3.79208051967024));
#86843=CARTESIAN_POINT('Ctrl Pts',(20.1004542643475,0.937285531215521,-3.81968386558024));
#86844=CARTESIAN_POINT('Ctrl Pts',(20.0945900511762,0.824718905618889,-3.84730580320189));
#86845=CARTESIAN_POINT('Ctrl Pts',(20.0887258380049,0.711042355264937,-3.86992001847493));
#86846=CARTESIAN_POINT('Ctrl Pts',(20.0828616248336,0.596738729076179,-3.88746599846488));
#86847=CARTESIAN_POINT('Ctrl Pts',(20.0769887762593,0.482266783993507,-3.90503781595486));
#86848=CARTESIAN_POINT('Ctrl Pts',(20.071115927685,0.367166329539215,-3.91752645852448));
#86849=CARTESIAN_POINT('Ctrl Pts',(20.0652430791107,0.251923316113332,-3.92492339323947));
#86850=CARTESIAN_POINT('Ctrl Pts',(20.063648334498,0.220629613833267,-3.9269319963285));
#86851=CARTESIAN_POINT('Ctrl Pts',(20.0620535898852,0.189325385389403,-3.92856544945613));
#86852=CARTESIAN_POINT('Ctrl Pts',(20.0604588452725,0.158020311487698,-3.92982424303649));
#86853=CARTESIAN_POINT('Ctrl Pts',(20.0545863991385,0.0427433205923004,
-3.934459591816));
#86854=CARTESIAN_POINT('Ctrl Pts',(20.0487139530046,-0.072930801677193,
-3.93402611889401));
#86855=CARTESIAN_POINT('Ctrl Pts',(20.0428415068707,-0.188519030851017,
-3.92847929547898));
#86856=CARTESIAN_POINT('Ctrl Pts',(20.0369766679259,-0.303957526592885,
-3.9229396574401));
#86857=CARTESIAN_POINT('Ctrl Pts',(20.031111828981,-0.41930994143253,-3.91229986102818));
#86858=CARTESIAN_POINT('Ctrl Pts',(20.0252469900362,-0.534090234586468,
-3.89656728689745));
#86859=CARTESIAN_POINT('Ctrl Pts',(20.0193881799161,-0.648752538092979,
-3.88085088523696));
#86860=CARTESIAN_POINT('Ctrl Pts',(20.0135293697961,-0.762843482644825,
-3.8600521747055));
#86861=CARTESIAN_POINT('Ctrl Pts',(20.0076705596761,-0.875879812045625,
-3.83423050361489));
#86862=CARTESIAN_POINT('Ctrl Pts',(20.0015847707951,-0.993295332009472,
-3.807408463714));
#86863=CARTESIAN_POINT('Ctrl Pts',(19.9954989819141,-1.10957241568892,-3.77516642014239));
#86864=CARTESIAN_POINT('Ctrl Pts',(19.9894131930332,-1.22417805782623,-3.73762987503268));
#86865=CARTESIAN_POINT('Ctrl Pts',(19.9835611629549,-1.33438162847987,-3.70153513114445));
#86866=CARTESIAN_POINT('Ctrl Pts',(19.9777091328766,-1.44303936204964,-3.66054525357306));
#86867=CARTESIAN_POINT('Ctrl Pts',(19.9718571027983,-1.54969130213815,-3.61482307562588));
#86868=CARTESIAN_POINT('Ctrl Pts',(19.9660059624198,-1.65632702764745,-3.5691078489435));
#86869=CARTESIAN_POINT('Ctrl Pts',(19.9601548220413,-1.76095718619479,-3.51866191524246));
#86870=CARTESIAN_POINT('Ctrl Pts',(19.9543036816628,-1.86314166519393,-3.46369631108421));
#86871=CARTESIAN_POINT('Ctrl Pts',(19.9484520140953,-1.96533535103594,-3.40872575451357));
#86872=CARTESIAN_POINT('Ctrl Pts',(19.9426003465278,-2.06508255522672,-3.34923491379087));
#86873=CARTESIAN_POINT('Ctrl Pts',(19.9367486789603,-2.16196827819438,-3.28548050733545));
#86874=CARTESIAN_POINT('Ctrl Pts',(19.9308950672761,-2.25888618979084,-3.221704919566));
#86875=CARTESIAN_POINT('Ctrl Pts',(19.9250414555919,-2.3529403846782,-3.15366317654784));
#86876=CARTESIAN_POINT('Ctrl Pts',(19.9191878439077,-2.44374592020367,-3.0816545681643));
#86877=CARTESIAN_POINT('Ctrl Pts',(19.9133275778078,-2.53465468392592,-3.00956410002681));
#86878=CARTESIAN_POINT('Ctrl Pts',(19.9074673117079,-2.62230709292485,-2.93349802259585));
#86879=CARTESIAN_POINT('Ctrl Pts',(19.901607045608,-2.7063522331158,-2.85379512059102));
#86880=CARTESIAN_POINT('Ctrl Pts',(19.8957428324367,-2.79045398032162,-2.77403853620375));
#86881=CARTESIAN_POINT('Ctrl Pts',(19.8898786192654,-2.87094333452931,-2.6906405464676));
#86882=CARTESIAN_POINT('Ctrl Pts',(19.8840144060941,-2.94750831036257,-2.60397460823711));
#86883=CARTESIAN_POINT('Ctrl Pts',(19.8781415575198,-3.02418603268067,-2.51718104925334));
#86884=CARTESIAN_POINT('Ctrl Pts',(19.8722687089455,-3.09692758439631,-2.42711025785644));
#86885=CARTESIAN_POINT('Ctrl Pts',(19.8663958603712,-3.16546302917209,-2.33416640600979));
#86886=CARTESIAN_POINT('Ctrl Pts',(19.8648011157584,-3.18407350924169,-2.30892793695128));
#86887=CARTESIAN_POINT('Ctrl Pts',(19.8632063711456,-3.20237410142416,-2.28347776576456));
#86888=CARTESIAN_POINT('Ctrl Pts',(19.8616116265327,-3.22035998380339,-2.25782430111775));
#86889=CARTESIAN_POINT('Ctrl Pts',(19.8556714388557,-3.28735473394137,-2.16226894175588));
#86890=CARTESIAN_POINT('Ctrl Pts',(19.8497312511786,-3.35020127333526,-2.06357478088844));
#86891=CARTESIAN_POINT('Ctrl Pts',(19.8437910635016,-3.408595750654,-1.96213251556145));
#86892=CARTESIAN_POINT('Ctrl Pts',(19.8378589838667,-3.4669105225975,-1.86082871356512));
#86893=CARTESIAN_POINT('Ctrl Pts',(19.8319269042319,-3.52078512172335,-1.75678461211711));
#86894=CARTESIAN_POINT('Ctrl Pts',(19.8259948245971,-3.56995767443358,-1.65042152274891));
#86895=CARTESIAN_POINT('Ctrl Pts',(19.8200695201429,-3.61907406590691,-1.54417991340013));
#86896=CARTESIAN_POINT('Ctrl Pts',(19.8141442156888,-3.66349892815091,-1.43562494691014));
#86897=CARTESIAN_POINT('Ctrl Pts',(19.8082189112347,-3.7030155051032,-1.32520382166869));
#86898=CARTESIAN_POINT('Ctrl Pts',(19.8022998744631,-3.74249028211675,-1.21489949794766));
#86899=CARTESIAN_POINT('Ctrl Pts',(19.7963808376916,-3.77706697789933,-1.10273332201382));
#86900=CARTESIAN_POINT('Ctrl Pts',(19.7904618009201,-3.80657661320366,-0.989173133385114));
#86901=CARTESIAN_POINT('Ctrl Pts',(19.7845464878454,-3.83606768384311,-0.875684386061103));
#86902=CARTESIAN_POINT('Ctrl Pts',(19.7786311747707,-3.86049793596701,-0.7608037578258));
#86903=CARTESIAN_POINT('Ctrl Pts',(19.772715861696,-3.87974806231536,-0.645014707553379));
#86904=CARTESIAN_POINT('Ctrl Pts',(19.7668024441909,-3.89899201993626,-0.529262762029275));
#86905=CARTESIAN_POINT('Ctrl Pts',(19.7608890266857,-3.91305908525392,-0.412603368035265));
#86906=CARTESIAN_POINT('Ctrl Pts',(19.7549756091806,-3.92188103807962,-0.295530240671769));
#86907=CARTESIAN_POINT('Ctrl Pts',(19.7499715801321,-3.92934631651909,-0.196461076415751));
#86908=CARTESIAN_POINT('Ctrl Pts',(19.7449675510835,-3.93305652182695,-0.0970959558208752));
#86909=CARTESIAN_POINT('Ctrl Pts',(19.739963522035,-3.93299934888168,0.00226311650535728));
#86910=CARTESIAN_POINT('',(18.4899641225863,-3.93462928533228,0.00227594938782067));
#86911=CARTESIAN_POINT('Ctrl Pts',(19.7399620606286,-3.9278079804333,0.00228910842207941));
#86912=CARTESIAN_POINT('Ctrl Pts',(19.7142295096835,-3.93046244247961,0.512557092329908));
#86913=CARTESIAN_POINT('Ctrl Pts',(19.6222145524918,-3.60059902134384,2.33387743482087));
#86914=CARTESIAN_POINT('Ctrl Pts',(19.4639171890534,-0.847591389378432,
4.57379261204712));
#86915=CARTESIAN_POINT('Ctrl Pts',(19.2650699703139,3.38921377376182,3.18609792961681));
#86916=CARTESIAN_POINT('Ctrl Pts',(19.0662227515741,4.51275657002401,-1.1282810647494));
#86917=CARTESIAN_POINT('Ctrl Pts',(18.8673755328346,1.49097359512779,-4.40624417843557));
#86918=CARTESIAN_POINT('Ctrl Pts',(18.6752897180372,-2.75106770730041,-3.66288770573472));
#86919=CARTESIAN_POINT('Ctrl Pts',(18.5494863094863,-3.92972806296831,-1.17034855638654));
#86920=CARTESIAN_POINT('Ctrl Pts',(18.489965307182,-3.93784438422833,0.00225448157776348));
#86921=CARTESIAN_POINT('',(17.2399634336168,-3.93317891120594,-0.00339957664883343));
#86922=CARTESIAN_POINT('Ctrl Pts',(18.489963522035,-3.93299933516336,0.00228683286660641));
#86923=CARTESIAN_POINT('Ctrl Pts',(18.4832027131417,-3.9329219864051,0.135314750767533));
#86924=CARTESIAN_POINT('Ctrl Pts',(18.4764419042485,-3.9260959776598,0.268144188695659));
#86925=CARTESIAN_POINT('Ctrl Pts',(18.4696810953553,-3.91257804618956,0.400277444375149));
#86926=CARTESIAN_POINT('Ctrl Pts',(18.4638086492214,-3.90083635586009,0.515048537410222));
#86927=CARTESIAN_POINT('Ctrl Pts',(18.4579362030875,-3.88402070381646,0.629494700770946));
#86928=CARTESIAN_POINT('Ctrl Pts',(18.4520637569536,-3.86215543622327,0.743131473193722));
#86929=CARTESIAN_POINT('Ctrl Pts',(18.4461989180087,-3.84031849298093,0.856621040109026));
#86930=CARTESIAN_POINT('Ctrl Pts',(18.4403340790639,-3.81344501987382,0.969302898987156));
#86931=CARTESIAN_POINT('Ctrl Pts',(18.4344692401191,-3.78161117631,1.08069695623115));
#86932=CARTESIAN_POINT('Ctrl Pts',(18.428610429999,-3.74981005669104,1.1919765047455));
#86933=CARTESIAN_POINT('Ctrl Pts',(18.422751619879,-3.7130588218373,1.30197048969573));
#86934=CARTESIAN_POINT('Ctrl Pts',(18.416892809759,-3.6714846802617,1.4102089357977));
#86935=CARTESIAN_POINT('Ctrl Pts',(18.410807020878,-3.62829989643136,1.52264069553817));
#86936=CARTESIAN_POINT('Ctrl Pts',(18.404721231997,-3.57991104108909,1.63317769496063));
#86937=CARTESIAN_POINT('Ctrl Pts',(18.3986354431161,-3.52651785693774,1.74131008286843));
#86938=CARTESIAN_POINT('Ctrl Pts',(18.3927834130378,-3.47517553702818,1.84528904087194));
#86939=CARTESIAN_POINT('Ctrl Pts',(18.3869313829595,-3.41920643531677,1.94704430010447));
#86940=CARTESIAN_POINT('Ctrl Pts',(18.3810793528812,-3.35883690100393,2.04614360992926));
#86941=CARTESIAN_POINT('Ctrl Pts',(18.3752282125027,-3.2984765448325,2.14522785342151));
#86942=CARTESIAN_POINT('Ctrl Pts',(18.3693770721242,-3.23371730125901,2.24165659745801));
#86943=CARTESIAN_POINT('Ctrl Pts',(18.3635259317456,-3.16483042551607,2.33502406362927));
#86944=CARTESIAN_POINT('Ctrl Pts',(18.3576742641781,-3.09593734305105,2.42839994222899));
#86945=CARTESIAN_POINT('Ctrl Pts',(18.3518225966106,-3.0229161345377,2.51871366201266));
#86946=CARTESIAN_POINT('Ctrl Pts',(18.3459709290431,-2.94607971883014,2.6055907756779));
#86947=CARTESIAN_POINT('Ctrl Pts',(18.3401173173588,-2.86921777553405,2.69249675278229));
#86948=CARTESIAN_POINT('Ctrl Pts',(18.3342637056745,-2.78853837832446,2.77596354399245));
#86949=CARTESIAN_POINT('Ctrl Pts',(18.3284100939903,-2.70439233029071,2.85565248653697));
#86950=CARTESIAN_POINT('Ctrl Pts',(18.3225498278904,-2.62015062459991,2.93543201987826));
#86951=CARTESIAN_POINT('Ctrl Pts',(18.3166895617905,-2.53243470247297,3.0114248481223));
#86952=CARTESIAN_POINT('Ctrl Pts',(18.3108292956905,-2.44162964300481,3.08333158878512));
#86953=CARTESIAN_POINT('Ctrl Pts',(18.3049650825192,-2.35076342350592,3.15528676087341));
#86954=CARTESIAN_POINT('Ctrl Pts',(18.2991008693479,-2.2568042579867,3.22315012394814));
#86955=CARTESIAN_POINT('Ctrl Pts',(18.2932366561766,-2.16016603332199,3.28666574334567));
#86956=CARTESIAN_POINT('Ctrl Pts',(18.2873638076022,-2.06338550311883,3.35027489327369));
#86957=CARTESIAN_POINT('Ctrl Pts',(18.2814909590279,-1.96391839398079,3.40952331104666));
#86958=CARTESIAN_POINT('Ctrl Pts',(18.2756181104536,-1.8622030414123,3.46420103812622));
#86959=CARTESIAN_POINT('Ctrl Pts',(18.2740233658409,-1.83458271228516,3.47904851964917));
#86960=CARTESIAN_POINT('Ctrl Pts',(18.2724286212283,-1.80679671513932,3.49355924844205));
#86961=CARTESIAN_POINT('Ctrl Pts',(18.2708338766156,-1.77885405692203,3.50772964240005));
#86962=CARTESIAN_POINT('Ctrl Pts',(18.2649614304817,-1.6759587381894,3.55991033299644));
#86963=CARTESIAN_POINT('Ctrl Pts',(18.2590889843477,-1.57059321014312,3.60764706896696));
#86964=CARTESIAN_POINT('Ctrl Pts',(18.2532165382138,-1.46317817013717,3.65069837735659));
#86965=CARTESIAN_POINT('Ctrl Pts',(18.247351699269,-1.35590227598285,3.69369391691749));
#86966=CARTESIAN_POINT('Ctrl Pts',(18.2414868603241,-1.24658252976148,3.73201594665387));
#86967=CARTESIAN_POINT('Ctrl Pts',(18.2356220213793,-1.13566397065819,3.76546894101503));
#86968=CARTESIAN_POINT('Ctrl Pts',(18.2297632112593,-1.02485943149117,3.79888754700769));
#86969=CARTESIAN_POINT('Ctrl Pts',(18.2239044011392,-0.912459741861291,
3.82744695455661));
#86970=CARTESIAN_POINT('Ctrl Pts',(18.2180455910192,-0.798929032112439,
3.85100005214852));
#86971=CARTESIAN_POINT('Ctrl Pts',(18.2119598021382,-0.680999978791925,
3.87546563073887));
#86972=CARTESIAN_POINT('Ctrl Pts',(18.2058740132573,-0.561850919989012,
3.89452898167878));
#86973=CARTESIAN_POINT('Ctrl Pts',(18.1997882243763,-0.442018749999848,
3.90808244854795));
#86974=CARTESIAN_POINT('Ctrl Pts',(18.193936194298,-0.326789405565467,3.9211153186219));
#86975=CARTESIAN_POINT('Ctrl Pts',(18.1880841642198,-0.21092890806477,3.92905372190601));
#86976=CARTESIAN_POINT('Ctrl Pts',(18.1822321341415,-0.0949232599168263,
3.93185434302019));
#86977=CARTESIAN_POINT('Ctrl Pts',(18.176380993763,0.0210647515827713,3.93465453834848));
#86978=CARTESIAN_POINT('Ctrl Pts',(18.1705298533845,0.137197456728115,3.93231849463597));
#86979=CARTESIAN_POINT('Ctrl Pts',(18.164678713006,0.252986840622257,3.9248549856615));
#86980=CARTESIAN_POINT('Ctrl Pts',(18.1588270454385,0.368786657164403,3.9173908042233));
#86981=CARTESIAN_POINT('Ctrl Pts',(18.152975377871,0.484242678437045,3.90479826572867));
#86982=CARTESIAN_POINT('Ctrl Pts',(18.1471237103035,0.598870717603099,3.88713813281668));
#86983=CARTESIAN_POINT('Ctrl Pts',(18.1412700986193,0.713536839979979,3.86947213262675));
#86984=CARTESIAN_POINT('Ctrl Pts',(18.135416486935,0.827374024943987,3.84673525314798));
#86985=CARTESIAN_POINT('Ctrl Pts',(18.1295628752508,0.939907703530585,3.81903947463807));
#86986=CARTESIAN_POINT('Ctrl Pts',(18.1237026091509,1.05256931097761,3.79131221142574));
#86987=CARTESIAN_POINT('Ctrl Pts',(18.117842343051,1.16392405274187,3.75861489615878));
#86988=CARTESIAN_POINT('Ctrl Pts',(18.1119820769512,1.27351186939958,3.72110958162997));
#86989=CARTESIAN_POINT('Ctrl Pts',(18.1061178637799,1.38317349685899,3.68357900610576));
#86990=CARTESIAN_POINT('Ctrl Pts',(18.1002536506086,1.49106544568376,3.64123413378783));
#86991=CARTESIAN_POINT('Ctrl Pts',(18.0943894374372,1.59674862848231,3.59428474351155));
#86992=CARTESIAN_POINT('Ctrl Pts',(18.088516588863,1.70258743605868,3.54726621746326));
#86993=CARTESIAN_POINT('Ctrl Pts',(18.0826437402887,1.80621061761258,3.49562982473978));
#86994=CARTESIAN_POINT('Ctrl Pts',(18.0767708917144,1.90720454165451,3.4396307703433));
#86995=CARTESIAN_POINT('Ctrl Pts',(18.0751761471016,1.93462897023533,3.42442448855497));
#86996=CARTESIAN_POINT('Ctrl Pts',(18.0735814024888,1.96185969781174,3.40889675970325));
#86997=CARTESIAN_POINT('Ctrl Pts',(18.071986657876,1.98888884093666,3.39305322363173));
#86998=CARTESIAN_POINT('Ctrl Pts',(18.0661142117421,2.08842025541688,3.33471139798524));
#86999=CARTESIAN_POINT('Ctrl Pts',(18.0602417656082,2.18554904312068,3.27188871847559));
#87000=CARTESIAN_POINT('Ctrl Pts',(18.0543693194743,2.27984459947886,3.2048085125678));
#87001=CARTESIAN_POINT('Ctrl Pts',(18.0485044805294,2.37401800501449,3.13781520261403));
#87002=CARTESIAN_POINT('Ctrl Pts',(18.0426396415846,2.4653651441655,3.06657557146715));
#87003=CARTESIAN_POINT('Ctrl Pts',(18.0367748026397,2.55348090185147,2.99135826738955));
#87004=CARTESIAN_POINT('Ctrl Pts',(18.0309159925197,2.64150607998831,2.91621828375575));
#87005=CARTESIAN_POINT('Ctrl Pts',(18.0250571823997,2.72630617126706,2.83710902698035));
#87006=CARTESIAN_POINT('Ctrl Pts',(18.0191983722797,2.80750646414212,2.75434138294443));
#87007=CARTESIAN_POINT('Ctrl Pts',(18.0131125833987,2.89185257357177,2.66836720090754));
#87008=CARTESIAN_POINT('Ctrl Pts',(18.0070267945177,2.97231395040191,2.57844569957846));
#87009=CARTESIAN_POINT('Ctrl Pts',(18.0009410056368,3.04850972884881,2.48497030829629));
#87010=CARTESIAN_POINT('Ctrl Pts',(17.9950889755585,3.12177878172414,2.39508536288336));
#87011=CARTESIAN_POINT('Ctrl Pts',(17.9892369454802,3.19110359464856,2.30191485552831));
#87012=CARTESIAN_POINT('Ctrl Pts',(17.983384915402,3.25618494385395,2.20584419472882));
#87013=CARTESIAN_POINT('Ctrl Pts',(17.9775337750235,3.32125639856811,2.10978813980833));
#87014=CARTESIAN_POINT('Ctrl Pts',(17.9716826346449,3.38208544055183,2.01083315026287));
#87015=CARTESIAN_POINT('Ctrl Pts',(17.9658314942664,3.43841557573441,1.90939449264603));
#87016=CARTESIAN_POINT('Ctrl Pts',(17.9599798266989,3.49475078627407,1.8079466953847));
#87017=CARTESIAN_POINT('Ctrl Pts',(17.9541281591314,3.5465860835206,1.70401514659803));
#87018=CARTESIAN_POINT('Ctrl Pts',(17.9482764915639,3.59371077676712,1.59804000355057));
#87019=CARTESIAN_POINT('Ctrl Pts',(17.9424228798797,3.64085112638916,1.49202965206942));
#87020=CARTESIAN_POINT('Ctrl Pts',(17.9365692681955,3.68327759220414,1.383974733776));
#87021=CARTESIAN_POINT('Ctrl Pts',(17.9307156565112,3.7208277687047,1.27433500918558));
#87022=CARTESIAN_POINT('Ctrl Pts',(17.9248553904113,3.75842063243765,1.16457064559638));
#87023=CARTESIAN_POINT('Ctrl Pts',(17.9189951243115,3.79112600842261,1.05321827103378));
#87024=CARTESIAN_POINT('Ctrl Pts',(17.9131348582116,3.81883145807233,0.940752515190457));
#87025=CARTESIAN_POINT('Ctrl Pts',(17.9072706450403,3.84655556820376,0.828211010163995));
#87026=CARTESIAN_POINT('Ctrl Pts',(17.901406431869,3.86927296559918,0.714555035009219));
#87027=CARTESIAN_POINT('Ctrl Pts',(17.8955422186977,3.88692269903637,0.600267383518262));
#87028=CARTESIAN_POINT('Ctrl Pts',(17.8896693701234,3.90459842275671,0.485811436657047));
#87029=CARTESIAN_POINT('Ctrl Pts',(17.8837965215491,3.917191544189,0.370722366361768));
#87030=CARTESIAN_POINT('Ctrl Pts',(17.8779236729748,3.92469308927438,0.255486115086346));
#87031=CARTESIAN_POINT('Ctrl Pts',(17.876328928362,3.92673009882118,0.224194249035622));
#87032=CARTESIAN_POINT('Ctrl Pts',(17.8747341837492,3.92839196811639,0.192891516277938));
#87033=CARTESIAN_POINT('Ctrl Pts',(17.8731394391363,3.92967917878615,0.161587597960445));
#87034=CARTESIAN_POINT('Ctrl Pts',(17.8672669930024,3.93441916991728,0.0463148623622432));
#87035=CARTESIAN_POINT('Ctrl Pts',(17.8613945468685,3.93409070193677,-0.0693596057384894));
#87036=CARTESIAN_POINT('Ctrl Pts',(17.8555221007346,3.92864880759938,-0.184952822492626));
#87037=CARTESIAN_POINT('Ctrl Pts',(17.8496572617897,3.92321396271262,-0.300396299353858));
#87038=CARTESIAN_POINT('Ctrl Pts',(17.8437924228449,3.91267888341305,-0.415758325086691));
#87039=CARTESIAN_POINT('Ctrl Pts',(17.8379275839,3.89705050914172,-0.530552852408001));
#87040=CARTESIAN_POINT('Ctrl Pts',(17.83206877378,3.88143820022727,-0.645229375449533));
#87041=CARTESIAN_POINT('Ctrl Pts',(17.82620996366,3.86074306587699,-0.759339153307035));
#87042=CARTESIAN_POINT('Ctrl Pts',(17.82035115354,3.83502401569583,-0.872398876109003));
#87043=CARTESIAN_POINT('Ctrl Pts',(17.814265364659,3.8083085723865,-0.989838695768315));
#87044=CARTESIAN_POINT('Ctrl Pts',(17.808179575778,3.77617209420852,-1.10614499969457));
#87045=CARTESIAN_POINT('Ctrl Pts',(17.802093786897,3.7387395994,-1.22078466892337));
#87046=CARTESIAN_POINT('Ctrl Pts',(17.7962417568188,3.70274490917848,-1.33102095966742));
#87047=CARTESIAN_POINT('Ctrl Pts',(17.7903897267405,3.66185368403598,-1.43971585758892));
#87048=CARTESIAN_POINT('Ctrl Pts',(17.7845376966622,3.61622833968109,-1.54640925866582));
#87049=CARTESIAN_POINT('Ctrl Pts',(17.7786865562837,3.57060993186908,-1.65308643886017));
#87050=CARTESIAN_POINT('Ctrl Pts',(17.7728354159052,3.52025899840678,-1.75776234728274));
#87051=CARTESIAN_POINT('Ctrl Pts',(17.7669842755267,3.46538617625046,-1.8599966799573));
#87052=CARTESIAN_POINT('Ctrl Pts',(17.7611326079592,3.41050841004128,-1.96224022396685));
#87053=CARTESIAN_POINT('Ctrl Pts',(17.7552809403917,3.35110814071534,-2.06204139068277));
#87054=CARTESIAN_POINT('Ctrl Pts',(17.7494292728242,3.2874417098647,-2.15898494766449));
#87055=CARTESIAN_POINT('Ctrl Pts',(17.74357566114,3.22375412692838,-2.25596071248945));
#87056=CARTESIAN_POINT('Ctrl Pts',(17.7377220494557,3.15579779092312,-2.35007663444583));
#87057=CARTESIAN_POINT('Ctrl Pts',(17.7318684377715,3.08387164217203,-2.44094749935496));
#87058=CARTESIAN_POINT('Ctrl Pts',(17.7260081716716,3.01186372740773,-2.53192166672735));
#87059=CARTESIAN_POINT('Ctrl Pts',(17.7201479055717,2.93587724898755,-2.61964308963168));
#87060=CARTESIAN_POINT('Ctrl Pts',(17.7142876394718,2.85625067294446,-2.70376054659142));
#87061=CARTESIAN_POINT('Ctrl Pts',(17.7084234263005,2.7765704659268,-2.78793465927364));
#87062=CARTESIAN_POINT('Ctrl Pts',(17.7025592131292,2.69324557586156,-2.86849968598149));
#87063=CARTESIAN_POINT('Ctrl Pts',(17.6966949999579,2.6066491762404,-2.94514330245665));
#87064=CARTESIAN_POINT('Ctrl Pts',(17.6908221513836,2.5199252582658,-3.02189978121959));
#87065=CARTESIAN_POINT('Ctrl Pts',(17.6849493028093,2.42992053611577,-3.09472306595429));
#87066=CARTESIAN_POINT('Ctrl Pts',(17.679076454235,2.33703893654878,-3.16334285354195));
#87067=CARTESIAN_POINT('Ctrl Pts',(17.6774817096222,2.31181737180677,-3.18197623650794));
#87068=CARTESIAN_POINT('Ctrl Pts',(17.6758869650094,2.28638382371883,-3.20029992388997));
#87069=CARTESIAN_POINT('Ctrl Pts',(17.6742922203967,2.26074669657243,-3.21830908614087));
#87070=CARTESIAN_POINT('Ctrl Pts',(17.6684197742627,2.16634120556882,-3.28462555737223));
#87071=CARTESIAN_POINT('Ctrl Pts',(17.6625473281288,2.06885720586434,-3.34689561649549));
#87072=CARTESIAN_POINT('Ctrl Pts',(17.6566748819949,1.96867667352833,-3.40482028235052));
#87073=CARTESIAN_POINT('Ctrl Pts',(17.6508100430501,1.86862591543521,-3.46266991237292));
#87074=CARTESIAN_POINT('Ctrl Pts',(17.6449452041052,1.76588592578803,-3.51618513828397));
#87075=CARTESIAN_POINT('Ctrl Pts',(17.6390803651604,1.66086932412086,-3.56510898686061));
#87076=CARTESIAN_POINT('Ctrl Pts',(17.6332215550404,1.55596067540873,-3.61398254363633));
#87077=CARTESIAN_POINT('Ctrl Pts',(17.6273627449204,1.44878044204021,-3.6582739374224));
#87078=CARTESIAN_POINT('Ctrl Pts',(17.6215039348003,1.33976704161409,-3.69777139290744));
#87079=CARTESIAN_POINT('Ctrl Pts',(17.6154181459194,1.22653030470003,-3.73879903683058));
#87080=CARTESIAN_POINT('Ctrl Pts',(17.6093323570384,1.11131588226435,-3.77465355433522));
#87081=CARTESIAN_POINT('Ctrl Pts',(17.6032465681574,0.994639837373666,-3.8051518489949));
#87082=CARTESIAN_POINT('Ctrl Pts',(17.5973945380792,0.882445389378838,-3.83447868585616));
#87083=CARTESIAN_POINT('Ctrl Pts',(17.5915425080009,0.768899968198137,-3.85885306701172));
#87084=CARTESIAN_POINT('Ctrl Pts',(17.5856904779226,0.654478437272971,-3.87816283504764));
#87085=CARTESIAN_POINT('Ctrl Pts',(17.5798393375441,0.540074302158601,-3.89746966736797));
#87086=CARTESIAN_POINT('Ctrl Pts',(17.5739881971656,0.424794729621852,-3.91171334878648));
#87087=CARTESIAN_POINT('Ctrl Pts',(17.5681370567871,0.309124000851478,-3.92083299212012));
#87088=CARTESIAN_POINT('Ctrl Pts',(17.5622853892196,0.193442850123971,-3.92995345713555));
#87089=CARTESIAN_POINT('Ctrl Pts',(17.5564337216521,0.0773708852054871,
-3.93394893380431));
#87090=CARTESIAN_POINT('Ctrl Pts',(17.5505820540846,-0.0386039901499777,
-3.93281053852642));
#87091=CARTESIAN_POINT('Ctrl Pts',(17.5447284424004,-0.154617396179694,
-3.93167176503613));
#87092=CARTESIAN_POINT('Ctrl Pts',(17.5388748307161,-0.27053323538834,-3.92539573209044));
#87093=CARTESIAN_POINT('Ctrl Pts',(17.5330212190319,-0.385865822081359,
-3.91402562170324));
#87094=CARTESIAN_POINT('Ctrl Pts',(17.527160952932,-0.50132951944777,-3.90264258571651));
#87095=CARTESIAN_POINT('Ctrl Pts',(17.5213006868321,-0.616208229278308,
-3.8861539542776));
#87096=CARTESIAN_POINT('Ctrl Pts',(17.5154404207322,-0.730023488886417,
-3.86465453898199));
#87097=CARTESIAN_POINT('Ctrl Pts',(17.5095762075609,-0.843915406610444,
-3.84314064316176));
#87098=CARTESIAN_POINT('Ctrl Pts',(17.5037119943896,-0.956742046483424,
-3.81660933773218));
#87099=CARTESIAN_POINT('Ctrl Pts',(17.4978477812183,-1.06803889982722,-3.78520566263656));
#87100=CARTESIAN_POINT('Ctrl Pts',(17.491974932644,-1.17949964441291,-3.75375574375994));
#87101=CARTESIAN_POINT('Ctrl Pts',(17.4861020840697,-1.2894257155315,-3.71741926488159));
#87102=CARTESIAN_POINT('Ctrl Pts',(17.4802292354954,-1.39737132445573,-3.67638985712735));
#87103=CARTESIAN_POINT('Ctrl Pts',(17.4786344908827,-1.426683450612,-3.66524851299863));
#87104=CARTESIAN_POINT('Ctrl Pts',(17.4770397462699,-1.45584967964805,-3.65376139101638));
#87105=CARTESIAN_POINT('Ctrl Pts',(17.4754450016571,-1.48486140462146,-3.64193294955654));
#87106=CARTESIAN_POINT('Ctrl Pts',(17.4695725555232,-1.591693426998,-3.59837620400363));
#87107=CARTESIAN_POINT('Ctrl Pts',(17.4637001093892,-1.69678615261499,-3.55004185303041));
#87108=CARTESIAN_POINT('Ctrl Pts',(17.4578276632553,-1.79968153748353,-3.49708955613678));
#87109=CARTESIAN_POINT('Ctrl Pts',(17.4519628243105,-1.90244363127891,-3.44420585385007));
#87110=CARTESIAN_POINT('Ctrl Pts',(17.4460979853656,-2.00301368073523,-3.38671628932404));
#87111=CARTESIAN_POINT('Ctrl Pts',(17.4402331464208,-2.10095241007959,-3.32482901373601));
#87112=CARTESIAN_POINT('Ctrl Pts',(17.4343743363008,-2.19879046224462,-3.26300535584431));
#87113=CARTESIAN_POINT('Ctrl Pts',(17.4285155261807,-2.29400222713966,-3.19679319824423));
#87114=CARTESIAN_POINT('Ctrl Pts',(17.4226567160607,-2.38617250060025,-3.12644683264871));
#87115=CARTESIAN_POINT('Ctrl Pts',(17.4165709271797,-2.48191358349775,-3.05337514730866));
#87116=CARTESIAN_POINT('Ctrl Pts',(17.4104851382988,-2.5743723411495,-2.9758426528553));
#87117=CARTESIAN_POINT('Ctrl Pts',(17.4043993494178,-2.66311571062527,-2.89418446402797));
#87118=CARTESIAN_POINT('Ctrl Pts',(17.3985473193395,-2.7484503940289,-2.81566281523259));
#87119=CARTESIAN_POINT('Ctrl Pts',(17.3926952892613,-2.83034951258053,-2.73332687224123));
#87120=CARTESIAN_POINT('Ctrl Pts',(17.386843259183,-2.90846195493877,-2.64751544975167));
#87121=CARTESIAN_POINT('Ctrl Pts',(17.3809921188045,-2.98656252165387,-2.56171707340174));
#87122=CARTESIAN_POINT('Ctrl Pts',(17.375140978426,-3.0608772786748,-2.4724445737531));
#87123=CARTESIAN_POINT('Ctrl Pts',(17.3692898380475,-3.13109315136304,-2.38007241013535));
#87124=CARTESIAN_POINT('Ctrl Pts',(17.36343817048,-3.20131535051627,-2.28769192376609));
#87125=CARTESIAN_POINT('Ctrl Pts',(17.3575865029125,-3.26743768102214,-2.19221154734077));
#87126=CARTESIAN_POINT('Ctrl Pts',(17.351734835345,-3.32918885536161,-2.09403690639302));
#87127=CARTESIAN_POINT('Ctrl Pts',(17.3458812236607,-3.39096054547549,-1.99582964859534));
#87128=CARTESIAN_POINT('Ctrl Pts',(17.3400276119765,-3.44835797176212,-1.8949266960883));
#87129=CARTESIAN_POINT('Ctrl Pts',(17.3341740002923,-3.50115484408842,-1.79175996096468));
#87130=CARTESIAN_POINT('Ctrl Pts',(17.3283137341924,-3.55401173616876,-1.68847594536982));
#87131=CARTESIAN_POINT('Ctrl Pts',(17.3224534680925,-3.60225744709231,-1.58292337876656));
#87132=CARTESIAN_POINT('Ctrl Pts',(17.3165932019926,-3.64571302354465,-1.4755560138324));
#87133=CARTESIAN_POINT('Ctrl Pts',(17.3107289888213,-3.68919786867878,-1.36811633363985));
#87134=CARTESIAN_POINT('Ctrl Pts',(17.30486477565,-3.72788601748201,-1.25885980992159));
#87135=CARTESIAN_POINT('Ctrl Pts',(17.2990005624787,-3.76164831424909,-1.14825561610079));
#87136=CARTESIAN_POINT('Ctrl Pts',(17.2931277139044,-3.79546032800798,-1.03748855102045));
#87137=CARTESIAN_POINT('Ctrl Pts',(17.2872548653301,-3.82433191027645,-0.925370253913503));
#87138=CARTESIAN_POINT('Ctrl Pts',(17.2813820167558,-3.84818490275428,-0.812380424563512));
#87139=CARTESIAN_POINT('Ctrl Pts',(17.279787272143,-3.85466207150327,-0.781698563899738));
#87140=CARTESIAN_POINT('Ctrl Pts',(17.2781925275302,-3.86076948077279,-0.750952467568144));
#87141=CARTESIAN_POINT('Ctrl Pts',(17.2765977829174,-3.86650622712652,-0.720151786494933));
#87142=CARTESIAN_POINT('Ctrl Pts',(17.2677944531138,-3.89817428842386,-0.550125469122141));
#87143=CARTESIAN_POINT('Ctrl Pts',(17.2589911233102,-3.9186344127923,-0.377951252578233));
#87144=CARTESIAN_POINT('Ctrl Pts',(17.2501877935066,-3.927662822198,-0.204826158299304));
#87145=CARTESIAN_POINT('Ctrl Pts',(17.2467797030161,-3.93115804922311,-0.137803111264485));
#87146=CARTESIAN_POINT('Ctrl Pts',(17.2433716125255,-3.93294038466564,-0.0706378330955611));
#87147=CARTESIAN_POINT('Ctrl Pts',(17.239963522035,-3.9329985293756,-0.00340116588511312));
#87148=CARTESIAN_POINT('',(15.989963522035,-3.92659065282687,-0.000639758371446531));
#87149=CARTESIAN_POINT('Ctrl Pts',(17.2399625682156,-3.93494441549702,-0.00338402184785404));
#87150=CARTESIAN_POINT('Ctrl Pts',(17.185891900203,-3.92519397476945,1.06388872901601));
#87151=CARTESIAN_POINT('Ctrl Pts',(17.0655388259439,-2.92427844162612,3.45556040462417));
#87152=CARTESIAN_POINT('Ctrl Pts',(16.8789033454381,1.12418408352393,4.5137789232215));
#87153=CARTESIAN_POINT('Ctrl Pts',(16.6800561266984,4.40488891136011,1.49497280909776));
#87154=CARTESIAN_POINT('Ctrl Pts',(16.4812089079589,3.63935299032934,-2.89708471280141));
#87155=CARTESIAN_POINT('Ctrl Pts',(16.2823616892191,-0.46921805946625,-4.62793954520115));
#87156=CARTESIAN_POINT('Ctrl Pts',(16.1186132272446,-3.49764510045685,-2.5525207092964));
#87157=CARTESIAN_POINT('Ctrl Pts',(16.0211471715165,-3.92748632721169,-0.619480281848567));
#87158=CARTESIAN_POINT('Ctrl Pts',(15.989963522035,-3.92659065282687,-0.000639758371446531));
#87159=CARTESIAN_POINT('',(14.7399635092212,-3.9329983210553,0.00363408533045304));
#87160=CARTESIAN_POINT('Ctrl Pts',(15.989963522035,-3.92659065282687,-0.000639758371446531));
#87161=CARTESIAN_POINT('Ctrl Pts',(15.95486476527,-3.92558252652043,0.69589619463605));
#87162=CARTESIAN_POINT('Ctrl Pts',(15.8534836022582,-3.41615124407677,2.70918611068639));
#87163=CARTESIAN_POINT('Ctrl Pts',(15.6858200330004,-0.195332983705196,
4.64756226928094));
#87164=CARTESIAN_POINT('Ctrl Pts',(15.4869728142606,3.80395226557352,2.67730035345362));
#87165=CARTESIAN_POINT('Ctrl Pts',(15.2881255955209,4.30900486257963,-1.75227484020969));
#87166=CARTESIAN_POINT('Ctrl Pts',(15.0892783767814,0.855893834375464,-4.57224624945369));
#87167=CARTESIAN_POINT('Ctrl Pts',(14.9065576856193,-3.03961470054979,-3.30416404160057));
#87168=CARTESIAN_POINT('Ctrl Pts',(14.7901194007039,-3.92350144596277,-0.987888984853184));
#87169=CARTESIAN_POINT('Ctrl Pts',(14.739963522035,-3.93258919388794,0.00363345398641773));
#87170=CARTESIAN_POINT('',(13.4899631080426,-3.93529776951097,-0.00102838428343817));
#87171=CARTESIAN_POINT('Ctrl Pts',(14.7399635092212,-3.9329983210553,0.00363408533045304));
#87172=CARTESIAN_POINT('Ctrl Pts',(14.7323650281588,-3.93285951130317,0.15386130138135));
#87173=CARTESIAN_POINT('Ctrl Pts',(14.7247665470964,-3.92410999965482,0.30370417608665));
#87174=CARTESIAN_POINT('Ctrl Pts',(14.717168066034,-3.90690212688664,0.452332588842152));
#87175=CARTESIAN_POINT('Ctrl Pts',(14.7093791901893,-3.8892630772605,0.604685176739965));
#87176=CARTESIAN_POINT('Ctrl Pts',(14.7015903143445,-3.86273644131324,0.755762030018039));
#87177=CARTESIAN_POINT('Ctrl Pts',(14.6938014384998,-3.82753406574427,0.904694410045241));
#87178=CARTESIAN_POINT('Ctrl Pts',(14.6930622721006,-3.82419335089489,0.91882813271221));
#87179=CARTESIAN_POINT('Ctrl Pts',(14.6923231057013,-3.82077453694752,0.932942558131614));
#87180=CARTESIAN_POINT('Ctrl Pts',(14.6915839393021,-3.8172778270376,0.947036953453815));
#87181=CARTESIAN_POINT('Ctrl Pts',(14.6857114931682,-3.78949755914025,1.05901252134163));
#87182=CARTESIAN_POINT('Ctrl Pts',(14.6798390470342,-3.75673958706406,1.16995217037249));
#87183=CARTESIAN_POINT('Ctrl Pts',(14.6739666009003,-3.71909620862784,1.27937968991619));
#87184=CARTESIAN_POINT('Ctrl Pts',(14.6681017619555,-3.6815015935673,1.38866545663461));
#87185=CARTESIAN_POINT('Ctrl Pts',(14.6622369230106,-3.63903429065255,1.49644260198653));
#87186=CARTESIAN_POINT('Ctrl Pts',(14.6563720840658,-3.59183728025604,1.60224653289153));
#87187=CARTESIAN_POINT('Ctrl Pts',(14.6505132739458,-3.54468878653844,1.70794170149779));
#87188=CARTESIAN_POINT('Ctrl Pts',(14.6446544638257,-3.49282042341684,1.8116673149959));
#87189=CARTESIAN_POINT('Ctrl Pts',(14.6387956537057,-3.4364242878107,1.91297598368216));
#87190=CARTESIAN_POINT('Ctrl Pts',(14.6327098648247,-3.37784328450623,2.01820949642721));
#87191=CARTESIAN_POINT('Ctrl Pts',(14.6266240759438,-3.31437673623003,2.12083457529475));
#87192=CARTESIAN_POINT('Ctrl Pts',(14.6205382870628,-3.24629416493512,2.22037456180442));
#87193=CARTESIAN_POINT('Ctrl Pts',(14.6146862569845,-3.18082668605661,2.31609115770327));
#87194=CARTESIAN_POINT('Ctrl Pts',(14.6088342269062,-3.11109150630972,2.40895491723037));
#87195=CARTESIAN_POINT('Ctrl Pts',(14.602982196828,-3.03737356597209,2.49856975502667));
#87196=CARTESIAN_POINT('Ctrl Pts',(14.5971310564494,-2.96366683316973,2.58817096843992));
#87197=CARTESIAN_POINT('Ctrl Pts',(14.5912799160709,-2.8859788062546,2.67452392310072));
#87198=CARTESIAN_POINT('Ctrl Pts',(14.5854287756924,-2.80463515812238,2.75726506339595));
#87199=CARTESIAN_POINT('Ctrl Pts',(14.5795771081249,-2.72328418091027,2.8400136586854));
#87200=CARTESIAN_POINT('Ctrl Pts',(14.5737254405574,-2.63827721752455,2.91914949791004));
#87201=CARTESIAN_POINT('Ctrl Pts',(14.5678737729899,-2.54997677940284,2.9943459092941));
#87202=CARTESIAN_POINT('Ctrl Pts',(14.5620201613056,-2.46164700496657,3.06956730340333));
#87203=CARTESIAN_POINT('Ctrl Pts',(14.5561665496214,-2.37002189458091,3.14084639932784));
#87204=CARTESIAN_POINT('Ctrl Pts',(14.5503129379371,-2.27549642959328,3.20789728621542));
#87205=CARTESIAN_POINT('Ctrl Pts',(14.5444526718372,-2.18086350757442,3.27502439689356));
#87206=CARTESIAN_POINT('Ctrl Pts',(14.5385924057373,-2.08332398732458,3.33791346532767));
#87207=CARTESIAN_POINT('Ctrl Pts',(14.5327321396374,-1.98330125572515,3.39632229463563));
#87208=CARTESIAN_POINT('Ctrl Pts',(14.5268679264661,-1.88321115570634,3.45477046410603));
#87209=CARTESIAN_POINT('Ctrl Pts',(14.5210037132948,-1.78063487894454,3.50873219386432));
#87210=CARTESIAN_POINT('Ctrl Pts',(14.5151395001235,-1.67601821744151,3.55801235731471));
#87211=CARTESIAN_POINT('Ctrl Pts',(14.5092666515492,-1.57124750167656,3.60736508873945));
#87212=CARTESIAN_POINT('Ctrl Pts',(14.5033938029749,-1.46443078454555,3.6520223361943));
#87213=CARTESIAN_POINT('Ctrl Pts',(14.4975209544006,-1.35603159153177,3.69183793289573));
#87214=CARTESIAN_POINT('Ctrl Pts',(14.4959262097878,-1.32659629673441,3.70264967229946));
#87215=CARTESIAN_POINT('Ctrl Pts',(14.4943314651751,-1.29704438562647,3.71310469202366));
#87216=CARTESIAN_POINT('Ctrl Pts',(14.4927367205623,-1.26738527970299,3.72320071347116));
#87217=CARTESIAN_POINT('Ctrl Pts',(14.4868642744284,-1.15816935853068,3.76037804057635));
#87218=CARTESIAN_POINT('Ctrl Pts',(14.4809918282945,-1.04713336591795,3.79280794662146));
#87219=CARTESIAN_POINT('Ctrl Pts',(14.4751193821606,-0.934727800867599,
3.82031058139063));
#87220=CARTESIAN_POINT('Ctrl Pts',(14.4692545432157,-0.822467846414021,
3.84777758914205));
#87221=CARTESIAN_POINT('Ctrl Pts',(14.4633897042709,-0.70884224548679,3.87032992141478));
#87222=CARTESIAN_POINT('Ctrl Pts',(14.457524865326,-0.594319128877981,3.88783664433702));
#87223=CARTESIAN_POINT('Ctrl Pts',(14.451666055206,-0.479913737549473,3.90532537103348));
#87224=CARTESIAN_POINT('Ctrl Pts',(14.445807245086,-0.364613071820371,3.91777874290011));
#87225=CARTESIAN_POINT('Ctrl Pts',(14.439948434966,-0.248897348668801,3.92511644538422));
#87226=CARTESIAN_POINT('Ctrl Pts',(14.433862646085,-0.12869863137231,3.93273842105418));
#87227=CARTESIAN_POINT('Ctrl Pts',(14.4277768572041,-0.00805248771519723,
3.93484022583765));
#87228=CARTESIAN_POINT('Ctrl Pts',(14.4216910683231,0.11249437966016,3.93139084988314));
#87229=CARTESIAN_POINT('Ctrl Pts',(14.4158390382448,0.228410969525238,3.92807396652885));
#87230=CARTESIAN_POINT('Ctrl Pts',(14.4099870081666,0.344235317561232,3.91962449732425));
#87231=CARTESIAN_POINT('Ctrl Pts',(14.4041349780883,0.459480163107657,3.90606796916164));
#87232=CARTESIAN_POINT('Ctrl Pts',(14.3982838377098,0.574707487672586,3.8925135020342));
#87233=CARTESIAN_POINT('Ctrl Pts',(14.3924326973313,0.68935507451161,3.87385356804228));
#87234=CARTESIAN_POINT('Ctrl Pts',(14.3865815569528,0.802941002732841,3.85016554788627));
#87235=CARTESIAN_POINT('Ctrl Pts',(14.3807298893853,0.916537165070234,3.82647539343463));
#87236=CARTESIAN_POINT('Ctrl Pts',(14.3748782218178,1.02907107395979,3.79775633662782));
#87237=CARTESIAN_POINT('Ctrl Pts',(14.3690265542503,1.14007191654556,3.76413669054461));
#87238=CARTESIAN_POINT('Ctrl Pts',(14.3631729425661,1.25110963726782,3.73050587490748));
#87239=CARTESIAN_POINT('Ctrl Pts',(14.3573193308819,1.36061288350438,3.6919713523002));
#87240=CARTESIAN_POINT('Ctrl Pts',(14.3514657191977,1.46812757403888,3.64871078962785));
#87241=CARTESIAN_POINT('Ctrl Pts',(14.3456054530978,1.57576448782272,3.60540104812691));
#87242=CARTESIAN_POINT('Ctrl Pts',(14.3397451869979,1.68140795011717,3.55735469744872));
#87243=CARTESIAN_POINT('Ctrl Pts',(14.333884920898,1.78462529312407,3.50479693607801));
#87244=CARTESIAN_POINT('Ctrl Pts',(14.3280207077267,1.88791215622052,3.45220377542099));
#87245=CARTESIAN_POINT('Ctrl Pts',(14.3221564945554,1.98876928745983,3.39509335683575));
#87246=CARTESIAN_POINT('Ctrl Pts',(14.3162922813841,2.08679150031032,3.33373517757974));
#87247=CARTESIAN_POINT('Ctrl Pts',(14.3104194328098,2.18495805670444,3.27228664475215));
#87248=CARTESIAN_POINT('Ctrl Pts',(14.3045465842355,2.28028102401497,3.20657810107659));
#87249=CARTESIAN_POINT('Ctrl Pts',(14.2986737356612,2.37238681246571,3.13692043444503));
#87250=CARTESIAN_POINT('Ctrl Pts',(14.2970789910484,2.39739770932159,3.11800522026959));
#87251=CARTESIAN_POINT('Ctrl Pts',(14.2954842464356,2.42217158603637,3.09879902543088));
#87252=CARTESIAN_POINT('Ctrl Pts',(14.2938895018228,2.44670143153496,3.07930854331371));
#87253=CARTESIAN_POINT('Ctrl Pts',(14.2880170556889,2.53702949736151,3.00753729829005));
#87254=CARTESIAN_POINT('Ctrl Pts',(14.2821446095549,2.62434812153707,2.93166801376936));
#87255=CARTESIAN_POINT('Ctrl Pts',(14.276272163421,2.70826242303331,2.85198240667535));
#87256=CARTESIAN_POINT('Ctrl Pts',(14.2704073244762,2.79206802162401,2.77240002462006));
#87257=CARTESIAN_POINT('Ctrl Pts',(14.2645424855313,2.87247777042338,2.68901143322388));
#87258=CARTESIAN_POINT('Ctrl Pts',(14.2586776465865,2.94912840357876,2.60213963099696));
#87259=CARTESIAN_POINT('Ctrl Pts',(14.2528188364665,3.02570024288419,2.51535712958161));
#87260=CARTESIAN_POINT('Ctrl Pts',(14.2469600263465,3.09852038085622,2.42509884744537));
#87261=CARTESIAN_POINT('Ctrl Pts',(14.2411012162264,3.16726159794009,2.33172532048995));
#87262=CARTESIAN_POINT('Ctrl Pts',(14.2350154273455,3.23866594899831,2.23473436832026));
#87263=CARTESIAN_POINT('Ctrl Pts',(14.2289296384645,3.30566861111373,2.13438222418711));
#87264=CARTESIAN_POINT('Ctrl Pts',(14.2228438495835,3.36794789080634,2.03111201188244));
#87265=CARTESIAN_POINT('Ctrl Pts',(14.2169918195052,3.42783498599518,1.93180847039984));
#87266=CARTESIAN_POINT('Ctrl Pts',(14.211139789427,3.4833546281127,1.82980728184328));
#87267=CARTESIAN_POINT('Ctrl Pts',(14.2052877593487,3.53426482377998,1.72553213687589));
#87268=CARTESIAN_POINT('Ctrl Pts',(14.1994366189702,3.58516727943433,1.6212728451371));
#87269=CARTESIAN_POINT('Ctrl Pts',(14.1935854785917,3.631461500727,1.51474065573167));
#87270=CARTESIAN_POINT('Ctrl Pts',(14.1877343382131,3.67295200143222,1.40638280534676));
#87271=CARTESIAN_POINT('Ctrl Pts',(14.1818826706456,3.71444624044032,1.29801519189666));
#87272=CARTESIAN_POINT('Ctrl Pts',(14.1760310030781,3.75113575064304,1.18782197652054));
#87273=CARTESIAN_POINT('Ctrl Pts',(14.1701793355106,3.78287389681412,1.07626859138524));
#87274=CARTESIAN_POINT('Ctrl Pts',(14.1643257238264,3.8146225874429,0.964678144540481));
#87275=CARTESIAN_POINT('Ctrl Pts',(14.1584721121422,3.84141652998987,0.85172702674279));
#87276=CARTESIAN_POINT('Ctrl Pts',(14.1526185004579,3.86315965307619,0.737893281473863));
#87277=CARTESIAN_POINT('Ctrl Pts',(14.146758234358,3.88492749385586,0.623930129422035));
#87278=CARTESIAN_POINT('Ctrl Pts',(14.1408979682581,3.9016329771412,0.509082753451748));
#87279=CARTESIAN_POINT('Ctrl Pts',(14.1350377021582,3.91323159399635,0.393836884698193));
#87280=CARTESIAN_POINT('Ctrl Pts',(14.1291734889869,3.92483802288055,0.278513394269038));
#87281=CARTESIAN_POINT('Ctrl Pts',(14.1233092758156,3.93133071323441,0.16279128832216));
#87282=CARTESIAN_POINT('Ctrl Pts',(14.1174450626443,3.93271728004675,0.0471571333064215));
#87283=CARTESIAN_POINT('Ctrl Pts',(14.11157221407,3.93410588866127,-0.0686472998861706));
#87284=CARTESIAN_POINT('Ctrl Pts',(14.1056993654957,3.93037338044257,-0.184363112078128));
#87285=CARTESIAN_POINT('Ctrl Pts',(14.0998265169215,3.92157927323944,-0.299507935953051));
#87286=CARTESIAN_POINT('Ctrl Pts',(14.0982317723086,3.91919127448394,-0.330774975319696));
#87287=CARTESIAN_POINT('Ctrl Pts',(14.0966370276958,3.91643034098348,-0.361999967454853));
#87288=CARTESIAN_POINT('Ctrl Pts',(14.095042283083,3.91329831231293,-0.393173395397972));
#87289=CARTESIAN_POINT('Ctrl Pts',(14.0891698369491,3.90176501130031,-0.507965616632582));
#87290=CARTESIAN_POINT('Ctrl Pts',(14.0832973908152,3.88515716701732,-0.622442120640527));
#87291=CARTESIAN_POINT('Ctrl Pts',(14.0774249446813,3.86349824603618,-0.736118402755522));
#87292=CARTESIAN_POINT('Ctrl Pts',(14.0715601057364,3.84186738210372,-0.849647428182004));
#87293=CARTESIAN_POINT('Ctrl Pts',(14.0656952667916,3.81519853019166,-0.962377890856129));
#87294=CARTESIAN_POINT('Ctrl Pts',(14.0598304278468,3.7835669779599,-1.07382955970274));
#87295=CARTESIAN_POINT('Ctrl Pts',(14.0539716177267,3.75196794172543,-1.18516666059724));
#87296=CARTESIAN_POINT('Ctrl Pts',(14.0481128076067,3.71541646443954,-1.29522718711191));
#87297=CARTESIAN_POINT('Ctrl Pts',(14.0422539974867,3.67403890115292,-1.40354093378676));
#87298=CARTESIAN_POINT('Ctrl Pts',(14.0361682086057,3.63105831133817,-1.51605091135319));
#87299=CARTESIAN_POINT('Ctrl Pts',(14.0300824197247,3.58287021860048,-1.62667557985427));
#87300=CARTESIAN_POINT('Ctrl Pts',(14.0239966308438,3.52967343966517,-1.73490472629544));
#87301=CARTESIAN_POINT('Ctrl Pts',(14.0181446007655,3.47851998092954,-1.8389767262788));
#87302=CARTESIAN_POINT('Ctrl Pts',(14.0122925706873,3.4227357108332,-1.94083343120115));
#87303=CARTESIAN_POINT('Ctrl Pts',(14.006440540609,3.362546193441,-2.04004218019516));
#87304=CARTESIAN_POINT('Ctrl Pts',(14.0005894002305,3.3023658268218,-2.13923584621824));
#87305=CARTESIAN_POINT('Ctrl Pts',(13.994738259852,3.23778175892049,-2.23578200345887));
#87306=CARTESIAN_POINT('Ctrl Pts',(13.9888871194734,3.16906450782115,-2.32927438170523));
#87307=CARTESIAN_POINT('Ctrl Pts',(13.983035451906,3.10034106528297,-2.42277518363463));
#87308=CARTESIAN_POINT('Ctrl Pts',(13.9771837843385,3.0274839440693,-2.51322132651705));
#87309=CARTESIAN_POINT('Ctrl Pts',(13.971332116771,2.95080538269953,-2.60023779555476));
#87310=CARTESIAN_POINT('Ctrl Pts',(13.9654785050867,2.87410134618564,-2.68728317433008));
#87311=CARTESIAN_POINT('Ctrl Pts',(13.9596248934025,2.79357361811643,-2.77089630356811));
#87312=CARTESIAN_POINT('Ctrl Pts',(13.9537712817183,2.70957238615181,-2.85073788416326));
#87313=CARTESIAN_POINT('Ctrl Pts',(13.9479110156184,2.62547566115773,-2.93067022907494));
#87314=CARTESIAN_POINT('Ctrl Pts',(13.9420507495185,2.53789785058966,-3.0068221826623));
#87315=CARTESIAN_POINT('Ctrl Pts',(13.9361904834186,2.44722348937104,-3.07889366381346));
#87316=CARTESIAN_POINT('Ctrl Pts',(13.9303262702473,2.35648805615109,-3.15101368734784));
#87317=CARTESIAN_POINT('Ctrl Pts',(13.924462057076,2.26265225322036,-3.21904752393788));
#87318=CARTESIAN_POINT('Ctrl Pts',(13.9185978439047,2.16612950211537,-3.2827384879191));
#87319=CARTESIAN_POINT('Ctrl Pts',(13.9127249953304,2.06946461551345,-3.34652324063628));
#87320=CARTESIAN_POINT('Ctrl Pts',(13.9068521467561,1.97010523737935,-3.40595214594057));
#87321=CARTESIAN_POINT('Ctrl Pts',(13.9009792981818,1.86848932130979,-3.46081444982988));
#87322=CARTESIAN_POINT('Ctrl Pts',(13.899384553569,1.84089599369804,-3.47571205232472));
#87323=CARTESIAN_POINT('Ctrl Pts',(13.8977898089563,1.81313638695708,-3.49027320341912));
#87324=CARTESIAN_POINT('Ctrl Pts',(13.8961950643435,1.78521950151592,-3.50449430466184));
#87325=CARTESIAN_POINT('Ctrl Pts',(13.8903226182096,1.68241908779071,-3.55686171844305));
#87326=CARTESIAN_POINT('Ctrl Pts',(13.8844501720757,1.57714040070536,-3.60478966965293));
#87327=CARTESIAN_POINT('Ctrl Pts',(13.8785777259417,1.46980369851994,-3.64803592194719));
#87328=CARTESIAN_POINT('Ctrl Pts',(13.8727128869969,1.36260604070707,-3.69122615288163));
#87329=CARTESIAN_POINT('Ctrl Pts',(13.8668480480521,1.25335604931443,-3.7297465923615));
#87330=CARTESIAN_POINT('Ctrl Pts',(13.8609832091072,1.14249840781187,-3.76340090717789));
#87331=CARTESIAN_POINT('Ctrl Pts',(13.8551243989872,1.0317547236246,-3.79702062667624));
#87332=CARTESIAN_POINT('Ctrl Pts',(13.8492655888672,0.919407069599642,-3.82578405177716));
#87333=CARTESIAN_POINT('Ctrl Pts',(13.8434067787472,0.8059193082311,-3.84954322856885));
#87334=CARTESIAN_POINT('Ctrl Pts',(13.8373209898662,0.688034867173198,-3.87422287016465));
#87335=CARTESIAN_POINT('Ctrl Pts',(13.8312352009852,0.568920614755863,-3.89350250796558));
#87336=CARTESIAN_POINT('Ctrl Pts',(13.8251494121042,0.449113248937317,-3.90727351098294));
#87337=CARTESIAN_POINT('Ctrl Pts',(13.819297382026,0.333907755930442,-3.92051556151109));
#87338=CARTESIAN_POINT('Ctrl Pts',(13.8134453519477,0.218061861757758,-3.92866429952059));
#87339=CARTESIAN_POINT('Ctrl Pts',(13.8075933218694,0.102061489397147,-3.93167552735243));
#87340=CARTESIAN_POINT('Ctrl Pts',(13.8017421814909,-0.0139212471172105,
-3.93468629737927));
#87341=CARTESIAN_POINT('Ctrl Pts',(13.7958910411124,-0.130058002017154,
-3.93256109952536));
#87342=CARTESIAN_POINT('Ctrl Pts',(13.7900399007339,-0.245860745280993,
-3.92530782155105));
#87343=CARTESIAN_POINT('Ctrl Pts',(13.7841882331664,-0.361673922396517,
-3.91805389005486));
#87344=CARTESIAN_POINT('Ctrl Pts',(13.7783365655989,-0.477152615477489,
-3.90567098578471));
#87345=CARTESIAN_POINT('Ctrl Pts',(13.7724848980314,-0.591812528168616,
-3.88821899222545));
#87346=CARTESIAN_POINT('Ctrl Pts',(13.7666312863472,-0.706510534659967,
-3.870761200539));
#87347=CARTESIAN_POINT('Ctrl Pts',(13.7607776746629,-0.820388811420534,
-3.848231032963));
#87348=CARTESIAN_POINT('Ctrl Pts',(13.7549240629787,-0.932972586964773,
-3.82073960797805));
#87349=CARTESIAN_POINT('Ctrl Pts',(13.7490637968788,-1.04568434831993,-3.7932169306008));
#87350=CARTESIAN_POINT('Ctrl Pts',(13.7432035307789,-1.15709826940755,-3.76072183671057));
#87351=CARTESIAN_POINT('Ctrl Pts',(13.737343264679,-1.26675399735092,-3.723415543583));
#87352=CARTESIAN_POINT('Ctrl Pts',(13.7314790515077,-1.3764835818362,-3.68608412350716));
#87353=CARTESIAN_POINT('Ctrl Pts',(13.7256148383364,-1.48445223108702,-3.64393520167339));
#87354=CARTESIAN_POINT('Ctrl Pts',(13.7197506251651,-1.59022047757638,-3.59717775939649));
#87355=CARTESIAN_POINT('Ctrl Pts',(13.7138777765908,-1.69614447410502,-3.55035146400239));
#87356=CARTESIAN_POINT('Ctrl Pts',(13.7080049280165,-1.79986123212222,-3.49890328701583));
#87357=CARTESIAN_POINT('Ctrl Pts',(13.7021320794423,-1.9009566574887,-3.44308768205943));
#87358=CARTESIAN_POINT('Ctrl Pts',(13.7005373348294,-1.92840864828039,-3.4279312151101));
#87359=CARTESIAN_POINT('Ctrl Pts',(13.6989425902166,-1.95566752198257,-3.41245294995782));
#87360=CARTESIAN_POINT('Ctrl Pts',(13.6973478456038,-1.98272538492187,-3.39665851212429));
#87361=CARTESIAN_POINT('Ctrl Pts',(13.6914753994699,-2.0823625565004,-3.33849748455399));
#87362=CARTESIAN_POINT('Ctrl Pts',(13.685602953336,-2.17960524037133,-3.27585124847258));
#87363=CARTESIAN_POINT('Ctrl Pts',(13.6797305072021,-2.27402242721818,-3.20894234920304));
#87364=CARTESIAN_POINT('Ctrl Pts',(13.6738656682572,-2.36831730568186,-3.14212012397626));
#87365=CARTESIAN_POINT('Ctrl Pts',(13.6680008293124,-2.45979363172764,-3.07104645339295));
#87366=CARTESIAN_POINT('Ctrl Pts',(13.6621359903676,-2.5480458032047,-2.99598924977559));
#87367=CARTESIAN_POINT('Ctrl Pts',(13.6562771802475,-2.63620725490464,-2.92100920202499));
#87368=CARTESIAN_POINT('Ctrl Pts',(13.6504183701275,-2.72115083138239,-2.84205403244364));
#87369=CARTESIAN_POINT('Ctrl Pts',(13.6445595600075,-2.80250125728835,-2.75943394610149));
#87370=CARTESIAN_POINT('Ctrl Pts',(13.6384737711265,-2.8870033161192,-2.67361303835645));
#87371=CARTESIAN_POINT('Ctrl Pts',(13.6323879822455,-2.96762781521578,-2.58383776498953));
#87372=CARTESIAN_POINT('Ctrl Pts',(13.6263021933646,-3.04399317514067,-2.49050086321949));
#87373=CARTESIAN_POINT('Ctrl Pts',(13.6204501632863,-3.11742529576768,-2.4007490878534));
#87374=CARTESIAN_POINT('Ctrl Pts',(13.614598133208,-3.18691914796908,-2.3077045950877));
#87375=CARTESIAN_POINT('Ctrl Pts',(13.6087461031298,-3.25217480875052,-2.21175224953622));
#87376=CARTESIAN_POINT('Ctrl Pts',(13.6028949627513,-3.31742054853965,-2.11581449187598));
#87377=CARTESIAN_POINT('Ctrl Pts',(13.5970438223727,-3.37842914568288,-2.01697010215551));
#87378=CARTESIAN_POINT('Ctrl Pts',(13.5911926819942,-3.43494335260479,-1.91563388057221));
#87379=CARTESIAN_POINT('Ctrl Pts',(13.5853410144267,-3.49146265146869,-1.81428852857393));
#87380=CARTESIAN_POINT('Ctrl Pts',(13.5794893468592,-3.54348655377244,-1.71045125943168));
#87381=CARTESIAN_POINT('Ctrl Pts',(13.5736376792917,-3.5908035700392,-1.60456184717003));
#87382=CARTESIAN_POINT('Ctrl Pts',(13.5677840676075,-3.63813630657747,-1.49863725495746));
#87383=CARTESIAN_POINT('Ctrl Pts',(13.5619304559233,-3.6807588790428,-1.39065954112105));
#87384=CARTESIAN_POINT('Ctrl Pts',(13.5560768442391,-3.7185080474881,-1.28108817056683));
#87385=CARTESIAN_POINT('Ctrl Pts',(13.5502165781392,-3.75630012938088,-1.17139223871892));
#87386=CARTESIAN_POINT('Ctrl Pts',(13.5443563120393,-3.78920761465667,-1.06009942515104));
#87387=CARTESIAN_POINT('Ctrl Pts',(13.5384960459394,-3.81711720321073,-0.947684154638398));
#87388=CARTESIAN_POINT('Ctrl Pts',(13.5326318327681,-3.84504558974039,-0.835193168946053));
#87389=CARTESIAN_POINT('Ctrl Pts',(13.5267676195968,-3.86796929513556,-0.721578625142255));
#87390=CARTESIAN_POINT('Ctrl Pts',(13.5209034064255,-3.88582649174952,-0.607323205564899));
#87391=CARTESIAN_POINT('Ctrl Pts',(13.5150305578512,-3.90370998414853,-0.492899538080586));
#87392=CARTESIAN_POINT('Ctrl Pts',(13.5091577092769,-3.91651203208837,-0.377833520606281));
#87393=CARTESIAN_POINT('Ctrl Pts',(13.5032848607027,-3.92422277928354,-0.262611078502395));
#87394=CARTESIAN_POINT('Ctrl Pts',(13.5016901160898,-3.9263165966866,-0.231322962267526));
#87395=CARTESIAN_POINT('Ctrl Pts',(13.500095371477,-3.92803529418511,-0.200023298266526));
#87396=CARTESIAN_POINT('Ctrl Pts',(13.4985006268642,-3.92937933582806,-0.168721768504988));
#87397=CARTESIAN_POINT('Ctrl Pts',(13.4956549252544,-3.93177767687659,-0.112866546977301));
#87398=CARTESIAN_POINT('Ctrl Pts',(13.4928092236447,-3.93298513356625,-0.056959824101717));
#87399=CARTESIAN_POINT('Ctrl Pts',(13.489963522035,-3.93299986357157,-0.00103592761850977));
#87400=CARTESIAN_POINT('',(12.239963913861,-3.93201440718328,-0.00312379772517306));
#87401=CARTESIAN_POINT('Ctrl Pts',(13.4899624084639,-3.93918085105486,-0.001015637292931));
#87402=CARTESIAN_POINT('Ctrl Pts',(13.4265260750175,-3.93478655511187,1.24759946057853));
#87403=CARTESIAN_POINT('Ctrl Pts',(13.2968073353243,-2.61735902960304,3.80880663961671));
#87404=CARTESIAN_POINT('Ctrl Pts',(13.1008061893849,1.74836256028053,4.31059373859052));
#87405=CARTESIAN_POINT('Ctrl Pts',(12.9019589706453,4.57146741630123,0.860044000654414));
#87406=CARTESIAN_POINT('Ctrl Pts',(12.7031117519055,3.19531592007835,-3.38052454395175));
#87407=CARTESIAN_POINT('Ctrl Pts',(12.504264533166,-1.11598734534858,-4.51581247024143));
#87408=CARTESIAN_POINT('Ctrl Pts',(12.3498822614166,-3.66733284149021,-2.17668070861014));
#87409=CARTESIAN_POINT('Ctrl Pts',(12.2617823959138,-3.93262971169265,-0.435322618273008));
#87410=CARTESIAN_POINT('Ctrl Pts',(12.2399649366575,-3.92944490519375,-0.00314202184111889));
#87411=CARTESIAN_POINT('',(10.9899630120657,-3.93123823607095,0.00233406685951829));
#87412=CARTESIAN_POINT('Ctrl Pts',(12.239963522035,-3.93299876499558,-0.00311681619685484));
#87413=CARTESIAN_POINT('Ctrl Pts',(12.2341198337128,-3.93309058247703,0.11274437622992));
#87414=CARTESIAN_POINT('Ctrl Pts',(12.2282761453906,-3.9280584152009,0.228670229510765));
#87415=CARTESIAN_POINT('Ctrl Pts',(12.2224324570685,-3.91791188187092,0.344173627540887));
#87416=CARTESIAN_POINT('Ctrl Pts',(12.216589862448,-3.90776724756089,0.459655408014585));
#87417=CARTESIAN_POINT('Ctrl Pts',(12.2107472678275,-3.89251018623907,0.574714478005286));
#87418=CARTESIAN_POINT('Ctrl Pts',(12.204904673207,-3.87220232072403,0.688867322043548));
#87419=CARTESIAN_POINT('Ctrl Pts',(12.1990617509642,-3.85189331644964,0.803026567178875));
#87420=CARTESIAN_POINT('Ctrl Pts',(12.1932188287215,-3.82653301736519,0.916279077516074));
#87421=CARTESIAN_POINT('Ctrl Pts',(12.1873759064787,-3.79623432426462,1.02815074540416));
#87422=CARTESIAN_POINT('Ctrl Pts',(12.181531235386,-3.76592656243685,1.14005589769482));
#87423=CARTESIAN_POINT('Ctrl Pts',(12.1756865642933,-3.73067757563759,1.25057898607222));
#87424=CARTESIAN_POINT('Ctrl Pts',(12.1698418932006,-3.69065015226566,1.35926099538736));
#87425=CARTESIAN_POINT('Ctrl Pts',(12.1639903674728,-3.65057578469843,1.46807046705312));
#87426=CARTESIAN_POINT('Ctrl Pts',(12.158138841745,-3.60571193471527,1.57503415949148));
#87427=CARTESIAN_POINT('Ctrl Pts',(12.1522873160171,-3.55626965542888,1.67971281410715));
#87428=CARTESIAN_POINT('Ctrl Pts',(12.1464320218302,-3.50679553466756,1.78445888314635));
#87429=CARTESIAN_POINT('Ctrl Pts',(12.1405767276432,-3.45273730610917,1.8869166182753));
#87430=CARTESIAN_POINT('Ctrl Pts',(12.1347214334563,-3.39435122124357,1.98667279309962));
#87431=CARTESIAN_POINT('Ctrl Pts',(12.1288565851549,-3.33586986749531,2.08659174060062));
#87432=CARTESIAN_POINT('Ctrl Pts',(12.1229917368535,-3.2730467801339,2.18379997792449));
#87433=CARTESIAN_POINT('Ctrl Pts',(12.1171268885522,-3.20618080333904,2.27791432154509));
#87434=CARTESIAN_POINT('Ctrl Pts',(12.113607957597,-3.16606096672959,2.3343832803438));
#87435=CARTESIAN_POINT('Ctrl Pts',(12.1100890266418,-3.12448644944354,2.38973906388321));
#87436=CARTESIAN_POINT('Ctrl Pts',(12.1065700956867,-3.08152830119491,2.44390513910315));
#87437=CARTESIAN_POINT('Ctrl Pts',(12.1006976495528,-3.00983908227655,2.53429831903999));
#87438=CARTESIAN_POINT('Ctrl Pts',(12.0948252034189,-2.93404909368788,2.62168577861705));
#87439=CARTESIAN_POINT('Ctrl Pts',(12.0889527572849,-2.85443969377792,2.70567238123632));
#87440=CARTESIAN_POINT('Ctrl Pts',(12.0830879183401,-2.77493342018747,2.78955018729103));
#87441=CARTESIAN_POINT('Ctrl Pts',(12.0772230793952,-2.69161785619536,2.87003560009203));
#87442=CARTESIAN_POINT('Ctrl Pts',(12.0713582404504,-2.60481567041912,2.94676506072999));
#87443=CARTESIAN_POINT('Ctrl Pts',(12.0654994303303,-2.5181027138914,3.0234156464865));
#87444=CARTESIAN_POINT('Ctrl Pts',(12.0596406202103,-2.42791057241676,3.09631768764274));
#87445=CARTESIAN_POINT('Ctrl Pts',(12.0537818100903,-2.33459948471038,3.16514363749736));
#87446=CARTESIAN_POINT('Ctrl Pts',(12.0476960212093,-2.23767339077667,3.23663600399595));
#87447=CARTESIAN_POINT('Ctrl Pts',(12.0416102323283,-2.13738211057119,3.30372973453318));
#87448=CARTESIAN_POINT('Ctrl Pts',(12.0355244434474,-2.03416847568164,3.36610273350993));
#87449=CARTESIAN_POINT('Ctrl Pts',(12.0296724133691,-1.93491933844161,3.42607994816902));
#87450=CARTESIAN_POINT('Ctrl Pts',(12.0238203832908,-1.83296859062397,3.48169216038219));
#87451=CARTESIAN_POINT('Ctrl Pts',(12.0179683532126,-1.7287397030445,3.53269699225926));
#87452=CARTESIAN_POINT('Ctrl Pts',(12.0121172128341,-1.62452666166115,3.58369406973552));
#87453=CARTESIAN_POINT('Ctrl Pts',(12.0062660724556,-1.51803654036001,3.63008497800266));
#87454=CARTESIAN_POINT('Ctrl Pts',(12.000414932077,-1.4097163981887,3.67167382493024));
#87455=CARTESIAN_POINT('Ctrl Pts',(11.9945632645096,-1.30138649634974,3.7132664190217));
#87456=CARTESIAN_POINT('Ctrl Pts',(11.9887115969421,-1.19122663177882,3.75005594350249));
#87457=CARTESIAN_POINT('Ctrl Pts',(11.9828599293746,-1.07970210334088,3.78189534070435));
#87458=CARTESIAN_POINT('Ctrl Pts',(11.9770063176903,-0.968140522780236,
3.81374531600296));
#87459=CARTESIAN_POINT('Ctrl Pts',(11.9711527060061,-0.855213774087097,
3.84064178042879));
#87460=CARTESIAN_POINT('Ctrl Pts',(11.9652990943218,-0.741399813336094,
3.86248822869212));
#87461=CARTESIAN_POINT('Ctrl Pts',(11.9594388282219,-0.627456468293577,
3.88435951210934));
#87462=CARTESIAN_POINT('Ctrl Pts',(11.953578562122,-0.512624304272825,3.90116924278434));
#87463=CARTESIAN_POINT('Ctrl Pts',(11.9477182960222,-0.39738901180531,3.91287247087052));
#87464=CARTESIAN_POINT('Ctrl Pts',(11.9418540828509,-0.282076104785633,
3.92458358144468));
#87465=CARTESIAN_POINT('Ctrl Pts',(11.9359898696795,-0.166359940346541,
3.93118131744411));
#87466=CARTESIAN_POINT('Ctrl Pts',(11.9301256565082,-0.0507270916490356,
3.93267285216719));
#87467=CARTESIAN_POINT('Ctrl Pts',(11.9242528079339,0.0650760333018407,
3.93416658326394));
#87468=CARTESIAN_POINT('Ctrl Pts',(11.9183799593596,0.180795186052275,3.93053911919053));
#87469=CARTESIAN_POINT('Ctrl Pts',(11.9125071107853,0.295947945456476,3.9218495398957));
#87470=CARTESIAN_POINT('Ctrl Pts',(11.9109123661726,0.327217139678331,3.91948992520577));
#87471=CARTESIAN_POINT('Ctrl Pts',(11.9093176215598,0.358444625222629,3.91675733775559));
#87472=CARTESIAN_POINT('Ctrl Pts',(11.907722876947,0.38962088346284,3.91365360848014));
#87473=CARTESIAN_POINT('Ctrl Pts',(11.9018504308131,0.504423526912368,3.90222451642464));
#87474=CARTESIAN_POINT('Ctrl Pts',(11.8959779846792,0.618915059751209,3.88572059659295));
#87475=CARTESIAN_POINT('Ctrl Pts',(11.8901055385453,0.732610956210603,3.86416487573191));
#87476=CARTESIAN_POINT('Ctrl Pts',(11.8842406996004,0.84615957057305,3.84263707823369));
#87477=CARTESIAN_POINT('Ctrl Pts',(11.8783758606556,0.958914195814496,3.8160705699254));
#87478=CARTESIAN_POINT('Ctrl Pts',(11.8725110217107,1.07039453271425,3.78454020249956));
#87479=CARTESIAN_POINT('Ctrl Pts',(11.8666522115907,1.18176027219244,3.75304224705694));
#87480=CARTESIAN_POINT('Ctrl Pts',(11.8607934014707,1.29185393346273,3.71659069377557));
#87481=CARTESIAN_POINT('Ctrl Pts',(11.8549345913506,1.4002051965583,3.67531147081865));
#87482=CARTESIAN_POINT('Ctrl Pts',(11.8488488024697,1.51275414398552,3.63243303117999));
#87483=CARTESIAN_POINT('Ctrl Pts',(11.8427630135887,1.62342251030598,3.58434537934897));
#87484=CARTESIAN_POINT('Ctrl Pts',(11.8366772247077,1.73169990225679,3.53124686881615));
#87485=CARTESIAN_POINT('Ctrl Pts',(11.8308251946295,1.83581829461074,3.48018790393473));
#87486=CARTESIAN_POINT('Ctrl Pts',(11.8249731645512,1.93772559649863,3.42449611863627));
#87487=CARTESIAN_POINT('Ctrl Pts',(11.8191211344729,2.03698894247253,3.36439668413887));
#87488=CARTESIAN_POINT('Ctrl Pts',(11.8132699940944,2.13623719717497,3.30430638671893));
#87489=CARTESIAN_POINT('Ctrl Pts',(11.8074188537159,2.23284194170572,3.23980998651906));
#87490=CARTESIAN_POINT('Ctrl Pts',(11.8015677133374,2.32639666045386,3.17117763271456));
#87491=CARTESIAN_POINT('Ctrl Pts',(11.7957160457699,2.41995980850207,3.10253909512038));
#87492=CARTESIAN_POINT('Ctrl Pts',(11.7898643782024,2.51047205116509,3.02976410764543));
#87493=CARTESIAN_POINT('Ctrl Pts',(11.7840127106349,2.59755809036092,2.95316456825565));
#87494=CARTESIAN_POINT('Ctrl Pts',(11.7781590989506,2.68467306240772,2.87653957997556));
#87495=CARTESIAN_POINT('Ctrl Pts',(11.7723054872664,2.76835925733957,2.79608778604424));
#87496=CARTESIAN_POINT('Ctrl Pts',(11.7664518755822,2.84827705830305,2.71215906597392));
#87497=CARTESIAN_POINT('Ctrl Pts',(11.7605916094823,2.92828571023082,2.62813493530599));
#87498=CARTESIAN_POINT('Ctrl Pts',(11.7547313433824,3.00451713239478,2.54062628879651));
#87499=CARTESIAN_POINT('Ctrl Pts',(11.7488710772825,3.07667089473987,2.45001738880779));
#87500=CARTESIAN_POINT('Ctrl Pts',(11.7430068641112,3.14887325488722,2.35934746090782));
#87501=CARTESIAN_POINT('Ctrl Pts',(11.7371426509399,3.2169922441767,2.2655734552825));
#87502=CARTESIAN_POINT('Ctrl Pts',(11.7312784377686,3.28077080176058,2.16910856028813));
#87503=CARTESIAN_POINT('Ctrl Pts',(11.7254055891943,3.34464327706713,2.07250161499349));
#87504=CARTESIAN_POINT('Ctrl Pts',(11.71953274062,3.40416235271693,1.97319622519693));
#87505=CARTESIAN_POINT('Ctrl Pts',(11.7136598920457,3.45911687723639,1.87163015299989));
#87506=CARTESIAN_POINT('Ctrl Pts',(11.7120651474329,3.47403952181282,1.844050360259));
#87507=CARTESIAN_POINT('Ctrl Pts',(11.7104704028201,3.48862586606958,1.81630398303906));
#87508=CARTESIAN_POINT('Ctrl Pts',(11.7088756582074,3.50287230338666,1.78840001849884));
#87509=CARTESIAN_POINT('Ctrl Pts',(11.7030032120734,3.55533301406993,1.68564718436352));
#87510=CARTESIAN_POINT('Ctrl Pts',(11.6971307659395,3.60335651369744,1.58041204790642));
#87511=CARTESIAN_POINT('Ctrl Pts',(11.6912583198056,3.64670018452956,1.47311464732112));
#87512=CARTESIAN_POINT('Ctrl Pts',(11.6853934808608,3.68998770780535,1.36595624019734));
#87513=CARTESIAN_POINT('Ctrl Pts',(11.6795286419159,3.72860730458444,1.25674126127248));
#87514=CARTESIAN_POINT('Ctrl Pts',(11.6736638029711,3.76236223807134,1.14591421560903));
#87515=CARTESIAN_POINT('Ctrl Pts',(11.6678049928511,3.7960824728083,1.03520109580903));
#87516=CARTESIAN_POINT('Ctrl Pts',(11.6619461827311,3.82494787117419,0.922879598464706));
#87517=CARTESIAN_POINT('Ctrl Pts',(11.656087372611,3.84881005824067,0.809413451571847));
#87518=CARTESIAN_POINT('Ctrl Pts',(11.6500015837301,3.87359670087795,0.691551462365815));
#87519=CARTESIAN_POINT('Ctrl Pts',(11.6439157948491,3.89298445832331,0.572454760379923));
#87520=CARTESIAN_POINT('Ctrl Pts',(11.6378300059681,3.9068642124379,0.452659944740006));
#87521=CARTESIAN_POINT('Ctrl Pts',(11.6319779758899,3.92021083686836,0.337466519851978));
#87522=CARTESIAN_POINT('Ctrl Pts',(11.6261259458116,3.92846473221161,0.221628070538059));
#87523=CARTESIAN_POINT('Ctrl Pts',(11.6202739157333,3.93158125972364,0.105630479454896));
#87524=CARTESIAN_POINT('Ctrl Pts',(11.6144227753548,3.93469731342168,-0.0103494762050065));
#87525=CARTESIAN_POINT('Ctrl Pts',(11.6085716349763,3.93267754116737,-0.126488112431964));
#87526=CARTESIAN_POINT('Ctrl Pts',(11.6027204945978,3.92552938770189,-0.242297392245137));
#87527=CARTESIAN_POINT('Ctrl Pts',(11.5968688270303,3.91838059018629,-0.358117106498744));
#87528=CARTESIAN_POINT('Ctrl Pts',(11.5910171594628,3.90610251837752,-0.473606992750635));
#87529=CARTESIAN_POINT('Ctrl Pts',(11.5851654918953,3.88875461610913,-0.588282700485007));
#87530=CARTESIAN_POINT('Ctrl Pts',(11.5793118802111,3.87140095029613,-0.702996507267154));
#87531=CARTESIAN_POINT('Ctrl Pts',(11.5734582685269,3.84897416656266,-0.81689518917469));
#87532=CARTESIAN_POINT('Ctrl Pts',(11.5676046568427,3.82158495236323,-0.929503874048374));
#87533=CARTESIAN_POINT('Ctrl Pts',(11.5617443907428,3.79416460196518,-1.0422405730503));
#87534=CARTESIAN_POINT('Ctrl Pts',(11.5558841246429,3.76177065897067,-1.15368394609837));
#87535=CARTESIAN_POINT('Ctrl Pts',(11.550023858543,3.72456392269728,-1.26337349415834));
#87536=CARTESIAN_POINT('Ctrl Pts',(11.5441596453717,3.68733212653026,-1.37313692153916));
#87537=CARTESIAN_POINT('Ctrl Pts',(11.5382954322004,3.6452812320772,-1.48114378756401));
#87538=CARTESIAN_POINT('Ctrl Pts',(11.5324312190291,3.59861982163417,-1.58695443518132));
#87539=CARTESIAN_POINT('Ctrl Pts',(11.5265583704548,3.55188969948653,-1.69292089527609));
#87540=CARTESIAN_POINT('Ctrl Pts',(11.5206855218805,3.50053569399984,-1.79668431334494));
#87541=CARTESIAN_POINT('Ctrl Pts',(11.5148126733062,3.44481188279228,-1.89783036443543));
#87542=CARTESIAN_POINT('Ctrl Pts',(11.5132179286934,3.42968034200677,-1.92529610240638));
#87543=CARTESIAN_POINT('Ctrl Pts',(11.5116231840806,3.41422682784621,-1.9525690154841));
#87544=CARTESIAN_POINT('Ctrl Pts',(11.5100284394677,3.3984569586644,-1.97964120489182));
#87545=CARTESIAN_POINT('Ctrl Pts',(11.5041559933338,3.34038640205949,-2.07933113188455));
#87546=CARTESIAN_POINT('Ctrl Pts',(11.4982835471999,3.27782846516256,-2.17663064366548));
#87547=CARTESIAN_POINT('Ctrl Pts',(11.492411101066,3.21100530195031,-2.27110852907716));
#87548=CARTESIAN_POINT('Ctrl Pts',(11.4865462621211,3.14426870171793,-2.3654640274766));
#87549=CARTESIAN_POINT('Ctrl Pts',(11.4806814231763,3.07327809930128,-2.45700483392695));
#87550=CARTESIAN_POINT('Ctrl Pts',(11.4748165842314,2.99830103872154,-2.54532510324346));
#87551=CARTESIAN_POINT('Ctrl Pts',(11.4689577741114,2.9234010516246,-2.633554582781));
#87552=CARTESIAN_POINT('Ctrl Pts',(11.4630989639914,2.84452302326456,-2.71856979689325));
#87553=CARTESIAN_POINT('Ctrl Pts',(11.4572401538713,2.76197681792224,-2.79999518879232));
#87554=CARTESIAN_POINT('Ctrl Pts',(11.4511543649904,2.67623265343389,-2.8845751179068));
#87555=CARTESIAN_POINT('Ctrl Pts',(11.4450685761094,2.58653060504518,-2.96528107851399));
#87556=CARTESIAN_POINT('Ctrl Pts',(11.4389827872284,2.4932630634291,-3.04173113482111));
#87557=CARTESIAN_POINT('Ctrl Pts',(11.4331307571501,2.40357798405176,-3.11524469859156));
#87558=CARTESIAN_POINT('Ctrl Pts',(11.4272787270719,2.31059661361456,-3.18482298456818));
#87559=CARTESIAN_POINT('Ctrl Pts',(11.4214266969936,2.21470354431358,-3.25016572051409));
#87560=CARTESIAN_POINT('Ctrl Pts',(11.4155755566151,2.11882505389179,-3.3154985222295));
#87561=CARTESIAN_POINT('Ctrl Pts',(11.4097244162366,2.0200360862833,-3.37659682157969));
#87562=CARTESIAN_POINT('Ctrl Pts',(11.403873275858,1.91875120799459,-3.43320299455469));
#87563=CARTESIAN_POINT('Ctrl Pts',(11.3980216082905,1.81745720391705,-3.48981426775777));
#87564=CARTESIAN_POINT('Ctrl Pts',(11.392169940723,1.71366720296469,-3.54193240832468));
#87565=CARTESIAN_POINT('Ctrl Pts',(11.3863182731555,1.60782078699842,-3.58934552765484));
#87566=CARTESIAN_POINT('Ctrl Pts',(11.3804646614713,1.50193920536598,-3.63677439918511));
#87567=CARTESIAN_POINT('Ctrl Pts',(11.3746110497871,1.39400022723991,-3.67949497233228));
#87568=CARTESIAN_POINT('Ctrl Pts',(11.3687574381028,1.28446316915365,-3.71734359013096));
#87569=CARTESIAN_POINT('Ctrl Pts',(11.362897172003,1.17480158878038,-3.75523523443164));
#87570=CARTESIAN_POINT('Ctrl Pts',(11.3570369059031,1.06353869328584,-3.78824373371904));
#87571=CARTESIAN_POINT('Ctrl Pts',(11.3511766398032,0.951148804400062,-3.81625535726952));
#87572=CARTESIAN_POINT('Ctrl Pts',(11.3453124266319,0.838683217429767,-3.84428584751939));
#87573=CARTESIAN_POINT('Ctrl Pts',(11.3394482134606,0.72508952974335,-3.86731267862198));
#87574=CARTESIAN_POINT('Ctrl Pts',(11.3335840002893,0.610850367354952,-3.88527358479455));
#87575=CARTESIAN_POINT('Ctrl Pts',(11.327711151715,0.496442980999267,-3.90326093947068));
#87576=CARTESIAN_POINT('Ctrl Pts',(11.3218383031407,0.381388632167704,-3.91616743488324));
#87577=CARTESIAN_POINT('Ctrl Pts',(11.3159654545664,0.266173237073291,-3.92398277364541));
#87578=CARTESIAN_POINT('Ctrl Pts',(11.3143707099536,0.234887034422116,-3.92610499240012));
#87579=CARTESIAN_POINT('Ctrl Pts',(11.3127759653408,0.203588943489356,-3.92785210188751));
#87580=CARTESIAN_POINT('Ctrl Pts',(11.3111812207281,0.172288646697863,-3.9292245573674));
#87581=CARTESIAN_POINT('Ctrl Pts',(11.3053087745941,0.0570292469096958,
-3.93427845177297));
#87582=CARTESIAN_POINT('Ctrl Pts',(11.2994363284602,-0.0586456867649011,
-3.93426499989482));
#87583=CARTESIAN_POINT('Ctrl Pts',(11.2935638823263,-0.174253294726548,
-3.92913791935037));
#87584=CARTESIAN_POINT('Ctrl Pts',(11.2876990433815,-0.289711144153209,
-3.92401748044555));
#87585=CARTESIAN_POINT('Ctrl Pts',(11.2818342044366,-0.405101432160393,
-3.91379660422549));
#87586=CARTESIAN_POINT('Ctrl Pts',(11.2759693654918,-0.519938094369209,
-3.89848090645879));
#87587=CARTESIAN_POINT('Ctrl Pts',(11.2701105553717,-0.634656708984688,
-3.88318095262984));
#87588=CARTESIAN_POINT('Ctrl Pts',(11.2642517452517,-0.748822422514947,
-3.86279664880266));
#87589=CARTESIAN_POINT('Ctrl Pts',(11.2583929351317,-0.861951766452858,
-3.83738558817182));
#87590=CARTESIAN_POINT('Ctrl Pts',(11.2523071462508,-0.979463904471754,
-3.81099006637249));
#87591=CARTESIAN_POINT('Ctrl Pts',(11.2462213573698,-1.09585729399974,-3.77917044291681));
#87592=CARTESIAN_POINT('Ctrl Pts',(11.2401355684888,-1.21059847758865,-3.74205028374286));
#87593=CARTESIAN_POINT('Ctrl Pts',(11.2342835384106,-1.32093238346523,-3.70635593215681));
#87594=CARTESIAN_POINT('Ctrl Pts',(11.2284315083323,-1.4297382369095,-3.6657608661504));
#87595=CARTESIAN_POINT('Ctrl Pts',(11.222579478254,-1.53655549330081,-3.62042624783424));
#87596=CARTESIAN_POINT('Ctrl Pts',(11.2167283378755,-1.64335650997958,-3.57509852186108));
#87597=CARTESIAN_POINT('Ctrl Pts',(11.210877197497,-1.74816915033764,-3.52503283774727));
#87598=CARTESIAN_POINT('Ctrl Pts',(11.2050260571185,-1.8505525384064,-3.47043863259353));
#87599=CARTESIAN_POINT('Ctrl Pts',(11.199174389551,-1.95294515123991,-3.41583950849044));
#87600=CARTESIAN_POINT('Ctrl Pts',(11.1933227219835,-2.05290771191474,-3.35671124674412));
#87601=CARTESIAN_POINT('Ctrl Pts',(11.187471054416,-2.15002429143809,-3.29330905719857));
#87602=CARTESIAN_POINT('Ctrl Pts',(11.1816174427318,-2.24717313628831,-3.2298858033571));
#87603=CARTESIAN_POINT('Ctrl Pts',(11.1757638310476,-2.34147377391848,-3.16218602410032));
#87604=CARTESIAN_POINT('Ctrl Pts',(11.1699102193634,-2.43254017747779,-3.09050760959366));
#87605=CARTESIAN_POINT('Ctrl Pts',(11.1640499532635,-2.52371010579004,-3.0187477106991));
#87606=CARTESIAN_POINT('Ctrl Pts',(11.1581896871636,-2.61163813647035,-2.94300040474197));
#87607=CARTESIAN_POINT('Ctrl Pts',(11.1523294210637,-2.69597212760409,-2.86360320002298));
#87608=CARTESIAN_POINT('Ctrl Pts',(11.1464652078924,-2.78036292030289,-2.78415251881808));
#87609=CARTESIAN_POINT('Ctrl Pts',(11.1406009947211,-2.86115456593174,-2.70104733950031));
#87610=CARTESIAN_POINT('Ctrl Pts',(11.1347367815498,-2.93803372513164,-2.61465998362867));
#87611=CARTESIAN_POINT('Ctrl Pts',(11.1288639329755,-3.01502609346969,-2.5281454172333));
#87612=CARTESIAN_POINT('Ctrl Pts',(11.1229910844012,-3.08809421693889,-2.43833934760837));
#87613=CARTESIAN_POINT('Ctrl Pts',(11.117118235827,-3.15696669341386,-2.34564496390131));
#87614=CARTESIAN_POINT('Ctrl Pts',(11.1155234912141,-3.17566869286801,-2.32047423675136));
#87615=CARTESIAN_POINT('Ctrl Pts',(11.1139287466013,-3.19406157517828,-2.2950906836513));
#87616=CARTESIAN_POINT('Ctrl Pts',(11.1123340019885,-3.21214048792809,-2.26950269570518));
#87617=CARTESIAN_POINT('Ctrl Pts',(11.1063993270745,-3.27941926667771,-2.1742796807209));
#87618=CARTESIAN_POINT('Ctrl Pts',(11.1004646521605,-3.34256962426546,-2.07590768305915));
#87619=CARTESIAN_POINT('Ctrl Pts',(11.0945299772465,-3.40128662071416,-1.97477551224204));
#87620=CARTESIAN_POINT('Ctrl Pts',(11.0886033536864,-3.45992395798658,-1.87378054369873));
#87621=CARTESIAN_POINT('Ctrl Pts',(11.0826767301263,-3.5141396972636,-1.77003319406172));
#87622=CARTESIAN_POINT('Ctrl Pts',(11.0767501065661,-3.56367074985205,-1.66395306023004));
#87623=CARTESIAN_POINT('Ctrl Pts',(11.0708301927134,-3.61314572685761,-1.55799302288384));
#87624=CARTESIAN_POINT('Ctrl Pts',(11.0649102788607,-3.6579463995249,-1.44970581711695));
#87625=CARTESIAN_POINT('Ctrl Pts',(11.0589903650079,-3.69785469604635,-1.33953710173625));
#87626=CARTESIAN_POINT('Ctrl Pts',(11.0530765800023,-3.73772167577604,-1.22948244328781));
#87627=CARTESIAN_POINT('Ctrl Pts',(11.0471627949967,-3.7727062283439,-1.11755053000092));
#87628=CARTESIAN_POINT('Ctrl Pts',(11.0412490099911,-3.80263797799915,-1.00420785113367));
#87629=CARTESIAN_POINT('Ctrl Pts',(11.0353388793976,-3.83255123138704,-0.890935212157697));
#87630=CARTESIAN_POINT('Ctrl Pts',(11.0294287488041,-3.85741779186855,-0.776253929583021));
#87631=CARTESIAN_POINT('Ctrl Pts',(11.0235186182106,-3.8771169050801,-0.660646277778147));
#87632=CARTESIAN_POINT('Ctrl Pts',(11.0176101824024,-3.89681036938656,-0.545071777549431));
#87633=CARTESIAN_POINT('Ctrl Pts',(11.0117017465942,-3.91133926234982,-0.42857183151326));
#87634=CARTESIAN_POINT('Ctrl Pts',(11.0057933107859,-3.92063388177004,-0.31163915850992));
#87635=CARTESIAN_POINT('Ctrl Pts',(11.0005167145356,-3.92893454806693,-0.207211096001756));
#87636=CARTESIAN_POINT('Ctrl Pts',(10.9952401182853,-3.9330612436711,-0.102438247546336));
#87637=CARTESIAN_POINT('Ctrl Pts',(10.989963522035,-3.93299931278836,0.00232499597257397));
#87638=CARTESIAN_POINT('',(9.73996412712546,-3.93468200878748,0.00220793234553757));
#87639=CARTESIAN_POINT('Ctrl Pts',(10.9899620430679,-3.92789199627619,0.00235130254412344));
#87640=CARTESIAN_POINT('Ctrl Pts',(10.9644702897948,-3.93059709637408,0.50781727451283));
#87641=CARTESIAN_POINT('Ctrl Pts',(10.8726961302754,-3.60487430294788,2.32421058671237));
#87642=CARTESIAN_POINT('Ctrl Pts',(10.714639564509,-0.864193458227065,4.57068481609948));
#87643=CARTESIAN_POINT('Ctrl Pts',(10.5157923457696,3.37762255948928,3.19838332083506));
#87644=CARTESIAN_POINT('Ctrl Pts',(10.3169451270298,4.51682366238826,-1.11188759515321));
#87645=CARTESIAN_POINT('Ctrl Pts',(10.1180979082903,1.50696304637114,-4.40080133592016));
#87646=CARTESIAN_POINT('Ctrl Pts',(9.92577130003029,-2.74307050786764,-3.67194027927687));
#87647=CARTESIAN_POINT('Ctrl Pts',(9.79972709801699,-3.92999336875819,-1.17507727859808));
#87648=CARTESIAN_POINT('Ctrl Pts',(9.73996530225019,-3.93794979387841,0.00218662693770836));
#87649=CARTESIAN_POINT('',(8.489963468396,-3.93310746533601,-0.00342879478566001));
#87650=CARTESIAN_POINT('Ctrl Pts',(9.73996352203497,-3.93299937407447,0.00221890284016636));
#87651=CARTESIAN_POINT('Ctrl Pts',(9.7334435049603,-3.93292700297544,0.130496483113836));
#87652=CARTESIAN_POINT('Ctrl Pts',(9.72692348788562,-3.92657937860584,0.25859433429193));
#87653=CARTESIAN_POINT('Ctrl Pts',(9.72040347081094,-3.91400567965978,0.386068050466482));
#87654=CARTESIAN_POINT('Ctrl Pts',(9.714531024677,-3.90268080597933,0.50088102152982));
#87655=CARTESIAN_POINT('Ctrl Pts',(9.70865857854307,-3.88628082419871,0.615387488854809));
#87656=CARTESIAN_POINT('Ctrl Pts',(9.70278613240914,-3.86482832122034,0.729102905969475));
#87657=CARTESIAN_POINT('Ctrl Pts',(9.69692129346427,-3.84340360789598,0.842671015700072));
#87658=CARTESIAN_POINT('Ctrl Pts',(9.69105645451941,-3.81693946508308,0.955449710595288));
#87659=CARTESIAN_POINT('Ctrl Pts',(9.68519161557455,-3.7855103084452,1.06695862368468));
#87660=CARTESIAN_POINT('Ctrl Pts',(9.67933280545452,-3.75411345974988,1.17835290997703));
#87661=CARTESIAN_POINT('Ctrl Pts',(9.67347399533448,-3.71776186051044,1.28847961528162));
#87662=CARTESIAN_POINT('Ctrl Pts',(9.66761518521445,-3.67658101189881,1.39686830551242));
#87663=CARTESIAN_POINT('Ctrl Pts',(9.66152939633348,-3.63380475776958,1.5094561300561));
#87664=CARTESIAN_POINT('Ctrl Pts',(9.65544360745251,-3.58581758647112,1.62016810300132));
#87665=CARTESIAN_POINT('Ctrl Pts',(9.64935781857155,-3.53281738809582,1.72849365123735));
#87666=CARTESIAN_POINT('Ctrl Pts',(9.64350578849328,-3.48185295914286,1.83265835016494));
#87667=CARTESIAN_POINT('Ctrl Pts',(9.63765375841501,-3.42625370453409,1.93461616504343));
#87668=CARTESIAN_POINT('Ctrl Pts',(9.63180172833674,-3.36624440245535,2.03393402620096));
#87669=CARTESIAN_POINT('Ctrl Pts',(9.62595058795822,-3.30624422375095,2.13323678779901));
#87670=CARTESIAN_POINT('Ctrl Pts',(9.6200994475797,-3.24183554439956,2.22990004001445));
#87671=CARTESIAN_POINT('Ctrl Pts',(9.61424830720118,-3.17328814444511,2.32351702217224));
#87672=CARTESIAN_POINT('Ctrl Pts',(9.60839663963368,-3.10473456835549,2.41714243923982));
#87673=CARTESIAN_POINT('Ctrl Pts',(9.60254497206618,-3.03204177458839,2.50772070709806));
#87674=CARTESIAN_POINT('Ctrl Pts',(9.59669330449868,-2.95552132029931,2.59487624468995));
#87675=CARTESIAN_POINT('Ctrl Pts',(9.59083969281444,-2.87897544339443,2.68206073822267));
#87676=CARTESIAN_POINT('Ctrl Pts',(9.5849860811302,-2.79859964989581,2.76581992988817));
#87677=CARTESIAN_POINT('Ctrl Pts',(9.57913246944596,-2.71474351087968,2.84581388536508));
#87678=CARTESIAN_POINT('Ctrl Pts',(9.57327220334606,-2.63079204377651,2.92589877837906));
#87679=CARTESIAN_POINT('Ctrl Pts',(9.56741193724617,-2.54335263343562,3.00220960630231));
#87680=CARTESIAN_POINT('Ctrl Pts',(9.56155167114628,-2.45280926934149,3.07444559038414));
#87681=CARTESIAN_POINT('Ctrl Pts',(9.55568745797496,-2.36220492147658,3.14673022764712));
#87682=CARTESIAN_POINT('Ctrl Pts',(9.54982324480365,-2.26849279042965,3.21493431350354));
#87683=CARTESIAN_POINT('Ctrl Pts',(9.54395903163234,-2.17208583103624,3.27880041213423));
#87684=CARTESIAN_POINT('Ctrl Pts',(9.53808618305805,-2.07553690665617,3.34276055739701));
#87685=CARTESIAN_POINT('Ctrl Pts',(9.53221333448375,-1.97628558702804,3.40236975434652));
#87686=CARTESIAN_POINT('Ctrl Pts',(9.52634048590945,-1.87476944239729,3.45741645421163));
#87687=CARTESIAN_POINT('Ctrl Pts',(9.52474574129675,-1.84720320725529,3.47236412857212));
#87688=CARTESIAN_POINT('Ctrl Pts',(9.52315099668404,-1.81947008242169,3.48697565397087));
#87689=CARTESIAN_POINT('Ctrl Pts',(9.52155625207134,-1.79157906177759,3.50124741562206));
#87690=CARTESIAN_POINT('Ctrl Pts',(9.51568380593743,-1.68887389190436,3.55380137997778));
#87691=CARTESIAN_POINT('Ctrl Pts',(9.50981135980352,-1.58368239279322,3.60192038844979));
#87692=CARTESIAN_POINT('Ctrl Pts',(9.50393891366961,-1.47642438222513,3.64536144210298));
#87693=CARTESIAN_POINT('Ctrl Pts',(9.49807407472477,-1.36930531409211,3.68874622204996));
#87694=CARTESIAN_POINT('Ctrl Pts',(9.49220923577993,-1.26012543763137,3.72746494430459));
#87695=CARTESIAN_POINT('Ctrl Pts',(9.48634439683508,-1.14932907913176,3.7613204686469));
#87696=CARTESIAN_POINT('Ctrl Pts',(9.48048558671507,-1.03864661495097,3.79514119083564));
#87697=CARTESIAN_POINT('Ctrl Pts',(9.47462677659505,-0.926351366844571,
3.82410853868028));
#87698=CARTESIAN_POINT('Ctrl Pts',(9.46876796647504,-0.812906927927939,
3.84807371635819));
#87699=CARTESIAN_POINT('Ctrl Pts',(9.46268217759406,-0.695067487696164,
3.87296733961191));
#87700=CARTESIAN_POINT('Ctrl Pts',(9.45659638871309,-0.575988434281552,
3.89246320072552));
#87701=CARTESIAN_POINT('Ctrl Pts',(9.45051059983211,-0.456206267535364,
3.90645169449994));
#87702=CARTESIAN_POINT('Ctrl Pts',(9.44465856975385,-0.341025005689439,
3.91990288183466));
#87703=CARTESIAN_POINT('Ctrl Pts',(9.43880653967558,-0.225194096689067,
3.92826192771017));
#87704=CARTESIAN_POINT('Ctrl Pts',(9.43295450959732,-0.109199382469267,
3.93148375233427));
#87705=CARTESIAN_POINT('Ctrl Pts',(9.4271033692188,0.00677769676451066,
3.93470508713577));
#87706=CARTESIAN_POINT('Ctrl Pts',(9.42125222884029,0.122918118616052,3.93279074214541));
#87707=CARTESIAN_POINT('Ctrl Pts',(9.41540108846178,0.238733839547532,3.92574771907912));
#87708=CARTESIAN_POINT('Ctrl Pts',(9.40954942089428,0.354559995499951,3.91870406143495));
#87709=CARTESIAN_POINT('Ctrl Pts',(9.40369775332678,0.470060979755278,3.90653083220509));
#87710=CARTESIAN_POINT('Ctrl Pts',(9.39784608575928,0.58475238803632,3.88928703552281));
#87711=CARTESIAN_POINT('Ctrl Pts',(9.39199247407505,0.699481900581413,3.87203750988322));
#87712=CARTESIAN_POINT('Ctrl Pts',(9.38613886239082,0.813400893779758,3.84971412847263));
#87713=CARTESIAN_POINT('Ctrl Pts',(9.38028525070659,0.926034395189715,3.82242714762827));
#87714=CARTESIAN_POINT('Ctrl Pts',(9.3744249846067,1.03879593893931,3.79510914680474));
#87715=CARTESIAN_POINT('Ctrl Pts',(9.36856471850681,1.15026867211446,3.76281638139967));
#87716=CARTESIAN_POINT('Ctrl Pts',(9.36270445240692,1.2599919499029,3.72570923264013));
#87717=CARTESIAN_POINT('Ctrl Pts',(9.35684023923562,1.36978912973027,3.68857709106222));
#87718=CARTESIAN_POINT('Ctrl Pts',(9.35097602606431,1.47783412352762,3.64662425864128));
#87719=CARTESIAN_POINT('Ctrl Pts',(9.345111812893,1.58368708508111,3.60005891848276));
#87720=CARTESIAN_POINT('Ctrl Pts',(9.33923896431871,1.6896959214218,3.55342500808888));
#87721=CARTESIAN_POINT('Ctrl Pts',(9.33336611574442,1.79350591403744,3.50216521641961));
#87722=CARTESIAN_POINT('Ctrl Pts',(9.32749326717013,1.89470250750391,3.44653324487932));
#87723=CARTESIAN_POINT('Ctrl Pts',(9.3258985225573,1.92218197002126,3.43142664272661));
#87724=CARTESIAN_POINT('Ctrl Pts',(9.32430377794448,1.94946890000054,3.41599789229209));
#87725=CARTESIAN_POINT('Ctrl Pts',(9.32270903333165,1.97655539356812,3.400252604757));
#87726=CARTESIAN_POINT('Ctrl Pts',(9.31683658719773,2.07629799382696,3.34227256696972));
#87727=CARTESIAN_POINT('Ctrl Pts',(9.31096414106382,2.17365425333958,3.27980298080728));
#87728=CARTESIAN_POINT('Ctrl Pts',(9.3050916949299,2.2681927594629,3.21306560871702));
#87729=CARTESIAN_POINT('Ctrl Pts',(9.29922685598505,2.3626088000456,3.14641468847256));
#87730=CARTESIAN_POINT('Ctrl Pts',(9.29336201704021,2.45421401146745,3.07550721272152));
#87731=CARTESIAN_POINT('Ctrl Pts',(9.28749717809536,2.54260230584417,3.00061035696338));
#87732=CARTESIAN_POINT('Ctrl Pts',(9.28163836797534,2.63089974051472,2.9257904922407));
#87733=CARTESIAN_POINT('Ctrl Pts',(9.27577955785533,2.71598652220557,2.84698967010068));
#87734=CARTESIAN_POINT('Ctrl Pts',(9.26992074773531,2.79748681300003,2.76451741377965));
#87735=CARTESIAN_POINT('Ctrl Pts',(9.26383495885434,2.88214454270148,2.67885006320415));
#87736=CARTESIAN_POINT('Ctrl Pts',(9.25774916997336,2.96293189831491,2.58922131371123));
#87737=CARTESIAN_POINT('Ctrl Pts',(9.25166338109239,3.03946658800689,2.49602320910479));
#87738=CARTESIAN_POINT('Ctrl Pts',(9.24581135101413,3.11306153434305,2.40640489961994));
#87739=CARTESIAN_POINT('Ctrl Pts',(9.23995932093587,3.18272419675997,2.31348672813126));
#87740=CARTESIAN_POINT('Ctrl Pts',(9.2341072908576,3.24815395402568,2.21765301410012));
#87741=CARTESIAN_POINT('Ctrl Pts',(9.22825615047909,3.31357376383076,2.12183386992431));
#87742=CARTESIAN_POINT('Ctrl Pts',(9.22240501010057,3.37476171504071,2.02310040583366));
#87743=CARTESIAN_POINT('Ctrl Pts',(9.21655386972206,3.43145980742328,1.92186695430214));
#87744=CARTESIAN_POINT('Ctrl Pts',(9.21070220215456,3.48816300831595,1.82062438161526));
#87745=CARTESIAN_POINT('Ctrl Pts',(9.20485053458707,3.54037534419892,1.71688173437947));
#87746=CARTESIAN_POINT('Ctrl Pts',(9.19899886701957,3.58788452752248,1.61107840192983));
#87747=CARTESIAN_POINT('Ctrl Pts',(9.19314525533533,3.63540949496186,1.50523991812761));
#87748=CARTESIAN_POINT('Ctrl Pts',(9.1872916436511,3.67822803358777,1.39733976465732));
#87749=CARTESIAN_POINT('Ctrl Pts',(9.18143803196686,3.71617606955139,1.28783710930133));
#87750=CARTESIAN_POINT('Ctrl Pts',(9.17557776586697,3.75416724503605,1.17820997076762));
#87751=CARTESIAN_POINT('Ctrl Pts',(9.16971749976709,3.78727673113501,1.06697708503089));
#87752=CARTESIAN_POINT('Ctrl Pts',(9.1638572336672,3.81539036659949,0.954612670385135));
#87753=CARTESIAN_POINT('Ctrl Pts',(9.1579930204959,3.84352293747151,0.842172574812675));
#87754=CARTESIAN_POINT('Ctrl Pts',(9.15212880732459,3.86665287530667,0.72859983684903));
#87755=CARTESIAN_POINT('Ctrl Pts',(9.14626459415329,3.88471747623753,0.614377025786864));
#87756=CARTESIAN_POINT('Ctrl Pts',(9.140391745579,3.90280867836863,0.499986014835841));
#87757=CARTESIAN_POINT('Ctrl Pts',(9.13451889700471,3.9158196106186,0.384943429456174));
#87758=CARTESIAN_POINT('Ctrl Pts',(9.12864604843042,3.92373953450778,0.269735176313091));
#87759=CARTESIAN_POINT('Ctrl Pts',(9.12705130381763,3.92589015286551,0.238450913024903));
#87760=CARTESIAN_POINT('Ctrl Pts',(9.12545655920482,3.92766567290221,0.207154420949471));
#87761=CARTESIAN_POINT('Ctrl Pts',(9.12386181459203,3.92906654108815,0.175855382918928));
#87762=CARTESIAN_POINT('Ctrl Pts',(9.11798936845811,3.93422506170433,0.0606006183611476));
#87763=CARTESIAN_POINT('Ctrl Pts',(9.11211692232419,3.93431661533117,-0.0550742798645938));
#87764=CARTESIAN_POINT('Ctrl Pts',(9.10624447619028,3.92929448128277,-0.170686494371317));
#87765=CARTESIAN_POINT('Ctrl Pts',(9.10037963724543,3.92427885292593,-0.286148944375347));
#87766=CARTESIAN_POINT('Ctrl Pts',(9.09451479830059,3.91416272802553,-0.401548462979302));
#87767=CARTESIAN_POINT('Ctrl Pts',(9.08864995935575,3.8989512811163,-0.516398980906778));
#87768=CARTESIAN_POINT('Ctrl Pts',(9.08279114923572,3.88375547097896,-0.631131436998315));
#87769=CARTESIAN_POINT('Ctrl Pts',(9.0769323391157,3.86347481103469,-0.745315607620525));
#87770=CARTESIAN_POINT('Ctrl Pts',(9.07107352899568,3.83816645557921,-0.85846797218446));
#87771=CARTESIAN_POINT('Ctrl Pts',(9.06498774011471,3.81187761790205,-0.97600402268136));
#87772=CARTESIAN_POINT('Ctrl Pts',(9.05890195123374,3.78016366524417,-1.09242624895059));
#87773=CARTESIAN_POINT('Ctrl Pts',(9.05281616235277,3.74314767923944,-1.2072010815951));
#87774=CARTESIAN_POINT('Ctrl Pts',(9.0469641322745,3.70755349946864,-1.31756734404697));
#87775=CARTESIAN_POINT('Ctrl Pts',(9.04111210219623,3.66705722018621,-1.42641000338649));
#87776=CARTESIAN_POINT('Ctrl Pts',(9.03526007211797,3.62181958537068,-1.53326836888567));
#87777=CARTESIAN_POINT('Ctrl Pts',(9.02940893173945,3.57658882815353,-1.64011048842231));
#87778=CARTESIAN_POINT('Ctrl Pts',(9.02355779136093,3.52661830977212,-1.74496853340364));
#87779=CARTESIAN_POINT('Ctrl Pts',(9.01770665098242,3.47211706702969,-1.84740143792332));
#87780=CARTESIAN_POINT('Ctrl Pts',(9.01185498341492,3.41761091371376,-1.94984357166936));
#87781=CARTESIAN_POINT('Ctrl Pts',(9.00600331584742,3.35857341870767,-2.04985976564441));
#87782=CARTESIAN_POINT('Ctrl Pts',(9.00015164827992,3.29525941418505,-2.14703385935686));
#87783=CARTESIAN_POINT('Ctrl Pts',(8.99429803659569,3.23192437466436,-2.24424023750446));
#87784=CARTESIAN_POINT('Ctrl Pts',(8.98844442491144,3.16431022599136,-2.3386022916798));
#87785=CARTESIAN_POINT('Ctrl Pts',(8.9825908132272,3.09271450778762,-2.42973372477725));
#87786=CARTESIAN_POINT('Ctrl Pts',(8.97673054712731,3.02103739920585,-2.52096875655319));
#87787=CARTESIAN_POINT('Ctrl Pts',(8.97087028102742,2.9453699423276,-2.60896551165607));
#87788=CARTESIAN_POINT('Ctrl Pts',(8.96501001492753,2.86604932565287,-2.69337154193861));
#87789=CARTESIAN_POINT('Ctrl Pts',(8.95914580175622,2.78667528407667,-2.77783442230678));
#87790=CARTESIAN_POINT('Ctrl Pts',(8.95328158858492,2.70364347871848,-2.85870147450845));
#87791=CARTESIAN_POINT('Ctrl Pts',(8.94741737541361,2.61732594654579,-2.93565902133374));
#87792=CARTESIAN_POINT('Ctrl Pts',(8.94154452683932,2.53088130666863,-3.0127298927279));
#87793=CARTESIAN_POINT('Ctrl Pts',(8.93567167826502,2.44114160263122,-3.085879508777));
#87794=CARTESIAN_POINT('Ctrl Pts',(8.92979882969073,2.34850977704589,-3.15483610146706));
#87795=CARTESIAN_POINT('Ctrl Pts',(8.92820408507795,2.3233560372626,-3.17356094228616));
#87796=CARTESIAN_POINT('Ctrl Pts',(8.92660934046517,2.29798919101159,-3.19197685928441));
#87797=CARTESIAN_POINT('Ctrl Pts',(8.92501459585239,2.27241762498861,-3.21007899243011));
#87798=CARTESIAN_POINT('Ctrl Pts',(8.91914214971847,2.1782535545624,-3.27673781726956));
#87799=CARTESIAN_POINT('Ctrl Pts',(8.91326970358456,2.08099630301674,-3.33936143488604));
#87800=CARTESIAN_POINT('Ctrl Pts',(8.90739725745064,1.9810267582882,-3.39764947911731));
#87801=CARTESIAN_POINT('Ctrl Pts',(8.9015324185058,1.88118671448837,-3.45586201679425));
#87802=CARTESIAN_POINT('Ctrl Pts',(8.89566757956095,1.77864171843713,-3.50974994365985));
#87803=CARTESIAN_POINT('Ctrl Pts',(8.8898027406161,1.6738034538666,-3.55905478994413));
#87804=CARTESIAN_POINT('Ctrl Pts',(8.88394393049609,1.56907295892763,-3.60830895277672));
#87805=CARTESIAN_POINT('Ctrl Pts',(8.87808512037608,1.46205425625753,-3.65298923105742));
#87806=CARTESIAN_POINT('Ctrl Pts',(8.87222631025606,1.3531849915988,-3.69288225895597));
#87807=CARTESIAN_POINT('Ctrl Pts',(8.86614052137509,1.24009797447974,-3.73432080033894));
#87808=CARTESIAN_POINT('Ctrl Pts',(8.86005473249412,1.12501450101084,-3.77059343047534));
#87809=CARTESIAN_POINT('Ctrl Pts',(8.85396894361315,1.0084499660249,-3.80151518029645));
#87810=CARTESIAN_POINT('Ctrl Pts',(8.84811691353488,0.896362744772546,-3.83124920715228));
#87811=CARTESIAN_POINT('Ctrl Pts',(8.84226488345661,0.782906576640369,-3.85603571639762));
#87812=CARTESIAN_POINT('Ctrl Pts',(8.83641285337835,0.668555914690499,-3.87576082710638));
#87813=CARTESIAN_POINT('Ctrl Pts',(8.83056171299983,0.554222637776941,-3.89548293895392));
#87814=CARTESIAN_POINT('Ctrl Pts',(8.82471057262132,0.438995544672728,-3.91014511203182));
#87815=CARTESIAN_POINT('Ctrl Pts',(8.81885943224281,0.323358692289862,-3.91968470111061));
#87816=CARTESIAN_POINT('Ctrl Pts',(8.81300776467532,0.207711421002246,-3.92922514970839));
#87817=CARTESIAN_POINT('Ctrl Pts',(8.80715609710782,0.0916547290259299,
-3.93364206280956));
#87818=CARTESIAN_POINT('Ctrl Pts',(8.80130442954033,-0.0243235153582555,
-3.93292478527121));
#87819=CARTESIAN_POINT('Ctrl Pts',(8.7954508178561,-0.140340291535808,-3.93220726942963));
#87820=CARTESIAN_POINT('Ctrl Pts',(8.78959720617188,-0.25627815516653,-3.92635217372918));
#87821=CARTESIAN_POINT('Ctrl Pts',(8.78374359448765,-0.371651266961712,
-3.91540091635145));
#87822=CARTESIAN_POINT('Ctrl Pts',(8.77788332838776,-0.487155535499663,
-3.90443720952839));
#87823=CARTESIAN_POINT('Ctrl Pts',(8.77202306228787,-0.602093359015705,
-3.88836581679333));
#87824=CARTESIAN_POINT('Ctrl Pts',(8.76616279618798,-0.715985933712069,
-3.8672798117962));
#87825=CARTESIAN_POINT('Ctrl Pts',(8.76029858301667,-0.829955218598503,
-3.84617960471912));
#87826=CARTESIAN_POINT('Ctrl Pts',(8.75443436984537,-0.942877451107107,
-3.82005815303478));
#87827=CARTESIAN_POINT('Ctrl Pts',(8.74857015667407,-1.05428759897505,-3.78905880907745));
#87828=CARTESIAN_POINT('Ctrl Pts',(8.74269730809978,-1.1658618049178,-3.7580138167408));
#87829=CARTESIAN_POINT('Ctrl Pts',(8.73682445952549,-1.27591909083997,-3.7220767241443));
#87830=CARTESIAN_POINT('Ctrl Pts',(8.73095161095121,-1.38401296786932,-3.68143954245748));
#87831=CARTESIAN_POINT('Ctrl Pts',(8.72935686633839,-1.41336535553788,-3.67040470548605));
#87832=CARTESIAN_POINT('Ctrl Pts',(8.72776212172556,-1.44257310258369,-3.65902356318122));
#87833=CARTESIAN_POINT('Ctrl Pts',(8.72616737711274,-1.47162758593249,-3.64730054263732));
#87834=CARTESIAN_POINT('Ctrl Pts',(8.72029493097883,-1.57861706063779,-3.60413199632748));
#87835=CARTESIAN_POINT('Ctrl Pts',(8.71442248484491,-1.68388459775975,-3.55617956062416));
#87836=CARTESIAN_POINT('Ctrl Pts',(8.70855003871099,-1.78697157659788,-3.50360123079544));
#87837=CARTESIAN_POINT('Ctrl Pts',(8.70268519976615,-1.88992501617127,-3.45109101113529));
#87838=CARTESIAN_POINT('Ctrl Pts',(8.6968203608213,-1.99070314995889,-3.39396700018268));
#87839=CARTESIAN_POINT('Ctrl Pts',(8.69095552187646,-2.08886594927692,-3.33243575271173));
#87840=CARTESIAN_POINT('Ctrl Pts',(8.68509671175643,-2.18692784108041,-3.27096775695419));
#87841=CARTESIAN_POINT('Ctrl Pts',(8.67923790163641,-2.28237939777625,-3.20510175424569));
#87842=CARTESIAN_POINT('Ctrl Pts',(8.67337909151639,-2.37480449459196,-3.13509052699692));
#87843=CARTESIAN_POINT('Ctrl Pts',(8.66729330263542,-2.4708102730693,-3.06236696374684));
#87844=CARTESIAN_POINT('Ctrl Pts',(8.66120751375445,-2.56354994534687,-2.98517070251276));
#87845=CARTESIAN_POINT('Ctrl Pts',(8.65512172487348,-2.6525892345319,-2.90383528335294));
#87846=CARTESIAN_POINT('Ctrl Pts',(8.64926969479521,-2.73820847119117,-2.82562400644849));
#87847=CARTESIAN_POINT('Ctrl Pts',(8.64341766471695,-2.82040601552851,-2.74358598579513));
#87848=CARTESIAN_POINT('Ctrl Pts',(8.63756563463868,-2.89882952826502,-2.65805875895527));
#87849=CARTESIAN_POINT('Ctrl Pts',(8.63171449426016,-2.97724111806558,-2.57254453504796));
#87850=CARTESIAN_POINT('Ctrl Pts',(8.62586335388165,-3.05187953783439,-2.48354246429099));
#87851=CARTESIAN_POINT('Ctrl Pts',(8.62001221350314,-3.12243035531733,-2.39142586675667));
#87852=CARTESIAN_POINT('Ctrl Pts',(8.61416054593563,-3.19298752944389,-2.29930096949737));
#87853=CARTESIAN_POINT('Ctrl Pts',(8.60830887836813,-3.25945611779732,-2.20406131580116));
#87854=CARTESIAN_POINT('Ctrl Pts',(8.60245721080062,-3.3215633618016,-2.10611154346993));
#87855=CARTESIAN_POINT('Ctrl Pts',(8.59660359911638,-3.38369123987837,-2.00812922899749));
#87856=CARTESIAN_POINT('Ctrl Pts',(8.59074998743213,-3.44145467115868,-1.90743535442846));
#87857=CARTESIAN_POINT('Ctrl Pts',(8.58489637574788,-3.49462579870807,-1.80446100733819));
#87858=CARTESIAN_POINT('Ctrl Pts',(8.57903610964799,-3.54785737146671,-1.70136959848446));
#87859=CARTESIAN_POINT('Ctrl Pts',(8.5731758435481,-3.59648603068227,-1.59599291016126));
#87860=CARTESIAN_POINT('Ctrl Pts',(8.56731557744821,-3.64033117662272,-1.48878404226693));
#87861=CARTESIAN_POINT('Ctrl Pts',(8.56145136427691,-3.68420585363208,-1.38150296586699));
#87862=CARTESIAN_POINT('Ctrl Pts',(8.5555871511056,-3.7232904629761,-1.27238764088816));
#87863=CARTESIAN_POINT('Ctrl Pts',(8.5497229379343,-3.75745414621014,-1.16190676869024));
#87864=CARTESIAN_POINT('Ctrl Pts',(8.54385008936,-3.79166813750154,-1.051263206831));
#87865=CARTESIAN_POINT('Ctrl Pts',(8.5379772407857,-3.82094663625831,-0.939250482913397));
#87866=CARTESIAN_POINT('Ctrl Pts',(8.5321043922114,-3.84520974288296,-0.826348009762216));
#87867=CARTESIAN_POINT('Ctrl Pts',(8.53050964759863,-3.8517982762138,-0.795689870266806));
#87868=CARTESIAN_POINT('Ctrl Pts',(8.52891490298586,-3.85801728574547,-0.764966152912951));
#87869=CARTESIAN_POINT('Ctrl Pts',(8.52732015837309,-3.86386583300464,-0.734186505282812));
#87870=CARTESIAN_POINT('Ctrl Pts',(8.51861044952465,-3.89580771473652,-0.566083244629494));
#87871=CARTESIAN_POINT('Ctrl Pts',(8.50990074067621,-3.91678675781709,-0.395835647213497));
#87872=CARTESIAN_POINT('Ctrl Pts',(8.50119103182777,-3.92658132922545,-0.224606466910645));
#87873=CARTESIAN_POINT('Ctrl Pts',(8.4974485285635,-3.93078999062915,-0.151030440734303));
#87874=CARTESIAN_POINT('Ctrl Pts',(8.49370602529924,-3.9329341093572,-0.0772734915122383));
#87875=CARTESIAN_POINT('Ctrl Pts',(8.48996352203497,-3.93299850454534,-0.00342975860908187));
#87876=CARTESIAN_POINT('',(7.23996352203496,-3.92656899063656,-0.000561720325250592));
#87877=CARTESIAN_POINT('Ctrl Pts',(8.48996263443681,-3.93480154809321,-0.00341380960952649));
#87878=CARTESIAN_POINT('Ctrl Pts',(8.43613273616902,-3.9250547143977,1.05920602663723));
#87879=CARTESIAN_POINT('Ctrl Pts',(8.31602043165469,-2.93158872492316,3.44630354530614));
#87880=CARTESIAN_POINT('Ctrl Pts',(8.1296257208938,1.10778692872341,4.51783113251438));
#87881=CARTESIAN_POINT('Ctrl Pts',(7.93077850215417,4.39943155644481,1.51095731293844));
#87882=CARTESIAN_POINT('Ctrl Pts',(7.7319312834145,3.64984844976654,-2.8838509523037));
#87883=CARTESIAN_POINT('Ctrl Pts',(7.5330840646749,-0.452410699785362,-4.62961278943379));
#87884=CARTESIAN_POINT('Ctrl Pts',(7.36909481088169,-3.49281806885017,-2.56216828706881));
#87885=CARTESIAN_POINT('Ctrl Pts',(7.27138796333505,-3.92736124061847,-0.624189342625645));
#87886=CARTESIAN_POINT('Ctrl Pts',(7.23996352203496,-3.92656899063656,-0.000561720325250592));
#87887=CARTESIAN_POINT('',(5.98996351374692,-3.9329983211402,0.00363399344691532));
#87888=CARTESIAN_POINT('Ctrl Pts',(7.23996352203496,-3.92656899063656,-0.000561720325250592));
#87889=CARTESIAN_POINT('Ctrl Pts',(7.2051055570885,-3.92569017717304,0.691205225988917));
#87890=CARTESIAN_POINT('Ctrl Pts',(7.10396518589552,-3.42135043251264,2.69956464192561));
#87891=CARTESIAN_POINT('Ctrl Pts',(6.93654240845595,-0.212207213519058,
4.64682236801925));
#87892=CARTESIAN_POINT('Ctrl Pts',(6.7376951897163,3.79420578519414,2.69109503379691));
#87893=CARTESIAN_POINT('Ctrl Pts',(6.53884797097666,4.31533904892208,-1.73661708911133));
#87894=CARTESIAN_POINT('Ctrl Pts',(6.34000075223702,0.872490233572671,-4.56910831715266));
#87895=CARTESIAN_POINT('Ctrl Pts',(6.15703926925645,-3.03273667556589,-3.31352679892515));
#87896=CARTESIAN_POINT('Ctrl Pts',(6.04036019252243,-3.92357217526684,-0.992555741609356));
#87897=CARTESIAN_POINT('Ctrl Pts',(5.98996352203496,-3.93273349467542,0.00363358492567481));
#87898=CARTESIAN_POINT('',(4.73996306897106,-3.93526991228507,-0.00111206807604383));
#87899=CARTESIAN_POINT('Ctrl Pts',(5.98996351374692,-3.9329983211402,0.00363399344691532));
#87900=CARTESIAN_POINT('Ctrl Pts',(5.98202064724872,-3.93285324270482,0.160649478238822));
#87901=CARTESIAN_POINT('Ctrl Pts',(5.97407778075052,-3.9233014529818,0.317245508222898));
#87902=CARTESIAN_POINT('Ctrl Pts',(5.96613491425232,-3.90451705950222,0.472478075741249));
#87903=CARTESIAN_POINT('Ctrl Pts',(5.95819204775412,-3.88573266602263,0.627710643259604));
#87904=CARTESIAN_POINT('Ctrl Pts',(5.95024918125592,-3.85771583767056,0.781580297371852));
#87905=CARTESIAN_POINT('Ctrl Pts',(5.94230631475772,-3.82069139828797,0.933169994721377));
#87906=CARTESIAN_POINT('Ctrl Pts',(5.93643386862468,-3.79331790209118,1.04524569588167));
#87907=CARTESIAN_POINT('Ctrl Pts',(5.93056142249165,-3.76096297306108,1.15630355929294));
#87908=CARTESIAN_POINT('Ctrl Pts',(5.92468897635861,-3.72371717926471,1.26586704232668));
#87909=CARTESIAN_POINT('Ctrl Pts',(5.91882413741464,-3.68651963381137,1.37528859640749));
#87910=CARTESIAN_POINT('Ctrl Pts',(5.91295929847068,-3.64444395475189,1.4832192320268));
#87911=CARTESIAN_POINT('Ctrl Pts',(5.90709445952671,-3.59763143455672,1.58919383999855));
#87912=CARTESIAN_POINT('Ctrl Pts',(5.90123564940756,-3.55086703579952,1.6950595102224));
#87913=CARTESIAN_POINT('Ctrl Pts',(5.89537683928841,-3.49937564720674,1.79897277639081));
#87914=CARTESIAN_POINT('Ctrl Pts',(5.88951802916926,-3.44334773993833,1.9004855542365));
#87915=CARTESIAN_POINT('Ctrl Pts',(5.88343224028796,-3.38514923065708,2.00593108364589));
#87916=CARTESIAN_POINT('Ctrl Pts',(5.87734645140666,-3.32205573726382,2.10878593601703));
#87917=CARTESIAN_POINT('Ctrl Pts',(5.87126066252536,-3.25433504916551,2.20857247736472));
#87918=CARTESIAN_POINT('Ctrl Pts',(5.86540863244795,-3.18921555334596,2.30452615776302));
#87919=CARTESIAN_POINT('Ctrl Pts',(5.85955660237055,-3.11981802600965,2.39764251681994));
#87920=CARTESIAN_POINT('Ctrl Pts',(5.85370457229313,-3.04642596735118,2.48752443715604));
#87921=CARTESIAN_POINT('Ctrl Pts',(5.84785343191546,-2.97304506668316,2.57739269250401));
#87922=CARTESIAN_POINT('Ctrl Pts',(5.84200229153779,-2.89567110356855,2.66402716678029));
#87923=CARTESIAN_POINT('Ctrl Pts',(5.83615115116012,-2.81462842866851,2.74706312423487));
#87924=CARTESIAN_POINT('Ctrl Pts',(5.83029948359346,-2.73357845180618,2.83010656324692));
#87925=CARTESIAN_POINT('Ctrl Pts',(5.8244478160268,-2.64885939478492,2.90955054506941));
#87926=CARTESIAN_POINT('Ctrl Pts',(5.81859614846013,-2.56083258049191,2.98506708378407));
#87927=CARTESIAN_POINT('Ctrl Pts',(5.81274253677673,-2.47277652079121,3.06060871158074));
#87928=CARTESIAN_POINT('Ctrl Pts',(5.80688892509331,-2.38141083219527,3.13222003270251));
#87929=CARTESIAN_POINT('Ctrl Pts',(5.8010353134099,-2.28712945529186,3.19961370398621));
#87930=CARTESIAN_POINT('Ctrl Pts',(5.79517504731083,-2.19274089883748,3.26708398873976));
#87931=CARTESIAN_POINT('Ctrl Pts',(5.78931478121175,-2.0954303747829,3.33032681318384));
#87932=CARTESIAN_POINT('Ctrl Pts',(5.78345451511267,-1.99562038779009,3.38909844469536));
#87933=CARTESIAN_POINT('Ctrl Pts',(5.77759030194217,-1.89574317566776,3.44790966072803));
#87934=CARTESIAN_POINT('Ctrl Pts',(5.77172608877166,-1.7933635127187,3.50224349405051));
#87935=CARTESIAN_POINT('Ctrl Pts',(5.76586187560116,-1.68892647949197,3.55190320066171));
#87936=CARTESIAN_POINT('Ctrl Pts',(5.75998902702765,-1.58433565651648,3.60163603414722));
#87937=CARTESIAN_POINT('Ctrl Pts',(5.75411617845415,-1.47768179613982,3.64668084374541));
#87938=CARTESIAN_POINT('Ctrl Pts',(5.74824332988064,-1.36942789005103,3.68688978055357));
#87939=CARTESIAN_POINT('Ctrl Pts',(5.74664858525979,-1.34003204708651,3.69780832968393));
#87940=CARTESIAN_POINT('Ctrl Pts',(5.74505384063894,-1.31051829331303,3.70837058492205));
#87941=CARTESIAN_POINT('Ctrl Pts',(5.74345909601809,-1.28089604188996,3.71857423347587));
#87942=CARTESIAN_POINT('Ctrl Pts',(5.73758664988517,-1.17181583334536,3.75614788364412));
#87943=CARTESIAN_POINT('Ctrl Pts',(5.73171420375225,-1.06089832724938,3.78898075281574));
#87944=CARTESIAN_POINT('Ctrl Pts',(5.72584175761934,-0.948593366590205,
3.81689135617731));
#87945=CARTESIAN_POINT('Ctrl Pts',(5.7199769186755,-0.836433886204774,3.84476580403699));
#87946=CARTESIAN_POINT('Ctrl Pts',(5.71411207973167,-0.722890922930174,
3.86773056754548));
#87947=CARTESIAN_POINT('Ctrl Pts',(5.70824724078784,-0.608432129045196,
3.88565301388911));
#87948=CARTESIAN_POINT('Ctrl Pts',(5.70238843066883,-0.494090994319299,
3.90355703665956));
#87949=CARTESIAN_POINT('Ctrl Pts',(5.69652962054982,-0.378836307483879,
3.91642898857999));
#87950=CARTESIAN_POINT('Ctrl Pts',(5.69067081043082,-0.263147990725255,
3.92418681193662));
#87951=CARTESIAN_POINT('Ctrl Pts',(5.68458502154947,-0.142977741556796,
3.93224518457001));
#87952=CARTESIAN_POINT('Ctrl Pts',(5.67849923266812,-0.0223400249760971,
3.9347850473329));
#87953=CARTESIAN_POINT('Ctrl Pts',(5.67241344378677,0.098218572576491,3.93177340547507));
#87954=CARTESIAN_POINT('Ctrl Pts',(5.66656141370954,0.214146442027974,3.92887744258883));
#87955=CARTESIAN_POINT('Ctrl Pts',(5.6607093836323,0.330000706919892,3.92084859275499));
#87956=CARTESIAN_POINT('Ctrl Pts',(5.65485735355507,0.445294017114708,3.90771061343107));
#87957=CARTESIAN_POINT('Ctrl Pts',(5.6490062131776,0.560569798959709,3.89457463150924));
#87958=CARTESIAN_POINT('Ctrl Pts',(5.64315507280013,0.675284385091858,3.87633111132621));
#87959=CARTESIAN_POINT('Ctrl Pts',(5.63730393242266,0.788955576823385,3.85305568319474));
#87960=CARTESIAN_POINT('Ctrl Pts',(5.63145226485621,0.902637010353221,3.82977815794229));
#87961=CARTESIAN_POINT('Ctrl Pts',(5.62560059728976,1.01527445761994,3.80146790639584));
#87962=CARTESIAN_POINT('Ctrl Pts',(5.61974892972331,1.12639664296063,3.76825153124457));
#87963=CARTESIAN_POINT('Ctrl Pts',(5.61389531804012,1.23755574675206,3.73502412051919));
#87964=CARTESIAN_POINT('Ctrl Pts',(5.60804170635693,1.34719819176531,3.6968874634026));
#87965=CARTESIAN_POINT('Ctrl Pts',(5.60218809467374,1.45486925466066,3.65401757683829));
#87966=CARTESIAN_POINT('Ctrl Pts',(5.5963278285749,1.56266271857008,3.61109895556803));
#87967=CARTESIAN_POINT('Ctrl Pts',(5.59046756247606,1.6684799429835,3.56343651803073));
#87968=CARTESIAN_POINT('Ctrl Pts',(5.58460729637722,1.77188744524885,3.5112538901893));
#87969=CARTESIAN_POINT('Ctrl Pts',(5.57874308320696,1.87536459568188,3.45903611572568));
#87970=CARTESIAN_POINT('Ctrl Pts',(5.57287887003671,1.97642843265265,3.40229229064337));
#87971=CARTESIAN_POINT('Ctrl Pts',(5.56701465686646,2.07467279374348,3.34129043917176));
#87972=CARTESIAN_POINT('Ctrl Pts',(5.56114180829321,2.17306182550464,3.28019875884234));
#87973=CARTESIAN_POINT('Ctrl Pts',(5.55526895971995,2.26862275522921,3.21483677054345));
#87974=CARTESIAN_POINT('Ctrl Pts',(5.5493961111467,2.36098086675533,3.14551400359548));
#87975=CARTESIAN_POINT('Ctrl Pts',(5.54780136652395,2.38606028092498,3.12668972974507));
#87976=CARTESIAN_POINT('Ctrl Pts',(5.54620662190119,2.41090373307759,3.10757361651467));
#87977=CARTESIAN_POINT('Ctrl Pts',(5.54461187727843,2.43550418788018,3.08817233178754));
#87978=CARTESIAN_POINT('Ctrl Pts',(5.53873943113927,2.52609226309035,3.01672954529684));
#87979=CARTESIAN_POINT('Ctrl Pts',(5.5328669850001,2.61368579665593,2.94117781889425));
#87980=CARTESIAN_POINT('Ctrl Pts',(5.52699453886093,2.697888887224,2.86179743381555));
#87981=CARTESIAN_POINT('Ctrl Pts',(5.52112969991083,2.78198290078835,2.78251987838954));
#87982=CARTESIAN_POINT('Ctrl Pts',(5.51526486096071,2.86269490746571,2.69942380821862));
#87983=CARTESIAN_POINT('Ctrl Pts',(5.50940002201061,2.9396604709751,2.61283090064903));
#87984=CARTESIAN_POINT('Ctrl Pts',(5.50354121188531,3.01654691689862,2.52632700719807));
#87985=CARTESIAN_POINT('Ctrl Pts',(5.49768240176003,3.08969430693681,2.436333733331));
#87986=CARTESIAN_POINT('Ctrl Pts',(5.49182359163473,3.15877411456896,2.34321042442395));
#87987=CARTESIAN_POINT('Ctrl Pts',(5.48573780275574,3.23053017357422,2.24647938422938));
#87988=CARTESIAN_POINT('Ctrl Pts',(5.47965201387674,3.29789677730239,2.14637119149389));
#87989=CARTESIAN_POINT('Ctrl Pts',(5.47356622499774,3.36055062539171,2.04332779900322));
#87990=CARTESIAN_POINT('Ctrl Pts',(5.46771419491422,3.42079790165401,1.9442423649284));
#87991=CARTESIAN_POINT('Ctrl Pts',(5.46186216483071,3.47668754891229,1.84244344313218));
#87992=CARTESIAN_POINT('Ctrl Pts',(5.45601013474719,3.52797603694193,1.73835384279596));
#87993=CARTESIAN_POINT('Ctrl Pts',(5.45015899436344,3.57925672744571,1.63428006747979));
#87994=CARTESIAN_POINT('Ctrl Pts',(5.44430785397969,3.6259374669571,1.52791667676196));
#87995=CARTESIAN_POINT('Ctrl Pts',(5.43845671359594,3.66782114660131,1.41971019456234));
#87996=CARTESIAN_POINT('Ctrl Pts',(5.43260504602323,3.70970859997375,1.31149396293624));
#87997=CARTESIAN_POINT('Ctrl Pts',(5.42675337845052,3.74679798505335,1.20143469522053));
#87998=CARTESIAN_POINT('Ctrl Pts',(5.42090171087781,3.77894097757415,1.08999728807505));
#87999=CARTESIAN_POINT('Ctrl Pts',(5.41504809918838,3.81109464905581,0.978522857752298));
#88000=CARTESIAN_POINT('Ctrl Pts',(5.40919448749896,3.8382985457707,0.865669774521691));
#88001=CARTESIAN_POINT('Ctrl Pts',(5.40334087580953,3.86045486117469,0.751915729874504));
#88002=CARTESIAN_POINT('Ctrl Pts',(5.39748060970452,3.88263636399089,0.638032369049923));
#88003=CARTESIAN_POINT('Ctrl Pts',(5.39162034359951,3.89975875333545,0.523246408476939));
#88004=CARTESIAN_POINT('Ctrl Pts',(5.3857600774945,3.91177575685306,0.408043414475324));
#88005=CARTESIAN_POINT('Ctrl Pts',(5.3798958643181,3.92380085419607,0.292762827676268));
#88006=CARTESIAN_POINT('Ctrl Pts',(5.37403165114171,3.93071369410298,0.177065059762018));
#88007=CARTESIAN_POINT('Ctrl Pts',(5.36816743796531,3.93252012476649,0.0614367016249753));
#88008=CARTESIAN_POINT('Ctrl Pts',(5.36229458938602,3.93432921550666,-0.0543619261508433));
#88009=CARTESIAN_POINT('Ctrl Pts',(5.35642174080672,3.93101690137764,-0.170090528525728));
#88010=CARTESIAN_POINT('Ctrl Pts',(5.35054889222743,3.92264094833718,-0.285266525250295));
#88011=CARTESIAN_POINT('Ctrl Pts',(5.34895414766455,3.92036649746554,-0.31654202845293));
#88012=CARTESIAN_POINT('Ctrl Pts',(5.34735940310168,3.91771896165528,-0.34777683884738));
#88013=CARTESIAN_POINT('Ctrl Pts',(5.3457646585388,3.91470014591244,-0.378961432857152));
#88014=CARTESIAN_POINT('Ctrl Pts',(5.33989221241209,3.90358373690938,-0.493794775179618));
#88015=CARTESIAN_POINT('Ctrl Pts',(5.33401976628539,3.88739167171587,-0.608330828265449));
#88016=CARTESIAN_POINT('Ctrl Pts',(5.32814732015868,3.86614565748962,-0.722085005435037));
#88017=CARTESIAN_POINT('Ctrl Pts',(5.32228248122103,3.84492716543104,-0.835691825010722));
#88018=CARTESIAN_POINT('Ctrl Pts',(5.31641764228337,3.81866781899638,-0.948518380274054));
#88019=CARTESIAN_POINT('Ctrl Pts',(5.31055280334572,3.78744116160702,-1.06008416994352));
#88020=CARTESIAN_POINT('Ctrl Pts',(5.30469399323286,3.75624660399882,-1.17153527434944));
#88021=CARTESIAN_POINT('Ctrl Pts',(5.29883518312001,3.72009500269545,-1.28172779534265));
#88022=CARTESIAN_POINT('Ctrl Pts',(5.29297637300715,3.67911100457593,-1.39019107176254));
#88023=CARTESIAN_POINT('Ctrl Pts',(5.28689058412348,3.63653922713999,-1.50285637225994));
#88024=CARTESIAN_POINT('Ctrl Pts',(5.28080479523981,3.58875313545733,-1.61365528480874));
#88025=CARTESIAN_POINT('Ctrl Pts',(5.27471900635615,3.53594969233564,-1.72207687786333));
#88026=CARTESIAN_POINT('Ctrl Pts',(5.26886697628494,3.48517446123275,-1.82633393229826));
#88027=CARTESIAN_POINT('Ctrl Pts',(5.26301494621373,3.42976040546521,-1.92839252097583));
#88028=CARTESIAN_POINT('Ctrl Pts',(5.25716291614252,3.36993151659851,-2.02781916684798));
#88029=CARTESIAN_POINT('Ctrl Pts',(5.25131177577101,3.31011172367697,-2.12723069662262));
#88030=CARTESIAN_POINT('Ctrl Pts',(5.2454606353995,3.24587864528334,-2.22401072512109));
#88031=CARTESIAN_POINT('Ctrl Pts',(5.239609495028,3.17750132253168,-2.31775200254674));
#88032=CARTESIAN_POINT('Ctrl Pts',(5.23375782746744,3.1091178389681,-2.41150172608223));
#88033=CARTESIAN_POINT('Ctrl Pts',(5.22790615990689,3.0365896123767,-2.50221182029704));
#88034=CARTESIAN_POINT('Ctrl Pts',(5.22205449234634,2.96022751752167,-2.58950613911369));
#88035=CARTESIAN_POINT('Ctrl Pts',(5.21620088066899,2.88384005266226,-2.67682945997979));
#88036=CARTESIAN_POINT('Ctrl Pts',(5.21034726899164,2.80361645880228,-2.760734437947));
#88037=CARTESIAN_POINT('Ctrl Pts',(5.20449365731428,2.71990568928164,-2.84088050459948));
#88038=CARTESIAN_POINT('Ctrl Pts',(5.19863339122115,2.63609975692873,-2.92111768171171));
#88039=CARTESIAN_POINT('Ctrl Pts',(5.192773125128,2.54879903517819,-2.99758713241532));
#88040=CARTESIAN_POINT('Ctrl Pts',(5.18691285903486,2.45838696680936,-3.06998738131313));
#88041=CARTESIAN_POINT('Ctrl Pts',(5.18104864587024,2.36791400310042,-3.14243639403043));
#88042=CARTESIAN_POINT('Ctrl Pts',(5.17518443270562,2.27432585298839,-3.21081050433854));
#88043=CARTESIAN_POINT('Ctrl Pts',(5.16932021954099,2.17803500324615,-3.27485152711303));
#88044=CARTESIAN_POINT('Ctrl Pts',(5.16344737097323,2.08160235949294,-3.3389868541076));
#88045=CARTESIAN_POINT('Ctrl Pts',(5.15757452240548,1.98245942568906,-3.39877614624009));
#88046=CARTESIAN_POINT('Ctrl Pts',(5.15170167383772,1.88104338728578,-3.45400706066858));
#88047=CARTESIAN_POINT('Ctrl Pts',(5.1501069291582,1.85350433433802,-3.46900475827881));
#88048=CARTESIAN_POINT('Ctrl Pts',(5.14851218447868,1.8257977816723,-3.4836666104459));
#88049=CARTESIAN_POINT('Ctrl Pts',(5.14691743979915,1.79793271659332,-3.4979889860609));
#88050=CARTESIAN_POINT('Ctrl Pts',(5.14104499366954,1.69532312919306,-3.55072932771384));
#88051=CARTESIAN_POINT('Ctrl Pts',(5.13517254753993,1.59021916487394,-3.59903923479842));
#88052=CARTESIAN_POINT('Ctrl Pts',(5.12930010141032,1.48304019955298,-3.64267494658937));
#88053=CARTESIAN_POINT('Ctrl Pts',(5.12343526246986,1.37600007427319,-3.68625413251255));
#88054=CARTESIAN_POINT('Ctrl Pts',(5.1175704235294,1.266890672711,-3.72517100989488));
#88055=CARTESIAN_POINT('Ctrl Pts',(5.11170558458894,1.15615596250871,-3.75922763215472));
#88056=CARTESIAN_POINT('Ctrl Pts',(5.10584677447338,1.04553508325471,-3.79324924553974));
#88057=CARTESIAN_POINT('Ctrl Pts',(5.09998796435781,0.933292611302778,-3.82242042064039));
#88058=CARTESIAN_POINT('Ctrl Pts',(5.09412915424225,0.819891868860637,-3.84659152021321));
#88059=CARTESIAN_POINT('Ctrl Pts',(5.08804336535964,0.702097817846483,-3.87169904309917));
#88060=CARTESIAN_POINT('Ctrl Pts',(5.08195757647703,0.583054355908134,-3.89141106328964));
#88061=CARTESIAN_POINT('Ctrl Pts',(5.07587178759441,0.463297783022315,-3.90561700173565));
#88062=CARTESIAN_POINT('Ctrl Pts',(5.07001975752076,0.348141132082977,-3.91927728154721));
#88063=CARTESIAN_POINT('Ctrl Pts',(5.0641677274471,0.23232559014042,-3.92784660775168));
#88064=CARTESIAN_POINT('Ctrl Pts',(5.05831569737345,0.116336916484687,-3.9312790185718));
#88065=CARTESIAN_POINT('Ctrl Pts',(5.0524645569996,0.000365876897616496,
-3.93471090755331));
#88066=CARTESIAN_POINT('Ctrl Pts',(5.04661341662574,-0.115777829003163,
-3.93300742176772));
#88067=CARTESIAN_POINT('Ctrl Pts',(5.04076227625189,-0.231606145773011,
-3.92617467686299));
#88068=CARTESIAN_POINT('Ctrl Pts',(5.03491060868909,-0.347444898697882,
-3.91934131632654));
#88069=CARTESIAN_POINT('Ctrl Pts',(5.0290589411263,-0.462967793337763,-3.90737780230802));
#88070=CARTESIAN_POINT('Ctrl Pts',(5.0232072735635,-0.577690319090831,-3.89034225939425));
#88071=CARTESIAN_POINT('Ctrl Pts',(5.01735366188401,-0.692450959445473,
-3.87330105671203));
#88072=CARTESIAN_POINT('Ctrl Pts',(5.01150005020452,-0.806410293512435,
-3.85118453510873));
#88073=CARTESIAN_POINT('Ctrl Pts',(5.00564643852502,-0.919093149460135,
-3.82410208841441));
#88074=CARTESIAN_POINT('Ctrl Pts',(4.99978617242991,-1.03190410385344,-3.7969888542565));
#88075=CARTESIAN_POINT('Ctrl Pts',(4.99392590633479,-1.14343528161755,-3.7648985238529));
#88076=CARTESIAN_POINT('Ctrl Pts',(4.98806564023968,-1.25322574752353,-3.72799064185307));
#88077=CARTESIAN_POINT('Ctrl Pts',(4.98220142707317,-1.3630901607212,-3.69105790124742));
#88078=CARTESIAN_POINT('Ctrl Pts',(4.97633721390667,-1.47121114287337,-3.64930129660987));
#88079=CARTESIAN_POINT('Ctrl Pts',(4.97047300074017,-1.5771484705297,-3.60292821214992));
#88080=CARTESIAN_POINT('Ctrl Pts',(4.96460015217067,-1.68324179720764,-3.55648684056243));
#88081=CARTESIAN_POINT('Ctrl Pts',(4.95872730360118,-1.78714468219978,-3.50541560327032));
#88082=CARTESIAN_POINT('Ctrl Pts',(4.95285445503169,-1.88844211016409,-3.4499674486231));
#88083=CARTESIAN_POINT('Ctrl Pts',(4.9512597103743,-1.91594895460962,-3.43491076065655));
#88084=CARTESIAN_POINT('Ctrl Pts',(4.9496649657169,-1.94326385169254,-3.41953157537305));
#88085=CARTESIAN_POINT('Ctrl Pts',(4.94807022105951,-1.97037888736429,-3.40383548959539));
#88086=CARTESIAN_POINT('Ctrl Pts',(4.94219777489032,-2.07022658813591,-3.34603663234931));
#88087=CARTESIAN_POINT('Ctrl Pts',(4.93632532872113,-2.16769610294611,-3.28374390161609));
#88088=CARTESIAN_POINT('Ctrl Pts',(4.93045288255193,-2.26235561724438,-3.2171782762419));
#88089=CARTESIAN_POINT('Ctrl Pts',(4.92458804357171,-2.35689250924991,-3.15069888023051));
#88090=CARTESIAN_POINT('Ctrl Pts',(4.91872320459149,-2.44862630457141,-3.07995783255189));
#88091=CARTESIAN_POINT('Ctrl Pts',(4.91285836561127,-2.53715043092722,-3.00522157100701));
#88092=CARTESIAN_POINT('Ctrl Pts',(4.9069995554558,-2.62558355794854,-2.93056213541165));
#88093=CARTESIAN_POINT('Ctrl Pts',(4.90114074530033,-2.71081326476782,-2.85191591989841));
#88094=CARTESIAN_POINT('Ctrl Pts',(4.89528193514485,-2.79246315213798,-2.76959176485481));
#88095=CARTESIAN_POINT('Ctrl Pts',(4.88919614627715,-2.8772762733044,-2.68407825391778));
#88096=CARTESIAN_POINT('Ctrl Pts',(4.88311035740944,-2.9582262187963,-2.59459632385733));
#88097=CARTESIAN_POINT('Ctrl Pts',(4.87702456854174,-3.0349299856515,-2.5015373237658));
#88098=CARTESIAN_POINT('Ctrl Pts',(4.87117253842811,-3.10868751540201,-2.41205277497225));
#88099=CARTESIAN_POINT('Ctrl Pts',(4.86532050831447,-3.17851875865221,-2.31926123041867));
#88100=CARTESIAN_POINT('Ctrl Pts',(4.85946847820085,-3.24412239692127,-2.22354646315156));
#88101=CARTESIAN_POINT('Ctrl Pts',(4.85361733778706,-3.3097160612932,-2.12784624765729));
#88102=CARTESIAN_POINT('Ctrl Pts',(4.84776619737327,-3.37108316501876,-2.02922403397522));
#88103=CARTESIAN_POINT('Ctrl Pts',(4.84191505695948,-3.4279649560572,-1.9280936854945));
#88104=CARTESIAN_POINT('Ctrl Pts',(4.83606338935682,-3.4848518721558,-1.82695422515019));
#88105=CARTESIAN_POINT('Ctrl Pts',(4.83021172175417,-3.53725246954495,-1.72330654107269));
#88106=CARTESIAN_POINT('Ctrl Pts',(4.82436005415152,-3.5849536632997,-1.61758963646349));
#88107=CARTESIAN_POINT('Ctrl Pts',(4.81850644243229,-3.63267070496106,-1.51183760921898));
#88108=CARTESIAN_POINT('Ctrl Pts',(4.81265283071305,-3.67568506852689,-1.40401537104218));
#88109=CARTESIAN_POINT('Ctrl Pts',(4.80679921899382,-3.71383184678538,-1.29458179108261));
#88110=CARTESIAN_POINT('Ctrl Pts',(4.80093895285935,-3.75202199049317,-1.18502380647921));
#88111=CARTESIAN_POINT('Ctrl Pts',(4.7950786867249,-3.78533336808122,-1.07385121447151));
#88112=CARTESIAN_POINT('Ctrl Pts',(4.78921842059044,-3.81365095753085,-0.961538025313615));
#88113=CARTESIAN_POINT('Ctrl Pts',(4.78335420738475,-3.84198761975633,-0.849149189735145));
#88114=CARTESIAN_POINT('Ctrl Pts',(4.77748999417906,-3.86532371347404,-0.735618631212591));
#88115=CARTESIAN_POINT('Ctrl Pts',(4.77162578097338,-3.88359565880033,-0.62142880440744));
#88116=CARTESIAN_POINT('Ctrl Pts',(4.76575293236526,-3.90189451065192,-0.507070826296558));
#88117=CARTESIAN_POINT('Ctrl Pts',(4.75988008375715,-3.91511428388645,-0.392052051464341));
#88118=CARTESIAN_POINT('Ctrl Pts',(4.75400723514904,-3.9232433578633,-0.276858366284093));
#88119=CARTESIAN_POINT('Ctrl Pts',(4.75241249087265,-3.92545076947256,-0.245578065636703));
#88120=CARTESIAN_POINT('Ctrl Pts',(4.75081774659625,-3.92728310573871,-0.214284855227092));
#88121=CARTESIAN_POINT('Ctrl Pts',(4.74922300231986,-3.92874079555149,-0.182988418675829));
#88122=CARTESIAN_POINT('Ctrl Pts',(4.74613650889156,-3.93156203159178,-0.122416797774472));
#88123=CARTESIAN_POINT('Ctrl Pts',(4.74305001546326,-3.93298256131418,-0.0617794293185965));
#88124=CARTESIAN_POINT('Ctrl Pts',(4.73996352203496,-3.93299984043219,-0.00112033939962684));
#88125=CARTESIAN_POINT('',(3.48996393051077,-3.93195649834994,-0.00308191760686356));
#88126=CARTESIAN_POINT('Ctrl Pts',(4.73996229954107,-3.9391251331115,-0.00109802104096923));
#88127=CARTESIAN_POINT('Ctrl Pts',(4.67676679422078,-3.93442811003921,1.24282384787021));
#88128=CARTESIAN_POINT('Ctrl Pts',(4.54728888265397,-2.62580980838282,3.79991380728597));
#88129=CARTESIAN_POINT('Ctrl Pts',(4.35152856484057,1.7326990630354,4.31691369475902));
#88130=CARTESIAN_POINT('Ctrl Pts',(4.15268134610093,4.56831442476183,0.876637571345176));
#88131=CARTESIAN_POINT('Ctrl Pts',(3.95383412736129,3.20756968977473,-3.36889996732418));
#88132=CARTESIAN_POINT('Ctrl Pts',(3.75498690862166,-1.0995828420239,-4.51983480521305));
#88133=CARTESIAN_POINT('Ctrl Pts',(3.60036385291742,-3.66339751277891,-2.18634896287544));
#88134=CARTESIAN_POINT('Ctrl Pts',(3.51202320345975,-3.93249893558521,-0.440083035469798));
#88135=CARTESIAN_POINT('Ctrl Pts',(3.48996496024862,-3.9293289361394,-0.00310026290872592));
#88136=CARTESIAN_POINT('',(2.23996299489525,-3.93122786339409,0.00239984451894347));
#88137=CARTESIAN_POINT('Ctrl Pts',(3.48996352203496,-3.93299879819285,-0.00307464040323634));
#88138=CARTESIAN_POINT('Ctrl Pts',(3.48411632698161,-3.93308943701494,0.112868146911366));
#88139=CARTESIAN_POINT('Ctrl Pts',(3.47826913192826,-3.92804887411316,0.22887230601759));
#88140=CARTESIAN_POINT('Ctrl Pts',(3.47242193687491,-3.91788758060137,0.344450149904952));
#88141=CARTESIAN_POINT('Ctrl Pts',(3.46657571648118,-3.90772798085939,0.46000872830586));
#88142=CARTESIAN_POINT('Ctrl Pts',(3.46072949608744,-3.89244938353798,0.575140720950829));
#88143=CARTESIAN_POINT('Ctrl Pts',(3.45488327569371,-3.87211425780453,0.689362150474535));
#88144=CARTESIAN_POINT('Ctrl Pts',(3.44903661305097,-3.85177759377994,0.803592220506071));
#88145=CARTESIAN_POINT('Ctrl Pts',(3.44318995040824,-3.82638371318358,0.91691118327512));
#88146=CARTESIAN_POINT('Ctrl Pts',(3.4373432877655,-3.79604634517697,1.02884456808043));
#88147=CARTESIAN_POINT('Ctrl Pts',(3.43149476598082,-3.76569933038948,1.14081354584936));
#88148=CARTESIAN_POINT('Ctrl Pts',(3.42564624419614,-3.73040581037212,1.25139567053234));
#88149=CARTESIAN_POINT('Ctrl Pts',(3.41979772241146,-3.6903293742723,1.3601316514893));
#88150=CARTESIAN_POINT('Ctrl Pts',(3.41394225952107,-3.65020537490952,1.46899668179694));
#88151=CARTESIAN_POINT('Ctrl Pts',(3.40808679663068,-3.60528726960042,1.57601080554061));
#88152=CARTESIAN_POINT('Ctrl Pts',(3.40223133374028,-3.55578687625916,1.68073456875947));
#88153=CARTESIAN_POINT('Ctrl Pts',(3.39637201236529,-3.50625386440274,1.78552734019076));
#88154=CARTESIAN_POINT('Ctrl Pts',(3.3905126909903,-3.45213274449892,1.88802638072238));
#88155=CARTESIAN_POINT('Ctrl Pts',(3.38465336961531,-3.39368049041652,1.98781833399491));
#88156=CARTESIAN_POINT('Ctrl Pts',(3.37878453779344,-3.33513336066125,2.08777226269272));
#88157=CARTESIAN_POINT('Ctrl Pts',(3.37291570597156,-3.2722412835245,2.18500998390483));
#88158=CARTESIAN_POINT('Ctrl Pts',(3.36704687414968,-3.20530376084862,2.27914826211234));
#88159=CARTESIAN_POINT('Ctrl Pts',(3.36379540648058,-3.16821883535809,2.33130303112039));
#88160=CARTESIAN_POINT('Ctrl Pts',(3.36054393881147,-3.12989290496863,2.38250705129076));
#88161=CARTESIAN_POINT('Ctrl Pts',(3.35729247114236,-3.09038186934412,2.432699920177));
#88162=CARTESIAN_POINT('Ctrl Pts',(3.35142002361739,-3.01902133097346,2.52335282485225));
#88163=CARTESIAN_POINT('Ctrl Pts',(3.34554757609242,-2.94354913470549,2.61101491801737));
#88164=CARTESIAN_POINT('Ctrl Pts',(3.33967512856745,-2.86424520234117,2.6952900439221));
#88165=CARTESIAN_POINT('Ctrl Pts',(3.33381028825484,-2.78504400088289,2.77945599919956));
#88166=CARTESIAN_POINT('Ctrl Pts',(3.32794544794224,-2.70202121494443,2.8602434141433));
#88167=CARTESIAN_POINT('Ctrl Pts',(3.32208060762963,-2.61549819098514,2.9372875604805));
#88168=CARTESIAN_POINT('Ctrl Pts',(3.31622179616635,-2.52906410964768,3.01425250814827));
#88169=CARTESIAN_POINT('Ctrl Pts',(3.31036298470306,-2.43913725400455,3.08748156775208));
#88170=CARTESIAN_POINT('Ctrl Pts',(3.30450417323977,-2.3460766711313,3.15664588656591));
#88171=CARTESIAN_POINT('Ctrl Pts',(3.29841838487156,-2.2494108172567,3.22848970840077));
#88172=CARTESIAN_POINT('Ctrl Pts',(3.29233259650335,-2.14936382859677,3.29594714366392));
#88173=CARTESIAN_POINT('Ctrl Pts',(3.28624680813514,-2.04637736394949,3.35869449106571));
#88174=CARTESIAN_POINT('Ctrl Pts',(3.28039477678235,-1.94734664129446,3.41903169342689));
#88175=CARTESIAN_POINT('Ctrl Pts',(3.27454274542955,-1.84559847528112,3.47501373042732));
#88176=CARTESIAN_POINT('Ctrl Pts',(3.26869071407675,-1.74155545392517,3.52639668796684));
#88177=CARTESIAN_POINT('Ctrl Pts',(3.26283957245104,-1.63752825098992,3.57777183337991));
#88178=CARTESIAN_POINT('Ctrl Pts',(3.25698843082532,-1.53120725696807,3.62454910664573));
#88179=CARTESIAN_POINT('Ctrl Pts',(3.25113728919961,-1.42303881675763,3.66653099345976));
#88180=CARTESIAN_POINT('Ctrl Pts',(3.24528562041344,-1.31486063107721,3.70851666264523));
#88181=CARTESIAN_POINT('Ctrl Pts',(3.23943395162726,-1.20483505370261,3.74570593694982));
#88182=CARTESIAN_POINT('Ctrl Pts',(3.23358228284108,-1.09342684656628,3.77795006997288));
#88183=CARTESIAN_POINT('Ctrl Pts',(3.22772866996789,-0.98198162652704,3.81020491539313));
#88184=CARTESIAN_POINT('Ctrl Pts',(3.22187505709471,-0.869153260191447,
3.83751123784089));
#88185=CARTESIAN_POINT('Ctrl Pts',(3.21602144422152,-0.75541935019651,3.85977079699672));
#88186=CARTESIAN_POINT('Ctrl Pts',(3.21016117698241,-0.641556147904519,
3.88205566073879));
#88187=CARTESIAN_POINT('Ctrl Pts',(3.2043009097433,-0.52678575316777,3.89928223060361));
#88188=CARTESIAN_POINT('Ctrl Pts',(3.1984406425042,-0.411593690247987,3.91140379328804));
#88189=CARTESIAN_POINT('Ctrl Pts',(3.19257642822118,-0.296324042448196,
3.92353352016331));
#88190=CARTESIAN_POINT('Ctrl Pts',(3.18671221393815,-0.180632572544359,
3.9305513684321));
#88191=CARTESIAN_POINT('Ctrl Pts',(3.18084799965514,-0.0650058767105533,
3.93246274438717));
#88192=CARTESIAN_POINT('Ctrl Pts',(3.17497515001786,0.0507910853228681,
3.9343769349407));
#88193=CARTESIAN_POINT('Ctrl Pts',(3.1691023003806,0.166522671277312,3.93116965708302));
#88194=CARTESIAN_POINT('Ctrl Pts',(3.16322945074332,0.281706248466385,3.92289823849345));
#88195=CARTESIAN_POINT('Ctrl Pts',(3.16163471796312,0.312983573381783,3.92065219046255));
#88196=CARTESIAN_POINT('Ctrl Pts',(3.16003998518292,0.344220544794587,3.91803302618818));
#88197=CARTESIAN_POINT('Ctrl Pts',(3.15844525240272,0.375407637705265,3.91504254198502));
#88198=CARTESIAN_POINT('Ctrl Pts',(3.15257279710596,0.490251209761825,3.90403036175223));
#88199=CARTESIAN_POINT('Ctrl Pts',(3.14670034180919,0.604802094702504,3.88794224156575));
#88200=CARTESIAN_POINT('Ctrl Pts',(3.14082788651243,0.718575685062651,3.86679944978231));
#88201=CARTESIAN_POINT('Ctrl Pts',(3.13496303835688,0.832201893838007,3.84568404623677));
#88202=CARTESIAN_POINT('Ctrl Pts',(3.12909819020133,0.945052407752413,3.81952706714544));
#88203=CARTESIAN_POINT('Ctrl Pts',(3.12323334204578,1.05664665780864,3.78840162080815));
#88204=CARTESIAN_POINT('Ctrl Pts',(3.11737452267839,1.1681261942224,3.75730816996633));
#88205=CARTESIAN_POINT('Ctrl Pts',(3.11151570331101,1.27835163963612,3.72125652106592));
#88206=CARTESIAN_POINT('Ctrl Pts',(3.10565688394362,1.386852218885,3.68037089475691));
#88207=CARTESIAN_POINT('Ctrl Pts',(3.09957109851527,1.4995560253613,3.63790139139486));
#88208=CARTESIAN_POINT('Ctrl Pts',(3.09348531308692,1.61039817633966,3.59021589026558));
#88209=CARTESIAN_POINT('Ctrl Pts',(3.08739952765856,1.71886756388629,3.53751089013442));
#88210=CARTESIAN_POINT('Ctrl Pts',(3.08154748829966,1.82317080175622,3.48683021155815));
#88211=CARTESIAN_POINT('Ctrl Pts',(3.07569544894075,1.92527977674601,3.43150870229928));
#88212=CARTESIAN_POINT('Ctrl Pts',(3.06984340958185,2.0247608077048,3.37176996124923));
#88213=CARTESIAN_POINT('Ctrl Pts',(3.06399225992613,2.1242267142625,3.31204030246009));
#88214=CARTESIAN_POINT('Ctrl Pts',(3.05814111027041,2.22106511691968,3.2478949599131));
#88215=CARTESIAN_POINT('Ctrl Pts',(3.0522899606147,2.31486852090247,3.1796026058196));
#88216=CARTESIAN_POINT('Ctrl Pts',(3.04643828378327,2.4086803763656,3.11130409873524));
#88217=CARTESIAN_POINT('Ctrl Pts',(3.04058660695183,2.49945635537347,3.03885808065493));
#88218=CARTESIAN_POINT('Ctrl Pts',(3.0347349301204,2.58682002889609,2.96257508564797));
#88219=CARTESIAN_POINT('Ctrl Pts',(3.02888130919533,2.67421272711832,2.88626674725826));
#88220=CARTESIAN_POINT('Ctrl Pts',(3.02302768827026,2.75819055443164,2.80611916890222));
#88221=CARTESIAN_POINT('Ctrl Pts',(3.01717406734519,2.83841262488372,2.72248099550772));
#88222=CARTESIAN_POINT('Ctrl Pts',(3.01131379208539,2.91872589094215,2.63874774311696));
#88223=CARTESIAN_POINT('Ctrl Pts',(3.00545351682559,2.99527459205026,2.55151627404036));
#88224=CARTESIAN_POINT('Ctrl Pts',(2.99959324156578,3.06775690394131,2.46116975812731));
#88225=CARTESIAN_POINT('Ctrl Pts',(2.99372901927034,3.14028803440413,2.37076239167353));
#88226=CARTESIAN_POINT('Ctrl Pts',(2.9878647969749,3.20874707857506,2.27723613345821));
#88227=CARTESIAN_POINT('Ctrl Pts',(2.98200057467946,3.27287547605126,2.18100323664643));
#88228=CARTESIAN_POINT('Ctrl Pts',(2.97612771710436,3.33709830491464,2.08462863340981));
#88229=CARTESIAN_POINT('Ctrl Pts',(2.97025485952926,3.39697754681083,1.98553978951168));
#88230=CARTESIAN_POINT('Ctrl Pts',(2.96438200195416,3.45230046115742,1.88417369843979));
#88231=CARTESIAN_POINT('Ctrl Pts',(2.96278734585713,3.46732228342025,1.8566497796162));
#88232=CARTESIAN_POINT('Ctrl Pts',(2.9611926897601,3.48200844963443,1.82895807502124));
#88233=CARTESIAN_POINT('Ctrl Pts',(2.95959803366308,3.49635532112986,1.80110756713943));
#88234=CARTESIAN_POINT('Ctrl Pts',(2.95372561157408,3.54918858419822,1.69854630770556));
#88235=CARTESIAN_POINT('Ctrl Pts',(2.94785318948509,3.59759371831676,1.59348666178647));
#88236=CARTESIAN_POINT('Ctrl Pts',(2.9419807673961,3.64132658202465,1.48634777997637));
#88237=CARTESIAN_POINT('Ctrl Pts',(2.93611595250998,3.68500279367965,1.37934768710173));
#88238=CARTESIAN_POINT('Ctrl Pts',(2.93025113762386,3.7240186164411,1.27027409385835));
#88239=CARTESIAN_POINT('Ctrl Pts',(2.92438632273774,3.75817570053078,1.15957078435943));
#88240=CARTESIAN_POINT('Ctrl Pts',(2.91852753666256,3.79229767241213,1.04898127373329));
#88241=CARTESIAN_POINT('Ctrl Pts',(2.91266875058738,3.82157071901731,0.936765771704727));
#88242=CARTESIAN_POINT('Ctrl Pts',(2.9068099645122,3.84584478224221,0.823387460980775));
#88243=CARTESIAN_POINT('Ctrl Pts',(2.90072416661267,3.87105939856231,0.705616052978784));
#88244=CARTESIAN_POINT('Ctrl Pts',(2.89463836871314,3.89087962997266,0.586590322926661));
#88245=CARTESIAN_POINT('Ctrl Pts',(2.88855257081361,3.90519440852007,0.466846475475124));
#88246=CARTESIAN_POINT('Ctrl Pts',(2.88270056459753,3.91895927130785,0.35170270120082));
#88247=CARTESIAN_POINT('Ctrl Pts',(2.87684855838146,3.92763381818308,0.235895414327885));
#88248=CARTESIAN_POINT('Ctrl Pts',(2.87099655216538,3.93117164634012,0.119910329044353));
#88249=CARTESIAN_POINT('Ctrl Pts',(2.86514543554189,3.9347089366943,0.00394287523073171));
#88250=CARTESIAN_POINT('Ctrl Pts',(2.85929431891841,3.93311104833125,-0.112201910197163));
#88251=CARTESIAN_POINT('Ctrl Pts',(2.85344320229492,3.92638365376652,-0.228035969608107));
#88252=CARTESIAN_POINT('Ctrl Pts',(2.84759155835066,3.91965565290812,-0.343880468343655));
#88253=CARTESIAN_POINT('Ctrl Pts',(2.84173991440638,3.90779725083232,-0.45941377270361));
#88254=CARTESIAN_POINT('Ctrl Pts',(2.83588827046212,3.89086613218934,-0.574151322720711));
#88255=CARTESIAN_POINT('Ctrl Pts',(2.83003468224454,3.87392938799522,-0.688926995555842));
#88256=CARTESIAN_POINT('Ctrl Pts',(2.82418109402696,3.85191663609957,-0.802905979592701));
#88257=CARTESIAN_POINT('Ctrl Pts',(2.81832750580938,3.82493683883739,-0.915613007173139));
#88258=CARTESIAN_POINT('Ctrl Pts',(2.81246726282683,3.79792636907092,-1.02844816791758));
#88259=CARTESIAN_POINT('Ctrl Pts',(2.80660701984427,3.76593767924005,-1.14000808370118));
#88260=CARTESIAN_POINT('Ctrl Pts',(2.80074677686172,3.72912989537711,-1.24983167802897));
#88261=CARTESIAN_POINT('Ctrl Pts',(2.79488258663309,3.69229731913259,-1.35972924552687));
#88262=CARTESIAN_POINT('Ctrl Pts',(2.78901839640448,3.65063933369313,-1.46788777801986));
#88263=CARTESIAN_POINT('Ctrl Pts',(2.78315420617585,3.60436292335855,-1.57386686753301));
#88264=CARTESIAN_POINT('Ctrl Pts',(2.77728138011082,3.55801836456807,-1.68000202600781));
#88265=CARTESIAN_POINT('Ctrl Pts',(2.77140855404578,3.5070419882155,-1.78395096617584));
#88266=CARTESIAN_POINT('Ctrl Pts',(2.76553572798075,3.45168636551509,-1.88529844696197));
#88267=CARTESIAN_POINT('Ctrl Pts',(2.76394075696164,3.43665261294448,-1.91282289480423));
#88268=CARTESIAN_POINT('Ctrl Pts',(2.76234578594253,3.42129609739214,-1.94015563395403));
#88269=CARTESIAN_POINT('Ctrl Pts',(2.76075081492342,3.40562241094693,-1.96728874191259));
#88270=CARTESIAN_POINT('Ctrl Pts',(2.75487835257712,3.34791406867954,-2.0671890867564));
#88271=CARTESIAN_POINT('Ctrl Pts',(2.74900589023081,3.28570967715722,-2.16471531238949));
#88272=CARTESIAN_POINT('Ctrl Pts',(2.7431334278845,3.21922982444765,-2.25943540234873));
#88273=CARTESIAN_POINT('Ctrl Pts',(2.73726857287381,3.15283609141345,-2.35403278951807));
#88274=CARTESIAN_POINT('Ctrl Pts',(2.73140371786311,3.08217814665517,-2.44583093479365));
#88275=CARTESIAN_POINT('Ctrl Pts',(2.72553886285242,3.00752206006605,-2.53442302274424));
#88276=CARTESIAN_POINT('Ctrl Pts',(2.71968003682938,2.93294271887362,-2.62292403928668));
#88277=CARTESIAN_POINT('Ctrl Pts',(2.71382121080633,2.85437367569844,-2.70822523980445));
#88278=CARTESIAN_POINT('Ctrl Pts',(2.70796238478329,2.77212343038123,-2.78994994340963));
#88279=CARTESIAN_POINT('Ctrl Pts',(2.70187660192498,2.68668700829345,-2.87484046556288));
#88280=CARTESIAN_POINT('Ctrl Pts',(2.69579081906666,2.5972786756073,-2.9558714255448));
#88281=CARTESIAN_POINT('Ctrl Pts',(2.68970503620834,2.50428943062393,-3.03265946780466));
#88282=CARTESIAN_POINT('Ctrl Pts',(2.68385299072671,2.41487163448912,-3.10649830271091));
#88283=CARTESIAN_POINT('Ctrl Pts',(2.67800094524509,2.32214326583393,-3.17641383745267));
#88284=CARTESIAN_POINT('Ctrl Pts',(2.67214889976346,2.2264878251748,-3.24210440367801));
#88285=CARTESIAN_POINT('Ctrl Pts',(2.66629774419067,2.13084693064702,-3.30778498047047));
#88286=CARTESIAN_POINT('Ctrl Pts',(2.66044658861787,2.03228018979642,-3.36924163227354));
#88287=CARTESIAN_POINT('Ctrl Pts',(2.65459543304507,1.93120123218828,-3.42621522978263));
#88288=CARTESIAN_POINT('Ctrl Pts',(2.64874375050741,1.83011317123999,-3.4831939584293));
#88289=CARTESIAN_POINT('Ctrl Pts',(2.64289206796976,1.72651280387504,-3.5356886271821));
#88290=CARTESIAN_POINT('Ctrl Pts',(2.6370403854321,1.62083894102801,-3.58348575094798));
#88291=CARTESIAN_POINT('Ctrl Pts',(2.63118675901707,1.51512997425494,-3.63129875249718));
#88292=CARTESIAN_POINT('Ctrl Pts',(2.62533313260203,1.40734651879081,-3.67441093587548));
#88293=CARTESIAN_POINT('Ctrl Pts',(2.61947950618699,1.29794729539229,-3.71265697558822));
#88294=CARTESIAN_POINT('Ctrl Pts',(2.61361922578293,1.18842371468409,-3.75094649069737));
#88295=CARTESIAN_POINT('Ctrl Pts',(2.60775894537886,1.0772810904951,-3.78435868498092));
#88296=CARTESIAN_POINT('Ctrl Pts',(2.60189866497479,0.964993330107935,-3.81277810432855));
#88297=CARTESIAN_POINT('Ctrl Pts',(2.59603443772972,0.852629945022748,-3.84121666387453));
#88298=CARTESIAN_POINT('Ctrl Pts',(2.59017021048466,0.739120291873598,-3.8646556695139));
#88299=CARTESIAN_POINT('Ctrl Pts',(2.58430598323959,0.624946769273544,-3.88303110154613));
#88300=CARTESIAN_POINT('Ctrl Pts',(2.57843312103693,0.510605128439833,-3.90143359103534));
#88301=CARTESIAN_POINT('Ctrl Pts',(2.57256025883427,0.395598076254214,-3.91475757881186));
#88302=CARTESIAN_POINT('Ctrl Pts',(2.56668739663161,0.280411490422355,-3.9229910012692));
#88303=CARTESIAN_POINT('Ctrl Pts',(2.56509279648233,0.249136016790644,-3.9252265409816));
#88304=CARTESIAN_POINT('Ctrl Pts',(2.56349819633306,0.217847295216401,-3.92708708476973));
#88305=CARTESIAN_POINT('Ctrl Pts',(2.56190359618379,0.186555007060496,-3.9285730525651));
#88306=CARTESIAN_POINT('Ctrl Pts',(2.55603109559877,0.0713135902165479,
-3.93404548824221));
#88307=CARTESIAN_POINT('Ctrl Pts',(2.55015859501375,-0.0443617374728357,
-3.93445201940534));
#88308=CARTESIAN_POINT('Ctrl Pts',(2.54428609442874,-0.159988279027446,
-3.92974461645714));
#88309=CARTESIAN_POINT('Ctrl Pts',(2.5384212006791,-0.275465045872865,-3.92504331115656));
#88310=CARTESIAN_POINT('Ctrl Pts',(2.53255630692948,-0.390892743054991,
-3.91524126166845));
#88311=CARTESIAN_POINT('Ctrl Pts',(2.52669141317984,-0.505785281191382,
-3.90034232463385));
#88312=CARTESIAN_POINT('Ctrl Pts',(2.52083254796891,-0.620559721005375,
-3.88545870225325));
#88313=CARTESIAN_POINT('Ctrl Pts',(2.51497368275798,-0.734799688480384,
-3.86548866603212));
#88314=CARTESIAN_POINT('Ctrl Pts',(2.50911481754705,-0.848021502043583,
-3.84048805909766));
#88315=CARTESIAN_POINT('Ctrl Pts',(2.50302904920943,-0.965628189226883,
-3.81451922441289));
#88316=CARTESIAN_POINT('Ctrl Pts',(2.49694328087181,-1.08213581160459,-3.78312230989147));
#88317=CARTESIAN_POINT('Ctrl Pts',(2.49085751253419,-1.1970104796669,-3.74641894501504));
#88318=CARTESIAN_POINT('Ctrl Pts',(2.48500542699977,-1.30747416246644,-3.7111249248122));
#88319=CARTESIAN_POINT('Ctrl Pts',(2.47915334146535,-1.41642755348199,-3.67092459374291));
#88320=CARTESIAN_POINT('Ctrl Pts',(2.47330125593093,-1.52340951961511,-3.62597744553742));
#88321=CARTESIAN_POINT('Ctrl Pts',(2.46745006005592,-1.63037522188609,-3.58103713039219));
#88322=CARTESIAN_POINT('Ctrl Pts',(2.46159886418091,-1.73536971420839,-3.53135159301352));
#88323=CARTESIAN_POINT('Ctrl Pts',(2.4557476683059,-1.83795135695881,-3.47712867312288));
#88324=CARTESIAN_POINT('Ctrl Pts',(2.4498959452606,-1.94054224192142,-3.42290086795532));
#88325=CARTESIAN_POINT('Ctrl Pts',(2.4440442222153,-2.04071947970455,-3.36413506079299));
#88326=CARTESIAN_POINT('Ctrl Pts',(2.43819249917,-2.13806621141756,-3.30108495431344));
#88327=CARTESIAN_POINT('Ctrl Pts',(2.43233883208575,-2.23544528332108,-3.23801390154818));
#88328=CARTESIAN_POINT('Ctrl Pts',(2.4264851650015,-2.32999163259134,-3.17065594387585));
#88329=CARTESIAN_POINT('Ctrl Pts',(2.42063149791725,-2.42131814732685,-3.09930757257579));
#88330=CARTESIAN_POINT('Ctrl Pts',(2.41477117681327,-2.51274847535099,-3.02787809767637));
#88331=CARTESIAN_POINT('Ctrl Pts',(2.4089108557093,-2.60095133753657,-2.95244941004886));
#88332=CARTESIAN_POINT('Ctrl Pts',(2.40305053460533,-2.68557336280993,-2.87335774190506));
#88333=CARTESIAN_POINT('Ctrl Pts',(2.39718626659246,-2.77025238076647,-2.79421280575722));
#88334=CARTESIAN_POINT('Ctrl Pts',(2.3913219985796,-2.85134547116981,-2.71140027139316));
#88335=CARTESIAN_POINT('Ctrl Pts',(2.38545773056673,-2.92853793868478,-2.62529132510734));
#88336=CARTESIAN_POINT('Ctrl Pts',(2.3795848278157,-3.00584406688915,-2.53905558921999));
#88337=CARTESIAN_POINT('Ctrl Pts',(2.37371192506467,-3.07923784846847,-2.44951407278266));
#88338=CARTESIAN_POINT('Ctrl Pts',(2.36783902231364,-3.14844641281899,-2.35706898193651));
#88339=CARTESIAN_POINT('Ctrl Pts',(2.36624480735714,-3.16723326032574,-2.33197451796702));
#88340=CARTESIAN_POINT('Ctrl Pts',(2.36465059240064,-3.18571196968848,-2.30666624977724));
#88341=CARTESIAN_POINT('Ctrl Pts',(2.36305637744414,-3.20387766288088,-2.28115254231122));
#88342=CARTESIAN_POINT('Ctrl Pts',(2.35712726773537,-3.27143843154284,-2.18626347479458));
#88343=CARTESIAN_POINT('Ctrl Pts',(2.3511981580266,-3.33489067772598,-2.0882153493576));
#88344=CARTESIAN_POINT('Ctrl Pts',(2.34526904831783,-3.39392837568789,-1.98739507413613));
#88345=CARTESIAN_POINT('Ctrl Pts',(2.33934793526716,-3.45288644883106,-1.88671077637341));
#88346=CARTESIAN_POINT('Ctrl Pts',(2.33342682221649,-3.5074416140155,-1.78326210911534));
#88347=CARTESIAN_POINT('Ctrl Pts',(2.32750570916582,-3.55732956871809,-1.67746694141017));
#88348=CARTESIAN_POINT('Ctrl Pts',(2.32159124251937,-3.60716152457223,-1.57179052797339));
#88349=CARTESIAN_POINT('Ctrl Pts',(2.31567677587291,-3.65233652121262,-1.46377321579088));
#88350=CARTESIAN_POINT('Ctrl Pts',(2.30976230922646,-3.69263517094391,-1.35385911169075));
#88351=CARTESIAN_POINT('Ctrl Pts',(2.30385383432241,-3.73289299550144,-1.24405635778293));
#88352=CARTESIAN_POINT('Ctrl Pts',(2.29794535941836,-3.76828417076304,-1.1323610144258));
#88353=CARTESIAN_POINT('Ctrl Pts',(2.29203688451431,-3.79863692299823,-1.01923820926933));
#88354=CARTESIAN_POINT('Ctrl Pts',(2.28613199697543,-3.82897124638201,-0.906184087286985));
#88355=CARTESIAN_POINT('Ctrl Pts',(2.28022710943655,-3.85427312892714,-0.791704615900504));
#88356=CARTESIAN_POINT('Ctrl Pts',(2.27432222189767,-3.87442036676633,-0.676280874774886));
#88357=CARTESIAN_POINT('Ctrl Pts',(2.26841882637633,-3.89456251390191,-0.560886298344636));
#88358=CARTESIAN_POINT('Ctrl Pts',(2.26251543085498,-3.9095525322712,-0.444548322261923));
#88359=CARTESIAN_POINT('Ctrl Pts',(2.25661203533364,-3.9193192342614,-0.32775866113442));
#88360=CARTESIAN_POINT('Ctrl Pts',(2.25106253090075,-3.92850045137508,-0.217970194513854));
#88361=CARTESIAN_POINT('Ctrl Pts',(2.24551302646786,-3.93306623672388,-0.107782941556682));
#88362=CARTESIAN_POINT('Ctrl Pts',(2.23996352203497,-3.93299927353876,0.00239046931868954));
#88363=CARTESIAN_POINT('Ctrl Pts',(2.23996202763734,-3.92797747181863,0.00241704723849157));
#88364=CARTESIAN_POINT('Ctrl Pts',(2.21471107132639,-3.93073062284058,0.50308190472603));
#88365=CARTESIAN_POINT('Ctrl Pts',(2.12317770876889,-3.60912558829099,2.31455042910235));
#88366=CARTESIAN_POINT('Ctrl Pts',(1.96536193996485,-0.880790531217901,
4.56748308540991));
#88367=CARTESIAN_POINT('Ctrl Pts',(1.76651472122522,3.36599905195296,3.21069095555329));
#88368=CARTESIAN_POINT('Ctrl Pts',(1.56766750248557,4.52080778991678,-1.09560268340907));
#88369=CARTESIAN_POINT('Ctrl Pts',(1.36882028374592,1.52297741527043,-4.39506475690675));
#88370=CARTESIAN_POINT('Ctrl Pts',(1.1762528813402,-2.73512533544538,-3.68141236753163));
#88371=CARTESIAN_POINT('Ctrl Pts',(1.04996788518101,-3.93019899042183,-1.17946347387552));
#88372=CARTESIAN_POINT('Ctrl Pts',(0.989965295268386,-3.93800215978868,
0.00238238590750563));
#88373=CARTESIAN_POINT('Origin',(-1.72497344927317,0.,0.));
#88374=CARTESIAN_POINT('',(48.9000264684934,-3.22327929659544,-0.000763835567893241));
#88375=CARTESIAN_POINT('Ctrl Pts',(48.4702430335869,1.79020435040156,2.68143717906899));
#88376=CARTESIAN_POINT('Ctrl Pts',(48.4828219278093,1.62211098738932,2.7961192948877));
#88377=CARTESIAN_POINT('Ctrl Pts',(48.5616832282783,0.502078434973499,3.41252236229075));
#88378=CARTESIAN_POINT('Ctrl Pts',(48.7049441319495,-2.11679622861173,3.15040696403668));
#88379=CARTESIAN_POINT('Ctrl Pts',(48.8356261413985,-3.22539994567256,1.0376522699003));
#88380=CARTESIAN_POINT('Ctrl Pts',(48.9000257446008,-3.22793943922082,-0.00075326948836482));
#88381=CARTESIAN_POINT('',(49.2909945592456,1.2393601841108,-2.97491241829753));
#88382=CARTESIAN_POINT('Ctrl Pts',(48.9000265507268,-3.22274990919558,-0.000765035863639074));
#88383=CARTESIAN_POINT('Ctrl Pts',(48.9019090850623,-3.22274271499011,-0.0310709680741342));
#88384=CARTESIAN_POINT('Ctrl Pts',(48.9037916193978,-3.22230804770656,-0.0613722117935458));
#88385=CARTESIAN_POINT('Ctrl Pts',(48.9056741537333,-3.22144623788179,-0.091660781893286));
#88386=CARTESIAN_POINT('Ctrl Pts',(48.9118583995395,-3.21861513743701,-0.191160673651801));
#88387=CARTESIAN_POINT('Ctrl Pts',(48.9180426453456,-3.21116499472643,-0.290701504167739));
#88388=CARTESIAN_POINT('Ctrl Pts',(48.9242268911518,-3.19908700253732,-0.389820359520634));
#88389=CARTESIAN_POINT('Ctrl Pts',(48.9304027454209,-3.18702539923738,-0.488804718352069));
#88390=CARTESIAN_POINT('Ctrl Pts',(48.93657859969,-3.17034848093281,-0.587367814511488));
#88391=CARTESIAN_POINT('Ctrl Pts',(48.9427544539591,-3.14909943357514,-0.685047677141335));
#88392=CARTESIAN_POINT('Ctrl Pts',(48.9489237340616,-3.12787300572422,-0.782623560036202));
#88393=CARTESIAN_POINT('Ctrl Pts',(48.9550930141641,-3.10208421720153,-0.879317658376768));
#88394=CARTESIAN_POINT('Ctrl Pts',(48.9612622942666,-3.07182782715444,-0.974675003690801));
#88395=CARTESIAN_POINT('Ctrl Pts',(48.9674269579693,-3.0415940776085,-1.06996099422378));
#88396=CARTESIAN_POINT('Ctrl Pts',(48.973591621672,-3.00689950462653,-1.16391180970599));
#88397=CARTESIAN_POINT('Ctrl Pts',(48.9797562853747,-2.96788931441195,-1.25608541902984));
#88398=CARTESIAN_POINT('Ctrl Pts',(48.9859185412005,-2.92889436131994,-1.34822302595085));
#88399=CARTESIAN_POINT('Ctrl Pts',(48.9920807970262,-2.88558730919526,-1.43858440828709));
#88400=CARTESIAN_POINT('Ctrl Pts',(48.998243052852,-2.8381620212258,-1.52674618184277));
#88401=CARTESIAN_POINT('Ctrl Pts',(49.0044045333619,-2.79074270015833,-1.61489686315875));
#88402=CARTESIAN_POINT('Ctrl Pts',(49.0105660138719,-2.73920637843116,-1.70084810504075));
#88403=CARTESIAN_POINT('Ctrl Pts',(49.0167274943819,-2.68379307216665,-1.78420074775522));
#88404=CARTESIAN_POINT('Ctrl Pts',(49.0228898310577,-2.62837206596986,-1.86756497270053));
#88405=CARTESIAN_POINT('Ctrl Pts',(49.0290521677335,-2.5690732447375,-1.94832952103033));
#88406=CARTESIAN_POINT('Ctrl Pts',(49.0352145044093,-2.50617962029353,-2.02612469342964));
#88407=CARTESIAN_POINT('Ctrl Pts',(49.0413831875777,-2.44322122270653,-2.10399998583911));
#88408=CARTESIAN_POINT('Ctrl Pts',(49.047551870746,-2.3766609011367,-2.1788994583169));
#88409=CARTESIAN_POINT('Ctrl Pts',(49.0537205539143,-2.30682151610866,-2.25048707068451));
#88410=CARTESIAN_POINT('Ctrl Pts',(49.0598925621146,-2.23694448638683,-2.32211327007212));
#88411=CARTESIAN_POINT('Ctrl Pts',(49.0660645703149,-2.16378518883442,-2.39042375825355));
#88412=CARTESIAN_POINT('Ctrl Pts',(49.0722365785152,-2.08770134427464,-2.45512131260634));
#88413=CARTESIAN_POINT('Ctrl Pts',(49.0784185897541,-2.01149418982764,-2.51992372296603));
#88414=CARTESIAN_POINT('Ctrl Pts',(49.084600600993,-1.93235336273051,-2.58110123805993));
#88415=CARTESIAN_POINT('Ctrl Pts',(49.0907826122319,-1.85066756157063,-2.63839859366439));
#88416=CARTESIAN_POINT('Ctrl Pts',(49.095362198979,-1.79015534346653,-2.68084403742443));
#88417=CARTESIAN_POINT('Ctrl Pts',(49.099941785726,-1.72824714873466,-2.72116104277473));
#88418=CARTESIAN_POINT('Ctrl Pts',(49.104521372473,-1.66510947631706,-2.75926221921352));
#88419=CARTESIAN_POINT('Ctrl Pts',(49.1106420329124,-1.58072538771954,-2.81018479721126));
#88420=CARTESIAN_POINT('Ctrl Pts',(49.1167626933517,-1.49384475876965,-2.85732827472905));
#88421=CARTESIAN_POINT('Ctrl Pts',(49.1228833537911,-1.40484385906841,-2.90043639718884));
#88422=CARTESIAN_POINT('Ctrl Pts',(49.1289958344773,-1.3159619016606,-2.94348690923157));
#88423=CARTESIAN_POINT('Ctrl Pts',(49.1351083151635,-1.22496569788788,-2.98251259017556));
#88424=CARTESIAN_POINT('Ctrl Pts',(49.1412207958498,-1.13225917457918,-3.01730123190928));
#88425=CARTESIAN_POINT('Ctrl Pts',(49.1474613693246,-1.03760989877726,-3.05281890238933));
#88426=CARTESIAN_POINT('Ctrl Pts',(49.1537019427994,-0.941178201573555,
-3.08391968990434));
#88427=CARTESIAN_POINT('Ctrl Pts',(49.1599425162742,-0.843419239519438,
-3.11042787232054));
#88428=CARTESIAN_POINT('Ctrl Pts',(49.1660444940328,-0.747831387769098,
-3.13634733952568));
#88429=CARTESIAN_POINT('Ctrl Pts',(49.1721464717913,-0.650975063991087,
-3.15787595500614));
#88430=CARTESIAN_POINT('Ctrl Pts',(49.1782484495498,-0.553293273769149,
-3.17489907173469));
#88431=CARTESIAN_POINT('Ctrl Pts',(49.1843484520425,-0.455643104031581,
-3.19191667792546));
#88432=CARTESIAN_POINT('Ctrl Pts',(49.1904484545353,-0.357168434074009,
-3.2044316067882));
#88433=CARTESIAN_POINT('Ctrl Pts',(49.1965484570281,-0.258322749635708,
-3.21238025761594));
#88434=CARTESIAN_POINT('Ctrl Pts',(49.2026481837623,-0.159481533645042,
-3.22032854911459));
#88435=CARTESIAN_POINT('Ctrl Pts',(49.2087479104966,-0.0602697775203343,
-3.22371093833049));
#88436=CARTESIAN_POINT('Ctrl Pts',(49.2148476372308,0.0388547353954878,
-3.22251576753898));
#88437=CARTESIAN_POINT('Ctrl Pts',(49.2211932140654,0.141974471787196,-3.22127242526835));
#88438=CARTESIAN_POINT('Ctrl Pts',(49.2275387908999,0.244999266023637,-3.21507473082441));
#88439=CARTESIAN_POINT('Ctrl Pts',(49.2338843677345,0.347416415296945,-3.20396931896706));
#88440=CARTESIAN_POINT('Ctrl Pts',(49.2399921014271,0.445994793531956,-3.19328015706109));
#88441=CARTESIAN_POINT('Ctrl Pts',(49.2460998351197,0.54400982278241,-3.17804471411179));
#88442=CARTESIAN_POINT('Ctrl Pts',(49.2522075688123,0.641013560227601,-3.15835703778157));
#88443=CARTESIAN_POINT('Ctrl Pts',(49.2583193274449,0.738081222237557,-3.13865638745494));
#88444=CARTESIAN_POINT('Ctrl Pts',(49.2644310860774,0.834135838720248,-3.11449777424306));
#88445=CARTESIAN_POINT('Ctrl Pts',(49.27054284471,0.928744167988292,-3.08602524826479));
#88446=CARTESIAN_POINT('Ctrl Pts',(49.2766633536017,1.02348794884321,-3.05751195791772));
#88447=CARTESIAN_POINT('Ctrl Pts',(49.2827838624935,1.11678089806089,-3.02467258443918));
#88448=CARTESIAN_POINT('Ctrl Pts',(49.2889043713853,1.20820971163147,-2.9876992578269));
#88449=CARTESIAN_POINT('Ctrl Pts',(49.289601100672,1.21861752790873,-2.98349039220225));
#88450=CARTESIAN_POINT('Ctrl Pts',(49.2902978299588,1.22900121482326,-2.97922800554118));
#88451=CARTESIAN_POINT('Ctrl Pts',(49.2909945592456,1.2393601841108,-2.97491241829753));
#88452=CARTESIAN_POINT('',(49.291,-2.41015873594064,-2.13945143204257));
#88453=CARTESIAN_POINT('Origin',(49.291,0.,0.));
#88454=CARTESIAN_POINT('',(49.1465717854694,-3.2227472468638,0.00421252083431657));
#88455=CARTESIAN_POINT('Ctrl Pts',(49.1474903455921,-3.22274716839108,0.00427213380650271));
#88456=CARTESIAN_POINT('Ctrl Pts',(49.1650705708236,-3.22309010045641,-0.254423729326887));
#88457=CARTESIAN_POINT('Ctrl Pts',(49.1822124068069,-3.19228378391878,-0.512269410551018));
#88458=CARTESIAN_POINT('Ctrl Pts',(49.1994094148614,-3.12714433700966,-0.779323094869068));
#88459=CARTESIAN_POINT('Ctrl Pts',(49.2004120277926,-3.12321643923212,-0.794918409833965));
#88460=CARTESIAN_POINT('Ctrl Pts',(49.2020467655877,-3.11659923137243,-0.820384935923119));
#88461=CARTESIAN_POINT('Ctrl Pts',(49.2026809294181,-3.11397939742035,-0.830273766931297));
#88462=CARTESIAN_POINT('Ctrl Pts',(49.2039110190088,-3.10879509514848,-0.849472700089948));
#88463=CARTESIAN_POINT('Ctrl Pts',(49.2045070891921,-3.10623578217984,-0.858784070798633));
#88464=CARTESIAN_POINT('Ctrl Pts',(49.2055926166077,-3.10148899624475,-0.875755114408501));
#88465=CARTESIAN_POINT('Ctrl Pts',(49.2060824606648,-3.09931490863572,-0.883418424629367));
#88466=CARTESIAN_POINT('Ctrl Pts',(49.2071415003678,-3.09454510556339,-0.899996870650155));
#88467=CARTESIAN_POINT('Ctrl Pts',(49.2077103950552,-3.09193922404829,-0.908909024532861));
#88468=CARTESIAN_POINT('Ctrl Pts',(49.2092569826489,-3.08473624647955,-0.933153829996632));
#88469=CARTESIAN_POINT('Ctrl Pts',(49.2102324709514,-3.08006334185425,-0.948463812509861));
#88470=CARTESIAN_POINT('Ctrl Pts',(49.2150163898034,-3.05651090350066,-1.02361932162588));
#88471=CARTESIAN_POINT('Ctrl Pts',(49.2187774945533,-3.03599960184945,-1.08294160467731));
#88472=CARTESIAN_POINT('Ctrl Pts',(49.2329378837279,-2.95137927520276,-1.30632930034826));
#88473=CARTESIAN_POINT('Ctrl Pts',(49.2430150479392,-2.87559309043842,-1.46564180250813));
#88474=CARTESIAN_POINT('Ctrl Pts',(49.2635841370677,-2.69537914954554,-1.77608354902012));
#88475=CARTESIAN_POINT('Ctrl Pts',(49.2740464936761,-2.59031496761603,-1.92608320209543));
#88476=CARTESIAN_POINT('Ctrl Pts',(49.2862759598952,-2.4607104270521,-2.08120065731826));
#88477=CARTESIAN_POINT('Ctrl Pts',(49.2874531705541,-2.44817050077093,-2.09593729593858));
#88478=CARTESIAN_POINT('Ctrl Pts',(49.2890902648496,-2.43065694474039,-2.1161472168388));
#88479=CARTESIAN_POINT('Ctrl Pts',(49.2895439284707,-2.42579581533941,-2.12171790930695));
#88480=CARTESIAN_POINT('Ctrl Pts',(49.2901723486313,-2.4190520374575,-2.12939258317444));
#88481=CARTESIAN_POINT('Ctrl Pts',(49.2903461654365,-2.41718569210517,-2.13151093428477));
#88482=CARTESIAN_POINT('Ctrl Pts',(49.29067995891,-2.41359963194504,-2.13557044011824));
#88483=CARTESIAN_POINT('Ctrl Pts',(49.2908399100741,-2.41188035194401,-2.13751197794312));
#88484=CARTESIAN_POINT('Ctrl Pts',(49.291,-2.4101587359407,-2.1394514320425));
#88485=CARTESIAN_POINT('Ctrl Pts',(48.7170675950372,1.78943621037805,2.68030513402632));
#88486=CARTESIAN_POINT('Ctrl Pts',(48.7232382856736,1.70649272707747,2.73568019955477));
#88487=CARTESIAN_POINT('Ctrl Pts',(48.72940897631,1.62086774339839,2.78727412820618));
#88488=CARTESIAN_POINT('Ctrl Pts',(48.7355796669464,1.53294127050646,2.83482073924931));
#88489=CARTESIAN_POINT('Ctrl Pts',(48.7417443526567,1.44510036210128,2.88232108093538));
#88490=CARTESIAN_POINT('Ctrl Pts',(48.7479090383669,1.35496279683326,2.92578173148518));
#88491=CARTESIAN_POINT('Ctrl Pts',(48.7540737240772,1.26293658646254,2.96498039472007));
#88492=CARTESIAN_POINT('Ctrl Pts',(48.7602345908057,1.17096738571528,3.00415477464455));
#88493=CARTESIAN_POINT('Ctrl Pts',(48.7663954575343,1.0771122630716,3.0390722466243));
#88494=CARTESIAN_POINT('Ctrl Pts',(48.7725563242629,0.981802016714291,3.06955735611436));
#88495=CARTESIAN_POINT('Ctrl Pts',(48.7787153068185,0.886520919013163,3.10003314236783));
#88496=CARTESIAN_POINT('Ctrl Pts',(48.7848742893742,0.789785994042781,3.12607912820188));
#88497=CARTESIAN_POINT('Ctrl Pts',(48.7910332719298,0.692045250913403,3.1475690513773));
#88498=CARTESIAN_POINT('Ctrl Pts',(48.7971920049047,0.594308468537029,3.1690581037155));
#88499=CARTESIAN_POINT('Ctrl Pts',(48.8033507378796,0.495566372007346,3.18599136788259));
#88500=CARTESIAN_POINT('Ctrl Pts',(48.8095094708544,0.396278299924899,3.19829346238094));
#88501=CARTESIAN_POINT('Ctrl Pts',(48.8156695881842,0.296967909951592,3.21059832213393));
#88502=CARTESIAN_POINT('Ctrl Pts',(48.821829705514,0.197111730224007,3.21826989073169));
#88503=CARTESIAN_POINT('Ctrl Pts',(48.8279898228438,0.0971743868641642,
3.22128463520962));
#88504=CARTESIAN_POINT('Ctrl Pts',(48.8341567551182,-0.00287351728887686,
3.22430271490269));
#88505=CARTESIAN_POINT('Ctrl Pts',(48.8403236873926,-0.103002330928318,
3.22265367266331));
#88506=CARTESIAN_POINT('Ctrl Pts',(48.846490619667,-0.202747397780817,3.21636612579991));
#88507=CARTESIAN_POINT('Ctrl Pts',(48.8526613491965,-0.302553882116546,
3.21007470741367));
#88508=CARTESIAN_POINT('Ctrl Pts',(48.8588320787259,-0.40197571916703,3.19913914457342));
#88509=CARTESIAN_POINT('Ctrl Pts',(48.8650028082554,-0.500555384876538,
3.18363972037841));
#88510=CARTESIAN_POINT('Ctrl Pts',(48.8711834038326,-0.599292664314238,
3.16811551498725));
#88511=CARTESIAN_POINT('Ctrl Pts',(48.8773639994097,-0.697184660345036,
3.14801296595449));
#88512=CARTESIAN_POINT('Ctrl Pts',(48.8835445949869,-0.793786020148058,
3.12346303271185));
#88513=CARTESIAN_POINT('Ctrl Pts',(48.8867982508315,-0.844639950807991,
3.11053919183246));
#88514=CARTESIAN_POINT('Ctrl Pts',(48.8900519066761,-0.895136486724309,
3.09638367876077));
#88515=CARTESIAN_POINT('Ctrl Pts',(48.8933055625207,-0.945212836742466,
3.0810209761956));
#88516=CARTESIAN_POINT('Ctrl Pts',(48.8994111530019,-1.03918272802978,3.05219236769266));
#88517=CARTESIAN_POINT('Ctrl Pts',(48.9055167434831,-1.13201835900593,3.01900355677363));
#88518=CARTESIAN_POINT('Ctrl Pts',(48.9116223339642,-1.22327913816598,2.98156095235833));
#88519=CARTESIAN_POINT('Ctrl Pts',(48.9177195243747,-1.31441436075667,2.94416986147383));
#88520=CARTESIAN_POINT('Ctrl Pts',(48.9238167147852,-1.40397862858924,2.9025367696119));
#88521=CARTESIAN_POINT('Ctrl Pts',(48.9299139051958,-1.4915453703454,2.85681815499363));
#88522=CARTESIAN_POINT('Ctrl Pts',(48.9360046026441,-1.579018861358,2.81114822660854));
#88523=CARTESIAN_POINT('Ctrl Pts',(48.9420953000925,-1.66449866145113,2.7614016246746));
#88524=CARTESIAN_POINT('Ctrl Pts',(48.9481859975408,-1.74757812433479,2.70778290522828));
#88525=CARTESIAN_POINT('Ctrl Pts',(48.9542724982055,-1.83060034147023,2.65420113166013));
#88526=CARTESIAN_POINT('Ctrl Pts',(48.9603589988702,-1.91122513459973,2.59675278074639));
#88527=CARTESIAN_POINT('Ctrl Pts',(48.9664454995349,-1.9890713277967,2.5356878387209));
#88528=CARTESIAN_POINT('Ctrl Pts',(48.9725298594353,-2.06689014067044,2.4746443746609));
#88529=CARTESIAN_POINT('Ctrl Pts',(48.9786142193356,-2.14193194468348,2.40998711920826));
#88530=CARTESIAN_POINT('Ctrl Pts',(48.9846985792359,-2.21384626928613,2.34200816789095));
#88531=CARTESIAN_POINT('Ctrl Pts',(48.9907825096814,-2.28575551793002,2.2740340147603));
#88532=CARTESIAN_POINT('Ctrl Pts',(48.9968664401268,-2.35453740258873,2.20273893687918));
#88533=CARTESIAN_POINT('Ctrl Pts',(49.0029503705722,-2.41987700851893,2.12845315338193));
#88534=CARTESIAN_POINT('Ctrl Pts',(49.0090355821478,-2.48523037340599,2.05415172707698));
#88535=CARTESIAN_POINT('Ctrl Pts',(49.0151207937233,-2.54713972663897,1.97685867842956));
#88536=CARTESIAN_POINT('Ctrl Pts',(49.0212060052988,-2.60533002987135,1.89693779496075));
#88537=CARTESIAN_POINT('Ctrl Pts',(49.0272986882685,-2.66359177888423,1.81691878500727));
#88538=CARTESIAN_POINT('Ctrl Pts',(49.0333913712382,-2.71812509887946,1.73426585845953));
#88539=CARTESIAN_POINT('Ctrl Pts',(49.0394840542079,-2.76869805694995,1.64937219327281));
#88540=CARTESIAN_POINT('Ctrl Pts',(49.0455805507553,-2.81930267002543,1.56442539080686));
#88541=CARTESIAN_POINT('Ctrl Pts',(49.0516770473028,-2.86594177980861,1.47723545091154));
#88542=CARTESIAN_POINT('Ctrl Pts',(49.0577735438503,-2.90843033892423,1.38821847204433));
#88543=CARTESIAN_POINT('Ctrl Pts',(49.0638816534136,-2.95099983309956,1.29903192765996));
#88544=CARTESIAN_POINT('Ctrl Pts',(49.069989762977,-2.98940281426851,1.20801180324768));
#88545=CARTESIAN_POINT('Ctrl Pts',(49.0760978725403,-3.02350306175496,1.11559257709002));
#88546=CARTESIAN_POINT('Ctrl Pts',(49.0814495087804,-3.05338008317195,1.03461922930564));
#88547=CARTESIAN_POINT('Ctrl Pts',(49.0868011450204,-3.07995486263722,0.952572294301333));
#88548=CARTESIAN_POINT('Ctrl Pts',(49.0921527812604,-3.10316810876065,0.869750108520173));
#88549=CARTESIAN_POINT('Ctrl Pts',(49.100662198562,-3.14007853939013,0.738057947647774));
#88550=CARTESIAN_POINT('Ctrl Pts',(49.1091716158637,-3.1686037383271,0.604007833156265));
#88551=CARTESIAN_POINT('Ctrl Pts',(49.1176810331654,-3.18851392237117,0.468504567048382));
#88552=CARTESIAN_POINT('Ctrl Pts',(49.1259255518801,-3.2078043013882,0.337219524404909));
#88553=CARTESIAN_POINT('Ctrl Pts',(49.1341700705947,-3.21900782770081,0.204569851518107));
#88554=CARTESIAN_POINT('Ctrl Pts',(49.1424145893094,-3.22195894791002,0.0714009837645678));
#88555=CARTESIAN_POINT('Ctrl Pts',(49.1438003213627,-3.22245496981362,0.0490180679220658));
#88556=CARTESIAN_POINT('Ctrl Pts',(49.1451860534161,-3.22271795685899,0.0266205482591167));
#88557=CARTESIAN_POINT('Ctrl Pts',(49.1465717854694,-3.2227472468638,0.00421252083431657));
#88558=CARTESIAN_POINT('Origin',(0.,0.,0.));
#88559=CARTESIAN_POINT('',(0.,-1.2491397351303E-16,1.02));
#88560=CARTESIAN_POINT('Origin',(0.,0.,0.));
#88561=CARTESIAN_POINT('',(2.448,-1.2491397351303E-16,1.02));
#88562=CARTESIAN_POINT('',(0.,-1.2491397351303E-16,1.02));
#88563=CARTESIAN_POINT('Origin',(2.448,0.,0.));
#88564=CARTESIAN_POINT('Origin',(2.448,0.,0.));
#88565=CARTESIAN_POINT('Origin',(49.291,5.160062080289E-16,2.1385152528819E-16));
#88566=CARTESIAN_POINT('',(49.291,-0.996446678860641,3.80467909503385));
#88567=CARTESIAN_POINT('',(49.291,-3.933,4.81653586104654E-16));
#88568=CARTESIAN_POINT('Origin',(49.291,0.,0.));
#88569=CARTESIAN_POINT('Ctrl Pts',(49.2910000000001,-0.996446678860644,
3.80467909503386));
#88570=CARTESIAN_POINT('Ctrl Pts',(49.2910000000001,-1.04787446395986,3.78642472561806));
#88571=CARTESIAN_POINT('Ctrl Pts',(49.2910000000001,-1.09885704840169,3.76701980464874));
#88572=CARTESIAN_POINT('Ctrl Pts',(49.2910000000001,-1.14935789175992,3.74645332354063));
#88573=CARTESIAN_POINT('Ctrl Pts',(49.2910000000001,-1.26368142516242,3.69989503592438));
#88574=CARTESIAN_POINT('Ctrl Pts',(49.2910000000001,-1.37553846253051,3.64738695884623));
#88575=CARTESIAN_POINT('Ctrl Pts',(49.2910000000001,-1.48464424221647,3.58930502949026));
#88576=CARTESIAN_POINT('Ctrl Pts',(49.2910000000001,-1.59375002190243,3.53122310013429));
#88577=CARTESIAN_POINT('Ctrl Pts',(49.2910000000001,-1.70010512777846,3.46756648039375));
#88578=CARTESIAN_POINT('Ctrl Pts',(49.2910000000001,-1.80338619496161,3.3986729028763));
#88579=CARTESIAN_POINT('Ctrl Pts',(49.2910000000001,-1.82145558081485,3.38661972925091));
#88580=CARTESIAN_POINT('Ctrl Pts',(49.2910000000001,-1.83943154385614,3.3744055478693));
#88581=CARTESIAN_POINT('Ctrl Pts',(49.2910000000001,-1.85729837010941,3.36204194363082));
#88582=CARTESIAN_POINT('Ctrl Pts',(49.2910000000001,-1.95673406302392,3.29323377720289));
#88583=CARTESIAN_POINT('Ctrl Pts',(49.2910000000001,-2.05289507009515,3.21973309797708));
#88584=CARTESIAN_POINT('Ctrl Pts',(49.2910000000001,-2.14551174396067,3.14189100840979));
#88585=CARTESIAN_POINT('Ctrl Pts',(49.2910000000001,-2.23824482167426,3.06395108420442));
#88586=CARTESIAN_POINT('Ctrl Pts',(49.2910000000001,-2.32742518903523,2.98165804209933));
#88587=CARTESIAN_POINT('Ctrl Pts',(49.2910000000001,-2.41274059201778,2.89533360211057));
#88588=CARTESIAN_POINT('Ctrl Pts',(49.2910000000001,-2.43810143532588,2.8696728126203));
#88589=CARTESIAN_POINT('Ctrl Pts',(49.2910000000001,-2.46312044856481,2.84365563256905));
#88590=CARTESIAN_POINT('Ctrl Pts',(49.2910000000001,-2.4877886142742,2.81729014790106));
#88591=CARTESIAN_POINT('Ctrl Pts',(49.2910000000001,-2.50844926697038,2.79520791737331));
#88592=CARTESIAN_POINT('Ctrl Pts',(49.2910000000001,-2.52886359911005,2.77288158200795));
#88593=CARTESIAN_POINT('Ctrl Pts',(49.2910000000001,-2.54902671268354,2.75031513412511));
#88594=CARTESIAN_POINT('Ctrl Pts',(49.2910000000001,-2.56454011453025,2.73295261851046));
#88595=CARTESIAN_POINT('Ctrl Pts',(49.291,-2.57990529901037,2.71544717523286));
#88596=CARTESIAN_POINT('Ctrl Pts',(49.291,-2.59510362438686,2.69782010081254));
#88597=CARTESIAN_POINT('Ctrl Pts',(49.2910000000001,-2.67265098507086,2.60788038284924));
#88598=CARTESIAN_POINT('Ctrl Pts',(49.291,-2.74595669984527,2.51466762988873));
#88599=CARTESIAN_POINT('Ctrl Pts',(49.291,-2.81476512078422,2.41850780437463));
#88600=CARTESIAN_POINT('Ctrl Pts',(49.291,-2.88294028953555,2.3232329493196));
#88601=CARTESIAN_POINT('Ctrl Pts',(49.291,-2.94670096158189,2.2250642295418));
#88602=CARTESIAN_POINT('Ctrl Pts',(49.291,-3.0057531650948,2.12429641591241));
#88603=CARTESIAN_POINT('Ctrl Pts',(49.291,-3.06309302084408,2.02645058537676));
#88604=CARTESIAN_POINT('Ctrl Pts',(49.291,-3.11599369344923,1.92615350792922));
#88605=CARTESIAN_POINT('Ctrl Pts',(49.291,-3.16413915873218,1.82366487194788));
#88606=CARTESIAN_POINT('Ctrl Pts',(49.291,-3.21154220550962,1.72275664358147));
#88607=CARTESIAN_POINT('Ctrl Pts',(49.291,-3.25433581187686,1.61972334371028));
#88608=CARTESIAN_POINT('Ctrl Pts',(49.291,-3.29216896681703,1.51481212425853));
#88609=CARTESIAN_POINT('Ctrl Pts',(49.291,-3.2971950076517,1.50087492885909));
#88610=CARTESIAN_POINT('Ctrl Pts',(49.291,-3.30213229857781,1.48690762923938));
#88611=CARTESIAN_POINT('Ctrl Pts',(49.291,-3.30697750441129,1.47291855471233));
#88612=CARTESIAN_POINT('Ctrl Pts',(49.291,-3.3435823316148,1.36723312598158));
#88613=CARTESIAN_POINT('Ctrl Pts',(49.291,-3.37498240661714,1.26017600349772));
#88614=CARTESIAN_POINT('Ctrl Pts',(49.291,-3.4009150635724,1.15201104588828));
#88615=CARTESIAN_POINT('Ctrl Pts',(49.291,-3.41583937901282,1.08976181513079));
#88616=CARTESIAN_POINT('Ctrl Pts',(49.291,-3.42895196485492,1.02714544974631));
#88617=CARTESIAN_POINT('Ctrl Pts',(49.291,-3.44019492225294,0.964211348562105));
#88618=CARTESIAN_POINT('Ctrl Pts',(49.291,-3.46010351309487,0.852770094617592));
#88619=CARTESIAN_POINT('Ctrl Pts',(49.291,-3.47415249335439,0.740331870820918));
#88620=CARTESIAN_POINT('Ctrl Pts',(49.291,-3.48247133759665,0.627292733384211));
#88621=CARTESIAN_POINT('Ctrl Pts',(49.291,-3.48859838156326,0.544036484697046));
#88622=CARTESIAN_POINT('Ctrl Pts',(49.291,-3.4916158426533,0.460454247766092));
#88623=CARTESIAN_POINT('Ctrl Pts',(49.291,-3.49155833914504,0.376709317963282));
#88624=CARTESIAN_POINT('Ctrl Pts',(49.291,-3.49152958739091,0.334836853061878));
#88625=CARTESIAN_POINT('Ctrl Pts',(49.291,-3.49073187737215,0.292923804538428));
#88626=CARTESIAN_POINT('Ctrl Pts',(49.291,-3.48916828433049,0.250991241296264));
#88627=CARTESIAN_POINT('Ctrl Pts',(49.291,-3.48819573164138,0.224909245498223));
#88628=CARTESIAN_POINT('Ctrl Pts',(49.291,-3.48692685474254,0.198819676470504));
#88629=CARTESIAN_POINT('Ctrl Pts',(49.291,-3.48536224038303,0.17272774885287));
#88630=CARTESIAN_POINT('Ctrl Pts',(49.291,-3.48441139192721,0.156871145636885));
#88631=CARTESIAN_POINT('Ctrl Pts',(49.291,-3.48335133632153,0.141014949767345));
#88632=CARTESIAN_POINT('Ctrl Pts',(49.291,-3.48218335319603,0.125173095621732));
#88633=CARTESIAN_POINT('Ctrl Pts',(49.291,-3.47400097567051,0.014192013366608));
#88634=CARTESIAN_POINT('Ctrl Pts',(49.291,-3.4605166069301,-0.0962534958503473));
#88635=CARTESIAN_POINT('Ctrl Pts',(49.291,-3.44188652183421,-0.205793275630291));
#88636=CARTESIAN_POINT('Ctrl Pts',(49.291,-3.42320843589755,-0.315615287160677));
#88637=CARTESIAN_POINT('Ctrl Pts',(49.291,-3.39935769259813,-0.424527765102663));
#88638=CARTESIAN_POINT('Ctrl Pts',(49.291,-3.37044206707646,-0.532141159658396));
#88639=CARTESIAN_POINT('Ctrl Pts',(49.291,-3.34195964367767,-0.638142334172885));
#88640=CARTESIAN_POINT('Ctrl Pts',(49.291,-3.30856248028982,-0.742883787691385));
#88641=CARTESIAN_POINT('Ctrl Pts',(49.291,-3.2703120890578,-0.84596544270122));
#88642=CARTESIAN_POINT('Ctrl Pts',(49.291,-3.24749664417666,-0.907451188137614));
#88643=CARTESIAN_POINT('Ctrl Pts',(49.291,-3.22295374005823,-0.968345820777564));
#88644=CARTESIAN_POINT('Ctrl Pts',(49.291,-3.19669027020856,-1.02855802508857));
#88645=CARTESIAN_POINT('Ctrl Pts',(49.291,-3.18377971124691,-1.05815705440256));
#88646=CARTESIAN_POINT('Ctrl Pts',(49.291,-3.17045331195658,-1.0875910939131));
#88647=CARTESIAN_POINT('Ctrl Pts',(49.291,-3.15671152110727,-1.11684879068458));
#88648=CARTESIAN_POINT('Ctrl Pts',(49.291,-3.15009342463488,-1.13093940390357));
#88649=CARTESIAN_POINT('Ctrl Pts',(49.291,-3.14338306198869,-1.1449803992522));
#88650=CARTESIAN_POINT('Ctrl Pts',(49.291,-3.13658146830333,-1.15896934835303));
#88651=CARTESIAN_POINT('Ctrl Pts',(49.291,-3.08957842437905,-1.25564127841209));
#88652=CARTESIAN_POINT('Ctrl Pts',(49.291,-3.03821155674967,-1.34985216107223));
#88653=CARTESIAN_POINT('Ctrl Pts',(49.291,-2.98257948506975,-1.44125037056837));
#88654=CARTESIAN_POINT('Ctrl Pts',(49.291,-2.92773294523813,-1.53135802585232));
#88655=CARTESIAN_POINT('Ctrl Pts',(49.291,-2.86874034172397,-1.61873250557023));
#88656=CARTESIAN_POINT('Ctrl Pts',(49.291,-2.80565945595285,-1.70300335032673));
#88657=CARTESIAN_POINT('Ctrl Pts',(49.291,-2.74451889583004,-1.78468208053875));
#88658=CARTESIAN_POINT('Ctrl Pts',(49.291,-2.67953722771974,-1.86344557020302));
#88659=CARTESIAN_POINT('Ctrl Pts',(49.291,-2.61073916422542,-1.9389175189001));
#88660=CARTESIAN_POINT('Ctrl Pts',(49.291,-2.54714019487492,-2.00868602557333));
#88661=CARTESIAN_POINT('Ctrl Pts',(49.291,-2.48027938346939,-2.07564162707797));
#88662=CARTESIAN_POINT('Ctrl Pts',(49.291,-2.41015873594071,-2.1394514320425));
#88663=CARTESIAN_POINT('Ctrl Pts',(49.2909999999999,1.24155974343475,-2.97996389319987));
#88664=CARTESIAN_POINT('Ctrl Pts',(49.2909999999999,1.30609747649074,-2.96119741864278));
#88665=CARTESIAN_POINT('Ctrl Pts',(49.2909999999999,1.36990375724753,-2.94029757439427));
#88666=CARTESIAN_POINT('Ctrl Pts',(49.2909999999999,1.43287202055253,-2.91725941417401));
#88667=CARTESIAN_POINT('Ctrl Pts',(49.2909999999999,1.52953857307307,-2.8818920813619));
#88668=CARTESIAN_POINT('Ctrl Pts',(49.2909999999999,1.62423083505432,-2.84148829030612));
#88669=CARTESIAN_POINT('Ctrl Pts',(49.291,1.71676866792147,-2.7964134037744));
#88670=CARTESIAN_POINT('Ctrl Pts',(49.291,1.77471818041898,-2.76818637900559));
#88671=CARTESIAN_POINT('Ctrl Pts',(49.2909999999999,1.83182274814194,-2.7381264400551));
#88672=CARTESIAN_POINT('Ctrl Pts',(49.2909999999999,1.88803631231024,-2.70631314436809));
#88673=CARTESIAN_POINT('Ctrl Pts',(49.2909999999999,1.92428874636053,-2.68579657650977));
#88674=CARTESIAN_POINT('Ctrl Pts',(49.291,1.96017057617847,-2.66455062778348));
#88675=CARTESIAN_POINT('Ctrl Pts',(49.291,1.99566895445841,-2.64259506607457));
#88676=CARTESIAN_POINT('Ctrl Pts',(49.291,2.01164126184652,-2.63271627731052));
#88677=CARTESIAN_POINT('Ctrl Pts',(49.291,2.02753526337067,-2.62269413617559));
#88678=CARTESIAN_POINT('Ctrl Pts',(49.291,2.043338740134,-2.61253776460566));
#88679=CARTESIAN_POINT('Ctrl Pts',(49.291,2.13272190540694,-2.55509416202361));
#88680=CARTESIAN_POINT('Ctrl Pts',(49.291,2.21930400701889,-2.49330331451299));
#88681=CARTESIAN_POINT('Ctrl Pts',(49.291,2.30289476104567,-2.42754176486054));
#88682=CARTESIAN_POINT('Ctrl Pts',(49.291,2.3885789038207,-2.36013332866288));
#88683=CARTESIAN_POINT('Ctrl Pts',(49.291,2.4711206813037,-2.28855247169546));
#88684=CARTESIAN_POINT('Ctrl Pts',(49.291,2.55029884082011,-2.21315276753045));
#88685=CARTESIAN_POINT('Ctrl Pts',(49.291,2.57674354345376,-2.18797003068122));
#88686=CARTESIAN_POINT('Ctrl Pts',(49.291,2.60281285880127,-2.16236090782209));
#88687=CARTESIAN_POINT('Ctrl Pts',(49.291,2.62849794204176,-2.13633743752041));
#88688=CARTESIAN_POINT('Ctrl Pts',(49.291,2.64321859230724,-2.12142285066009));
#88689=CARTESIAN_POINT('Ctrl Pts',(49.291,2.65781302871306,-2.1063721544104));
#88690=CARTESIAN_POINT('Ctrl Pts',(49.291,2.67227953262755,-2.09118753901551));
#88691=CARTESIAN_POINT('Ctrl Pts',(49.291,2.68411484151633,-2.07876473011725));
#88692=CARTESIAN_POINT('Ctrl Pts',(49.291,2.6958637113429,-2.06625304941116));
#88693=CARTESIAN_POINT('Ctrl Pts',(49.291,2.70751679354967,-2.05366306839897));
#88694=CARTESIAN_POINT('Ctrl Pts',(49.291,2.78348489802944,-1.97158718701738));
#88695=CARTESIAN_POINT('Ctrl Pts',(49.291,2.85548187030216,-1.88608530691149));
#88696=CARTESIAN_POINT('Ctrl Pts',(49.291,2.92330271970775,-1.79755683447092));
#88697=CARTESIAN_POINT('Ctrl Pts',(49.291,2.99192600729937,-1.70798091677628));
#88698=CARTESIAN_POINT('Ctrl Pts',(49.291,3.05627448257204,-1.61530580669057));
#88699=CARTESIAN_POINT('Ctrl Pts',(49.291,3.11611202188338,-1.51989684308203));
#88700=CARTESIAN_POINT('Ctrl Pts',(49.291,3.17581269028068,-1.4247061155876));
#88701=CARTESIAN_POINT('Ctrl Pts',(49.291,3.23102371579603,-1.32679334572647));
#88702=CARTESIAN_POINT('Ctrl Pts',(49.291,3.28147664994958,-1.22648294339381));
#88703=CARTESIAN_POINT('Ctrl Pts',(49.291,3.31382283080201,-1.16217234442335));
#88704=CARTESIAN_POINT('Ctrl Pts',(49.291,3.34421258369244,-1.09687550021422));
#88705=CARTESIAN_POINT('Ctrl Pts',(49.291,3.37256580457531,-1.03067154124884));
#88706=CARTESIAN_POINT('Ctrl Pts',(49.291,3.38259777691676,-1.00724717306227));
#88707=CARTESIAN_POINT('Ctrl Pts',(49.291,3.39237472274341,-0.983709205287762));
#88708=CARTESIAN_POINT('Ctrl Pts',(49.291,3.40189284016588,-0.960061026530207));
#88709=CARTESIAN_POINT('Ctrl Pts',(49.291,3.40733925000965,-0.94652918321965));
#88710=CARTESIAN_POINT('Ctrl Pts',(49.291,3.41269973962293,-0.932964063311978));
#88711=CARTESIAN_POINT('Ctrl Pts',(49.291,3.41797075710576,-0.919374174560089));
#88712=CARTESIAN_POINT('Ctrl Pts',(49.291,3.45985945406193,-0.811375532276965));
#88713=CARTESIAN_POINT('Ctrl Pts',(49.291,3.49615814443692,-0.701673043089189));
#88714=CARTESIAN_POINT('Ctrl Pts',(49.291,3.526628671481,-0.590647306950014));
#88715=CARTESIAN_POINT('Ctrl Pts',(49.291,3.54303568422161,-0.530864925610285));
#88716=CARTESIAN_POINT('Ctrl Pts',(49.291,3.55775234160509,-0.470698196068018));
#88717=CARTESIAN_POINT('Ctrl Pts',(49.291,3.57073680375558,-0.410202350230981));
#88718=CARTESIAN_POINT('Ctrl Pts',(49.291,3.59424040049109,-0.300696854489483));
#88719=CARTESIAN_POINT('Ctrl Pts',(49.2910000000001,3.61207160669811,-0.190114079831296));
#88720=CARTESIAN_POINT('Ctrl Pts',(49.2910000000001,3.62443023878303,-0.0788005633581947));
#88721=CARTESIAN_POINT('Ctrl Pts',(49.2910000000001,3.63678887086796,0.0325129531149071));
#88722=CARTESIAN_POINT('Ctrl Pts',(49.291,3.6436748240379,0.144557927003784));
#88723=CARTESIAN_POINT('Ctrl Pts',(49.291,3.64523740891943,0.257002790496591));
#88724=CARTESIAN_POINT('Ctrl Pts',(49.291,3.64573156500446,0.292562659392238));
#88725=CARTESIAN_POINT('Ctrl Pts',(49.2910000000001,3.6456929614631,0.32816258953133));
#88726=CARTESIAN_POINT('Ctrl Pts',(49.2910000000001,3.64512529508925,0.363792226448562));
#88727=CARTESIAN_POINT('Ctrl Pts',(49.2910000000001,3.64486222011793,0.380304153421158));
#88728=CARTESIAN_POINT('Ctrl Pts',(49.2910000000001,3.64448543221427,0.396825027320545));
#88729=CARTESIAN_POINT('Ctrl Pts',(49.2910000000001,3.64399552440606,0.413345378021866));
#88730=CARTESIAN_POINT('Ctrl Pts',(49.2910000000001,3.64053542637784,0.530024540776952));
#88731=CARTESIAN_POINT('Ctrl Pts',(49.291,3.63144663106782,0.646416163441864));
#88732=CARTESIAN_POINT('Ctrl Pts',(49.2910000000001,3.61697648681964,0.762139257707719));
#88733=CARTESIAN_POINT('Ctrl Pts',(49.2910000000001,3.60244319778279,0.878367344197995));
#88734=CARTESIAN_POINT('Ctrl Pts',(49.2910000000001,3.58248137580691,0.993921830073509));
#88735=CARTESIAN_POINT('Ctrl Pts',(49.2910000000001,3.55728842902304,1.10843304586257));
#88736=CARTESIAN_POINT('Ctrl Pts',(49.2910000000001,3.53175390717093,1.22449684605884));
#88737=CARTESIAN_POINT('Ctrl Pts',(49.2910000000001,3.50084540844511,1.33948972685971));
#88738=CARTESIAN_POINT('Ctrl Pts',(49.2910000000001,3.46471501177006,1.45303135874471));
#88739=CARTESIAN_POINT('Ctrl Pts',(49.291,3.43001588946358,1.56207513723098));
#88740=CARTESIAN_POINT('Ctrl Pts',(49.291,3.39049995192555,1.66978108778202));
#88741=CARTESIAN_POINT('Ctrl Pts',(49.291,3.34625722541054,1.77580515381087));
#88742=CARTESIAN_POINT('Ctrl Pts',(49.291,3.33687123746234,1.7982979042436));
#88743=CARTESIAN_POINT('Ctrl Pts',(49.291,3.32726976310538,1.82072057743119));
#88744=CARTESIAN_POINT('Ctrl Pts',(49.291,3.31746764588934,1.84303814040658));
#88745=CARTESIAN_POINT('Ctrl Pts',(49.291,3.26814654678819,1.95533293457664));
#88746=CARTESIAN_POINT('Ctrl Pts',(49.291,3.21370135735444,2.06509026310669));
#88747=CARTESIAN_POINT('Ctrl Pts',(49.291,3.15434087104448,2.17191824325322));
#88748=CARTESIAN_POINT('Ctrl Pts',(49.291,3.09490644304957,2.27887929240478));
#88749=CARTESIAN_POINT('Ctrl Pts',(49.291,3.03054427425482,2.38290458632646));
#88750=CARTESIAN_POINT('Ctrl Pts',(49.291,2.96141160421367,2.48359656129828));
#88751=CARTESIAN_POINT('Ctrl Pts',(49.291,2.89240794490613,2.58410063168675));
#88752=CARTESIAN_POINT('Ctrl Pts',(49.291,2.81865136104634,2.68128471430845));
#88753=CARTESIAN_POINT('Ctrl Pts',(49.291,2.74024916152721,2.7747358172889));
#88754=CARTESIAN_POINT('Ctrl Pts',(49.291,2.66184696200807,2.86818692026936));
#88755=CARTESIAN_POINT('Ctrl Pts',(49.291,2.57879895493468,2.95790597872136));
#88756=CARTESIAN_POINT('Ctrl Pts',(49.291,2.49116634986212,3.04344857313454));
#88757=CARTESIAN_POINT('Origin',(49.291,0.,0.));
#88758=CARTESIAN_POINT('Ctrl Pts',(0.173056187199666,-1.43083790675438,
2.88251867495153));
#88759=CARTESIAN_POINT('Ctrl Pts',(0.239338593446214,-2.39121159098777,
2.40580395875854));
#88760=CARTESIAN_POINT('Ctrl Pts',(0.37190340593931,-3.78114133209139,0.425036707075511));
#88761=CARTESIAN_POINT('Ctrl Pts',(0.570750624678953,-2.39953276490048,
-2.95773654621702));
#88762=CARTESIAN_POINT('Ctrl Pts',(0.769597843418598,1.18945394678139,-3.61436653776285));
#88763=CARTESIAN_POINT('Ctrl Pts',(0.968445062158239,3.68418171216641,-0.955516875925982));
#88764=CARTESIAN_POINT('Ctrl Pts',(1.16729228089789,2.79555519642049,2.58343267463272));
#88765=CARTESIAN_POINT('Ctrl Pts',(1.36613949963753,-0.661460018592585,
3.74805170741327));
#88766=CARTESIAN_POINT('Ctrl Pts',(1.56498671837718,-3.51063697999909,1.47043618308769));
#88767=CARTESIAN_POINT('Ctrl Pts',(1.76383393711682,-3.1351373407493,-2.15823110503949));
#88768=CARTESIAN_POINT('Ctrl Pts',(1.96268115585646,0.120299360187439,-3.8042141985468));
#88769=CARTESIAN_POINT('Ctrl Pts',(2.16152837459611,3.26519802508846,-1.95581670897684));
#88770=CARTESIAN_POINT('Ctrl Pts',(2.36037559333575,3.41077016481472,1.68920239984469));
#88771=CARTESIAN_POINT('Ctrl Pts',(2.5592228120754,0.423269523206983,3.78252945499563));
#88772=CARTESIAN_POINT('Ctrl Pts',(2.75807003081503,-2.95303304907864,2.40131564870111));
#88773=CARTESIAN_POINT('Ctrl Pts',(2.95691724955468,-3.6167424373011,-1.18570445582992));
#88774=CARTESIAN_POINT('Ctrl Pts',(3.15576446829432,-0.958184980230354,
-3.68355711222238));
#88775=CARTESIAN_POINT('Ctrl Pts',(3.35461168703397,2.58054089412746,-2.79777152901459));
#88776=CARTESIAN_POINT('Ctrl Pts',(3.55345890577361,3.74883510575342,0.657990674924371));
#88777=CARTESIAN_POINT('Ctrl Pts',(3.75230612451326,1.47352597266888,3.50933560299747));
#88778=CARTESIAN_POINT('Ctrl Pts',(3.95115334325289,-2.15533384583538,3.13707698173024));
#88779=CARTESIAN_POINT('Ctrl Pts',(4.15000056199255,-3.80434818238047,-0.116836453731265));
#88780=CARTESIAN_POINT('Ctrl Pts',(4.34884778073217,-1.95876615891209,-3.26342624165674));
#88781=CARTESIAN_POINT('Ctrl Pts',(4.54769499947184,1.68609833178183,-3.41229955232396));
#88782=CARTESIAN_POINT('Ctrl Pts',(4.74654221821145,3.78214743079572,-0.426704352531632));
#88783=CARTESIAN_POINT('Ctrl Pts',(4.94538943695112,2.40399334842639,2.95085271673614));
#88784=CARTESIAN_POINT('Ctrl Pts',(5.14423665569075,-1.18241979186214,3.61781691467976));
#88785=CARTESIAN_POINT('Ctrl Pts',(5.3430838744304,-3.6826863264606,0.961528579047624));
#88786=CARTESIAN_POINT('Ctrl Pts',(5.54193109317004,-2.80011261657801,-2.57800021721949));
#88787=CARTESIAN_POINT('Ctrl Pts',(5.74077831190969,0.654587200762842,-3.74943080807304));
#88788=CARTESIAN_POINT('Ctrl Pts',(5.93962553064932,3.50799662053473,-1.47671104058992));
#88789=CARTESIAN_POINT('Ctrl Pts',(6.13847274938897,3.13903218278845,2.15248524787444));
#88790=CARTESIAN_POINT('Ctrl Pts',(6.33731996812863,-0.113382935647901,
3.80445266722274));
#88791=CARTESIAN_POINT('Ctrl Pts',(6.53616718686825,-3.26164681132122,1.96172777553185));
#88792=CARTESIAN_POINT('Ctrl Pts',(6.73501440560792,-3.41382871943484,-1.683000077672));
#88793=CARTESIAN_POINT('Ctrl Pts',(6.93386162434754,-0.430137475655535,
-3.78175852470304));
#88794=CARTESIAN_POINT('Ctrl Pts',(7.1327088430872,2.94866924473366,-2.40667103532393));
#88795=CARTESIAN_POINT('Ctrl Pts',(7.33155606182684,3.61888878095798,1.17913518231027));
#88796=CARTESIAN_POINT('Ctrl Pts',(7.53040328056648,0.96487119207266,3.68181196828677));
#88797=CARTESIAN_POINT('Ctrl Pts',(7.72925049930613,-2.57545731482602,2.80245167783803));
#88798=CARTESIAN_POINT('Ctrl Pts',(7.92809771804577,-3.75002347358853,-0.651183334125902));
#88799=CARTESIAN_POINT('Ctrl Pts',(8.12694493678541,-1.47989486401989,-3.50665467055948));
#88800=CARTESIAN_POINT('Ctrl Pts',(8.32579215552506,2.14963486174807,-3.14098483731869));
#88801=CARTESIAN_POINT('Ctrl Pts',(8.5246393742647,3.80455402461192,0.109929345116928));
#88802=CARTESIAN_POINT('Ctrl Pts',(8.72348659300433,1.96468777167325,3.25986468230605));
#88803=CARTESIAN_POINT('Ctrl Pts',(8.92233381174399,-1.67990043464857,3.41535507916472));
#88804=CARTESIAN_POINT('Ctrl Pts',(9.12118103048362,-3.78136650338711,0.433570241334211));
#88805=CARTESIAN_POINT('Ctrl Pts',(9.32002824922328,-2.40934673847672,-2.946483341358));
#88806=CARTESIAN_POINT('Ctrl Pts',(9.51887546796291,1.17584960081515,-3.61995766596401));
#88807=CARTESIAN_POINT('Ctrl Pts',(9.71772268670256,3.68093457632498,-0.968213009582048));
#88808=CARTESIAN_POINT('Ctrl Pts',(9.91656990544221,2.80478842969927,2.57291228994185));
#88809=CARTESIAN_POINT('Ctrl Pts',(10.1154171241818,-0.647778930849038,
3.75061304907035));
#88810=CARTESIAN_POINT('Ctrl Pts',(10.3142643429215,-3.50530983100003,1.48307746790353));
#88811=CARTESIAN_POINT('Ctrl Pts',(10.5131115616611,-3.14293490355597,-2.14678270421539));
#88812=CARTESIAN_POINT('Ctrl Pts',(10.7119587804008,0.106475663994328,-3.80465224693213));
#88813=CARTESIAN_POINT('Ctrl Pts',(10.9108059991404,3.25807986705142,-1.96764614883441));
#88814=CARTESIAN_POINT('Ctrl Pts',(11.1096532178801,3.4168786245208,1.67679940732383));
#88815=CARTESIAN_POINT('Ctrl Pts',(11.3085004366197,0.437002649736691,3.7809713660952));
#88816=CARTESIAN_POINT('Ctrl Pts',(11.5073476553593,-2.9442950099774,2.41202045624221));
#88817=CARTESIAN_POINT('Ctrl Pts',(11.706194874099,-3.62102356799794,-1.17256305037815));
#88818=CARTESIAN_POINT('Ctrl Pts',(11.9050420928386,-0.971554029250149,
-3.68005415114459));
#88819=CARTESIAN_POINT('Ctrl Pts',(12.1038893115783,2.57036514488798,-2.80712287031647));
#88820=CARTESIAN_POINT('Ctrl Pts',(12.3027365303179,3.75119953391568,0.644373993779587));
#88821=CARTESIAN_POINT('Ctrl Pts',(12.5015837490575,1.48625884967945,3.50396210294263));
#88822=CARTESIAN_POINT('Ctrl Pts',(12.7004309677972,-2.14392877765862,3.14488237990484));
#88823=CARTESIAN_POINT('Ctrl Pts',(12.8992781865368,-3.80474733408567,-0.103021895132036));
#88824=CARTESIAN_POINT('Ctrl Pts',(13.0981254052765,-1.97060290458628,-3.25629236702493));
#88825=CARTESIAN_POINT('Ctrl Pts',(13.2969726240161,1.67369699825765,-3.41839935424929));
#88826=CARTESIAN_POINT('Ctrl Pts',(13.4958198427558,3.78057311315052,-0.440434698033706));
#88827=CARTESIAN_POINT('Ctrl Pts',(13.6946670614954,2.41469218641841,2.94210425239463));
#88828=CARTESIAN_POINT('Ctrl Pts',(13.893514280235,-1.16927553370817,3.62208648618171));
#88829=CARTESIAN_POINT('Ctrl Pts',(14.0923614989747,-3.67917069347074,0.974894248323716));
#88830=CARTESIAN_POINT('Ctrl Pts',(14.2912087177143,-2.80945499776618,-2.56781588176319));
#88831=CARTESIAN_POINT('Ctrl Pts',(14.490055936454,0.640968525723349,-3.7517829276413));
#88832=CARTESIAN_POINT('Ctrl Pts',(14.6889031551936,3.5026114874978,-1.48943900672608));
#88833=CARTESIAN_POINT('Ctrl Pts',(14.8877503739333,3.14682726476055,2.14107308442948));
#88834=CARTESIAN_POINT('Ctrl Pts',(15.0865975926729,-0.0995680413761137,
3.80483928599425));
#88835=CARTESIAN_POINT('Ctrl Pts',(15.2854448114125,-3.25450218369954,1.97355803649236));
#88836=CARTESIAN_POINT('Ctrl Pts',(15.4842920301522,-3.41991726709704,-1.67059321000658));
#88837=CARTESIAN_POINT('Ctrl Pts',(15.6831392488918,-0.4438663833971,-3.78017174488127));
#88838=CARTESIAN_POINT('Ctrl Pts',(15.8819864676315,2.93991107041495,-2.41736192680373));
#88839=CARTESIAN_POINT('Ctrl Pts',(16.0808336863711,3.62314641963944,1.16598705351417));
#88840=CARTESIAN_POINT('Ctrl Pts',(16.2796809051108,0.978233664050299,3.67828420403148));
#88841=CARTESIAN_POINT('Ctrl Pts',(16.4785281238504,-2.56526450266828,2.81178481012661));
#88842=CARTESIAN_POINT('Ctrl Pts',(16.6773753425901,-3.75236322976644,-0.637562529486655));
#88843=CARTESIAN_POINT('Ctrl Pts',(16.8762225613297,-1.49261793642279,-3.50125798577849));
#88844=CARTESIAN_POINT('Ctrl Pts',(17.0750697800694,2.13821562688115,-3.14876955652043));
#88845=CARTESIAN_POINT('Ctrl Pts',(17.273916998809,3.80492810258206,0.0961141055726008));
#88846=CARTESIAN_POINT('Ctrl Pts',(17.4727642175486,1.97651154211755,3.25270931855043));
#88847=CARTESIAN_POINT('Ctrl Pts',(17.6716114362883,-1.66748804512824,3.42143236181325));
#88848=CARTESIAN_POINT('Ctrl Pts',(17.8704586550279,-3.77976726161816,0.447297702999042));
#88849=CARTESIAN_POINT('Ctrl Pts',(18.0693058737676,-2.42002967519819,-2.93771546584566));
#88850=CARTESIAN_POINT('Ctrl Pts',(18.2681530925072,1.16269761250606,-3.62420336749765));
#88851=CARTESIAN_POINT('Ctrl Pts',(18.4670003112469,3.67739468355725,-0.981572273678105));
#88852=CARTESIAN_POINT('Ctrl Pts',(18.6658475299865,2.81411230547795,2.5627110097056));
#88853=CARTESIAN_POINT('Ctrl Pts',(18.8646947487261,-0.634156007876128,
3.75294043981293));
#88854=CARTESIAN_POINT('Ctrl Pts',(19.0635419674658,-3.49990159890004,1.49579563615007));
#88855=CARTESIAN_POINT('Ctrl Pts',(19.2623891862054,-3.15070925358397,-2.13535640736833));
#88856=CARTESIAN_POINT('Ctrl Pts',(19.4612364049451,0.0926600905677234,
-3.80501378377591));
#88857=CARTESIAN_POINT('Ctrl Pts',(19.6600836236847,3.25091377305496,-1.97946341902805));
#88858=CARTESIAN_POINT('Ctrl Pts',(19.8589308424244,3.42294463714945,1.66438150618135));
#88859=CARTESIAN_POINT('Ctrl Pts',(20.057778061164,0.450728654012033,3.77935966369453));
#88860=CARTESIAN_POINT('Ctrl Pts',(20.2566252799037,-2.93551744049599,2.42269542940348));
#88861=CARTESIAN_POINT('Ctrl Pts',(20.4554724986433,-3.62525732888544,-1.15940721339442));
#88862=CARTESIAN_POINT('Ctrl Pts',(20.6543197173829,-0.984910074455989,
-3.67650213278107));
#88863=CARTESIAN_POINT('Ctrl Pts',(20.8531669361226,2.56015540497932,-2.81643748190223));
#88864=CARTESIAN_POINT('Ctrl Pts',(21.0520141548622,3.75351455730514,0.630748963698809));
#88865=CARTESIAN_POINT('Ctrl Pts',(21.2508613736019,1.49897210328941,3.49854232798016));
#88866=CARTESIAN_POINT('Ctrl Pts',(21.4497085923415,-2.13249542824708,3.15264635435279));
#88867=CARTESIAN_POINT('Ctrl Pts',(21.6485558110811,-3.80509632950521,-0.0892059992077045));
#88868=CARTESIAN_POINT('Ctrl Pts',(21.8474030298208,-1.98241366479137,-3.24911554869277));
#88869=CARTESIAN_POINT('Ctrl Pts',(22.0462502485605,1.66127359572584,-3.42445409185943));
#88870=CARTESIAN_POINT('Ctrl Pts',(22.2450974673001,3.77894895144623,-0.454159233608839));
#88871=CARTESIAN_POINT('Ctrl Pts',(22.4439446860397,2.42535918722295,2.93331699617719));
#88872=CARTESIAN_POINT('Ctrl Pts',(22.6427919047794,-1.15611585889066,3.62630830293429));
#88873=CARTESIAN_POINT('Ctrl Pts',(22.841639123519,-3.67560655243846,0.988247063633482));
#88874=CARTESIAN_POINT('Ctrl Pts',(23.0404863422586,-2.81876033748343,-2.55759769059541));
#88875=CARTESIAN_POINT('Ctrl Pts',(23.2393335609983,0.627341399762283,-3.75408558176995));
#88876=CARTESIAN_POINT('Ctrl Pts',(23.4381807797379,3.49718017413892,-1.50214733522328));
#88877=CARTESIAN_POINT('Ctrl Pts',(23.6370279984776,3.15458085723069,2.12963269187493));
#88878=CARTESIAN_POINT('Ctrl Pts',(23.8358752172172,-0.0857518343388183,
3.80517573970196));
#88879=CARTESIAN_POINT('Ctrl Pts',(24.0347224359569,-3.24731464694565,1.98536227697641));
#88880=CARTESIAN_POINT('Ctrl Pts',(24.2335696546965,-3.42596072469933,-1.65816431632281));
#88881=CARTESIAN_POINT('Ctrl Pts',(24.4324168734362,-0.457589438962482,
-3.7785351252117));
#88882=CARTESIAN_POINT('Ctrl Pts',(24.6312640921758,2.93111413470251,-2.42802094646151));
#88883=CARTESIAN_POINT('Ctrl Pts',(24.8301113109155,3.62735628877816,1.15282355170697));
#88884=CARTESIAN_POINT('Ctrl Pts',(25.0289585296551,0.991583238460796,3.67470794326736));
#88885=CARTESIAN_POINT('Ctrl Pts',(25.2278057483947,-2.55503786866146,2.82108087030743));
#88886=CARTESIAN_POINT('Ctrl Pts',(25.4266529671344,-3.75465351273682,-0.623933318874501));
#88887=CARTESIAN_POINT('Ctrl Pts',(25.6255001858741,-1.50532132933512,-3.49581513849881));
#88888=CARTESIAN_POINT('Ctrl Pts',(25.8243474046136,2.12676820061089,-3.1565127606235));
#88889=CARTESIAN_POINT('Ctrl Pts',(26.0231946233533,3.80525201430065,0.0822975988073659));
#88890=CARTESIAN_POINT('Ctrl Pts',(26.2220418420929,1.98830925315355,3.24551106929751));
#88891=CARTESIAN_POINT('Ctrl Pts',(26.4208890608326,-1.65505367053418,3.42746453442775));
#88892=CARTESIAN_POINT('Ctrl Pts',(26.6197362795722,-3.77811818533196,0.461019267246552));
#88893=CARTESIAN_POINT('Ctrl Pts',(26.8185834983119,-2.4306807049259,-2.92890885788714));
#88894=CARTESIAN_POINT('Ctrl Pts',(27.0174307170515,1.14953029455628,-3.62840128555349));
#88895=CARTESIAN_POINT('Ctrl Pts',(27.2162779357912,3.6738063060083,-0.994918596188816));
#88896=CARTESIAN_POINT('Ctrl Pts',(27.4151251545308,2.82339907846205,2.55247594128687));
#88897=CARTESIAN_POINT('Ctrl Pts',(27.6139723732705,-0.620524723843828,
3.75521834973777));
#88898=CARTESIAN_POINT('Ctrl Pts',(27.8128195920101,-3.49444722218464,1.50849408300949));
#88899=CARTESIAN_POINT('Ctrl Pts',(28.0116668107498,-3.15844206293931,-2.12390195681543));
#88900=CARTESIAN_POINT('Ctrl Pts',(28.2105140294894,0.0788432954598658,
-3.80532515323851));
#88901=CARTESIAN_POINT('Ctrl Pts',(28.409361248229,3.24370481723469,-1.99125459089417));
#88902=CARTESIAN_POINT('Ctrl Pts',(28.6082084669687,3.42896551980536,1.6519416609235));
#88903=CARTESIAN_POINT('Ctrl Pts',(28.8070556857083,0.464448715634499,3.7776981321506));
#88904=CARTESIAN_POINT('Ctrl Pts',(29.005902904448,-2.92670116754833,2.43333846042424));
#88905=CARTESIAN_POINT('Ctrl Pts',(29.2047501231876,-3.62944329239912,-1.14623609015233));
#88906=CARTESIAN_POINT('Ctrl Pts',(29.4035973419273,-0.998253134069163,
-3.67290164140422));
#88907=CARTESIAN_POINT('Ctrl Pts',(29.6024445606669,2.54991191058275,-2.82571496003703));
#88908=CARTESIAN_POINT('Ctrl Pts',(29.8012917794065,3.75578009230734,0.617115617479058));
#88909=CARTESIAN_POINT('Ctrl Pts',(30.0001389981462,1.51166559363194,3.49307642632366));
#88910=CARTESIAN_POINT('Ctrl Pts',(30.1989862168858,-2.1210339628504,3.16036876258829));
#88911=CARTESIAN_POINT('Ctrl Pts',(30.3978334356255,-3.80539515645523,-0.0753889271427265));
#88912=CARTESIAN_POINT('Ctrl Pts',(30.5966806543651,-1.99419828777131,-3.24189589224556));
#88913=CARTESIAN_POINT('Ctrl Pts',(30.7955278731047,1.64882829005506,-3.43046367959534));
#88914=CARTESIAN_POINT('Ctrl Pts',(30.9943750918444,3.77727496601373,-0.467877781300454));
#88915=CARTESIAN_POINT('Ctrl Pts',(31.1932223105841,2.43599421076651,2.92449106550537));
#88916=CARTESIAN_POINT('Ctrl Pts',(31.3920695293236,-1.1429409412098,3.63048230845643));
#88917=CARTESIAN_POINT('Ctrl Pts',(31.5909167480633,-3.67199395020061,1.00158684935393));
#88918=CARTESIAN_POINT('Ctrl Pts',(31.789763966803,-2.82802851312397,-2.54734577866189));
#88919=CARTESIAN_POINT('Ctrl Pts',(31.9886111855426,0.613706002589339,-3.75633873998267));
#88920=CARTESIAN_POINT('Ctrl Pts',(32.1874584042823,3.49170275204543,-1.51483585858905));
#88921=CARTESIAN_POINT('Ctrl Pts',(32.3863056230219,3.16229285798277,2.11816422107915));
#88922=CARTESIAN_POINT('Ctrl Pts',(32.5851528417615,-0.071934496702472,
3.80546202389314));
#88923=CARTESIAN_POINT('Ctrl Pts',(32.7840000605012,-3.24008429582074,1.99714034135926));
#88924=CARTESIAN_POINT('Ctrl Pts',(32.9828472792408,-3.43195901256317,-1.64571356049439));
#88925=CARTESIAN_POINT('Ctrl Pts',(33.1816944979805,-0.471306461418734,
-3.77684868727006));
#88926=CARTESIAN_POINT('Ctrl Pts',(33.3805417167201,2.92227855357939,-2.43864795376427));
#88927=CARTESIAN_POINT('Ctrl Pts',(33.5793889354597,3.63151833286923,1.13964485044393));
#88928=CARTESIAN_POINT('Ctrl Pts',(33.7782361541994,1.00491973929605,3.67108323314547));
#88929=CARTESIAN_POINT('Ctrl Pts',(33.977083372939,-2.544777547639,2.83033973581637));
#88930=CARTESIAN_POINT('Ctrl Pts',(34.1759305916787,-3.75689429230335,-0.610295881984437));
#88931=CARTESIAN_POINT('Ctrl Pts',(34.3747778104184,-1.5180048752684,-3.49032620048186));
#88932=CARTESIAN_POINT('Ctrl Pts',(34.573625029158,2.11529273386641,-3.16421434753728));
#88933=CARTESIAN_POINT('Ctrl Pts',(34.7724722478976,3.80552575549711,0.0684800069856816));
#88934=CARTESIAN_POINT('Ctrl Pts',(34.9713194666373,2.00008074923364,3.23827002945302));
#88935=CARTESIAN_POINT('Ctrl Pts',(35.1701666853769,-1.64259747480814,3.43345151747663));
#88936=CARTESIAN_POINT('Ctrl Pts',(35.3690139041165,-3.77641929627087,0.47473475316399));
#88937=CARTESIAN_POINT('Ctrl Pts',(35.5678611228562,-2.44129968723075,-2.92006363359358));
#88938=CARTESIAN_POINT('Ctrl Pts',(35.7667083415958,1.13634782057081,-3.63255136478379));
#88939=CARTESIAN_POINT('Ctrl Pts',(35.9655555603355,3.67016949098924,-1.00825180114912));
#88940=CARTESIAN_POINT('Ctrl Pts',(36.1644027790751,2.83264862620975,2.54220721963035));
#88941=CARTESIAN_POINT('Ctrl Pts',(36.3632499978148,-0.606885258474397,
3.75744674881163));
#88942=CARTESIAN_POINT('Ctrl Pts',(36.5620972165544,-3.48894677276732,1.52117264105857));
#88943=CARTESIAN_POINT('Ctrl Pts',(36.760944435294,-3.1661332296684,-2.11241950357836));
#88944=CARTESIAN_POINT('Ctrl Pts',(36.9597916540338,0.0650254608388847,
-3.80558635121468));
#88945=CARTESIAN_POINT('Ctrl Pts',(37.1586388727733,3.23645309463745,-2.00301950897151));
#88946=CARTESIAN_POINT('Ctrl Pts',(37.357486091513,3.43494119310586,1.63948003556406));
#88947=CARTESIAN_POINT('Ctrl Pts',(37.5563333102526,0.478162653711198,3.77598679336999));
#88948=CARTESIAN_POINT('Ctrl Pts',(37.7551805289923,-2.91784630737312,2.44394940898082));
#88949=CARTESIAN_POINT('Ctrl Pts',(37.9540277477319,-3.63358140334888,-1.13304985430729));
#88950=CARTESIAN_POINT('Ctrl Pts',(38.1528749664715,-1.01158303216742,-3.66925272448487));
#88951=CARTESIAN_POINT('Ctrl Pts',(38.3517221852113,2.53963479675394,-2.83495518240152));
#88952=CARTESIAN_POINT('Ctrl Pts',(38.5505694039508,3.75799610905227,0.603474134869659));
#88953=CARTESIAN_POINT('Ctrl Pts',(38.7494166226906,1.52433915334921,3.48756447003854));
#88954=CARTESIAN_POINT('Ctrl Pts',(38.9482638414301,-2.10954453258275,3.16804950279488));
#88955=CARTESIAN_POINT('Ctrl Pts',(39.1471110601698,-3.80564381099585,-0.0615708611088804));
#88956=CARTESIAN_POINT('Ctrl Pts',(39.3459582789094,-2.00595661815121,-3.23463349287117));
#88957=CARTESIAN_POINT('Ctrl Pts',(39.5448054976491,1.63636124533099,-3.43642803822336));
#88958=CARTESIAN_POINT('Ctrl Pts',(39.7436527163887,3.77555117892381,-0.481590160235665));
#88959=CARTESIAN_POINT('Ctrl Pts',(39.9424999351283,2.44659711683104,2.91562657674516));
#88960=CARTESIAN_POINT('Ctrl Pts',(40.141347153868,-1.12975095437104,3.63460844771571));
#88961=CARTESIAN_POINT('Ctrl Pts',(40.3401943726076,-3.66833293438782,1.01491342960588));
#88962=CARTESIAN_POINT('Ctrl Pts',(40.5390415913473,-2.83725940249097,-2.53706028112956));
#88963=CARTESIAN_POINT('Ctrl Pts',(40.7378888100869,0.600062513981104,-3.75854237257257));
#88964=CARTESIAN_POINT('Ctrl Pts',(40.9367360288266,3.48617929343457,-1.52750440953102));
#88965=CARTESIAN_POINT('Ctrl Pts',(41.1355832475663,3.16996316533766,2.10666782324859));
#88966=CARTESIAN_POINT('Ctrl Pts',(41.3344304663058,-0.0581162106423564,
3.80569813479336));
#88967=CARTESIAN_POINT('Ctrl Pts',(41.5332776850456,-3.23281122565374,2.00889207435229));
#88968=CARTESIAN_POINT('Ctrl Pts',(41.732124903785,-3.43791205160379,-1.63324110667881));
#88969=CARTESIAN_POINT('Ctrl Pts',(41.9309721225249,-0.48501726991304,-3.77511245329163));
#88970=CARTESIAN_POINT('Ctrl Pts',(42.1298193412644,2.91340444353883,-2.44924280859897));
#88971=CARTESIAN_POINT('Ctrl Pts',(42.3286665600041,3.63563249703791,1.12645112347912));
#88972=CARTESIAN_POINT('Ctrl Pts',(42.5275137787437,1.01824299072025,3.66741012145854));
#88973=CARTESIAN_POINT('Ctrl Pts',(42.7263609974834,-2.53448367487889,2.83956128457451));
#88974=CARTESIAN_POINT('Ctrl Pts',(42.925208216223,-3.75908553892202,-0.59665039861077));
#88975=CARTESIAN_POINT('Ctrl Pts',(43.1240554349627,-1.53066840699641,-3.48479124411454));
#88976=CARTESIAN_POINT('Ctrl Pts',(43.3229026537023,2.10378937794771,-3.17187421568591));
#88977=CARTESIAN_POINT('Ctrl Pts',(43.521749872442,3.80574932255986,0.0546615122211324));
#88978=CARTESIAN_POINT('Ctrl Pts',(43.7205970911815,2.01182587516079,3.23098629461087));
#88979=CARTESIAN_POINT('Ctrl Pts',(43.9194443099213,-1.63011962218803,3.43939323178678));
#88980=CARTESIAN_POINT('Ctrl Pts',(44.1182915286608,-3.77467061681703,0.488443980373654));
#88981=CARTESIAN_POINT('Ctrl Pts',(44.3171387474006,-2.45188648213872,-2.91117991045481));
#88982=CARTESIAN_POINT('Ctrl Pts',(44.5159859661402,1.12315036441649,-3.63665354880811));
#88983=CARTESIAN_POINT('Ctrl Pts',(44.7148331848798,3.66648428633161,-1.02157171594932));
#88984=CARTESIAN_POINT('Ctrl Pts',(44.9136804036194,2.84186082699613,2.53190498621347));
#88985=CARTESIAN_POINT('Ctrl Pts',(45.1125276223591,-0.59323779203106,3.75962559600542));
#88986=CARTESIAN_POINT('Ctrl Pts',(45.3113748410987,-3.48340032234089,1.53383116542125));
#88987=CARTESIAN_POINT('Ctrl Pts',(45.5102220598384,-3.17378265395104,-2.10090924168198));
#88988=CARTESIAN_POINT('Ctrl Pts',(45.7090692785781,0.0512067719178791,
-3.8057972926977));
#88989=CARTESIAN_POINT('Ctrl Pts',(45.9079164973176,3.22915869507492,-2.01475817418338));
#88990=CARTESIAN_POINT('Ctrl Pts',(46.1067637160574,3.44087158935841,1.62699709292146));
#88991=CARTESIAN_POINT('Ctrl Pts',(46.3056109347969,0.491870266206481,3.7742250988203));
#88992=CARTESIAN_POINT('Ctrl Pts',(46.5044581535366,-2.9089529361142,2.45452922773842));
#88993=CARTESIAN_POINT('Ctrl Pts',(46.7033053722762,-3.63767168485402,-1.11985076990585));
#88994=CARTESIAN_POINT('Ctrl Pts',(46.9021525910159,-1.02489944439545,-3.66555143137609));
#88995=CARTESIAN_POINT('Ctrl Pts',(47.1009998097555,2.52932391469176,-2.84416567720655));
#88996=CARTESIAN_POINT('Ctrl Pts',(47.2998470284952,3.76016312221924,0.589839331053052));
#88997=CARTESIAN_POINT('Ctrl Pts',(47.4986942472348,1.53699157481281,3.48197853288055));
#88998=CARTESIAN_POINT('Ctrl Pts',(47.6975414659745,-2.09802529825852,3.1757420386404));
#88999=CARTESIAN_POINT('Ctrl Pts',(47.896388684714,-3.80584609838521,-0.0478544593189315));
#89000=CARTESIAN_POINT('Ctrl Pts',(48.0952359034538,-2.01768121316929,-3.22713239264578));
#89001=CARTESIAN_POINT('Ctrl Pts',(48.2940831221933,1.62385866935796,-3.44272221687208));
#89002=CARTESIAN_POINT('Ctrl Pts',(48.4929303409331,3.77380444199112,-0.494578024227625));
#89003=CARTESIAN_POINT('Ctrl Pts',(48.6917775596727,2.45711528607269,2.90534518289334));
#89004=CARTESIAN_POINT('Ctrl Pts',(48.8906247784123,-1.11643535726112,3.64136445027353));
#89005=CARTESIAN_POINT('Ctrl Pts',(49.089471997152,-3.66492661322599,1.02274087396531));
#89006=CARTESIAN_POINT('Ctrl Pts',(49.2220368096451,-3.11846394970298,-1.33452918861123));
#89007=CARTESIAN_POINT('Ctrl Pts',(49.2883192158916,-2.4066862419943,-2.13636896613036));
#89008=CARTESIAN_POINT('Ctrl Pts',(0.311212348987778,-1.53723282329044,
3.09685835129577));
#89009=CARTESIAN_POINT('Ctrl Pts',(0.377494755234326,-2.56901842462149,
2.58469585852276));
#89010=CARTESIAN_POINT('Ctrl Pts',(0.510059567727422,-4.06230121368214,
0.456641786001921));
#89011=CARTESIAN_POINT('Ctrl Pts',(0.708906786467066,-2.57795834828882,
-3.17766930833127));
#89012=CARTESIAN_POINT('Ctrl Pts',(0.907754005206709,1.27789992154481,-3.88312530093257));
#89013=CARTESIAN_POINT('Ctrl Pts',(1.10660122394635,3.95813182483745,-1.02656764819223));
#89014=CARTESIAN_POINT('Ctrl Pts',(1.30544844268599,3.00342840161775,2.7755327738099));
#89015=CARTESIAN_POINT('Ctrl Pts',(1.50429566142564,-0.710645173066041,
4.02675109516382));
#89016=CARTESIAN_POINT('Ctrl Pts',(1.70314288016528,-3.77168257203434,1.5797755668379));
#89017=CARTESIAN_POINT('Ctrl Pts',(1.90199009890492,-3.36826135439415,-2.3187138663657));
#89018=CARTESIAN_POINT('Ctrl Pts',(2.10083731764456,0.12924463646661,-4.08708974316909));
#89019=CARTESIAN_POINT('Ctrl Pts',(2.29968453638421,3.50799315213455,-2.10124824565113));
#89020=CARTESIAN_POINT('Ctrl Pts',(2.49853175512385,3.66438981334077,1.81480890460361));
#89021=CARTESIAN_POINT('Ctrl Pts',(2.6973789738635,0.45474319704599,4.06379255528071));
#89022=CARTESIAN_POINT('Ctrl Pts',(2.89622619260314,-3.17261606634541,2.57987380459977));
#89023=CARTESIAN_POINT('Ctrl Pts',(3.09507341134279,-3.88567786872364,-1.27387162418561));
#89024=CARTESIAN_POINT('Ctrl Pts',(3.29392063008242,-1.02943414864856,-3.95746078059767));
#89025=CARTESIAN_POINT('Ctrl Pts',(3.49276784882208,2.77242596493276,-3.00580953731097));
#89026=CARTESIAN_POINT('Ctrl Pts',(3.69161506756171,4.02759274580539,0.706917854313252));
#89027=CARTESIAN_POINT('Ctrl Pts',(3.89046228630136,1.58309510844274,3.77028442663091));
#89028=CARTESIAN_POINT('Ctrl Pts',(4.089309505041,-2.31560117140205,3.37034522410938));
#89029=CARTESIAN_POINT('Ctrl Pts',(4.28815672378064,-4.08723368983554,-0.125524233587091));
#89030=CARTESIAN_POINT('Ctrl Pts',(4.48700394252029,-2.1044170121688,-3.50608962159895));
#89031=CARTESIAN_POINT('Ctrl Pts',(4.68585116125993,1.81147402279106,-3.66603292376414));
#89032=CARTESIAN_POINT('Ctrl Pts',(4.88469837999958,4.06338212434606,-0.458433435021463));
#89033=CARTESIAN_POINT('Ctrl Pts',(5.08354559873922,2.58275061397783,3.17027360782739));
#89034=CARTESIAN_POINT('Ctrl Pts',(5.28239281747886,-1.27034271763307,3.88683224259547));
#89035=CARTESIAN_POINT('Ctrl Pts',(5.48124003621851,-3.95652524453957,1.03302637235576));
#89036=CARTESIAN_POINT('Ctrl Pts',(5.68008725495814,-3.00832470456206,-2.76969636717897));
#89037=CARTESIAN_POINT('Ctrl Pts',(5.8789344736978,0.703261303022831,-4.02823274363765));
#89038=CARTESIAN_POINT('Ctrl Pts',(6.07778169243743,3.76884587948186,-1.58651701313895));
#89039=CARTESIAN_POINT('Ctrl Pts',(6.27662891117708,3.37244581092541,2.31254075605715));
#89040=CARTESIAN_POINT('Ctrl Pts',(6.47547612991672,-0.121813917185409,
4.08734594401073));
#89041=CARTESIAN_POINT('Ctrl Pts',(6.67432334865637,-3.5041778755475,2.107598850067));
#89042=CARTESIAN_POINT('Ctrl Pts',(6.87317056739601,-3.66767579740066,-1.80814538724816));
#89043=CARTESIAN_POINT('Ctrl Pts',(7.07201778613565,-0.462121839925715,
-4.06296429979165));
#89044=CARTESIAN_POINT('Ctrl Pts',(7.2708650048753,3.1679277761891,-2.58562740957428));
#89045=CARTESIAN_POINT('Ctrl Pts',(7.46971222361494,3.88798381120942,1.26681386954273));
#89046=CARTESIAN_POINT('Ctrl Pts',(7.66855944235458,1.03661753696874,3.95558587043034));
#89047=CARTESIAN_POINT('Ctrl Pts',(7.86740666109425,-2.766964378456,3.01083769483692));
#89048=CARTESIAN_POINT('Ctrl Pts',(8.06625387983386,-4.02886947885365,-0.699604330073128));
#89049=CARTESIAN_POINT('Ctrl Pts',(8.26510109857353,-1.58993758080563,-3.7674041441606));
#89050=CARTESIAN_POINT('Ctrl Pts',(8.46394831731315,2.30947841958156,-3.37454366185755));
#89051=CARTESIAN_POINT('Ctrl Pts',(8.6627955360528,4.08745483818023,0.118103522949025));
#89052=CARTESIAN_POINT('Ctrl Pts',(8.86164275479245,2.11077894699056,3.5022632301467));
#89053=CARTESIAN_POINT('Ctrl Pts',(9.06048997353207,-1.8048152595142,3.66931565490361));
#89054=CARTESIAN_POINT('Ctrl Pts',(9.25933719227176,-4.06254312837073,0.465809860805664));
#89055=CARTESIAN_POINT('Ctrl Pts',(9.45818441101136,-2.58850207391776,-3.16557933238444));
#89056=CARTESIAN_POINT('Ctrl Pts',(9.65703162975104,1.26328397723694,-3.88913217686831));
#89057=CARTESIAN_POINT('Ctrl Pts',(9.85587884849066,3.95464323694529,-1.04020784691275));
#89058=CARTESIAN_POINT('Ctrl Pts',(10.0547260672303,3.01334820398965,2.76423010941716));
#89059=CARTESIAN_POINT('Ctrl Pts',(10.25357328597,-0.695946780579781,4.02950289426584));
#89060=CARTESIAN_POINT('Ctrl Pts',(10.4524205047096,-3.76595930439009,1.59335683824238));
#89061=CARTESIAN_POINT('Ctrl Pts',(10.6512677234492,-3.37663873203523,-2.30641417998059));
#89062=CARTESIAN_POINT('Ctrl Pts',(10.8501149421889,0.114393031384766,-4.08756036416182));
#89063=CARTESIAN_POINT('Ctrl Pts',(11.0489621609285,3.50034569876179,-2.11395730454897));
#89064=CARTESIAN_POINT('Ctrl Pts',(11.2478093796682,3.67095248876026,1.80148364454438));
#89065=CARTESIAN_POINT('Ctrl Pts',(11.4466565984078,0.469497497842897,4.06211860927464));
#89066=CARTESIAN_POINT('Ctrl Pts',(11.6455038171475,-3.16322828003209,2.59137460524359));
#89067=CARTESIAN_POINT('Ctrl Pts',(11.8443510358871,-3.89027733774591,-1.25975304394023));
#89068=CARTESIAN_POINT('Ctrl Pts',(12.0431982546268,-1.0437972996892,-3.95369734469618));
#89069=CARTESIAN_POINT('Ctrl Pts',(12.2420454733664,2.76149356255603,-3.01585623003779));
#89070=CARTESIAN_POINT('Ctrl Pts',(12.4408926921061,4.03013298922653,0.692288657601849));
#89071=CARTESIAN_POINT('Ctrl Pts',(12.6397399108457,1.59677478269736,3.76451136133733));
#89072=CARTESIAN_POINT('Ctrl Pts',(12.8385871295853,-2.30334803981363,3.37873101974436));
#89073=CARTESIAN_POINT('Ctrl Pts',(13.037434348325,-4.08766252185056,-0.110682445556626));
#89074=CARTESIAN_POINT('Ctrl Pts',(13.2362815670646,-2.1171339201326,-3.49842528296947));
#89075=CARTESIAN_POINT('Ctrl Pts',(13.4351287858043,1.79815054508896,-3.67258629762356));
#89076=CARTESIAN_POINT('Ctrl Pts',(13.6339760045439,4.06169074285061,-0.473184747997776));
#89077=CARTESIAN_POINT('Ctrl Pts',(13.8328232232836,2.59424500118603,3.1608746210689));
#89078=CARTESIAN_POINT('Ctrl Pts',(14.0316704420232,-1.25622107256294,3.89141929289879));
#89079=CARTESIAN_POINT('Ctrl Pts',(14.2305176607629,-3.95274819446203,1.04738589234015));
#89080=CARTESIAN_POINT('Ctrl Pts',(14.4293648795025,-3.01836177091483,-2.7587547401275));
#89081=CARTESIAN_POINT('Ctrl Pts',(14.6282120982422,0.688629964153758,-4.03075976321656));
#89082=CARTESIAN_POINT('Ctrl Pts',(14.8270593169817,3.76306031619543,-1.60019141135405));
#89083=CARTESIAN_POINT('Ctrl Pts',(15.0259065357214,3.38082052326087,2.30028000160723));
#89084=CARTESIAN_POINT('Ctrl Pts',(15.2247537544611,-0.106971768522289,
4.08776131116228));
#89085=CARTESIAN_POINT('Ctrl Pts',(15.4236009732007,-3.49650198435228,2.12030879112374));
#89086=CARTESIAN_POINT('Ctrl Pts',(15.6224481919403,-3.67421708014717,-1.79481596389458));
#89087=CARTESIAN_POINT('Ctrl Pts',(15.82129541068,-0.476871608231848,-4.06125952945123));
#89088=CARTESIAN_POINT('Ctrl Pts',(16.0201426294196,3.15851835743435,-2.59711325937978));
#89089=CARTESIAN_POINT('Ctrl Pts',(16.2189898481593,3.89255804138596,1.25268806601546));
#89090=CARTESIAN_POINT('Ctrl Pts',(16.4178370668989,1.05097362190846,3.95179578702503));
#89091=CARTESIAN_POINT('Ctrl Pts',(16.6166842856386,-2.75601364438854,3.02086482455609));
#89092=CARTESIAN_POINT('Ctrl Pts',(16.8155315043782,-4.03138321571946,-0.684970703250532));
#89093=CARTESIAN_POINT('Ctrl Pts',(17.0143787231179,-1.60360672139697,-3.7616061701601));
#89094=CARTESIAN_POINT('Ctrl Pts',(17.2132259418575,2.29721006788957,-3.38290724086293));
#89095=CARTESIAN_POINT('Ctrl Pts',(17.4120731605971,4.08785673201563,0.103261003339431));
#89096=CARTESIAN_POINT('Ctrl Pts',(17.6109203793368,2.12348191490623,3.49457580449507));
#89097=CARTESIAN_POINT('Ctrl Pts',(17.8097675980764,-1.79147990370901,3.67584483498729));
#89098=CARTESIAN_POINT('Ctrl Pts',(18.0086148168161,-4.06082496943184,0.480558075507004));
#89099=CARTESIAN_POINT('Ctrl Pts',(18.2074620355557,-2.59997937746127,-3.15615949107014));
#89100=CARTESIAN_POINT('Ctrl Pts',(18.4063092542954,1.24915402720918,-3.89369358226904));
#89101=CARTESIAN_POINT('Ctrl Pts',(18.605156473035,3.95084012316994,-1.05456048543771));
#89102=CARTESIAN_POINT('Ctrl Pts',(18.8040036917746,3.02336538889901,2.75327027759783));
#89103=CARTESIAN_POINT('Ctrl Pts',(19.0028509105143,-0.681310877907465,
4.03200334622145));
#89104=CARTESIAN_POINT('Ctrl Pts',(19.2016981292539,-3.76014892442961,1.60702071001181));
#89105=CARTESIAN_POINT('Ctrl Pts',(19.4005453479936,-3.38499117083098,-2.29413824119044));
#89106=CARTESIAN_POINT('Ctrl Pts',(19.5993925667332,0.0995501530659145,
-4.08794878433189));
#89107=CARTESIAN_POINT('Ctrl Pts',(19.7982397854729,3.49264674498503,-2.1266532888653));
#89108=CARTESIAN_POINT('Ctrl Pts',(19.9970870042125,3.67746956080263,1.78814236728127));
#89109=CARTESIAN_POINT('Ctrl Pts',(20.1959342229522,0.484244146785501,4.06038706315052));
#89110=CARTESIAN_POINT('Ctrl Pts',(20.3947814416918,-3.15379802392003,2.60284335306874));
#89111=CARTESIAN_POINT('Ctrl Pts',(20.5936286604314,-3.89482591461231,-1.24561895905628));
#89112=CARTESIAN_POINT('Ctrl Pts',(20.7924758791711,-1.0581464799722,-3.94988120368429));
#89113=CARTESIAN_POINT('Ctrl Pts',(20.9913230979107,2.75052464201603,-3.02586346188301));
#89114=CARTESIAN_POINT('Ctrl Pts',(21.1901703166504,4.03262015421157,0.677650491140349));
#89115=CARTESIAN_POINT('Ctrl Pts',(21.38901753539,1.61043337438535,3.7586885802048));
#89116=CARTESIAN_POINT('Ctrl Pts',(21.5878647541296,-2.29106452404108,3.38707231144781));
#89117=CARTESIAN_POINT('Ctrl Pts',(21.7867119728693,-4.08803746803528,-0.0958392207596079));
#89118=CARTESIAN_POINT('Ctrl Pts',(21.9855591916089,-2.12982291038758,-3.49071480741183));
#89119=CARTESIAN_POINT('Ctrl Pts',(22.1844064103486,1.78480335736162,-3.67909125625429));
#89120=CARTESIAN_POINT('Ctrl Pts',(22.3832536290882,4.05994581096812,-0.487929819029873));
#89121=CARTESIAN_POINT('Ctrl Pts',(22.5821008478279,2.6057051838422,3.15143395792994));
#89122=CARTESIAN_POINT('Ctrl Pts',(22.7809480665675,-1.24208286446976,3.89595503748267));
#89123=CARTESIAN_POINT('Ctrl Pts',(22.9797952853071,-3.94891902935828,1.06173160255694));
#89124=CARTESIAN_POINT('Ctrl Pts',(23.1786425040468,-3.0283590414496,-2.74777673990566));
#89125=CARTESIAN_POINT('Ctrl Pts',(23.3774897227864,0.67398954596553,-4.0332336391815));
#89126=CARTESIAN_POINT('Ctrl Pts',(23.5763369415261,3.75722513868898,-1.61384471170543));
#89127=CARTESIAN_POINT('Ctrl Pts',(23.7751841602657,3.38915066099852,2.28798891897434));
#89128=CARTESIAN_POINT('Ctrl Pts',(23.9740313790054,-0.0921282094784277,
4.08812278305269));
#89129=CARTESIAN_POINT('Ctrl Pts',(24.172878597745,-3.48877999336747,2.13299077686121));
#89130=CARTESIAN_POINT('Ctrl Pts',(24.3717258164847,-3.68070992000593,-1.78146287670161));
#89131=CARTESIAN_POINT('Ctrl Pts',(24.5705730352243,-0.491615089202934,
-4.05950121324825));
#89132=CARTESIAN_POINT('Ctrl Pts',(24.769420253964,3.14906729504797,-2.60856486742333));
#89133=CARTESIAN_POINT('Ctrl Pts',(24.9682674727036,3.89708094994972,1.23854574636347));
#89134=CARTESIAN_POINT('Ctrl Pts',(25.1671146914432,1.06531585023767,3.94795360098474));
#89135=CARTESIAN_POINT('Ctrl Pts',(25.3659619101829,-2.74502657353107,3.03085212554231));
#89136=CARTESIAN_POINT('Ctrl Pts',(25.5648091289225,-4.03384380062572,-0.670328045399746));
#89137=CARTESIAN_POINT('Ctrl Pts',(25.7636563476621,-1.61725471916093,-3.75575860108816));
#89138=CARTESIAN_POINT('Ctrl Pts',(25.9625035664018,2.28491142852464,-3.39122621777043));
#89139=CARTESIAN_POINT('Ctrl Pts',(26.1613507851414,4.0882047293138,0.0884171222803186));
#89140=CARTESIAN_POINT('Ctrl Pts',(26.3601980038811,2.13615688567587,3.48684230444618));
#89141=CARTESIAN_POINT('Ctrl Pts',(26.5590452226207,-1.77812092805368,3.68232555072383));
#89142=CARTESIAN_POINT('Ctrl Pts',(26.7578924413604,-4.05905327035726,0.495299954268107));
#89143=CARTESIAN_POINT('Ctrl Pts',(26.9567396601,-2.61142240145579,-3.14669803722426));
#89144=CARTESIAN_POINT('Ctrl Pts',(27.1555868788397,1.23500760765211,-3.89820365108567));
#89145=CARTESIAN_POINT('Ctrl Pts',(27.3544340975793,3.94698491935925,-1.06889922006086));
#89146=CARTESIAN_POINT('Ctrl Pts',(27.5532813163189,3.03334271210678,2.74227414515849));
#89147=CARTESIAN_POINT('Ctrl Pts',(27.7521285350586,-0.666665992460189,
4.03445063804146));
#89148=CARTESIAN_POINT('Ctrl Pts',(27.9509757537983,-3.75428896861078,1.62066339394195));
#89149=CARTESIAN_POINT('Ctrl Pts',(28.1498229725379,-3.39329898005322,-2.28183205522795));
#89150=CARTESIAN_POINT('Ctrl Pts',(28.3486701912775,0.0847059622234647,
-4.08828330675111));
#89151=CARTESIAN_POINT('Ctrl Pts',(28.5475174100172,3.48490174224484,-2.13932123422241));
#89152=CARTESIAN_POINT('Ctrl Pts',(28.7463646287568,3.68393814707654,1.77477751417194));
#89153=CARTESIAN_POINT('Ctrl Pts',(28.9452118474964,0.498984411188661,4.05860198266432));
#89154=CARTESIAN_POINT('Ctrl Pts',(29.1440590662361,-3.14432618641123,2.61427778358472));
#89155=CARTESIAN_POINT('Ctrl Pts',(29.3429062849758,-3.89932313996533,-1.23146845125119));
#89156=CARTESIAN_POINT('Ctrl Pts',(29.5417535037154,-1.07248170907375,-3.94601298528001));
#89157=CARTESIAN_POINT('Ctrl Pts',(29.740600722455,2.73951945705602,-3.0358307990907));
#89158=CARTESIAN_POINT('Ctrl Pts',(29.9394479411946,4.03505415092864,0.663003390164515));
#89159=CARTESIAN_POINT('Ctrl Pts',(30.1382951599344,1.62407073323958,3.75281624246787));
#89160=CARTESIAN_POINT('Ctrl Pts',(30.3371423786739,-2.27875080162179,3.39536894613885));
#89161=CARTESIAN_POINT('Ctrl Pts',(30.5359895974136,-4.08835851529988,-0.0809947323659286));
#89162=CARTESIAN_POINT('Ctrl Pts',(30.7348368161532,-2.14248381989336,-3.48295830836248));
#89163=CARTESIAN_POINT('Ctrl Pts',(30.9336840348929,1.77143263781142,-3.68554770773524));
#89164=CARTESIAN_POINT('Ctrl Pts',(31.1325312536326,4.05814735054126,-0.502668456928601));
#89165=CARTESIAN_POINT('Ctrl Pts',(31.3313784723722,2.61713101145724,3.14195174456338));
#89166=CARTESIAN_POINT('Ctrl Pts',(31.5302256911118,-1.22792828007724,3.90043941566621));
#89167=CARTESIAN_POINT('Ctrl Pts',(31.7290729098515,-3.94503779954791,1.07606331432411));
#89168=CARTESIAN_POINT('Ctrl Pts',(31.9279201285911,-3.03831638444379,-2.73676251149355));
#89169=CARTESIAN_POINT('Ctrl Pts',(32.1267673473308,0.659340241530767,-4.03565433878998));
#89170=CARTESIAN_POINT('Ctrl Pts',(32.3256145660704,3.75134042387302,-1.62747673424613));
#89171=CARTESIAN_POINT('Ctrl Pts',(32.52446178481,3.39743611432164,2.27566767024519));
#89172=CARTESIAN_POINT('Ctrl Pts',(32.7233090035497,-0.0772834357659036,
4.0884303548981));
#89173=CARTESIAN_POINT('Ctrl Pts',(32.9221562222893,-3.48101200440053,2.14564464008266));
#89174=CARTESIAN_POINT('Ctrl Pts',(33.121003441029,-3.68715423137363,-1.7680863017284));
#89175=CARTESIAN_POINT('Ctrl Pts',(33.3198506597686,-0.506352088452131,
-4.05768937436273));
#89176=CARTESIAN_POINT('Ctrl Pts',(33.5186978785082,3.13957471363731,-2.61998208272218));
#89177=CARTESIAN_POINT('Ctrl Pts',(33.7175450972479,3.90155247726848,1.22438709704741));
#89178=CARTESIAN_POINT('Ctrl Pts',(33.9163923159875,1.0796440328606,3.94405936296661));
#89179=CARTESIAN_POINT('Ctrl Pts',(34.1152395347272,-2.73400331074305,3.04079946611777));
#89180=CARTESIAN_POINT('Ctrl Pts',(34.3140867534668,-4.03625120113083,-0.655676549577613));
#89181=CARTESIAN_POINT('Ctrl Pts',(34.5129339722065,-1.63088139415487,-3.7498615140423));
#89182=CARTESIAN_POINT('Ctrl Pts',(34.7117811909461,2.27258266363874,-3.39950048289815));
#89183=CARTESIAN_POINT('Ctrl Pts',(34.9106284096858,4.08849882548661,0.0735720754816196));
#89184=CARTESIAN_POINT('Ctrl Pts',(35.1094756284254,2.14880369218564,3.47906283196285));
#89185=CARTESIAN_POINT('Ctrl Pts',(35.3083228471651,-1.76473850868036,3.68875771666786));
#89186=CARTESIAN_POINT('Ctrl Pts',(35.5071700659047,-4.05722805450612,0.510035302723816));
#89187=CARTESIAN_POINT('Ctrl Pts',(35.7060172846443,-2.62283099503016,-3.13719509559179));
#89188=CARTESIAN_POINT('Ctrl Pts',(35.904864503384,1.22084490507974,-3.90266232385494));
#89189=CARTESIAN_POINT('Ctrl Pts',(36.1037117221236,3.94307767634231,-1.08322386173262));
#89190=CARTESIAN_POINT('Ctrl Pts',(36.3025589408633,3.04328004206655,2.73124185707811));
#89191=CARTESIAN_POINT('Ctrl Pts',(36.501406159603,-0.65201231732407,4.03684473745941));
#89192=CARTESIAN_POINT('Ctrl Pts',(36.7002533783425,-3.74837951419443,1.63428471016025));
#89193=CARTESIAN_POINT('Ctrl Pts',(36.8991005970822,-3.40156205016727,-2.26949578434459));
#89194=CARTESIAN_POINT('Ctrl Pts',(37.0979478158218,0.0698606545712825,
-4.08856392700898));
#89195=CARTESIAN_POINT('Ctrl Pts',(37.2967950345615,3.47711079265562,-2.15196097359922));
#89196=CARTESIAN_POINT('Ctrl Pts',(37.4956422533011,3.69035816229659,1.76138926142602));
#89197=CARTESIAN_POINT('Ctrl Pts',(37.6944894720408,0.513718096708562,4.05676339135156));
#89198=CARTESIAN_POINT('Ctrl Pts',(37.8933366907804,-3.13481289238768,2.62567774603361));
#89199=CARTESIAN_POINT('Ctrl Pts',(38.0921839095201,-3.90376895451103,-1.21730170709314));
#89200=CARTESIAN_POINT('Ctrl Pts',(38.2910311282597,-1.08680279799026,-3.94209274048399));
#89201=CARTESIAN_POINT('Ctrl Pts',(38.4898783469994,2.72847815277427,-3.04575811024604));
#89202=CARTESIAN_POINT('Ctrl Pts',(38.688725565739,4.03743494728661,0.648347547789554));
#89203=CARTESIAN_POINT('Ctrl Pts',(38.8875727844787,1.63768667945778,3.74689442555066));
#89204=CARTESIAN_POINT('Ctrl Pts',(39.0864200032183,-2.26640703490652,3.40362081443016));
#89205=CARTESIAN_POINT('Ctrl Pts',(39.2852672219579,-4.08862565941151,-0.0661491760933774));
#89206=CARTESIAN_POINT('Ctrl Pts',(39.4841144406975,-2.15511648172164,-3.47515588808729));
#89207=CARTESIAN_POINT('Ctrl Pts',(39.6829616594372,1.75803856272522,-3.69195556694108));
#89208=CARTESIAN_POINT('Ctrl Pts',(39.8818088781768,4.05629538528197,-0.517400467371642));
#89209=CARTESIAN_POINT('Ctrl Pts',(40.0806560969165,2.62852233338666,3.132428105988));
#89210=CARTESIAN_POINT('Ctrl Pts',(40.2795033156561,-1.21375750600731,3.90487236832485));
#89211=CARTESIAN_POINT('Ctrl Pts',(40.4783505343958,-3.94110455620326,1.09038083868435));
#89212=CARTESIAN_POINT('Ctrl Pts',(40.6771977531354,-3.04823366861422,-2.72571220010894));
#89213=CARTESIAN_POINT('Ctrl Pts',(40.8760449718751,0.64468224399396,-4.03802183012611));
#89214=CARTESIAN_POINT('Ctrl Pts',(41.0748921906147,3.74540624933471,-1.64108729924416));
#89215=CARTESIAN_POINT('Ctrl Pts',(41.2737394093544,3.40567677399036,2.26331641786971));
#89216=CARTESIAN_POINT('Ctrl Pts',(41.472586628094,-0.0624376431062618,
4.08868402264345));
#89217=CARTESIAN_POINT('Ctrl Pts',(41.6714338468336,-3.47319811986895,2.15827021395247));
#89218=CARTESIAN_POINT('Ctrl Pts',(41.8702810655733,-3.69354992928488,-1.75468641533891));
#89219=CARTESIAN_POINT('Ctrl Pts',(42.0691282843129,-0.521082411678686,
-4.05582403668333));
#89220=CARTESIAN_POINT('Ctrl Pts',(42.2679755030526,3.13004073835791,-2.63136475474465));
#89221=CARTESIAN_POINT('Ctrl Pts',(42.4668227217923,3.90597256438712,1.21021230474138));
#89222=CARTESIAN_POINT('Ctrl Pts',(42.6656699405318,1.09395798086656,3.94011312431713));
#89223=CARTESIAN_POINT('Ctrl Pts',(42.8645171592716,-2.72294400136152,3.05070671512597));
#89224=CARTESIAN_POINT('Ctrl Pts',(43.0633643780111,-4.03860538549387,-0.641016408947679));
#89225=CARTESIAN_POINT('Ctrl Pts',(43.2622115967508,-1.64448656671789,-3.74391498679197));
#89226=CARTESIAN_POINT('Ctrl Pts',(43.4610588154904,2.26022393578235,-3.40772992711721));
#89227=CARTESIAN_POINT('Ctrl Pts',(43.6599060342301,4.08873901665392,0.0587260585986082));
#89228=CARTESIAN_POINT('Ctrl Pts',(43.8587532529697,2.16142216769827,3.47123748974718));
#89229=CARTESIAN_POINT('Ctrl Pts',(44.0576004717093,-1.75133282203951,3.69514124775901));
#89230=CARTESIAN_POINT('Ctrl Pts',(44.2564476904491,-4.05534934592483,0.524763927083821));
#89231=CARTESIAN_POINT('Ctrl Pts',(44.4552949091886,-2.63420500780209,-3.1276507923989));
#89232=CARTESIAN_POINT('Ctrl Pts',(44.6541421279284,1.20666610628738,-3.90706954000401));
#89233=CARTESIAN_POINT('Ctrl Pts',(44.8529893466679,3.93911844550736,-1.09753422500833));
#89234=CARTESIAN_POINT('Ctrl Pts',(45.0518365654076,3.0531772480021,2.72017356535418));
#89235=CARTESIAN_POINT('Ctrl Pts',(45.2506837841472,-0.637350046166439,
4.03918560039532));
#89236=CARTESIAN_POINT('Ctrl Pts',(45.4495310028869,-3.74242063820434,1.6478845030179));
#89237=CARTESIAN_POINT('Ctrl Pts',(45.6483782216265,-3.40978027393047,-2.25712963699257));
#89238=CARTESIAN_POINT('Ctrl Pts',(45.8472254403661,0.0550144290946424,
-4.08879055377777));
#89239=CARTESIAN_POINT('Ctrl Pts',(46.0460726591059,3.46927399270728,-2.16457250798764));
#89240=CARTESIAN_POINT('Ctrl Pts',(46.2449198778454,3.69672953373671,1.74797810627639));
#89241=CARTESIAN_POINT('Ctrl Pts',(46.4437670965851,0.528444986286493,4.05487069989181));
#89242=CARTESIAN_POINT('Ctrl Pts',(46.6426143153247,-3.12525822365519,2.63704426391929));
#89243=CARTESIAN_POINT('Ctrl Pts',(46.8414615340643,-3.90816338308783,-1.20312115897968));
#89244=CARTESIAN_POINT('Ctrl Pts',(47.0403087528041,-1.10110939824789,-3.93811622488528));
#89245=CARTESIAN_POINT('Ctrl Pts',(47.2391559715436,2.71740056930501,-3.0556534833461));
#89246=CARTESIAN_POINT('Ctrl Pts',(47.4380031902834,4.03976309623561,0.63369888083219));
#89247=CARTESIAN_POINT('Ctrl Pts',(47.6368504090229,1.65127991561411,3.74089312665609));
#89248=CARTESIAN_POINT('Ctrl Pts',(47.8356976277626,-2.25403124795064,3.41188535546605));
#89249=CARTESIAN_POINT('Ctrl Pts',(48.0345448465023,-4.08884298858149,-0.051412843662276));
#89250=CARTESIAN_POINT('Ctrl Pts',(48.2333920652418,-2.16771289967819,-3.46709701753122));
#89251=CARTESIAN_POINT('Ctrl Pts',(48.4322392839815,1.74460631434076,-3.69871777107951));
#89252=CARTESIAN_POINT('Ctrl Pts',(48.6310865027212,4.05441876366472,-0.531354089049278));
#89253=CARTESIAN_POINT('Ctrl Pts',(48.8299337214608,2.63982261759276,3.12138220342728));
#89254=CARTESIAN_POINT('Ctrl Pts',(49.0287809402005,-1.19945178147874,3.91213073689135));
#89255=CARTESIAN_POINT('Ctrl Pts',(49.2276281589401,-3.93744494621396,1.09879031982473));
#89256=CARTESIAN_POINT('Ctrl Pts',(49.3601929714332,-3.35034815551191,-1.43376273628772));
#89257=CARTESIAN_POINT('Ctrl Pts',(49.4264753776797,-2.5856437469894,-2.29522609227205));
#89258=CARTESIAN_POINT('Ctrl Pts',(0.44936851077589,-1.6436277398265,3.31119802764001));
#89259=CARTESIAN_POINT('Ctrl Pts',(0.515650917022438,-2.74682525825521,
2.76358775828697));
#89260=CARTESIAN_POINT('Ctrl Pts',(0.648215729515534,-4.34346109527289,
0.488246864928335));
#89261=CARTESIAN_POINT('Ctrl Pts',(0.847062948255177,-2.75638393167717,
-3.39760207044552));
#89262=CARTESIAN_POINT('Ctrl Pts',(1.04591016699482,1.36634589630823,-4.15188406410229));
#89263=CARTESIAN_POINT('Ctrl Pts',(1.24475738573446,4.23208193750849,-1.09761842045847));
#89264=CARTESIAN_POINT('Ctrl Pts',(1.44360460447411,3.21130160681502,2.96763287298708));
#89265=CARTESIAN_POINT('Ctrl Pts',(1.64245182321375,-0.759830327539506,
4.30545048291438));
#89266=CARTESIAN_POINT('Ctrl Pts',(1.8412990419534,-4.03272816406958,1.68911495058811));
#89267=CARTESIAN_POINT('Ctrl Pts',(2.04014626069303,-3.60138536803899,-2.47919662769191));
#89268=CARTESIAN_POINT('Ctrl Pts',(2.23899347943268,0.138189912745784,-4.36996528779138));
#89269=CARTESIAN_POINT('Ctrl Pts',(2.43784069817232,3.75078827918065,-2.24667978232544));
#89270=CARTESIAN_POINT('Ctrl Pts',(2.63668791691197,3.91800946186683,1.94041540936253));
#89271=CARTESIAN_POINT('Ctrl Pts',(2.83553513565161,0.486216870884996,4.34505565556579));
#89272=CARTESIAN_POINT('Ctrl Pts',(3.03438235439126,-3.39219908361218,2.75843196049844));
#89273=CARTESIAN_POINT('Ctrl Pts',(3.2332295731309,-4.1546133001462,-1.36203879254129));
#89274=CARTESIAN_POINT('Ctrl Pts',(3.43207679187054,-1.10068331706675,-4.23136444897295));
#89275=CARTESIAN_POINT('Ctrl Pts',(3.63092401061018,2.96431103573806,-3.21384754560735));
#89276=CARTESIAN_POINT('Ctrl Pts',(3.82977122934983,4.30635038585737,0.75584503370213));
#89277=CARTESIAN_POINT('Ctrl Pts',(4.02861844808948,1.6926642442166,4.03123325026437));
#89278=CARTESIAN_POINT('Ctrl Pts',(4.22746566682911,-2.47586849696874,3.60361346648852));
#89279=CARTESIAN_POINT('Ctrl Pts',(4.42631288556876,-4.37011919729062,-0.134212013442915));
#89280=CARTESIAN_POINT('Ctrl Pts',(4.6251601043084,-2.25006786542551,-3.74875300154117));
#89281=CARTESIAN_POINT('Ctrl Pts',(4.82400732304805,1.93684971380027,-3.91976629520431));
#89282=CARTESIAN_POINT('Ctrl Pts',(5.02285454178769,4.34461681789642,-0.490162517511296));
#89283=CARTESIAN_POINT('Ctrl Pts',(5.22170176052733,2.76150787952927,3.38969449891865));
#89284=CARTESIAN_POINT('Ctrl Pts',(5.42054897926698,-1.35826564340401,4.15584757051117));
#89285=CARTESIAN_POINT('Ctrl Pts',(5.61939619800662,-4.23036416261854,1.10452416566391));
#89286=CARTESIAN_POINT('Ctrl Pts',(5.81824341674627,-3.21653679254611,-2.96139251713847));
#89287=CARTESIAN_POINT('Ctrl Pts',(6.01709063548591,0.751935405282821,-4.30703467920225));
#89288=CARTESIAN_POINT('Ctrl Pts',(6.21593785422555,4.02969513842899,-1.69632298568797));
#89289=CARTESIAN_POINT('Ctrl Pts',(6.41478507296519,3.60585943906238,2.47259626423985));
#89290=CARTESIAN_POINT('Ctrl Pts',(6.61363229170484,-0.13024489872292,4.37023922079874));
#89291=CARTESIAN_POINT('Ctrl Pts',(6.81247951044448,-3.74670893977377,2.25346992460214));
#89292=CARTESIAN_POINT('Ctrl Pts',(7.01132672918414,-3.92152287536647,-1.93329069682433));
#89293=CARTESIAN_POINT('Ctrl Pts',(7.21017394792375,-0.494106204195895,
-4.34417007488025));
#89294=CARTESIAN_POINT('Ctrl Pts',(7.40902116666343,3.38718630764454,-2.76458378382463));
#89295=CARTESIAN_POINT('Ctrl Pts',(7.60786838540304,4.15707884146084,1.35449255677521));
#89296=CARTESIAN_POINT('Ctrl Pts',(7.80671560414271,1.10836388186483,4.2293597725739));
#89297=CARTESIAN_POINT('Ctrl Pts',(8.00556282288234,-2.95847144208599,3.21922371183582));
#89298=CARTESIAN_POINT('Ctrl Pts',(8.20441004162199,-4.30771548411879,-0.748025326020356));
#89299=CARTESIAN_POINT('Ctrl Pts',(8.40325726036163,-1.69998029759137,-4.02815361776172));
#89300=CARTESIAN_POINT('Ctrl Pts',(8.60210447910126,2.46932197741505,-3.60810248639643));
#89301=CARTESIAN_POINT('Ctrl Pts',(8.80095169784093,4.37035565174856,0.12627770078113));
#89302=CARTESIAN_POINT('Ctrl Pts',(8.99979891658055,2.25687012230786,3.74466177798734));
#89303=CARTESIAN_POINT('Ctrl Pts',(9.19864613532021,-1.92973008437983,3.92327623064252));
#89304=CARTESIAN_POINT('Ctrl Pts',(9.39749335405985,-4.34371975335436,0.498049480277108));
#89305=CARTESIAN_POINT('Ctrl Pts',(9.59634057279949,-2.76765740935881,-3.38467532341086));
#89306=CARTESIAN_POINT('Ctrl Pts',(9.79518779153912,1.35071835365874,-4.15830668777264));
#89307=CARTESIAN_POINT('Ctrl Pts',(9.99403501027879,4.22835189756562,-1.11220268424345));
#89308=CARTESIAN_POINT('Ctrl Pts',(10.1928822290185,3.22190797828005,2.95554792889247));
#89309=CARTESIAN_POINT('Ctrl Pts',(10.3917294477581,-0.744114630310529,
4.30839273946131));
#89310=CARTESIAN_POINT('Ctrl Pts',(10.5905766664978,-4.02660877778014,1.70363620858125));
#89311=CARTESIAN_POINT('Ctrl Pts',(10.7894238852374,-3.61034256051451,-2.46604565574581));
#89312=CARTESIAN_POINT('Ctrl Pts',(10.988271103977,0.122310398775208,-4.37046848139152));
#89313=CARTESIAN_POINT('Ctrl Pts',(11.1871183227167,3.74261153047214,-2.26026846026354));
#89314=CARTESIAN_POINT('Ctrl Pts',(11.3859655414563,3.92502635299973,1.92616788176494));
#89315=CARTESIAN_POINT('Ctrl Pts',(11.584812760196,0.501992345949099,4.34326585245409));
#89316=CARTESIAN_POINT('Ctrl Pts',(11.7836599789356,-3.38216155008677,2.77072875424496));
#89317=CARTESIAN_POINT('Ctrl Pts',(11.9825071976753,-4.15953110749387,-1.34694303750231));
#89318=CARTESIAN_POINT('Ctrl Pts',(12.1813544164149,-1.11604057012827,-4.22734053824777));
#89319=CARTESIAN_POINT('Ctrl Pts',(12.3802016351546,2.95262198022411,-3.22458958975909));
#89320=CARTESIAN_POINT('Ctrl Pts',(12.5790488538942,4.30906644453736,0.74020332142411));
#89321=CARTESIAN_POINT('Ctrl Pts',(12.7778960726339,1.70729071571528,4.02506061973202));
#89322=CARTESIAN_POINT('Ctrl Pts',(12.9767432913735,-2.46276730196863,3.6125796595839));
#89323=CARTESIAN_POINT('Ctrl Pts',(13.1755905101131,-4.37057770961544,-0.118342995981215));
#89324=CARTESIAN_POINT('Ctrl Pts',(13.3744377288527,-2.26366493567891,-3.74055819891402));
#89325=CARTESIAN_POINT('Ctrl Pts',(13.5732849475924,1.92260409192027,-3.92677324099783));
#89326=CARTESIAN_POINT('Ctrl Pts',(13.772132166332,4.3428083725507,-0.505934797961845));
#89327=CARTESIAN_POINT('Ctrl Pts',(13.9709793850717,2.77379781595364,3.37964498974316));
#89328=CARTESIAN_POINT('Ctrl Pts',(14.1698266038113,-1.3431666114177,4.16075209961586));
#89329=CARTESIAN_POINT('Ctrl Pts',(14.368673822551,-4.22632569545333,1.11987753635658));
#89330=CARTESIAN_POINT('Ctrl Pts',(14.5675210412906,-3.22726854406347,-2.94969359849181));
#89331=CARTESIAN_POINT('Ctrl Pts',(14.7663682600303,0.736291402584172,-4.30973659879184));
#89332=CARTESIAN_POINT('Ctrl Pts',(14.9652154787699,4.02350914489306,-1.71094381598202));
#89333=CARTESIAN_POINT('Ctrl Pts',(15.1640626975095,3.61481378176121,2.45948691878498));
#89334=CARTESIAN_POINT('Ctrl Pts',(15.3629099162492,-0.114375495668469,
4.37068333633034));
#89335=CARTESIAN_POINT('Ctrl Pts',(15.5617571349889,-3.73850178500502,2.26705954575511));
#89336=CARTESIAN_POINT('Ctrl Pts',(15.7606043537285,-3.92851689319731,-1.91903871778258));
#89337=CARTESIAN_POINT('Ctrl Pts',(15.9594515724682,-0.50987683306659,-4.34234731402119));
#89338=CARTESIAN_POINT('Ctrl Pts',(16.1582987912078,3.37712564445375,-2.77686459195583));
#89339=CARTESIAN_POINT('Ctrl Pts',(16.3571460099474,4.16196966313251,1.33938907851674));
#89340=CARTESIAN_POINT('Ctrl Pts',(16.555993228687,1.12371357976661,4.22530737001858));
#89341=CARTESIAN_POINT('Ctrl Pts',(16.7548404474267,-2.94676278610879,3.22994483898557));
#89342=CARTESIAN_POINT('Ctrl Pts',(16.9536876661663,-4.31040320167247,-0.732378877014406));
#89343=CARTESIAN_POINT('Ctrl Pts',(17.152534884906,-1.71459550637115,-4.02195435454171));
#89344=CARTESIAN_POINT('Ctrl Pts',(17.3513821036456,2.45620450889799,-3.61704492520543));
#89345=CARTESIAN_POINT('Ctrl Pts',(17.5502293223853,4.37078536144919,0.110407901106263));
#89346=CARTESIAN_POINT('Ctrl Pts',(17.7490765411249,2.27045228769491,3.73644229043969));
#89347=CARTESIAN_POINT('Ctrl Pts',(17.9479237598646,-1.91547176228979,3.93025730816134));
#89348=CARTESIAN_POINT('Ctrl Pts',(18.1467709786042,-4.34188267724551,0.513818448014967));
#89349=CARTESIAN_POINT('Ctrl Pts',(18.3456181973439,-2.77992907972437,-3.37460351629462));
#89350=CARTESIAN_POINT('Ctrl Pts',(18.5444654160835,1.33561044191232,-4.16318379704042));
#89351=CARTESIAN_POINT('Ctrl Pts',(18.7433126348231,4.22428556278263,-1.12754869719732));
#89352=CARTESIAN_POINT('Ctrl Pts',(18.9421598535628,3.23261847232007,2.94382954549006));
#89353=CARTESIAN_POINT('Ctrl Pts',(19.1410070723024,-0.728465747938811,
4.31106625262998));
#89354=CARTESIAN_POINT('Ctrl Pts',(19.3398542910421,-4.02039624995918,1.71824578387354));
#89355=CARTESIAN_POINT('Ctrl Pts',(19.5387015097817,-3.619273088078,-2.45292007501254));
#89356=CARTESIAN_POINT('Ctrl Pts',(19.7375487285213,0.106440215564113,-4.37088378488787));
#89357=CARTESIAN_POINT('Ctrl Pts',(19.936395947261,3.73437971691508,-2.27384315870254));
#89358=CARTESIAN_POINT('Ctrl Pts',(20.1352431660006,3.93199448445579,1.91190322838119));
#89359=CARTESIAN_POINT('Ctrl Pts',(20.3340903847403,0.517759639558971,4.34141446260651));
#89360=CARTESIAN_POINT('Ctrl Pts',(20.5329376034799,-3.37207860734407,2.78299127673401));
#89361=CARTESIAN_POINT('Ctrl Pts',(20.7317848222196,-4.16439450033916,-1.33183070471814));
#89362=CARTESIAN_POINT('Ctrl Pts',(20.9306320409592,-1.13138288548842,-4.22326027458752));
#89363=CARTESIAN_POINT('Ctrl Pts',(21.1294792596989,2.94089387905273,-3.23528944186379));
#89364=CARTESIAN_POINT('Ctrl Pts',(21.3283264784385,4.31172575111801,0.724552018581892));
#89365=CARTESIAN_POINT('Ctrl Pts',(21.5271736971781,1.72189464548128,4.01883483242943));
#89366=CARTESIAN_POINT('Ctrl Pts',(21.7260209159178,-2.44963361983509,3.62149826854283));
#89367=CARTESIAN_POINT('Ctrl Pts',(21.9248681346574,-4.37097860656534,-0.102472442311512));
#89368=CARTESIAN_POINT('Ctrl Pts',(22.1237153533971,-2.27723215598379,-3.73231406613089));
#89369=CARTESIAN_POINT('Ctrl Pts',(22.3225625721367,1.90833311899741,-3.93372842064914));
#89370=CARTESIAN_POINT('Ctrl Pts',(22.5214097908764,4.34094267049002,-0.521700404450909));
#89371=CARTESIAN_POINT('Ctrl Pts',(22.720257009616,2.78605118046146,3.3695509196827));
#89372=CARTESIAN_POINT('Ctrl Pts',(22.9191042283557,-1.32804987004886,4.16560177203107));
#89373=CARTESIAN_POINT('Ctrl Pts',(23.1179514470953,-4.2222315062781,1.13521614148041));
#89374=CARTESIAN_POINT('Ctrl Pts',(23.3167986658349,-3.23795774541576,-2.93795578921591));
#89375=CARTESIAN_POINT('Ctrl Pts',(23.5156458845746,0.720637692168774,-4.31238169659305));
#89376=CARTESIAN_POINT('Ctrl Pts',(23.7144931033142,4.01727010323906,-1.72554208818758));
#89377=CARTESIAN_POINT('Ctrl Pts',(23.9133403220539,3.62372046476637,2.44634514607375));
#89378=CARTESIAN_POINT('Ctrl Pts',(24.1121875407935,-0.098504584618038,
4.37106982640343));
#89379=CARTESIAN_POINT('Ctrl Pts',(24.3110347595331,-3.73024533978929,2.280619276746));
#89380=CARTESIAN_POINT('Ctrl Pts',(24.5098819782728,-3.93545911531253,-1.90476143708042));
#89381=CARTESIAN_POINT('Ctrl Pts',(24.7087291970124,-0.525640739443385,
-4.3404673012848));
#89382=CARTESIAN_POINT('Ctrl Pts',(24.9075764157521,3.36702045539343,-2.78910878838517));
#89383=CARTESIAN_POINT('Ctrl Pts',(25.1064236344917,4.16680561112128,1.32426794101998));
#89384=CARTESIAN_POINT('Ctrl Pts',(25.3052708532314,1.13904846201456,4.22119925870213));
#89385=CARTESIAN_POINT('Ctrl Pts',(25.504118071971,-2.93501527840068,3.24062338077717));
#89386=CARTESIAN_POINT('Ctrl Pts',(25.7029652907107,-4.31303408851464,-0.716722771924983));
#89387=CARTESIAN_POINT('Ctrl Pts',(25.9018125094503,-1.72918810898676,-4.01570206367753));
#89388=CARTESIAN_POINT('Ctrl Pts',(26.1006597281899,2.44305465643839,-3.62593967491736));
#89389=CARTESIAN_POINT('Ctrl Pts',(26.2995069469296,4.37115744432694,0.0945366457532685));
#89390=CARTESIAN_POINT('Ctrl Pts',(26.4983541656693,2.28400451819822,3.72817353959486));
#89391=CARTESIAN_POINT('Ctrl Pts',(26.6972013844089,-1.90118818557316,3.93718656701993));
#89392=CARTESIAN_POINT('Ctrl Pts',(26.8960486031485,-4.33998835538258,0.529580641289662));
#89393=CARTESIAN_POINT('Ctrl Pts',(27.0948958218882,-2.79216409798571,-3.36448721656139));
#89394=CARTESIAN_POINT('Ctrl Pts',(27.2937430406278,1.32048492074795,-4.16800601661785));
#89395=CARTESIAN_POINT('Ctrl Pts',(27.4925902593675,4.2201635327102,-1.1428798439329));
#89396=CARTESIAN_POINT('Ctrl Pts',(27.6914374781071,3.24328634575149,2.93207234903013));
#89397=CARTESIAN_POINT('Ctrl Pts',(27.8902846968467,-0.71280726107655,4.31368292634515));
#89398=CARTESIAN_POINT('Ctrl Pts',(28.0891319155864,-4.01413071503691,1.7328327048744));
#89399=CARTESIAN_POINT('Ctrl Pts',(28.287979134326,-3.62815589716714,-2.43976215364049));
#89400=CARTESIAN_POINT('Ctrl Pts',(28.4868263530657,0.0905686289870616,
-4.37124146026373));
#89401=CARTESIAN_POINT('Ctrl Pts',(28.6856735718053,3.72609866725499,-2.28738787755066));
#89402=CARTESIAN_POINT('Ctrl Pts',(28.884520790545,3.93891077434772,1.89761336742039));
#89403=CARTESIAN_POINT('Ctrl Pts',(29.0833680092846,0.533520106742824,4.33950583317804));
#89404=CARTESIAN_POINT('Ctrl Pts',(29.2822152280243,-3.36195120527411,2.79521710674521));
#89405=CARTESIAN_POINT('Ctrl Pts',(29.4810624467639,-4.16920298753154,-1.31670081235005));
#89406=CARTESIAN_POINT('Ctrl Pts',(29.6799096655036,-1.14671028407833,-4.21912432915579));
#89407=CARTESIAN_POINT('Ctrl Pts',(29.8787568842432,2.92912700352929,-3.24594663814438));
#89408=CARTESIAN_POINT('Ctrl Pts',(30.0776041029828,4.31432820954993,0.708891162849975));
#89409=CARTESIAN_POINT('Ctrl Pts',(30.2764513217225,1.73647587284724,4.01255605861208));
#89410=CARTESIAN_POINT('Ctrl Pts',(30.4752985404621,-2.43646764039318,3.63036912968944));
#89411=CARTESIAN_POINT('Ctrl Pts',(30.6741457592018,-4.37132187414452,-0.086600537589134));
#89412=CARTESIAN_POINT('Ctrl Pts',(30.8729929779414,-2.29076935201543,-3.72402072447939));
#89413=CARTESIAN_POINT('Ctrl Pts',(31.071840196681,1.89403698556779,-3.94063173587515));
#89414=CARTESIAN_POINT('Ctrl Pts',(31.2706874154207,4.33901973506879,-0.537459132556749));
#89415=CARTESIAN_POINT('Ctrl Pts',(31.4695346341603,2.79826781214797,3.3594124236214));
#89416=CARTESIAN_POINT('Ctrl Pts',(31.6683818529,-1.31291561894468,4.170396522876));
#89417=CARTESIAN_POINT('Ctrl Pts',(31.8672290716396,-4.21808164889521,1.15053977929429));
#89418=CARTESIAN_POINT('Ctrl Pts',(32.0660762903793,-3.2486042557636,-2.92617924432523));
#89419=CARTESIAN_POINT('Ctrl Pts',(32.2649235091189,0.704974480472183,-4.31496993759728));
#89420=CARTESIAN_POINT('Ctrl Pts',(32.4637707278585,4.01097809570062,-1.7401176099032));
#89421=CARTESIAN_POINT('Ctrl Pts',(32.6626179465982,3.63257937066049,2.43317111941123));
#89422=CARTESIAN_POINT('Ctrl Pts',(32.8614651653378,-0.0826323748293277,
4.37139868590308));
#89423=CARTESIAN_POINT('Ctrl Pts',(33.0603123840775,-3.72193971298034,2.29414893880605));
#89424=CARTESIAN_POINT('Ctrl Pts',(33.2591596028171,-3.94234945018409,-1.8904590429624));
#89425=CARTESIAN_POINT('Ctrl Pts',(33.4580068215568,-0.541397715485528,
-4.3385300614554));
#89426=CARTESIAN_POINT('Ctrl Pts',(33.6568540402964,3.35687087369524,-2.80131621168008));
#89427=CARTESIAN_POINT('Ctrl Pts',(33.8557012590361,4.17158662166775,1.30912934365088));
#89428=CARTESIAN_POINT('Ctrl Pts',(34.0545484777757,1.15436832642516,4.21703549278773));
#89429=CARTESIAN_POINT('Ctrl Pts',(34.2533956965153,-2.9232290738471,3.25125919641916));
#89430=CARTESIAN_POINT('Ctrl Pts',(34.452242915255,-4.3156081099583,-0.701057217170789));
#89431=CARTESIAN_POINT('Ctrl Pts',(34.6510901339946,-1.74375791304135,-4.00939682760275));
#89432=CARTESIAN_POINT('Ctrl Pts',(34.8499373527343,2.42987259341109,-3.63478661825904));
#89433=CARTESIAN_POINT('Ctrl Pts',(35.0487845714739,4.3714718954761,0.0786641439775557));
#89434=CARTESIAN_POINT('Ctrl Pts',(35.2476317902135,2.29752663513765,3.71985563447269));
#89435=CARTESIAN_POINT('Ctrl Pts',(35.4464790089532,-1.88687954255259,3.94406391585908));
#89436=CARTESIAN_POINT('Ctrl Pts',(35.6453262276928,-4.33803681274136,0.545335852283642));
#89437=CARTESIAN_POINT('Ctrl Pts',(35.8441734464325,-2.80436230282958,-3.35432655758999));
#89438=CARTESIAN_POINT('Ctrl Pts',(36.0430206651721,1.30534198958868,-4.17277328292609));
#89439=CARTESIAN_POINT('Ctrl Pts',(36.2418678839118,4.21598586169539,-1.15819592231613));
#89440=CARTESIAN_POINT('Ctrl Pts',(36.4407151026514,3.25391145792333,2.92027649452588));
#89441=CARTESIAN_POINT('Ctrl Pts',(36.639562321391,-0.697139376173743,4.31624272610719));
#89442=CARTESIAN_POINT('Ctrl Pts',(36.8384095401307,-4.00781225562154,1.74739677926192));
#89443=CARTESIAN_POINT('Ctrl Pts',(37.0372567588703,-3.63699087066615,-2.42657206511082));
#89444=CARTESIAN_POINT('Ctrl Pts',(37.23610397761,0.0746958483036821,-4.37154150280327));
#89445=CARTESIAN_POINT('Ctrl Pts',(37.4349511963496,3.71776849067378,-2.30090243822691));
#89446=CARTESIAN_POINT('Ctrl Pts',(37.6337984150893,3.94577513148733,1.88329848728799));
#89447=CARTESIAN_POINT('Ctrl Pts',(37.8326456338289,0.549273539705922,4.33753998933313));
#89448=CARTESIAN_POINT('Ctrl Pts',(38.0314928525686,-3.35177947740222,2.80740608308638));
#89449=CARTESIAN_POINT('Ctrl Pts',(38.2303400713082,-4.17395650567318,-1.30155355987898));
#89450=CARTESIAN_POINT('Ctrl Pts',(38.4291872900478,-1.16202256381311,-4.21493275648311));
#89451=CARTESIAN_POINT('Ctrl Pts',(38.6280345087875,2.91732150879461,-3.25656103809055));
#89452=CARTESIAN_POINT('Ctrl Pts',(38.8268817275271,4.31687378552097,0.693220960709451));
#89453=CARTESIAN_POINT('Ctrl Pts',(39.0257289462668,1.75103420556635,4.00622438106276));
#89454=CARTESIAN_POINT('Ctrl Pts',(39.2245761650064,-2.4232695372303,3.63919212606545));
#89455=CARTESIAN_POINT('Ctrl Pts',(39.4234233837461,-4.37160750782718,-0.0707274910778739));
#89456=CARTESIAN_POINT('Ctrl Pts',(39.6222706024857,-2.30427634529205,-3.71567828330342));
#89457=CARTESIAN_POINT('Ctrl Pts',(39.8211178212254,1.87971588011944,-3.94748309565882));
#89458=CARTESIAN_POINT('Ctrl Pts',(40.0199650399649,4.33703959164013,-0.553210774507616));
#89459=CARTESIAN_POINT('Ctrl Pts',(40.2188122587047,2.81044754994229,3.34922963523084));
#89460=CARTESIAN_POINT('Ctrl Pts',(40.4176594774443,-1.29776405764359,4.175136288934));
#89461=CARTESIAN_POINT('Ctrl Pts',(40.6165066961839,-4.2138761780187,1.16584824776282));
#89462=CARTESIAN_POINT('Ctrl Pts',(40.8153539149236,-3.25920793473749,-2.9143641190883));
#89463=CARTESIAN_POINT('Ctrl Pts',(41.0142011336632,0.689301974006816,-4.31750128767965));
#89464=CARTESIAN_POINT('Ctrl Pts',(41.2130483524029,4.00463320523487,-1.75467018895728));
#89465=CARTESIAN_POINT('Ctrl Pts',(41.4118955711425,3.64139038264304,2.41996501249082));
#89466=CARTESIAN_POINT('Ctrl Pts',(41.6107427898821,-0.0667590755701654,
4.37166991049355));
#89467=CARTESIAN_POINT('Ctrl Pts',(41.8095900086218,-3.71358501408416,2.30764835355263));
#89468=CARTESIAN_POINT('Ctrl Pts',(42.0084372273614,-3.94918780696598,-1.87613172399901));
#89469=CARTESIAN_POINT('Ctrl Pts',(42.2072844461011,-0.55714755344433,-4.33653562007506));
#89470=CARTESIAN_POINT('Ctrl Pts',(42.4061316648407,3.34667703317699,-2.81348670089032));
#89471=CARTESIAN_POINT('Ctrl Pts',(42.6049788835804,4.17631263173634,1.29397348600364));
#89472=CARTESIAN_POINT('Ctrl Pts',(42.80382610232,1.16967297101287,4.21281612717571));
#89473=CARTESIAN_POINT('Ctrl Pts',(43.0026733210597,-2.91140432784414,3.26185214567742));
#89474=CARTESIAN_POINT('Ctrl Pts',(43.2015205397993,-4.31812523206573,-0.685382419284583));
#89475=CARTESIAN_POINT('Ctrl Pts',(43.4003677585389,-1.75830472643935,-4.0030387294694));
#89476=CARTESIAN_POINT('Ctrl Pts',(43.5992149772786,2.41665849361697,-3.64358563854853));
#89477=CARTESIAN_POINT('Ctrl Pts',(43.7980621960182,4.37172871074799,0.0627906049760806));
#89478=CARTESIAN_POINT('Ctrl Pts',(43.9969094147579,2.31101846023572,3.71148868488351));
#89479=CARTESIAN_POINT('Ctrl Pts',(44.1957566334975,-1.87254602189098,3.95088926373123));
#89480=CARTESIAN_POINT('Ctrl Pts',(44.3946038522372,-4.33602807503263,0.561083873793988));
#89481=CARTESIAN_POINT('Ctrl Pts',(44.5934510709768,-2.81652353346547,-3.34412167434298));
#89482=CARTESIAN_POINT('Ctrl Pts',(44.7922982897164,1.29018184815828,-4.17748553119992));
#89483=CARTESIAN_POINT('Ctrl Pts',(44.9911455084561,4.21175260468309,-1.17349673406733));
#89484=CARTESIAN_POINT('Ctrl Pts',(45.1899927271957,3.26449366900808,2.9084421444949));
#89485=CARTESIAN_POINT('Ctrl Pts',(45.3888399459354,-0.68146230030182,4.31874560478523));
#89486=CARTESIAN_POINT('Ctrl Pts',(45.587687164675,-4.00144095406779,1.76193784061454));
#89487=CARTESIAN_POINT('Ctrl Pts',(45.7865343834146,-3.64577789390988,-2.41335003230316));
#89488=CARTESIAN_POINT('Ctrl Pts',(45.9853816021543,0.0588220862714005,
-4.37178381485786));
#89489=CARTESIAN_POINT('Ctrl Pts',(46.184228820894,3.70938929033966,-2.31438684179189));
#89490=CARTESIAN_POINT('Ctrl Pts',(46.3830760396336,3.95258747811502,1.86895911963132));
#89491=CARTESIAN_POINT('Ctrl Pts',(46.5819232583732,0.565019706366512,4.33551630096333));
#89492=CARTESIAN_POINT('Ctrl Pts',(46.7807704771129,-3.34156351119619,2.81955930010015));
#89493=CARTESIAN_POINT('Ctrl Pts',(46.9796176958525,-4.17865508132162,-1.28639154805351));
#89494=CARTESIAN_POINT('Ctrl Pts',(47.1784649145922,-1.17731935210033,-4.21068101839448));
#89495=CARTESIAN_POINT('Ctrl Pts',(47.3773121333318,2.90547722391826,-3.26714128948564));
#89496=CARTESIAN_POINT('Ctrl Pts',(47.5761593520715,4.31936307025197,0.67755843061133));
#89497=CARTESIAN_POINT('Ctrl Pts',(47.7750065708111,1.76556825641542,3.99980772043163));
#89498=CARTESIAN_POINT('Ctrl Pts',(47.9738537895506,-2.41003719764277,3.6480286722917));
#89499=CARTESIAN_POINT('Ctrl Pts',(48.1727010082905,-4.37183987877779,-0.0549712280056266));
#89500=CARTESIAN_POINT('Ctrl Pts',(48.37154822703,-2.31774458618709,-3.70706164241665));
#89501=CARTESIAN_POINT('Ctrl Pts',(48.5703954457697,1.86535395932356,-3.95471332528694));
#89502=CARTESIAN_POINT('Ctrl Pts',(48.7692426645094,4.33503308533832,-0.56813015387093));
#89503=CARTESIAN_POINT('Ctrl Pts',(48.9680898832489,2.82252994911284,3.33741922396122));
#89504=CARTESIAN_POINT('Ctrl Pts',(49.1669371019887,-1.28246820569635,4.18289702350915));
#89505=CARTESIAN_POINT('Ctrl Pts',(49.3657843207282,-4.20996327920193,1.17483976568416));
#89506=CARTESIAN_POINT('Ctrl Pts',(49.4983491332213,-3.58223236132085,-1.53299628396422));
#89507=CARTESIAN_POINT('Ctrl Pts',(49.5646315394679,-2.76460125198451,-2.45408321841374));
#89508=CARTESIAN_POINT('Ctrl Pts',(0.587524672564003,-1.75002265636256,
3.52553770398425));
#89509=CARTESIAN_POINT('Ctrl Pts',(0.65380707881055,-2.92463209188894,2.94247965805119));
#89510=CARTESIAN_POINT('Ctrl Pts',(0.786371891303646,-4.62462097686364,
0.519851943854744));
#89511=CARTESIAN_POINT('Ctrl Pts',(0.985219110043291,-2.93480951506551,
-3.61753483255978));
#89512=CARTESIAN_POINT('Ctrl Pts',(1.18406632878293,1.45479187107165,-4.42064282727201));
#89513=CARTESIAN_POINT('Ctrl Pts',(1.38291354752258,4.50603205017953,-1.16866919272471));
#89514=CARTESIAN_POINT('Ctrl Pts',(1.58176076626222,3.41917481201227,3.15973297216424));
#89515=CARTESIAN_POINT('Ctrl Pts',(1.78060798500187,-0.80901548201296,4.58414987066494));
#89516=CARTESIAN_POINT('Ctrl Pts',(1.97945520374151,-4.29377375610484,1.79845433433831));
#89517=CARTESIAN_POINT('Ctrl Pts',(2.17830242248115,-3.83450938168383,-2.63967938901811));
#89518=CARTESIAN_POINT('Ctrl Pts',(2.3771496412208,0.147135189024952,-4.65284083241367));
#89519=CARTESIAN_POINT('Ctrl Pts',(2.57599685996044,3.99358340622675,-2.39211131899973));
#89520=CARTESIAN_POINT('Ctrl Pts',(2.77484407870008,4.17162911039287,2.06602191412145));
#89521=CARTESIAN_POINT('Ctrl Pts',(2.97369129743973,0.517690544724007,4.62631875585088));
#89522=CARTESIAN_POINT('Ctrl Pts',(3.17253851617937,-3.61178210087895,2.93699011639711));
#89523=CARTESIAN_POINT('Ctrl Pts',(3.37138573491902,-4.42354873156875,-1.45020596089697));
#89524=CARTESIAN_POINT('Ctrl Pts',(3.57023295365865,-1.17193248548496,-4.50526811734826));
#89525=CARTESIAN_POINT('Ctrl Pts',(3.7690801723983,3.15619610654337,-3.42188555390371));
#89526=CARTESIAN_POINT('Ctrl Pts',(3.96792739113794,4.58510802590933,0.804772213091007));
#89527=CARTESIAN_POINT('Ctrl Pts',(4.16677460987759,1.80223337999047,4.29218207389783));
#89528=CARTESIAN_POINT('Ctrl Pts',(4.36562182861723,-2.63613582253541,3.83688170886766));
#89529=CARTESIAN_POINT('Ctrl Pts',(4.56446904735687,-4.65300470474569,-0.142899793298736));
#89530=CARTESIAN_POINT('Ctrl Pts',(4.76331626609652,-2.39571871868222,-3.99141638148338));
#89531=CARTESIAN_POINT('Ctrl Pts',(4.96216348483616,2.06222540480949,-4.17349966664448));
#89532=CARTESIAN_POINT('Ctrl Pts',(5.1610107035758,4.62585151144676,-0.521891600001131));
#89533=CARTESIAN_POINT('Ctrl Pts',(5.35985792231545,2.9402651450807,3.60911539000991));
#89534=CARTESIAN_POINT('Ctrl Pts',(5.5587051410551,-1.44618856917494,4.42486289842688));
#89535=CARTESIAN_POINT('Ctrl Pts',(5.75755235979473,-4.50420308069752,1.17602195897205));
#89536=CARTESIAN_POINT('Ctrl Pts',(5.95639957853438,-3.42474888053015,-3.15308866709796));
#89537=CARTESIAN_POINT('Ctrl Pts',(6.15524679727402,0.800609507542814,-4.58583661476685));
#89538=CARTESIAN_POINT('Ctrl Pts',(6.35409401601367,4.29054439737612,-1.806128958237));
#89539=CARTESIAN_POINT('Ctrl Pts',(6.55294123475331,3.83927306719934,2.63265177242256));
#89540=CARTESIAN_POINT('Ctrl Pts',(6.75178845349296,-0.138675880260429,
4.65313249758675));
#89541=CARTESIAN_POINT('Ctrl Pts',(6.95063567223259,-3.98924000400005,2.3993409991373));
#89542=CARTESIAN_POINT('Ctrl Pts',(7.14948289097224,-4.17536995333229,-2.0584360064005));
#89543=CARTESIAN_POINT('Ctrl Pts',(7.34833010971188,-0.526090568466078,
-4.62537584996885));
#89544=CARTESIAN_POINT('Ctrl Pts',(7.54717732845153,3.60644483909998,-2.94354015807498));
#89545=CARTESIAN_POINT('Ctrl Pts',(7.74602454719117,4.42617387171228,1.44217124400768));
#89546=CARTESIAN_POINT('Ctrl Pts',(7.94487176593082,1.18011022676091,4.50313367471746));
#89547=CARTESIAN_POINT('Ctrl Pts',(8.14371898467045,-3.14997850571596,3.42760972883471));
#89548=CARTESIAN_POINT('Ctrl Pts',(8.3425662034101,-4.58656148938392,-0.796446321967582));
#89549=CARTESIAN_POINT('Ctrl Pts',(8.54141342214974,-1.81002301437711,-4.28890309136285));
#89550=CARTESIAN_POINT('Ctrl Pts',(8.74026064088939,2.62916553524853,-3.84166131093529));
#89551=CARTESIAN_POINT('Ctrl Pts',(8.93910785962903,4.65325646531687,0.134451878613232));
#89552=CARTESIAN_POINT('Ctrl Pts',(9.13795507836867,2.40296129762516,3.98706032582799));
#89553=CARTESIAN_POINT('Ctrl Pts',(9.33680229710831,-2.05464490924545,4.17723680638143));
#89554=CARTESIAN_POINT('Ctrl Pts',(9.53564951584797,-4.62489637833799,0.530289099748558));
#89555=CARTESIAN_POINT('Ctrl Pts',(9.73449673458759,-2.94681274479986,-3.6037713144373));
#89556=CARTESIAN_POINT('Ctrl Pts',(9.93334395332725,1.43815273008053,-4.42748119867695));
#89557=CARTESIAN_POINT('Ctrl Pts',(10.1321911720669,4.50206055818595,-1.18419752157415));
#89558=CARTESIAN_POINT('Ctrl Pts',(10.3310383908065,3.43046775257043,3.14686574836777));
#89559=CARTESIAN_POINT('Ctrl Pts',(10.5298856095462,-0.792282480041272,
4.58728258465681));
#89560=CARTESIAN_POINT('Ctrl Pts',(10.7287328282858,-4.28725825117018,1.81391557892011));
#89561=CARTESIAN_POINT('Ctrl Pts',(10.9275800470254,-3.84404638899377,-2.62567713151101));
#89562=CARTESIAN_POINT('Ctrl Pts',(11.1264272657651,0.13022776616565,-4.6533765986212));
#89563=CARTESIAN_POINT('Ctrl Pts',(11.3252744845047,3.9848773621825,-2.40657961597811));
#89564=CARTESIAN_POINT('Ctrl Pts',(11.5241217032444,4.17910021723919,2.0508521189855));
#89565=CARTESIAN_POINT('Ctrl Pts',(11.722968921984,0.534487194055304,4.62441309563352));
#89566=CARTESIAN_POINT('Ctrl Pts',(11.9218161407237,-3.60109482014146,2.95008290324633));
#89567=CARTESIAN_POINT('Ctrl Pts',(12.1206633594633,-4.42878487724183,-1.43413303106441));
#89568=CARTESIAN_POINT('Ctrl Pts',(12.3195105782029,-1.18828384056733,-4.50098373179936));
#89569=CARTESIAN_POINT('Ctrl Pts',(12.5183577969426,3.14375039789217,-3.43332294948041));
#89570=CARTESIAN_POINT('Ctrl Pts',(12.7172050156822,4.5879998998482,0.788117985246376));
#89571=CARTESIAN_POINT('Ctrl Pts',(12.9160522344219,1.81780664873319,4.28560987812672));
#89572=CARTESIAN_POINT('Ctrl Pts',(13.1148994531615,-2.62218656412363,3.84642829942343));
#89573=CARTESIAN_POINT('Ctrl Pts',(13.3137466719012,-4.65349289738031,-0.126003546405802));
#89574=CARTESIAN_POINT('Ctrl Pts',(13.5125938906408,-2.41019595122522,-3.98269111485857));
#89575=CARTESIAN_POINT('Ctrl Pts',(13.7114411093805,2.04705763875159,-4.18096018437209));
#89576=CARTESIAN_POINT('Ctrl Pts',(13.9102883281201,4.62392600225079,-0.538684847925919));
#89577=CARTESIAN_POINT('Ctrl Pts',(14.1091355468597,2.95335063072125,3.59841535841742));
#89578=CARTESIAN_POINT('Ctrl Pts',(14.3079827655994,-1.43011215027247,4.43008490633294));
#89579=CARTESIAN_POINT('Ctrl Pts',(14.506829984339,-4.49990319644462,1.19236918037302));
#89580=CARTESIAN_POINT('Ctrl Pts',(14.7056772030787,-3.43617531721211,-3.14063245685613));
#89581=CARTESIAN_POINT('Ctrl Pts',(14.9045244218183,0.783952841014584,-4.5887134343671));
#89582=CARTESIAN_POINT('Ctrl Pts',(15.1033716405579,4.28395797359069,-1.82169622061));
#89583=CARTESIAN_POINT('Ctrl Pts',(15.3022188592976,3.84880704026154,2.61869383596274));
#89584=CARTESIAN_POINT('Ctrl Pts',(15.5010660780373,-0.12177922281464,4.65360536149839));
#89585=CARTESIAN_POINT('Ctrl Pts',(15.6999132967769,-3.98050158565777,2.41381030038649));
#89586=CARTESIAN_POINT('Ctrl Pts',(15.8987605155165,-4.18281670624742,-2.04326147167056));
#89587=CARTESIAN_POINT('Ctrl Pts',(16.0976077342562,-0.542882057901342,
-4.62343509859117));
#89588=CARTESIAN_POINT('Ctrl Pts',(16.2964549529958,3.59573293147315,-2.95661592453187));
#89589=CARTESIAN_POINT('Ctrl Pts',(16.4953021717355,4.43138128487904,1.42609009101802));
#89590=CARTESIAN_POINT('Ctrl Pts',(16.6941493904751,1.19645353762478,4.49881895301213));
#89591=CARTESIAN_POINT('Ctrl Pts',(16.8929966092148,-3.13751192782905,3.43902485341504));
#89592=CARTESIAN_POINT('Ctrl Pts',(17.0918438279544,-4.58942318762548,-0.77978705077828));
#89593=CARTESIAN_POINT('Ctrl Pts',(17.290691046694,-1.82558429134533,-4.28230253892332));
#89594=CARTESIAN_POINT('Ctrl Pts',(17.4895382654337,2.61519894990641,-3.85118260954792));
#89595=CARTESIAN_POINT('Ctrl Pts',(17.6883854841733,4.65371399088276,0.117554798873092));
#89596=CARTESIAN_POINT('Ctrl Pts',(17.887232702913,2.41742266048359,3.97830877638432));
#89597=CARTESIAN_POINT('Ctrl Pts',(18.0860799216526,-2.03946362087056,4.18466978133538));
#89598=CARTESIAN_POINT('Ctrl Pts',(18.2849271403923,-4.62294038505918,0.547078820522931));
#89599=CARTESIAN_POINT('Ctrl Pts',(18.4837743591319,-2.95987878198744,-3.5930475415191));
#89600=CARTESIAN_POINT('Ctrl Pts',(18.6826215778715,1.42206685661543,-4.43267401181181));
#89601=CARTESIAN_POINT('Ctrl Pts',(18.8814687966112,4.49773100239534,-1.20053690895693));
#89602=CARTESIAN_POINT('Ctrl Pts',(19.0803160153508,3.44187155574113,3.1343888133823));
#89603=CARTESIAN_POINT('Ctrl Pts',(19.2791632340905,-0.775620617970148,
4.5901291590385));
#89604=CARTESIAN_POINT('Ctrl Pts',(19.4780104528301,-4.28064357548876,1.82947085773528));
#89605=CARTESIAN_POINT('Ctrl Pts',(19.6768576715698,-3.853555005325,-2.61170190883465));
#89606=CARTESIAN_POINT('Ctrl Pts',(19.8757048903094,0.1133302780623,-4.65381878544387));
#89607=CARTESIAN_POINT('Ctrl Pts',(20.0745521090491,3.97611268884515,-2.4210330285398));
#89608=CARTESIAN_POINT('Ctrl Pts',(20.2733993277887,4.18651940810897,2.0356640894811));
#89609=CARTESIAN_POINT('Ctrl Pts',(20.4722465465283,0.551275132332437,4.6224418620625));
#89610=CARTESIAN_POINT('Ctrl Pts',(20.671093765268,-3.5903591907681,2.96313920039928));
#89611=CARTESIAN_POINT('Ctrl Pts',(20.8699409840076,-4.43396308606603,-1.41804245038001));
#89612=CARTESIAN_POINT('Ctrl Pts',(21.0687882027473,-1.20461929100464,-4.49663934549075));
#89613=CARTESIAN_POINT('Ctrl Pts',(21.2676354214869,3.13126311608942,-3.44471542184459));
#89614=CARTESIAN_POINT('Ctrl Pts',(21.4664826402265,4.59083134802444,0.771453546023437));
#89615=CARTESIAN_POINT('Ctrl Pts',(21.6653298589662,1.83335591657723,4.27898108465407));
#89616=CARTESIAN_POINT('Ctrl Pts',(21.8641770777058,-2.6082027156291,3.85592422563786));
#89617=CARTESIAN_POINT('Ctrl Pts',(22.0630242964455,-4.65391974509539,-0.10910566386342));
#89618=CARTESIAN_POINT('Ctrl Pts',(22.2618715151851,-2.42464140158001,-3.97391332484995));
#89619=CARTESIAN_POINT('Ctrl Pts',(22.4607187339248,2.03186288063319,-4.18836558504399));
#89620=CARTESIAN_POINT('Ctrl Pts',(22.6595659526644,4.62193953001191,-0.555470989871944));
#89621=CARTESIAN_POINT('Ctrl Pts',(22.858413171404,2.96639717708072,3.58766788143545));
#89622=CARTESIAN_POINT('Ctrl Pts',(23.0572603901437,-1.41401687562795,4.43524850657946));
#89623=CARTESIAN_POINT('Ctrl Pts',(23.2561076088833,-4.49554398319792,1.20870068040387));
#89624=CARTESIAN_POINT('Ctrl Pts',(23.454954827623,-3.44755644938191,-3.12813483852616));
#89625=CARTESIAN_POINT('Ctrl Pts',(23.6538020463626,0.767285838372017,-4.59152975400461));
#89626=CARTESIAN_POINT('Ctrl Pts',(23.8526492651023,4.27731506778913,-1.83723946466974));
#89627=CARTESIAN_POINT('Ctrl Pts',(24.0514964838419,3.85829026853422,2.60470137317316));
#89628=CARTESIAN_POINT('Ctrl Pts',(24.2503437025816,-0.104880959757646,
4.65401686975417));
#89629=CARTESIAN_POINT('Ctrl Pts',(24.4491909213212,-3.97171068621112,2.4282477766308));
#89630=CARTESIAN_POINT('Ctrl Pts',(24.6480381400608,-4.19020831061913,-2.02805999745922));
#89631=CARTESIAN_POINT('Ctrl Pts',(24.8468853588005,-0.559666389683838,
-4.62143338932135));
#89632=CARTESIAN_POINT('Ctrl Pts',(25.0457325775401,3.58497361573888,-2.969652709347));
#89633=CARTESIAN_POINT('Ctrl Pts',(25.2445797962798,4.43653027229285,1.40999013567649));
#89634=CARTESIAN_POINT('Ctrl Pts',(25.4434270150194,1.21278107379143,4.49444491641952));
#89635=CARTESIAN_POINT('Ctrl Pts',(25.6422742337591,-3.1250039832703,3.45039463601204));
#89636=CARTESIAN_POINT('Ctrl Pts',(25.8411214524987,-4.59222437640355,-0.763117498450222));
#89637=CARTESIAN_POINT('Ctrl Pts',(26.0399686712383,-1.84112149881258,-4.27564552626689));
#89638=CARTESIAN_POINT('Ctrl Pts',(26.238815889978,2.60119788435214,-3.86065313206429));
#89639=CARTESIAN_POINT('Ctrl Pts',(26.4376631087176,4.65411015934009,0.10065616922622));
#89640=CARTESIAN_POINT('Ctrl Pts',(26.6365103274573,2.43185215072055,3.96950477474354));
#89641=CARTESIAN_POINT('Ctrl Pts',(26.8353575461969,-2.02425544309264,4.19204758331602));
#89642=CARTESIAN_POINT('Ctrl Pts',(27.0342047649366,-4.62092344040788,0.563861328311218));
#89643=CARTESIAN_POINT('Ctrl Pts',(27.2330519836762,-2.97290579451561,-3.58227639589851));
#89644=CARTESIAN_POINT('Ctrl Pts',(27.4318992024159,1.40596223384379,-4.43780838215003));
#89645=CARTESIAN_POINT('Ctrl Pts',(27.6307464211555,4.49334214606115,-1.21686046780494));
#89646=CARTESIAN_POINT('Ctrl Pts',(27.8295936398951,3.45322997939622,3.12187055290175));
#89647=CARTESIAN_POINT('Ctrl Pts',(28.0284408586348,-0.758948529692909,
4.59291521464886));
#89648=CARTESIAN_POINT('Ctrl Pts',(28.2272880773744,-4.27397246146306,1.84500201580684));
#89649=CARTESIAN_POINT('Ctrl Pts',(28.4261352961141,-3.86301281428105,-2.59769225205302));
#89650=CARTESIAN_POINT('Ctrl Pts',(28.6249825148537,0.0964312957506612,
-4.65419961377633));
#89651=CARTESIAN_POINT('Ctrl Pts',(28.8238297335934,3.96729559226513,-2.43545452087891));
#89652=CARTESIAN_POINT('Ctrl Pts',(29.022676952333,4.19388340161891,2.02044922066884));
#89653=CARTESIAN_POINT('Ctrl Pts',(29.2215241710727,0.568055802296986,4.62040968369177));
#89654=CARTESIAN_POINT('Ctrl Pts',(29.4203713898123,-3.57957622413699,2.9761564299057));
#89655=CARTESIAN_POINT('Ctrl Pts',(29.6192186085519,-4.43908283509774,-1.40193317344891));
#89656=CARTESIAN_POINT('Ctrl Pts',(29.8180658272916,-1.22093885908292,-4.49223567303157));
#89657=CARTESIAN_POINT('Ctrl Pts',(30.0169130460312,3.11873455000258,-3.45606247719805));
#89658=CARTESIAN_POINT('Ctrl Pts',(30.2157602647709,4.59360226817123,0.754778935535434));
#89659=CARTESIAN_POINT('Ctrl Pts',(30.4146074835105,1.84888101245487,4.27229587475631));
#89660=CARTESIAN_POINT('Ctrl Pts',(30.6134547022501,-2.59418447916456,3.86536931324001));
#89661=CARTESIAN_POINT('Ctrl Pts',(30.8123019209898,-4.65428523298917,-0.0922063428123347));
#89662=CARTESIAN_POINT('Ctrl Pts',(31.0111491397294,-2.43905488413748,-3.9650831405963));
#89663=CARTESIAN_POINT('Ctrl Pts',(31.2099963584691,2.01664133332414,-4.19571576401506));
#89664=CARTESIAN_POINT('Ctrl Pts',(31.4088435772087,4.61989211959633,-0.572249808184896));
#89665=CARTESIAN_POINT('Ctrl Pts',(31.6076907959484,2.97940461283869,3.57687310267941));
#89666=CARTESIAN_POINT('Ctrl Pts',(31.806538014688,-1.39790295781212,4.44035363008579));
#89667=CARTESIAN_POINT('Ctrl Pts',(32.0053852334276,-4.49112549824252,1.22501624426447));
#89668=CARTESIAN_POINT('Ctrl Pts',(32.2042324521673,-3.45889212708342,-3.11559597715689));
#89669=CARTESIAN_POINT('Ctrl Pts',(32.403079670907,0.750608719413602,-4.59428553640459));
#89670=CARTESIAN_POINT('Ctrl Pts',(32.6019268896466,4.2706157675282,-1.85275848556028));
#89671=CARTESIAN_POINT('Ctrl Pts',(32.8007741083862,3.86772262699936,2.59067456857727));
#89672=CARTESIAN_POINT('Ctrl Pts',(32.9996213271259,-0.0879813138927531,
4.65436701690806));
#89673=CARTESIAN_POINT('Ctrl Pts',(33.1984685458655,-3.96286742156015,2.44265323752946));
#89674=CARTESIAN_POINT('Ctrl Pts',(33.3973157646052,-4.19754466899455,-2.01283178419641));
#89675=CARTESIAN_POINT('Ctrl Pts',(33.5961629833448,-0.576443342518929,
-4.61937074854807));
#89676=CARTESIAN_POINT('Ctrl Pts',(33.7950102020845,3.57416703375318,-2.982650340638));
#89677=CARTESIAN_POINT('Ctrl Pts',(33.9938574208241,4.44162076606701,1.39387159025436));
#89678=CARTESIAN_POINT('Ctrl Pts',(34.1927046395637,1.22909261998972,4.49001162260886));
#89679=CARTESIAN_POINT('Ctrl Pts',(34.3915518583034,-3.11245483695114,3.46171892672056));
#89680=CARTESIAN_POINT('Ctrl Pts',(34.590399077043,-4.59496501878578,-0.746437884763965));
#89681=CARTESIAN_POINT('Ctrl Pts',(34.7892462957827,-1.85663443192783,-4.26893214116319));
#89682=CARTESIAN_POINT('Ctrl Pts',(34.9880935145223,2.58716252318344,-3.87007275361991));
#89683=CARTESIAN_POINT('Ctrl Pts',(35.1869407332619,4.65444496546559,0.0837562124734973));
#89684=CARTESIAN_POINT('Ctrl Pts',(35.3857879520017,2.44624957808966,3.96064843698251));
#89685=CARTESIAN_POINT('Ctrl Pts',(35.5846351707412,-2.00902057642482,4.1993701150503));
#89686=CARTESIAN_POINT('Ctrl Pts',(35.7834823894809,-4.6188455709766,0.580636401843466));
#89687=CARTESIAN_POINT('Ctrl Pts',(35.9823296082206,-2.98589361062901,-3.57145801958819));
#89688=CARTESIAN_POINT('Ctrl Pts',(36.1811768269602,1.38983907409762,-4.44288424199724));
#89689=CARTESIAN_POINT('Ctrl Pts',(36.3800240456998,4.48889404704846,-1.23316798289963));
#89690=CARTESIAN_POINT('Ctrl Pts',(36.5788712644394,3.46454287378012,3.10931113197366));
#89691=CARTESIAN_POINT('Ctrl Pts',(36.7777184831791,-0.742266435023419,
4.59564071475496));
#89692=CARTESIAN_POINT('Ctrl Pts',(36.9765657019187,-4.26724499704864,1.8605088483636));
#89693=CARTESIAN_POINT('Ctrl Pts',(37.1754129206584,-3.87241969116504,-2.58364834587705));
#89694=CARTESIAN_POINT('Ctrl Pts',(37.374260139398,0.0795310420360833,-4.65451907859756));
#89695=CARTESIAN_POINT('Ctrl Pts',(37.5731073581377,3.95842618869195,-2.44984390285462));
#89696=CARTESIAN_POINT('Ctrl Pts',(37.7719545768773,4.20119210067807,2.00520771314995));
#89697=CARTESIAN_POINT('Ctrl Pts',(37.970801795617,0.584828982703287,4.6183165873147));
#89698=CARTESIAN_POINT('Ctrl Pts',(38.1696490143566,-3.56874606241678,2.98913442013916));
#89699=CARTESIAN_POINT('Ctrl Pts',(38.3684962330963,-4.44414405683533,-1.38580541266483));
#89700=CARTESIAN_POINT('Ctrl Pts',(38.5673434518359,-1.23724232963595,-4.48777277248224));
#89701=CARTESIAN_POINT('Ctrl Pts',(38.7661906705756,3.10616486481495,-3.46736396593507));
#89702=CARTESIAN_POINT('Ctrl Pts',(38.9650378893152,4.59631262375533,0.738094373629349));
#89703=CARTESIAN_POINT('Ctrl Pts',(39.1638851080548,1.86438173167491,4.26555433657488));
#89704=CARTESIAN_POINT('Ctrl Pts',(39.3627323267945,-2.58013203955406,3.87476343770075));
#89705=CARTESIAN_POINT('Ctrl Pts',(39.5615795455341,-4.65458935624285,-0.075305806062374));
#89706=CARTESIAN_POINT('Ctrl Pts',(39.7604267642738,-2.45343620886246,-3.95620067851954));
#89707=CARTESIAN_POINT('Ctrl Pts',(39.9592739830134,2.00139319751365,-4.20301062437656));
#89708=CARTESIAN_POINT('Ctrl Pts',(40.158121201753,4.61778379799829,-0.589021081643585));
#89709=CARTESIAN_POINT('Ctrl Pts',(40.3569684204926,2.99237276649791,3.56603116447367));
#89710=CARTESIAN_POINT('Ctrl Pts',(40.5558156392324,-1.38177060927986,4.44540020954315));
#89711=CARTESIAN_POINT('Ctrl Pts',(40.7546628579719,-4.48664779983415,1.24131565684128));
#89712=CARTESIAN_POINT('Ctrl Pts',(40.9535100767116,-3.47018220086074,-3.10301603806767));
#89713=CARTESIAN_POINT('Ctrl Pts',(41.1523572954513,0.733921704019672,-4.59698074523321));
#89714=CARTESIAN_POINT('Ctrl Pts',(41.3512045141909,4.26386016113502,-1.86825307867041));
#89715=CARTESIAN_POINT('Ctrl Pts',(41.5500517329305,3.87710399129574,2.57661360711193));
#89716=CARTESIAN_POINT('Ctrl Pts',(41.7488989516702,-0.0710805080340738,
4.65465579834364));
#89717=CARTESIAN_POINT('Ctrl Pts',(41.9477461704099,-3.95397190829937,2.4570264931528));
#89718=CARTESIAN_POINT('Ctrl Pts',(42.1465933891494,-4.20482568464708,-1.9975770326591));
#89719=CARTESIAN_POINT('Ctrl Pts',(42.3454406078891,-0.593212695209971,
-4.61724720346677));
#89720=CARTESIAN_POINT('Ctrl Pts',(42.5442878266288,3.56331332799607,-2.995608647036));
#89721=CARTESIAN_POINT('Ctrl Pts',(42.7431350453684,4.44665269908555,1.37773466726589));
#89722=CARTESIAN_POINT('Ctrl Pts',(42.941982264108,1.24538796115919,4.48551913003431));
#89723=CARTESIAN_POINT('Ctrl Pts',(43.1408294828477,-3.09986465432677,3.47299757622888));
#89724=CARTESIAN_POINT('Ctrl Pts',(43.3396767015873,-4.59764507863759,-0.729748429621486));
#89725=CARTESIAN_POINT('Ctrl Pts',(43.538523920327,-1.87212288616081,-4.26216247214683));
#89726=CARTESIAN_POINT('Ctrl Pts',(43.7373711390666,2.5730930514516,-3.87944134997984));
#89727=CARTESIAN_POINT('Ctrl Pts',(43.9362183578062,4.65471840484205,0.0668551513535571));
#89728=CARTESIAN_POINT('Ctrl Pts',(44.1350655765459,2.46061475277319,3.95173988001982));
#89729=CARTESIAN_POINT('Ctrl Pts',(44.3339127952855,-1.99375922174246,4.20663727970347));
#89730=CARTESIAN_POINT('Ctrl Pts',(44.5327600140252,-4.61670680414042,0.59740382050415));
#89731=CARTESIAN_POINT('Ctrl Pts',(44.7316072327648,-2.99884205912885,-3.56059255628707));
#89732=CARTESIAN_POINT('Ctrl Pts',(44.9304544515045,1.37369759002917,-4.44790152239582));
#89733=CARTESIAN_POINT('Ctrl Pts',(45.1293016702441,4.48438676385885,-1.24945924312633));
#89734=CARTESIAN_POINT('Ctrl Pts',(45.3281488889838,3.47581009001405,3.09671072363562));
#89735=CARTESIAN_POINT('Ctrl Pts',(45.5269961077234,-0.725574554437197,
4.59830560917513));
#89736=CARTESIAN_POINT('Ctrl Pts',(45.7258433264631,-4.26046126993124,1.87599117821119));
#89737=CARTESIAN_POINT('Ctrl Pts',(45.9246905452027,-3.8817755138893,-2.56957042761375));
#89738=CARTESIAN_POINT('Ctrl Pts',(46.1235377639424,0.0626297434481601,
-4.65477707593793));
#89739=CARTESIAN_POINT('Ctrl Pts',(46.3223849826819,3.94950458797202,-2.46420117559616));
#89740=CARTESIAN_POINT('Ctrl Pts',(46.5212322014217,4.20844542249333,1.98994013298625));
#89741=CARTESIAN_POINT('Ctrl Pts',(46.7200794201614,0.601594426446524,4.61616190203485));
#89742=CARTESIAN_POINT('Ctrl Pts',(46.9189266389009,-3.55786879873718,3.00207433628102));
#89743=CARTESIAN_POINT('Ctrl Pts',(47.1177738576406,-4.44914677955542,-1.36966193712735));
#89744=CARTESIAN_POINT('Ctrl Pts',(47.3166210763802,-1.25352930595277,-4.48324581190367));
#89745=CARTESIAN_POINT('Ctrl Pts',(47.5154682951199,3.09355387853151,-3.47862909562517));
#89746=CARTESIAN_POINT('Ctrl Pts',(47.7143155138595,4.59896304426834,0.721417980390469));
#89747=CARTESIAN_POINT('Ctrl Pts',(47.9131627325991,1.87985659721673,4.25872231420717));
#89748=CARTESIAN_POINT('Ctrl Pts',(48.1120099513388,-2.5660431473349,3.88417198911736));
#89749=CARTESIAN_POINT('Ctrl Pts',(48.3108571700785,-4.65483676897409,-0.0585296123489751));
#89750=CARTESIAN_POINT('Ctrl Pts',(48.509704388818,-2.46777627269599,-3.94702626730209));
#89751=CARTESIAN_POINT('Ctrl Pts',(48.7085516075577,1.98610160430635,-4.21070887949438));
#89752=CARTESIAN_POINT('Ctrl Pts',(48.9073988262974,4.61564740701194,-0.604906218692581));
#89753=CARTESIAN_POINT('Ctrl Pts',(49.106246045037,3.00523728063291,3.55345624449517));
#89754=CARTESIAN_POINT('Ctrl Pts',(49.3050932637767,-1.36548462991396,4.45366331012696));
#89755=CARTESIAN_POINT('Ctrl Pts',(49.5039404825163,-4.4824816121899,1.25088921154358));
#89756=CARTESIAN_POINT('Ctrl Pts',(49.6365052950094,-3.81411656712978,-1.63222983164071));
#89757=CARTESIAN_POINT('Ctrl Pts',(49.7027877012559,-2.94355875697961,-2.61294034455543));
#89758=CARTESIAN_POINT('Ctrl Pts',(49.291,-0.918523134026602,3.82423904224853));
#89759=CARTESIAN_POINT('Ctrl Pts',(49.291,-0.944497648971282,3.81771905984364));
#89760=CARTESIAN_POINT('Ctrl Pts',(49.291,-0.970472163915961,3.81119907743874));
#89761=CARTESIAN_POINT('Ctrl Pts',(49.291,-0.99644667886064,3.80467909503385));
#89762=CARTESIAN_POINT('Ctrl Pts',(0.585800000000001,-1.87561177831641,
-2.627495997809));
#89763=CARTESIAN_POINT('Ctrl Pts',(0.585800000000003,-1.93432966665696,
-2.59479265455963));
#89764=CARTESIAN_POINT('Ctrl Pts',(0.585800000000004,-1.99185820734684,
-2.56017313445794));
#89765=CARTESIAN_POINT('Ctrl Pts',(0.585800000000003,-2.04809242124784,
-2.52365641141691));
#89766=CARTESIAN_POINT('Ctrl Pts',(0.585800000000001,-2.13571955057025,
-2.4667541202605));
#89767=CARTESIAN_POINT('Ctrl Pts',(0.585800000000001,-2.22020527745289,
-2.40524808224379));
#89768=CARTESIAN_POINT('Ctrl Pts',(0.585800000000002,-2.30145114296921,
-2.33955241913762));
#89769=CARTESIAN_POINT('Ctrl Pts',(0.585800000000003,-2.38269700848554,
-2.27385675603146));
#89770=CARTESIAN_POINT('Ctrl Pts',(0.585800000000001,-2.46070346620059,
-2.20397085949305));
#89771=CARTESIAN_POINT('Ctrl Pts',(0.585800000000001,-2.53534969830284,
-2.13025947000897));
#89772=CARTESIAN_POINT('Ctrl Pts',(0.585800000000001,-2.54871288358938,
-2.11706364045853));
#89773=CARTESIAN_POINT('Ctrl Pts',(0.5858,-2.56196773078561,-2.10374556313248));
#89774=CARTESIAN_POINT('Ctrl Pts',(0.5858,-2.57510436638075,-2.09031685798063));
#89775=CARTESIAN_POINT('Ctrl Pts',(0.585799999999998,-2.6494041349224,-2.01436516720182));
#89776=CARTESIAN_POINT('Ctrl Pts',(0.585799999999997,-2.72000285773494,
-1.93480144575629));
#89777=CARTESIAN_POINT('Ctrl Pts',(0.585799999999998,-2.78679913428153,
-1.85203521699974));
#89778=CARTESIAN_POINT('Ctrl Pts',(0.585799999999999,-2.85526820090954,
-1.76719626003589));
#89779=CARTESIAN_POINT('Ctrl Pts',(0.585799999999998,-2.91974257549655,
-1.67899189202741));
#89780=CARTESIAN_POINT('Ctrl Pts',(0.585799999999997,-2.98008554188355,
-1.58781616186147));
#89781=CARTESIAN_POINT('Ctrl Pts',(0.585799999999997,-3.00023946869769,
-1.5573644107625));
#89782=CARTESIAN_POINT('Ctrl Pts',(0.585799999999998,-3.01993227833314,
-1.52658086018387));
#89783=CARTESIAN_POINT('Ctrl Pts',(0.585799999999997,-3.03915803741692,
-1.49547921963615));
#89784=CARTESIAN_POINT('Ctrl Pts',(0.585799999999997,-3.05017677172482,
-1.47765413859557));
#89785=CARTESIAN_POINT('Ctrl Pts',(0.585799999999998,-3.0610420854361,-1.45972456616738));
#89786=CARTESIAN_POINT('Ctrl Pts',(0.585799999999997,-3.07175279236073,
-1.44169302107519));
#89787=CARTESIAN_POINT('Ctrl Pts',(0.585799999999996,-3.08051536309559,
-1.42694117598772));
#89788=CARTESIAN_POINT('Ctrl Pts',(0.585799999999998,-3.08917383312795,
-1.41212200437087));
#89789=CARTESIAN_POINT('Ctrl Pts',(0.585799999999998,-3.09772145058444,
-1.39724789804343));
#89790=CARTESIAN_POINT('Ctrl Pts',(0.585799999999998,-3.15344467524449,
-1.30028132546107));
#89791=CARTESIAN_POINT('Ctrl Pts',(0.585799999999995,-3.20453203572293,
-1.20086197202072));
#89792=CARTESIAN_POINT('Ctrl Pts',(0.585799999999994,-3.25087290134545,
-1.09942493104332));
#89793=CARTESIAN_POINT('Ctrl Pts',(0.585799999999993,-3.29776205531203,
-0.996787723722996));
#89794=CARTESIAN_POINT('Ctrl Pts',(0.585799999999992,-3.33979230665747,
-0.892084098641399));
#89795=CARTESIAN_POINT('Ctrl Pts',(0.585799999999992,-3.37681507082798,
-0.785722893322618));
#89796=CARTESIAN_POINT('Ctrl Pts',(0.585799999999992,-3.41375314830139,
-0.679604980998846));
#89797=CARTESIAN_POINT('Ctrl Pts',(0.585799999999991,-3.44570713185698,
-0.571836247002017));
#89798=CARTESIAN_POINT('Ctrl Pts',(0.585799999999993,-3.47248778918825,
-0.462792851071621));
#89799=CARTESIAN_POINT('Ctrl Pts',(0.585799999999993,-3.48965728959878,
-0.392883415764099));
#89800=CARTESIAN_POINT('Ctrl Pts',(0.585799999999996,-3.5046995408535,-0.32244948748404));
#89801=CARTESIAN_POINT('Ctrl Pts',(0.585799999999994,-3.51755413072086,
-0.251586084815355));
#89802=CARTESIAN_POINT('Ctrl Pts',(0.585799999999994,-3.52200137504234,
-0.227069793874057));
#89803=CARTESIAN_POINT('Ctrl Pts',(0.585799999999992,-3.52618669576443,
-0.202502078237746));
#89804=CARTESIAN_POINT('Ctrl Pts',(0.585799999999994,-3.53010733730041,
-0.177886819619966));
#89805=CARTESIAN_POINT('Ctrl Pts',(0.585799999999996,-3.53249109853745,
-0.16292067216823));
#89806=CARTESIAN_POINT('Ctrl Pts',(0.585799999999995,-3.53477657935189,
-0.147939396482612));
#89807=CARTESIAN_POINT('Ctrl Pts',(0.585799999999995,-3.53696191341059,
-0.132953840569866));
#89808=CARTESIAN_POINT('Ctrl Pts',(0.585799999999995,-3.55367763747858,
-0.0183286112394999));
#89809=CARTESIAN_POINT('Ctrl Pts',(0.585799999999994,-3.56456403896117,
0.096709245982323));
#89810=CARTESIAN_POINT('Ctrl Pts',(0.585799999999995,-3.56947395842516,
0.211735564449169));
#89811=CARTESIAN_POINT('Ctrl Pts',(0.585799999999994,-3.57211763385812,
0.273669829258397));
#89812=CARTESIAN_POINT('Ctrl Pts',(0.585799999999994,-3.57302793677542,
0.335601297332963));
#89813=CARTESIAN_POINT('Ctrl Pts',(0.585799999999994,-3.57217641958998,
0.39746679596036));
#89814=CARTESIAN_POINT('Ctrl Pts',(0.585799999999995,-3.57064955014543,
0.508398837193222));
#89815=CARTESIAN_POINT('Ctrl Pts',(0.585799999999993,-3.56346125874838,
0.619118451061581));
#89816=CARTESIAN_POINT('Ctrl Pts',(0.585799999999995,-3.55087631125224,
0.729340653175641));
#89817=CARTESIAN_POINT('Ctrl Pts',(0.585799999999996,-3.53805158338041,
0.841662913398155));
#89818=CARTESIAN_POINT('Ctrl Pts',(0.585799999999993,-3.51962249756278,
0.953469303091311));
#89819=CARTESIAN_POINT('Ctrl Pts',(0.585799999999995,-3.49581515276092,
1.06446168404778));
#89820=CARTESIAN_POINT('Ctrl Pts',(0.585799999999996,-3.48835663508087,
1.09923408905997));
#89821=CARTESIAN_POINT('Ctrl Pts',(0.585799999999993,-3.48036986358895,
1.13392658392764));
#89822=CARTESIAN_POINT('Ctrl Pts',(0.585799999999993,-3.47186075378713,
1.16852990102506));
#89823=CARTESIAN_POINT('Ctrl Pts',(0.585799999999995,-3.46514795967475,
1.19582828460338));
#89824=CARTESIAN_POINT('Ctrl Pts',(0.585799999999993,-3.45810778648413,
1.22307890759173));
#89825=CARTESIAN_POINT('Ctrl Pts',(0.585799999999994,-3.45075610902602,
1.25023064681264));
#89826=CARTESIAN_POINT('Ctrl Pts',(0.585799999999994,-3.42093932181936,
1.36035213068536));
#89827=CARTESIAN_POINT('Ctrl Pts',(0.585799999999994,-3.38597425835464,
1.46897437338361));
#89828=CARTESIAN_POINT('Ctrl Pts',(0.585799999999994,-3.34616091262472,
1.57580281021644));
#89829=CARTESIAN_POINT('Ctrl Pts',(0.585799999999993,-3.30508145284811,
1.6860285245697));
#89830=CARTESIAN_POINT('Ctrl Pts',(0.585799999999995,-3.25884040932796,
1.7943452321113));
#89831=CARTESIAN_POINT('Ctrl Pts',(0.585799999999997,-3.20771203882439,
1.90043247757802));
#89832=CARTESIAN_POINT('Ctrl Pts',(0.585799999999999,-3.15612402547689,
2.00747344487728));
#89833=CARTESIAN_POINT('Ctrl Pts',(0.585799999999998,-3.09956014992837,
2.11224548851188));
#89834=CARTESIAN_POINT('Ctrl Pts',(0.585799999999997,-3.03824934181154,
2.2144110110577));
#89835=CARTESIAN_POINT('Ctrl Pts',(0.585799999999997,-2.99849863814183,
2.2806497630285));
#89836=CARTESIAN_POINT('Ctrl Pts',(0.585799999999997,-2.95675147643439,
2.34579265403001));
#89837=CARTESIAN_POINT('Ctrl Pts',(0.585799999999995,-2.91305938898694,
2.40974333609371));
#89838=CARTESIAN_POINT('Ctrl Pts',(0.585799999999995,-2.89642626520271,
2.43408869638647));
#89839=CARTESIAN_POINT('Ctrl Pts',(0.585799999999994,-2.87951163347175,
2.4582606131126));
#89840=CARTESIAN_POINT('Ctrl Pts',(0.585799999999996,-2.86231665815064,
2.48225550433344));
#89841=CARTESIAN_POINT('Ctrl Pts',(0.585799999999997,-2.84712565273625,
2.50345393676189));
#89842=CARTESIAN_POINT('Ctrl Pts',(0.585799999999995,-2.83171488921404,
2.52451508711931));
#89843=CARTESIAN_POINT('Ctrl Pts',(0.585799999999996,-2.81610831463341,
2.54540619518073));
#89844=CARTESIAN_POINT('Ctrl Pts',(0.585799999999997,-2.74275312496236,
2.64360014455544));
#89845=CARTESIAN_POINT('Ctrl Pts',(0.585799999999995,-2.66498329274227,
2.73817129382513));
#89846=CARTESIAN_POINT('Ctrl Pts',(0.585799999999995,-2.58308793541154,
2.82878454959318));
#89847=CARTESIAN_POINT('Ctrl Pts',(0.585799999999995,-2.50105380468771,
2.91955135141527));
#89848=CARTESIAN_POINT('Ctrl Pts',(0.585799999999995,-2.4148797735425,3.00634766584885));
#89849=CARTESIAN_POINT('Ctrl Pts',(0.585799999999996,-2.32480654965838,
3.08882057079662));
#89850=CARTESIAN_POINT('Ctrl Pts',(0.585799999999997,-2.23610653303497,
3.17003613880226));
#89851=CARTESIAN_POINT('Ctrl Pts',(0.585799999999995,-2.14362482415573,
3.2470598493341));
#89852=CARTESIAN_POINT('Ctrl Pts',(0.585799999999996,-2.04754958290616,
3.31952755214537));
#89853=CARTESIAN_POINT('Ctrl Pts',(0.585799999999997,-1.9514743416566,3.39199525495664));
#89854=CARTESIAN_POINT('Ctrl Pts',(0.585799999999997,-1.85180519811705,
3.45990776211604));
#89855=CARTESIAN_POINT('Ctrl Pts',(0.585799999999996,-1.74869447533108,
3.5228619944509));
#89856=CARTESIAN_POINT('Origin',(0.585799999999996,-5.160062080289E-16,
2.1385152528819E-16));
#89857=CARTESIAN_POINT('',(0.585799999999997,-3.933,-4.81653586104654E-16));
#89858=CARTESIAN_POINT('Origin',(0.585799999999996,0.,0.));
#89859=CARTESIAN_POINT('',(0.585799999999996,1.82083948017239,3.48611999039699));
#89860=CARTESIAN_POINT('Origin',(0.585799999999996,0.,0.));
#89861=CARTESIAN_POINT('Ctrl Pts',(0.585799999999996,1.82083948017239,3.48611999039699));
#89862=CARTESIAN_POINT('Ctrl Pts',(0.585799999999996,1.86689239886374,3.45684336336271));
#89863=CARTESIAN_POINT('Ctrl Pts',(0.585799999999994,1.91225446113732,3.4265446583295));
#89864=CARTESIAN_POINT('Ctrl Pts',(0.585799999999993,1.95688759198411,3.39522130376487));
#89865=CARTESIAN_POINT('Ctrl Pts',(0.585799999999993,2.05792862938297,3.32431110365171));
#89866=CARTESIAN_POINT('Ctrl Pts',(0.585799999999995,2.15523691577152,3.24815207496259));
#89867=CARTESIAN_POINT('Ctrl Pts',(0.585799999999993,2.24861882171376,3.16717424928343));
#89868=CARTESIAN_POINT('Ctrl Pts',(0.585799999999991,2.342000727656,3.08619642360427));
#89869=CARTESIAN_POINT('Ctrl Pts',(0.585799999999997,2.43145663514149,3.00039885361381));
#89870=CARTESIAN_POINT('Ctrl Pts',(0.585799999999992,2.51674675544355,2.91018295065707));
#89871=CARTESIAN_POINT('Ctrl Pts',(0.585799999999992,2.53166856913533,2.89439935355123));
#89872=CARTESIAN_POINT('Ctrl Pts',(0.585799999999993,2.54646336716743,2.87847967405364));
#89873=CARTESIAN_POINT('Ctrl Pts',(0.585799999999993,2.56111841909083,2.86243871338739));
#89874=CARTESIAN_POINT('Ctrl Pts',(0.585799999999993,2.64273316869577,2.77310576560654));
#89875=CARTESIAN_POINT('Ctrl Pts',(0.585799999999991,2.72010252438485,2.67992491422671));
#89876=CARTESIAN_POINT('Ctrl Pts',(0.585799999999991,2.79304166360886,2.58329939719082));
#89877=CARTESIAN_POINT('Ctrl Pts',(0.585799999999991,2.86593404565316,2.48673582133924));
#89878=CARTESIAN_POINT('Ctrl Pts',(0.585799999999991,2.93440222148946,2.38673110322598));
#89879=CARTESIAN_POINT('Ctrl Pts',(0.585799999999989,2.99821451712912,2.28366714323217));
#89880=CARTESIAN_POINT('Ctrl Pts',(0.585799999999988,3.03261534584538,2.22810597592068));
#89881=CARTESIAN_POINT('Ctrl Pts',(0.585799999999991,3.0656622305983,2.1716554512815));
#89882=CARTESIAN_POINT('Ctrl Pts',(0.585799999999992,3.09731265936069,2.11437429574504));
#89883=CARTESIAN_POINT('Ctrl Pts',(0.585799999999992,3.10817794722411,2.09471022582911));
#89884=CARTESIAN_POINT('Ctrl Pts',(0.585799999999988,3.11888004010657,2.07494541123311));
#89885=CARTESIAN_POINT('Ctrl Pts',(0.585799999999988,3.12940560295807,2.05510444625068));
#89886=CARTESIAN_POINT('Ctrl Pts',(0.585799999999988,3.18506667019072,1.95018185907613));
#89887=CARTESIAN_POINT('Ctrl Pts',(0.585799999999991,3.23586400154897,1.84300973943562));
#89888=CARTESIAN_POINT('Ctrl Pts',(0.585799999999991,3.28162189719394,1.73396327121137));
#89889=CARTESIAN_POINT('Ctrl Pts',(0.585799999999992,3.3269647454697,1.625905909875));
#89890=CARTESIAN_POINT('Ctrl Pts',(0.585799999999992,3.36735937924477,1.51600719065838));
#89891=CARTESIAN_POINT('Ctrl Pts',(0.58579999999999,3.40258571934794,1.40462038544498));
#89892=CARTESIAN_POINT('Ctrl Pts',(0.585799999999989,3.43679103713209,1.29646208520354));
#89893=CARTESIAN_POINT('Ctrl Pts',(0.58579999999999,3.46612334072379,1.18689998727959));
#89894=CARTESIAN_POINT('Ctrl Pts',(0.585799999999992,3.49033317665986,1.07625791163838));
#89895=CARTESIAN_POINT('Ctrl Pts',(0.585799999999994,3.5145408993762,0.965625493684133));
#89896=CARTESIAN_POINT('Ctrl Pts',(0.585799999999996,3.5336272953427,0.853912602230459));
#89897=CARTESIAN_POINT('Ctrl Pts',(0.585799999999991,3.54729199691672,0.741453780800409));
#89898=CARTESIAN_POINT('Ctrl Pts',(0.58579999999999,3.54907908440556,0.726746269502171));
#89899=CARTESIAN_POINT('Ctrl Pts',(0.585799999999992,3.55077294157688,0.712029231162681));
#89900=CARTESIAN_POINT('Ctrl Pts',(0.585799999999992,3.55237217730448,0.697311529599281));
#89901=CARTESIAN_POINT('Ctrl Pts',(0.585799999999991,3.564454224488,0.58612093921081));
#89902=CARTESIAN_POINT('Ctrl Pts',(0.585799999999992,3.57115664198564,0.474755467253984));
#89903=CARTESIAN_POINT('Ctrl Pts',(0.585799999999994,3.57228231247333,0.363530962342787));
#89904=CARTESIAN_POINT('Ctrl Pts',(0.585799999999995,3.57293014058781,0.299520790548671));
#89905=CARTESIAN_POINT('Ctrl Pts',(0.585799999999992,3.57172999413913,0.235557298783211));
#89906=CARTESIAN_POINT('Ctrl Pts',(0.585799999999993,3.56863646597307,0.171701567603425));
#89907=CARTESIAN_POINT('Ctrl Pts',(0.585799999999994,3.56316184516739,0.0586959973568367));
#89908=CARTESIAN_POINT('Ctrl Pts',(0.585799999999995,3.55176000723791,-0.0539733642235792));
#89909=CARTESIAN_POINT('Ctrl Pts',(0.585799999999996,3.53464522492657,-0.165950017323518));
#89910=CARTESIAN_POINT('Ctrl Pts',(0.585799999999996,3.51745024634637,-0.278451369459369));
#89911=CARTESIAN_POINT('Ctrl Pts',(0.585799999999995,3.49448812402454,-0.390254307938234));
#89912=CARTESIAN_POINT('Ctrl Pts',(0.585799999999996,3.46593137547018,-0.500970793960552));
#89913=CARTESIAN_POINT('Ctrl Pts',(0.585799999999996,3.45734555588329,-0.534258609359854));
#89914=CARTESIAN_POINT('Ctrl Pts',(0.585799999999996,3.44825373273905,-0.567447988369024));
#89915=CARTESIAN_POINT('Ctrl Pts',(0.585799999999996,3.43865992038094,-0.600527751346839));
#89916=CARTESIAN_POINT('Ctrl Pts',(0.585799999999996,3.43333132637031,-0.61890090899228));
#89917=CARTESIAN_POINT('Ctrl Pts',(0.585799999999998,3.42784720581633,-0.637242086460123));
#89918=CARTESIAN_POINT('Ctrl Pts',(0.585799999999998,3.42221506109668,-0.655528003234818));
#89919=CARTESIAN_POINT('Ctrl Pts',(0.585799999999997,3.3894351801136,-0.761954632055157));
#89920=CARTESIAN_POINT('Ctrl Pts',(0.585799999999997,3.35159967116233,-0.866672925050383));
#89921=CARTESIAN_POINT('Ctrl Pts',(0.585799999999998,3.30894399549316,-0.969356272713158));
#89922=CARTESIAN_POINT('Ctrl Pts',(0.585799999999998,3.26622213144329,-1.07219895308841));
#89923=CARTESIAN_POINT('Ctrl Pts',(0.585799999999998,3.21866454774918,-1.17300112326194));
#89924=CARTESIAN_POINT('Ctrl Pts',(0.585799999999997,3.16646307567001,-1.27140745990975));
#89925=CARTESIAN_POINT('Ctrl Pts',(0.585799999999996,3.11519187949628,-1.36806010953914));
#89926=CARTESIAN_POINT('Ctrl Pts',(0.585799999999999,3.05944019547891,-1.46240213536194));
#89927=CARTESIAN_POINT('Ctrl Pts',(0.585799999999999,2.99935592247331,-1.55406095152871));
#89928=CARTESIAN_POINT('Ctrl Pts',(0.585799999999999,2.94555794445917,-1.6361299977246));
#89929=CARTESIAN_POINT('Ctrl Pts',(0.585799999999998,2.88828584813885,-1.7160477730359));
#89930=CARTESIAN_POINT('Ctrl Pts',(0.585799999999998,2.8276281243483,-1.79351600647639));
#89931=CARTESIAN_POINT('Ctrl Pts',(0.585799999999998,2.81803085597279,-1.80577303460807));
#89932=CARTESIAN_POINT('Ctrl Pts',(0.585800000000001,2.80835473108984,-1.81796109589995));
#89933=CARTESIAN_POINT('Ctrl Pts',(0.585800000000001,2.79860130069776,-1.83007805473447));
#89934=CARTESIAN_POINT('Ctrl Pts',(0.5858,2.73119899243548,-1.91381382376484));
#89935=CARTESIAN_POINT('Ctrl Pts',(0.585799999999997,2.660092568064,-1.99417628046629));
#89936=CARTESIAN_POINT('Ctrl Pts',(0.585799999999997,2.58545667302995,-2.070844698974));
#89937=CARTESIAN_POINT('Ctrl Pts',(0.585799999999998,2.51187463795161,-2.14643055826412));
#89938=CARTESIAN_POINT('Ctrl Pts',(0.585799999999998,2.43486151262633,-2.21842647190396));
#89939=CARTESIAN_POINT('Ctrl Pts',(0.585799999999998,2.35455634075026,-2.28648423693865));
#89940=CARTESIAN_POINT('Ctrl Pts',(0.585799999999999,2.27672129251548,-2.35244859889035));
#89941=CARTESIAN_POINT('Ctrl Pts',(0.585799999999995,2.19579306375139,-2.41471364081201));
#89942=CARTESIAN_POINT('Ctrl Pts',(0.585799999999996,2.11187976848003,-2.47291808201015));
#89943=CARTESIAN_POINT('Ctrl Pts',(0.585799999999996,2.03430797415558,-2.52672389343481));
#89944=CARTESIAN_POINT('Ctrl Pts',(0.585799999999997,1.9541847994988,-2.57705949460462));
#89945=CARTESIAN_POINT('Ctrl Pts',(0.585799999999993,1.87158653173903,-2.62360084935061));
#89946=CARTESIAN_POINT('Ctrl Pts',(0.173952222118149,2.28357519912527,-3.20566422525929));
#89947=CARTESIAN_POINT('Ctrl Pts',(0.240279004907857,3.35237972307857,-2.44437977786446));
#89948=CARTESIAN_POINT('Ctrl Pts',(0.372888193944113,4.64898952799387,0.217548081197305));
#89949=CARTESIAN_POINT('Ctrl Pts',(0.571779789226917,2.32539586803166,4.03618744464615));
#89950=CARTESIAN_POINT('Ctrl Pts',(0.77062700796656,-2.13583691697174,4.13464652641104));
#89951=CARTESIAN_POINT('Ctrl Pts',(0.969474226706204,-4.63403193779818,
0.440985093923363));
#89952=CARTESIAN_POINT('Ctrl Pts',(1.16832144544584,-2.87607675100017,-3.6608002142644));
#89953=CARTESIAN_POINT('Ctrl Pts',(1.36716866418549,1.524085161197,-4.39826153122039));
#89954=CARTESIAN_POINT('Ctrl Pts',(1.56601588292513,4.52409602411104,-1.09639957599426));
#89955=CARTESIAN_POINT('Ctrl Pts',(1.76486310166478,3.36844732971546,3.21302626912509));
#89956=CARTESIAN_POINT('Ctrl Pts',(1.96371032040441,-0.881431179013023,
4.57080526913485));
#89957=CARTESIAN_POINT('Ctrl Pts',(2.16255753914406,-4.3216225377087,1.73005466709287));
#89958=CARTESIAN_POINT('Ctrl Pts',(2.3614047578837,-3.79207170539569,-2.69995067838618));
#89959=CARTESIAN_POINT('Ctrl Pts',(2.56025197662336,0.220804693931135,-4.64980423380701));
#89960=CARTESIAN_POINT('Ctrl Pts',(2.759099195363,4.03085120606417,-2.32845977156154));
#89961=CARTESIAN_POINT('Ctrl Pts',(2.95794641410263,4.13824202747698,2.13176900450027));
#89962=CARTESIAN_POINT('Ctrl Pts',(3.15679363284228,0.444327587898382,4.63379380141549));
#89963=CARTESIAN_POINT('Ctrl Pts',(3.35564085158192,-3.65773661521517,2.87931292379523));
#89964=CARTESIAN_POINT('Ctrl Pts',(3.55448807032156,-4.39987910846512,-1.52004710629562));
#89965=CARTESIAN_POINT('Ctrl Pts',(3.75333528906121,-1.10038262959936,-4.52312233170167));
#89966=CARTESIAN_POINT('Ctrl Pts',(3.95218250780086,3.20990273307694,-3.37135035508323));
#89967=CARTESIAN_POINT('Ctrl Pts',(4.15102972654051,4.57163721316586,0.877275198462322));
#89968=CARTESIAN_POINT('Ctrl Pts',(4.34987694528013,1.73395935114604,4.32005362547157));
#89969=CARTESIAN_POINT('Ctrl Pts',(4.54872416401979,-2.69649805273161,3.79451930930212));
#89970=CARTESIAN_POINT('Ctrl Pts',(4.74757138275942,-4.65000757025798,-0.216582764486197));
#89971=CARTESIAN_POINT('Ctrl Pts',(4.94641860149908,-2.33211535592997,-4.02873633259774));
#89972=CARTESIAN_POINT('Ctrl Pts',(5.1452658202387,2.12801026500781,-4.14017521473941));
#89973=CARTESIAN_POINT('Ctrl Pts',(5.34411303897837,4.63338923547031,-0.44853392512834));
#89974=CARTESIAN_POINT('Ctrl Pts',(5.54296025771799,2.88263173829438,3.65512144091822));
#89975=CARTESIAN_POINT('Ctrl Pts',(5.74180747645765,-1.51605224178122,4.4012571034094));
#89976=CARTESIAN_POINT('Ctrl Pts',(5.94065469519728,-4.52212167899159,1.10448812091657));
#89977=CARTESIAN_POINT('Ctrl Pts',(6.13950191393694,-3.37426274767644,-3.20684103101759));
#89978=CARTESIAN_POINT('Ctrl Pts',(6.33834913267657,0.873124844100889,-4.57243168299889));
#89979=CARTESIAN_POINT('Ctrl Pts',(6.53719635141622,4.31847783430739,-1.7378802270194));
#89980=CARTESIAN_POINT('Ctrl Pts',(6.73604357015585,3.7969655214586,2.69305241644208));
#89981=CARTESIAN_POINT('Ctrl Pts',(6.93489078889551,-0.212361563592659,
4.65020225960404));
#89982=CARTESIAN_POINT('Ctrl Pts',(7.13373800763515,-4.02661766515626,2.33577153581771));
#89983=CARTESIAN_POINT('Ctrl Pts',(7.33258522637479,-4.14210523822186,-2.12425108788485));
#89984=CARTESIAN_POINT('Ctrl Pts',(7.53143244511446,-0.452739763174514,
-4.63298016353779));
#89985=CARTESIAN_POINT('Ctrl Pts',(7.73027966385406,3.65250318693606,-2.88594853701702));
#89986=CARTESIAN_POINT('Ctrl Pts',(7.92912688259373,4.40263150697405,1.5120563159779));
#89987=CARTESIAN_POINT('Ctrl Pts',(8.12797410133337,1.10859268358586,4.52111720162066));
#89988=CARTESIAN_POINT('Ctrl Pts',(8.32682132007301,-3.20377667673212,3.37717241113287));
#89989=CARTESIAN_POINT('Ctrl Pts',(8.52566853881265,-4.57322239004683,-0.86897379711017));
#89990=CARTESIAN_POINT('Ctrl Pts',(8.7245157575523,-1.74179966817418,-4.31689847052698));
#89991=CARTESIAN_POINT('Ctrl Pts',(8.92336297629194,2.68960455960068,-3.79940861212176));
#89992=CARTESIAN_POINT('Ctrl Pts',(9.12221019503159,4.65039311774333,0.208140191542384));
#89993=CARTESIAN_POINT('Ctrl Pts',(9.32105741377122,2.33942579057017,4.02449567763527));
#89994=CARTESIAN_POINT('Ctrl Pts',(9.51990463251087,-2.12049016010714,4.14403184951306));
#89995=CARTESIAN_POINT('Ctrl Pts',(9.71875185125051,-4.63256727397068,0.456945227599198));
#89996=CARTESIAN_POINT('Ctrl Pts',(9.91759906999016,-2.88926295756309,-3.64988192287692));
#89997=CARTESIAN_POINT('Ctrl Pts',(10.1164462887298,1.50805914415905,-4.404002282766));
#89998=CARTESIAN_POINT('Ctrl Pts',(10.3152935074695,4.52010899870567,-1.11269633265763));
#89999=CARTESIAN_POINT('Ctrl Pts',(10.5141407262091,3.38007929167327,3.2007096823816));
#90000=CARTESIAN_POINT('Ctrl Pts',(10.7129879449488,-0.86482203405061,4.57400932862083));
#90001=CARTESIAN_POINT('Ctrl Pts',(10.9118351636884,-4.31531554947323,1.74571767401385));
#90002=CARTESIAN_POINT('Ctrl Pts',(11.1106823824281,-3.80184857193813,-2.68615448642514));
#90003=CARTESIAN_POINT('Ctrl Pts',(11.3095296011677,0.203918647976768,-4.65058014379897));
#90004=CARTESIAN_POINT('Ctrl Pts',(11.5083768199074,4.02237037378927,-2.34307811755224));
#90005=CARTESIAN_POINT('Ctrl Pts',(11.707224038647,4.14595504597677,2.11672748497051));
#90006=CARTESIAN_POINT('Ctrl Pts',(11.9060712573866,0.46115031548507,4.6321505670064));
#90007=CARTESIAN_POINT('Ctrl Pts',(12.1049184761263,-3.64725765118733,2.89257499725508));
#90008=CARTESIAN_POINT('Ctrl Pts',(12.3037656948659,-4.40536942950588,-1.50406072964653));
#90009=CARTESIAN_POINT('Ctrl Pts',(12.5026129136056,-1.1167990648287,-4.51909707106271));
#90010=CARTESIAN_POINT('Ctrl Pts',(12.7014601323452,3.19764005053429,-3.38298338690999));
#90011=CARTESIAN_POINT('Ctrl Pts',(12.9003073510849,4.57479249805102,0.860669558347425));
#90012=CARTESIAN_POINT('Ctrl Pts',(13.0991545698245,1.74963424132104,4.31372907244841));
#90013=CARTESIAN_POINT('Ctrl Pts',(13.2980017885641,-2.68270219976425,3.80428539889818));
#90014=CARTESIAN_POINT('Ctrl Pts',(13.4968490073038,-4.65076333761376,-0.199696936375007));
#90015=CARTESIAN_POINT('Ctrl Pts',(13.6956962260434,-2.34672851375597,-4.02024175536926));
#90016=CARTESIAN_POINT('Ctrl Pts',(13.8945434447831,2.11296306557631,-4.1478748260284));
#90017=CARTESIAN_POINT('Ctrl Pts',(14.0933906635227,4.63173004298792,-0.465355023366944));
#90018=CARTESIAN_POINT('Ctrl Pts',(14.2922378822624,2.89588465336402,3.64463037402978));
#90019=CARTESIAN_POINT('Ctrl Pts',(14.491085101002,-1.50006107573536,4.40673294606713));
#90020=CARTESIAN_POINT('Ctrl Pts',(14.6899323197417,-4.51808141952556,1.12090087671823));
#90021=CARTESIAN_POINT('Ctrl Pts',(14.8887795384813,-3.38588469444997,-3.19456778371962));
#90022=CARTESIAN_POINT('Ctrl Pts',(15.0876267572209,0.856516373422385,-4.57557189769205));
#90023=CARTESIAN_POINT('Ctrl Pts',(15.2864739759606,4.31213904075985,-1.75354936686836));
#90024=CARTESIAN_POINT('Ctrl Pts',(15.4853211947002,3.80671909099388,2.67924770246286));
#90025=CARTESIAN_POINT('Ctrl Pts',(15.6841684134399,-0.195475060215983,
4.65094269903676));
#90026=CARTESIAN_POINT('Ctrl Pts',(15.8830156321795,-4.01810982412929,2.35037697617328));
#90027=CARTESIAN_POINT('Ctrl Pts',(16.0818628509192,-4.14979118808601,-2.10919690502656));
#90028=CARTESIAN_POINT('Ctrl Pts',(16.2807100696588,-0.469559347780013,
-4.63130570226176));
#90029=CARTESIAN_POINT('Ctrl Pts',(16.4795572883984,3.64200009356924,-2.89919192316264));
#90030=CARTESIAN_POINT('Ctrl Pts',(16.6784045071381,4.40809283132617,1.49606018572135));
#90031=CARTESIAN_POINT('Ctrl Pts',(16.8772517258777,1.12500176494622,4.51706204493116));
#90032=CARTESIAN_POINT('Ctrl Pts',(17.0760989446174,-3.19149288446924,3.38878321190246));
#90033=CARTESIAN_POINT('Ctrl Pts',(17.274946163357,-4.57634752690168,-0.852362482697826));
#90034=CARTESIAN_POINT('Ctrl Pts',(17.4737933820967,-1.75746304742967,-4.31054545571777));
#90035=CARTESIAN_POINT('Ctrl Pts',(17.6726406008363,2.67579099736758,-3.8091496462198));
#90036=CARTESIAN_POINT('Ctrl Pts',(17.8714878195759,4.65111822792017,0.191253022978689));
#90037=CARTESIAN_POINT('Ctrl Pts',(18.0703350383156,2.35402350179763,4.01597458182621));
#90038=CARTESIAN_POINT('Ctrl Pts',(18.2691822570552,-2.10542900642473,4.15170413057039));
#90039=CARTESIAN_POINT('Ctrl Pts',(18.4680294757949,-4.63087754517756,0.473763285259743));
#90040=CARTESIAN_POINT('Ctrl Pts',(18.6668766945345,-2.90249680392564,-3.63936681197312));
#90041=CARTESIAN_POINT('Ctrl Pts',(18.8657239132742,1.49205806290137,-4.40944908416242));
#90042=CARTESIAN_POINT('Ctrl Pts',(19.0645711320138,4.51603894811952,-1.12910172613336));
#90043=CARTESIAN_POINT('Ctrl Pts',(19.2634183507534,3.39167893687894,3.18841535531705));
#90044=CARTESIAN_POINT('Ctrl Pts',(19.4622655694931,-0.84820788959677,4.57711938504072));
#90045=CARTESIAN_POINT('Ctrl Pts',(19.6611127882327,-4.3089483186353,1.7613752797799));
#90046=CARTESIAN_POINT('Ctrl Pts',(19.8599600069724,-3.81157706257311,-2.67233208732681));
#90047=CARTESIAN_POINT('Ctrl Pts',(20.058807225712,0.187030828142195,-4.65128992411937));
#90048=CARTESIAN_POINT('Ctrl Pts',(20.2576544444516,4.01383603021948,-2.35766808762422));
#90049=CARTESIAN_POINT('Ctrl Pts',(20.4565016631913,4.15361365190522,2.10165937287571));
#90050=CARTESIAN_POINT('Ctrl Pts',(20.6553488819309,0.477966832341934,4.63044557208816));
#90051=CARTESIAN_POINT('Ctrl Pts',(20.8541961006706,-3.6367305314113,2.90579929292968));
#90052=CARTESIAN_POINT('Ctrl Pts',(21.0530433194102,-4.41080170345829,-1.48805471057328));
#90053=CARTESIAN_POINT('Ctrl Pts',(21.2518905381499,-1.13320075690117,-4.51501212993371));
#90054=CARTESIAN_POINT('Ctrl Pts',(21.4507377568895,3.18533519879899,-3.39457186699324));
#90055=CARTESIAN_POINT('Ctrl Pts',(21.6495849756292,4.57788747147318,0.844052597542735));
#90056=CARTESIAN_POINT('Ctrl Pts',(21.8484321943688,1.7652860606952,4.30734763082863));
#90057=CARTESIAN_POINT('Ctrl Pts',(22.0472794131084,-2.66887097519087,3.81400133805345));
#90058=CARTESIAN_POINT('Ctrl Pts',(22.2461266318481,-4.65145778749283,-0.182808479185734));
#90059=CARTESIAN_POINT('Ctrl Pts',(22.4449738505877,-2.3613107306498,-4.01169417107137));
#90060=CARTESIAN_POINT('Ctrl Pts',(22.6438210693274,2.09788800748582,-4.15551975051701));
#90061=CARTESIAN_POINT('Ctrl Pts',(22.8426682880671,4.63000978334952,-0.482169985562706));
#90062=CARTESIAN_POINT('Ctrl Pts',(23.0415155068066,2.90909938745336,3.63409125405627));
#90063=CARTESIAN_POINT('Ctrl Pts',(23.2403627255463,-1.48405013203601,4.41215068809913));
#90064=CARTESIAN_POINT('Ctrl Pts',(23.4392099442859,-4.51398159121979,1.13729885387195));
#90065=CARTESIAN_POINT('Ctrl Pts',(23.6380571630256,-3.39746199986158,-3.18225241745317));
#90066=CARTESIAN_POINT('Ctrl Pts',(23.8369043817652,0.839896609959785,-4.57865178556615));
#90067=CARTESIAN_POINT('Ctrl Pts',(24.0357516005049,4.30574339361672,-1.769195386953));
#90068=CARTESIAN_POINT('Ctrl Pts',(24.2345988192446,3.81642247066319,2.66540766381184));
#90069=CARTESIAN_POINT('Ctrl Pts',(24.4334460379841,-0.178585979588697,
4.65162181790224));
#90070=CARTESIAN_POINT('Ctrl Pts',(24.6322932567239,-4.00954900614679,2.36495142787269));
#90071=CARTESIAN_POINT('Ctrl Pts',(24.8311404754634,-4.15742242483508,-2.0941149133627));
#90072=CARTESIAN_POINT('Ctrl Pts',(25.0299876942031,-0.4863727414586,-4.62957017932074));
#90073=CARTESIAN_POINT('Ctrl Pts',(25.2288349129427,3.63144898208279,-2.91239708477736));
#90074=CARTESIAN_POINT('Ctrl Pts',(25.4276821316824,4.41349603697337,1.48004433058948));
#90075=CARTESIAN_POINT('Ctrl Pts',(25.626529350422,1.14139601366861,4.5129473328271));
#90076=CARTESIAN_POINT('Ctrl Pts',(25.8253765691617,-3.17916701381997,3.40034933310223));
#90077=CARTESIAN_POINT('Ctrl Pts',(26.0242237879013,-4.57941232668972,-0.835739930272565));
#90078=CARTESIAN_POINT('Ctrl Pts',(26.2230710066409,-1.77310325533199,-4.30413560832147));
#90079=CARTESIAN_POINT('Ctrl Pts',(26.4219182253806,2.66194215604348,-3.81884045840728));
#90080=CARTESIAN_POINT('Ctrl Pts',(26.6207654441202,4.65178201521246,0.174363332830453));
#90081=CARTESIAN_POINT('Ctrl Pts',(26.8196126628599,2.36859017629287,4.00740053721347));
#90082=CARTESIAN_POINT('Ctrl Pts',(27.0184598815995,-2.09034009361562,4.15932167329157));
#90083=CARTESIAN_POINT('Ctrl Pts',(27.2173071003392,-4.62912676036407,0.490575096566251));
#90084=CARTESIAN_POINT('Ctrl Pts',(27.4161543190788,-2.91569238218416,-3.62880371766826));
#90085=CARTESIAN_POINT('Ctrl Pts',(27.6150015378185,1.47603730953467,-4.41483774897238));
#90086=CARTESIAN_POINT('Ctrl Pts',(27.8138487565581,4.5119093556078,-1.14549223291496));
#90087=CARTESIAN_POINT('Ctrl Pts',(28.0126959752978,3.40323386433599,3.17607899044191));
#90088=CARTESIAN_POINT('Ctrl Pts',(28.2115431940374,-0.831582561906483,
4.58016909421725));
#90089=CARTESIAN_POINT('Ctrl Pts',(28.410390412777,-4.30252427626788,1.77700966261172));
#90090=CARTESIAN_POINT('Ctrl Pts',(28.6092376315167,-3.82125529929308,-2.65847445474172));
#90091=CARTESIAN_POINT('Ctrl Pts',(28.8080848502563,0.170140542390847,-4.65193837929144));
#90092=CARTESIAN_POINT('Ctrl Pts',(29.006932068996,4.00524876604184,-2.37222697291178));
#90093=CARTESIAN_POINT('Ctrl Pts',(29.2057792877356,4.16121749432138,2.08656355135507));
#90094=CARTESIAN_POINT('Ctrl Pts',(29.4046265064753,0.494777047422964,4.62867952684493));
#90095=CARTESIAN_POINT('Ctrl Pts',(29.6034737252149,-3.62615546299245,2.91898527695842));
#90096=CARTESIAN_POINT('Ctrl Pts',(29.8023209439545,-4.41617582299051,-1.47202907217344));
#90097=CARTESIAN_POINT('Ctrl Pts',(30.0011681626942,-1.14958750823563,-4.51086766041727));
#90098=CARTESIAN_POINT('Ctrl Pts',(30.2000153814338,3.17298834986358,-3.40611559118592));
#90099=CARTESIAN_POINT('Ctrl Pts',(30.3988626001735,4.58092208752509,0.827424508287263));
#90100=CARTESIAN_POINT('Ctrl Pts',(30.5977098189131,1.78091460557327,4.30090939878366));
#90101=CARTESIAN_POINT('Ctrl Pts',(30.7965570376528,-2.65500456276395,3.82366699133076));
#90102=CARTESIAN_POINT('Ctrl Pts',(30.9954042563924,-4.65209091001037,-0.165917611749485));
#90103=CARTESIAN_POINT('Ctrl Pts',(31.1942514751321,-2.37586181473258,-4.00309369440504));
#90104=CARTESIAN_POINT('Ctrl Pts',(31.3930986938717,2.08278528969322,-4.16310988636228));
#90105=CARTESIAN_POINT('Ctrl Pts',(31.5919459126113,4.62822847913179,-0.498978590566));
#90106=CARTESIAN_POINT('Ctrl Pts',(31.790793131351,2.92227576638665,3.62350422023752));
#90107=CARTESIAN_POINT('Ctrl Pts',(31.9896403500906,-1.46801962180864,4.41751025792524));
#90108=CARTESIAN_POINT('Ctrl Pts',(32.1884875688303,-4.50982224811389,1.15368183625598));
#90109=CARTESIAN_POINT('Ctrl Pts',(32.3873347875699,-3.40899451127737,-3.16989509463177));
#90110=CARTESIAN_POINT('Ctrl Pts',(32.5861820063095,0.823265772841283,-4.58167130599281));
#90111=CARTESIAN_POINT('Ctrl Pts',(32.7850292250492,4.29929097719954,-1.78481808099885));
#90112=CARTESIAN_POINT('Ctrl Pts',(32.9838764437888,3.82607553253298,2.65153248296947));
#90113=CARTESIAN_POINT('Ctrl Pts',(33.1827236625285,-0.161694544386196,
4.65223960724354));
#90114=CARTESIAN_POINT('Ctrl Pts',(33.3815708812681,-4.00093532407891,2.37949469876008));
#90115=CARTESIAN_POINT('Ctrl Pts',(33.5804181000078,-4.1649988478549,-2.07900531174335));
#90116=CARTESIAN_POINT('Ctrl Pts',(33.7792653187474,-0.503179722533174,
-4.6277736175964));
#90117=CARTESIAN_POINT('Ctrl Pts',(33.9781125374871,3.62084999158835,-2.92556384775728));
#90118=CARTESIAN_POINT('Ctrl Pts',(34.1769597562267,4.41884105267683,1.46400896174433));
#90119=CARTESIAN_POINT('Ctrl Pts',(34.3758069749664,1.15777521360213,4.50877311955908));
#90120=CARTESIAN_POINT('Ctrl Pts',(34.574654193706,-3.16679922729543,3.41187062223805));
#90121=CARTESIAN_POINT('Ctrl Pts',(34.7735014124457,-4.58241674900297,-0.81910635899549));
#90122=CARTESIAN_POINT('Ctrl Pts',(34.9723486311852,-1.78872008567185,-4.29766901284916));
#90123=CARTESIAN_POINT('Ctrl Pts',(35.1711958499249,2.64805821821942,-3.82848092091503));
#90124=CARTESIAN_POINT('Ctrl Pts',(35.3700430686646,4.65238447086841,0.157471343780943));
#90125=CARTESIAN_POINT('Ctrl Pts',(35.5688902874042,2.38312562200067,3.99877365684203));
#90126=CARTESIAN_POINT('Ctrl Pts',(35.7677375061439,-2.07522362062035,4.16688437724269));
#90127=CARTESIAN_POINT('Ctrl Pts',(35.9665847248835,-4.62731494261354,0.507380439862646));
#90128=CARTESIAN_POINT('Ctrl Pts',(36.1654319436232,-2.9288495183609,-3.61819277923204));
#90129=CARTESIAN_POINT('Ctrl Pts',(36.3642791623628,1.45999709528542,-4.42016820614871));
#90130=CARTESIAN_POINT('Ctrl Pts',(36.5631263811024,4.50772027561737,-1.16186763690095));
#90131=CARTESIAN_POINT('Ctrl Pts',(36.7619735998421,3.4147439216979,3.1637007504056));
#90132=CARTESIAN_POINT('Ctrl Pts',(36.9608208185817,-0.814946270177291,
4.58315841594136));
#90133=CARTESIAN_POINT('Ctrl Pts',(37.1596680373214,-4.29604350706908,1.79262061637693));
#90134=CARTESIAN_POINT('Ctrl Pts',(37.358515256061,-3.83088315449479,-2.64458177137669));
#90135=CARTESIAN_POINT('Ctrl Pts',(37.5573624748007,0.153248013413796,-4.65252550076564));
#90136=CARTESIAN_POINT('Ctrl Pts',(37.7562096935402,3.99660869447566,-2.38675458146231));
#90137=CARTESIAN_POINT('Ctrl Pts',(37.95505691228,4.16876647297188,2.07144021944043));
#90138=CARTESIAN_POINT('Ctrl Pts',(38.1539041310195,0.51158073909287,4.6268524545612));
#90139=CARTESIAN_POINT('Ctrl Pts',(38.3527513497593,-3.61553258535822,2.93213277548999));
#90140=CARTESIAN_POINT('Ctrl Pts',(38.5515985684988,-4.42149171724726,-1.4559840257378));
#90141=CARTESIAN_POINT('Ctrl Pts',(38.7504457872385,-1.16595910278014,-4.5066637171564));
#90142=CARTESIAN_POINT('Ctrl Pts',(38.9492930059781,3.1605996665157,-3.41761440728918));
#90143=CARTESIAN_POINT('Ctrl Pts',(39.1481402247178,4.58389630619673,0.81078550981488));
#90144=CARTESIAN_POINT('Ctrl Pts',(39.3469874434575,1.7965196698999,4.2944144611987));
#90145=CARTESIAN_POINT('Ctrl Pts',(39.545834662197,-2.64110314530594,3.8332822312928));
#90146=CARTESIAN_POINT('Ctrl Pts',(39.7446818809367,-4.65266269681899,-0.149024556764877));
#90147=CARTESIAN_POINT('Ctrl Pts',(39.9435290996763,-2.39038157415463,-3.99444043876384));
#90148=CARTESIAN_POINT('Ctrl Pts',(40.1423763184159,2.06765511132127,-4.17064513349156));
#90149=CARTESIAN_POINT('Ctrl Pts',(40.3412235371556,4.62638615382046,-0.515780616762658));
#90150=CARTESIAN_POINT('Ctrl Pts',(40.5400707558953,2.93541361643903,3.61286941215899));
#90151=CARTESIAN_POINT('Ctrl Pts',(40.7389179746349,-1.45196975640838,4.42281158488186));
#90152=CARTESIAN_POINT('Ctrl Pts',(40.9377651933746,-4.50560344504676,1.17004960786819));
#90153=CARTESIAN_POINT('Ctrl Pts',(41.1366124121142,-3.42048207664657,-3.15749597818099));
#90154=CARTESIAN_POINT('Ctrl Pts',(41.3354596308539,0.806624081336881,-4.58463041916116));
#90155=CARTESIAN_POINT('Ctrl Pts',(41.5343068495934,4.29278187658053,-1.80041724302757));
#90156=CARTESIAN_POINT('Ctrl Pts',(41.7331540683332,3.83567814933202,2.63762234287354));
#90157=CARTESIAN_POINT('Ctrl Pts',(41.9320012870728,-0.144800977314504,
4.65279605891583));
#90158=CARTESIAN_POINT('Ctrl Pts',(42.1308485058124,-3.99226889149313,2.3940065970881));
#90159=CARTESIAN_POINT('Ctrl Pts',(42.3296957245521,-4.17252035725389,-2.06386829938026));
#90160=CARTESIAN_POINT('Ctrl Pts',(42.5285429432917,-0.519980069410792,
-4.62591604077868));
#90161=CARTESIAN_POINT('Ctrl Pts',(42.7273901620314,3.61020326182819,-2.9386920384986));
#90162=CARTESIAN_POINT('Ctrl Pts',(42.926237380771,4.42412780796626,1.44795429059375));
#90163=CARTESIAN_POINT('Ctrl Pts',(43.1250845995107,1.17413914879181,4.50453946018377));
#90164=CARTESIAN_POINT('Ctrl Pts',(43.3239318182503,-3.15438968795409,3.42334692736563));
#90165=CARTESIAN_POINT('Ctrl Pts',(43.52277903699,-4.58536075423916,-0.802461988093299));
#90166=CARTESIAN_POINT('Ctrl Pts',(43.7216262557296,-1.80431333253019,-4.29114575471113));
#90167=CARTESIAN_POINT('Ctrl Pts',(43.9204734744692,2.63413936691317,-3.8380709063487));
#90168=CARTESIAN_POINT('Ctrl Pts',(44.1193206932088,4.65292558701255,0.140577277989422));
#90169=CARTESIAN_POINT('Ctrl Pts',(44.3181679119485,2.39762964714867,3.99009405551234));
#90170=CARTESIAN_POINT('Ctrl Pts',(44.5170151306882,-2.06007978649544,4.17439214068712));
#90171=CARTESIAN_POINT('Ctrl Pts',(44.7158623494278,-4.62544211628707,0.524179097453273));
#90172=CARTESIAN_POINT('Ctrl Pts',(44.9147095681674,-2.9419680380799,-3.60753414397816));
#90173=CARTESIAN_POINT('Ctrl Pts',(45.1135567869071,1.44393762990557,-4.42544037123081));
#90174=CARTESIAN_POINT('Ctrl Pts',(45.3124040056467,4.50347176669087,-1.17822774931598));
#90175=CARTESIAN_POINT('Ctrl Pts',(45.5112512243863,3.42620895087503,3.15128085030174));
#90176=CARTESIAN_POINT('Ctrl Pts',(45.710098443126,-0.798299221633414,4.58608721153467));
#90177=CARTESIAN_POINT('Ctrl Pts',(45.9089456618656,-4.28950611966511,1.80820812513962));
#90178=CARTESIAN_POINT('Ctrl Pts',(46.1077928806053,-3.84046045689732,-2.63065458364033));
#90179=CARTESIAN_POINT('Ctrl Pts',(46.306640099345,0.13635337910788,-4.65305058595005));
#90180=CARTESIAN_POINT('Ctrl Pts',(46.5054873180845,3.98791609169654,-2.40125205093354));
#90181=CARTESIAN_POINT('Ctrl Pts',(46.7043345368243,4.17626017793529,2.05629211917988));
#90182=CARTESIAN_POINT('Ctrl Pts',(46.9031817555638,0.528378279558735,4.62495951542089));
#90183=CARTESIAN_POINT('Ctrl Pts',(47.1020289743036,-3.60486317437669,2.945250919464));
#90184=CARTESIAN_POINT('Ctrl Pts',(47.3008761930431,-4.42674714342192,-1.43993758120542));
#90185=CARTESIAN_POINT('Ctrl Pts',(47.4997234117828,-1.18231948092862,-4.50236630858751));
#90186=CARTESIAN_POINT('Ctrl Pts',(47.6985706305225,3.14817726267048,-3.42913329311644));
#90187=CARTESIAN_POINT('Ctrl Pts',(47.8974178492621,4.58679487950342,0.794260410053871));
#90188=CARTESIAN_POINT('Ctrl Pts',(48.0962650680017,1.81213014044313,4.28762456725067));
#90189=CARTESIAN_POINT('Ctrl Pts',(48.2951122867414,-2.62722255147639,3.84330292215117));
#90190=CARTESIAN_POINT('Ctrl Pts',(48.493959505481,-4.65306675230442,-0.133002451839397));
#90191=CARTESIAN_POINT('Ctrl Pts',(48.6928067242207,-2.40507281684978,-3.98405898298613));
#90192=CARTESIAN_POINT('Ctrl Pts',(48.8916539429603,2.05288141093679,-4.1813817027399));
#90193=CARTESIAN_POINT('Ctrl Pts',(49.0905011617,4.62378860970624,-0.52589063841688));
#90194=CARTESIAN_POINT('Ctrl Pts',(49.2230659741931,3.50770681921098,2.21507238733057));
#90195=CARTESIAN_POINT('Ctrl Pts',(49.2893483804396,2.49297831328899,3.04566224204766));
#90196=CARTESIAN_POINT('Ctrl Pts',(0.312305742378132,2.14453946293883,-3.01048699365514));
#90197=CARTESIAN_POINT('Ctrl Pts',(0.37863252516784,3.14826970167303,-2.29555343657973));
#90198=CARTESIAN_POINT('Ctrl Pts',(0.511241714204097,4.36593527088205,0.204302641486374));
#90199=CARTESIAN_POINT('Ctrl Pts',(0.710133309486899,2.18381387565399,3.79044371220078));
#90200=CARTESIAN_POINT('Ctrl Pts',(0.908980528226543,-2.00579624292731,
3.88290810155421));
#90201=CARTESIAN_POINT('Ctrl Pts',(1.10782774696618,-4.35188837526965,0.414135666234644));
#90202=CARTESIAN_POINT('Ctrl Pts',(1.30667496570583,-2.70096649031909,-3.43791197611196));
#90203=CARTESIAN_POINT('Ctrl Pts',(1.50552218444547,1.43129106250514,-4.13047287675976));
#90204=CARTESIAN_POINT('Ctrl Pts',(1.70436940318511,4.2486459222133,-1.02964516288757));
#90205=CARTESIAN_POINT('Ctrl Pts',(1.90321662192475,3.16335903024921,3.01740079864124));
#90206=CARTESIAN_POINT('Ctrl Pts',(2.1020638406644,-0.827765141249585,4.29251126953189));
#90207=CARTESIAN_POINT('Ctrl Pts',(2.30091105940404,-4.05850005710013,1.62472009156678));
#90208=CARTESIAN_POINT('Ctrl Pts',(2.49975827814369,-3.56119098754892,-2.53556387370365));
#90209=CARTESIAN_POINT('Ctrl Pts',(2.69860549688333,0.207360974982843,-4.36670037323892));
#90210=CARTESIAN_POINT('Ctrl Pts',(2.89745271562298,3.78543237111287,-2.18669123306836));
#90211=CARTESIAN_POINT('Ctrl Pts',(3.09629993436261,3.88628469012808,2.00197600577016));
#90212=CARTESIAN_POINT('Ctrl Pts',(3.29514715310227,0.417274652083158,4.35166473784776));
#90213=CARTESIAN_POINT('Ctrl Pts',(3.49399437184191,-3.43503490463991,2.70400562836479));
#90214=CARTESIAN_POINT('Ctrl Pts',(3.69284159058154,-4.13199196762965,-1.4274988650365));
#90215=CARTESIAN_POINT('Ctrl Pts',(3.8916888093212,-1.0333857078201,-4.24773151317723));
#90216=CARTESIAN_POINT('Ctrl Pts',(4.09053602806083,3.01446743944127,-3.16608530458669));
#90217=CARTESIAN_POINT('Ctrl Pts',(4.28938324680048,4.29329256055578,0.823862198048239));
#90218=CARTESIAN_POINT('Ctrl Pts',(4.48823046554012,1.62838703848647,4.05702666826332));
#90219=CARTESIAN_POINT('Ctrl Pts',(4.68707768427977,-2.53232146155544,3.56348956881262));
#90220=CARTESIAN_POINT('Ctrl Pts',(4.88592490301941,-4.36689132952691,-0.203396098193201));
#90221=CARTESIAN_POINT('Ctrl Pts',(5.08477212175905,-2.190124246766,-3.78344626195841));
#90222=CARTESIAN_POINT('Ctrl Pts',(5.2836193404987,1.99844611755997,-3.88810017506377));
#90223=CARTESIAN_POINT('Ctrl Pts',(5.48246655923833,4.35128480394624,-0.421224885991602));
#90224=CARTESIAN_POINT('Ctrl Pts',(5.68131377797799,2.70712237646502,3.432578955528));
#90225=CARTESIAN_POINT('Ctrl Pts',(5.88016099671762,-1.42374722830323,4.13328606319474));
#90226=CARTESIAN_POINT('Ctrl Pts',(6.07900821545728,-4.24679178532139,1.03724123583069));
#90227=CARTESIAN_POINT('Ctrl Pts',(6.27785543419691,-3.16882037582503,-3.01159214946066));
#90228=CARTESIAN_POINT('Ctrl Pts',(6.47670265293655,0.81996453848499,-4.2940386590025));
#90229=CARTESIAN_POINT('Ctrl Pts',(6.6755498716762,4.05554681932371,-1.63206919138556));
#90230=CARTESIAN_POINT('Ctrl Pts',(6.87439709041584,3.56578684306324,2.52908561322399));
#90231=CARTESIAN_POINT('Ctrl Pts',(7.0732443091555,-0.199431905597023,4.36707416518995));
#90232=CARTESIAN_POINT('Ctrl Pts',(7.27209152789513,-3.78145658982552,2.1935578197247));
#90233=CARTESIAN_POINT('Ctrl Pts',(7.47093874663477,-3.88991268884659,-1.99491581836445));
#90234=CARTESIAN_POINT('Ctrl Pts',(7.66978596537443,-0.425174651109135,
-4.35090063840494));
#90235=CARTESIAN_POINT('Ctrl Pts',(7.86863318411405,3.43012011423786,-2.71023723151952));
#90236=CARTESIAN_POINT('Ctrl Pts',(8.06748040285371,4.13457678604175,1.41999459489774));
#90237=CARTESIAN_POINT('Ctrl Pts',(8.26632762159334,1.04109589173419,4.24584846566965));
#90238=CARTESIAN_POINT('Ctrl Pts',(8.46517484033299,-3.00871436873501,3.17155288409039));
#90239=CARTESIAN_POINT('Ctrl Pts',(8.66402205907265,-4.29478122376174,-0.816066228463263));
#90240=CARTESIAN_POINT('Ctrl Pts',(8.86286927781226,-1.63574999691905,-4.05406361528703));
#90241=CARTESIAN_POINT('Ctrl Pts',(9.06171649655193,2.52584767953922,-3.56808118587302));
#90242=CARTESIAN_POINT('Ctrl Pts',(9.26056371529156,4.36725340290968,0.195467552265011));
#90243=CARTESIAN_POINT('Ctrl Pts',(9.45941093403121,2.1969895847602,3.7794637997565));
#90244=CARTESIAN_POINT('Ctrl Pts',(9.65825815277085,-1.99138387510301,3.8917219981898));
#90245=CARTESIAN_POINT('Ctrl Pts',(9.85710537151049,-4.35051288766617,0.429124065353151));
#90246=CARTESIAN_POINT('Ctrl Pts',(10.0559525902501,-2.713349853193,-3.42765844613962));
#90247=CARTESIAN_POINT('Ctrl Pts',(10.2547998089898,1.4162407913405,-4.13586410199344));
#90248=CARTESIAN_POINT('Ctrl Pts',(10.4536470277294,4.24490164730402,-1.04494968966466));
#90249=CARTESIAN_POINT('Ctrl Pts',(10.6524942464691,3.17428277887788,3.00583410868497));
#90250=CARTESIAN_POINT('Ctrl Pts',(10.8513414652087,-0.812167245970631,
4.295520249491));
#90251=CARTESIAN_POINT('Ctrl Pts',(11.0501886839484,-4.05257707056199,1.63942945452676));
#90252=CARTESIAN_POINT('Ctrl Pts',(11.249035902688,-3.57037258845796,-2.52260766446206));
#90253=CARTESIAN_POINT('Ctrl Pts',(11.4478831214276,0.191503037860384,-4.36742904186261));
#90254=CARTESIAN_POINT('Ctrl Pts',(11.6467303401673,3.77746789527733,-2.20041953939783));
#90255=CARTESIAN_POINT('Ctrl Pts',(11.8455775589069,3.89352810061769,1.98785029087078));
#90256=CARTESIAN_POINT('Ctrl Pts',(12.0444247776466,0.433073125983973,4.3501215519529));
#90257=CARTESIAN_POINT('Ctrl Pts',(12.2432719963862,-3.42519395353086,2.71646023897098));
#90258=CARTESIAN_POINT('Ctrl Pts',(12.4421192151259,-4.13714800984828,-1.41248582075117));
#90259=CARTESIAN_POINT('Ctrl Pts',(12.6409664338655,-1.04880262652003,-4.2439513309909));
#90260=CARTESIAN_POINT('Ctrl Pts',(12.8398136526051,3.00295137172242,-3.17701005794523));
#90261=CARTESIAN_POINT('Ctrl Pts',(13.0386608713448,4.29625573556119,0.808267594223766));
#90262=CARTESIAN_POINT('Ctrl Pts',(13.2375080900844,1.64310756118719,4.05108718637159));
#90263=CARTESIAN_POINT('Ctrl Pts',(13.4363553088241,-2.51936557066787,3.57266104893089));
#90264=CARTESIAN_POINT('Ctrl Pts',(13.6352025275637,-4.36760108190112,-0.187538365650509));
#90265=CARTESIAN_POINT('Ctrl Pts',(13.8340497463034,-2.20384768081277,-3.77546887803236));
#90266=CARTESIAN_POINT('Ctrl Pts',(14.032896965043,1.98431506858032,-3.89533099464214));
#90267=CARTESIAN_POINT('Ctrl Pts',(14.2317441837827,4.34972663158719,-0.437021829747384));
#90268=CARTESIAN_POINT('Ctrl Pts',(14.4305914025223,2.71956838629063,3.42272663844241));
#90269=CARTESIAN_POINT('Ctrl Pts',(14.6294386212619,-1.40872968622409,4.13842850854834));
#90270=CARTESIAN_POINT('Ctrl Pts',(14.8282858400016,-4.24299751751331,1.05265469912532));
#90271=CARTESIAN_POINT('Ctrl Pts',(15.0271330587412,-3.17973471904507,-3.00006616022283));
#90272=CARTESIAN_POINT('Ctrl Pts',(15.2259802774809,0.804367276436096,-4.29698768136627));
#90273=CARTESIAN_POINT('Ctrl Pts',(15.4248274962205,4.04959396394355,-1.6467843138695));
#90274=CARTESIAN_POINT('Ctrl Pts',(15.6236747149602,3.57494656540606,2.51612140082828));
#90275=CARTESIAN_POINT('Ctrl Pts',(15.8225219336998,-0.183573538902467,
4.36776952288344));
#90276=CARTESIAN_POINT('Ctrl Pts',(16.0213691524394,-3.77346674966885,2.20727400618009));
#90277=CARTESIAN_POINT('Ctrl Pts',(16.2202163711791,-3.89713067877753,-1.98077821114473));
#90278=CARTESIAN_POINT('Ctrl Pts',(16.4190635899187,-0.440970173389522,
-4.34932812689449));
#90279=CARTESIAN_POINT('Ctrl Pts',(16.6179108086584,3.42025650290739,-2.72267429259073));
#90280=CARTESIAN_POINT('Ctrl Pts',(16.816758027398,4.13970559703845,1.40497239085444));
#90281=CARTESIAN_POINT('Ctrl Pts',(17.0156052461377,1.05650590430629,4.24204020765723));
#90282=CARTESIAN_POINT('Ctrl Pts',(17.2144524648773,-2.99717847656365,3.18245675993221));
#90283=CARTESIAN_POINT('Ctrl Pts',(17.4132996836169,-4.2977160863031,-0.800466295821592));
#90284=CARTESIAN_POINT('Ctrl Pts',(17.6121469023566,-1.65045970954389,-4.04809740450832));
#90285=CARTESIAN_POINT('Ctrl Pts',(17.8109941210962,2.51287515761657,-3.57722913600011));
#90286=CARTESIAN_POINT('Ctrl Pts',(18.0098413398359,4.3679343646708,0.179608560883422));
#90287=CARTESIAN_POINT('Ctrl Pts',(18.2086885585755,2.21069851267633,3.77146151183666));
#90288=CARTESIAN_POINT('Ctrl Pts',(18.4075357773152,-1.97723972147858,3.89892715154078));
#90289=CARTESIAN_POINT('Ctrl Pts',(18.6063829960548,-4.34892603820315,0.444918153656803));
#90290=CARTESIAN_POINT('Ctrl Pts',(18.8052302147944,-2.72577795531192,-3.41778354896127));
#90291=CARTESIAN_POINT('Ctrl Pts',(19.0040774335341,1.40121393773835,-4.14097927426623));
#90292=CARTESIAN_POINT('Ctrl Pts',(19.2029246522737,4.24107940221153,-1.0603562388894));
#90293=CARTESIAN_POINT('Ctrl Pts',(19.4017718710134,3.18517617836356,2.99428832312454));
#90294=CARTESIAN_POINT('Ctrl Pts',(19.600619089753,-0.796564655594856,4.2984409497714));
#90295=CARTESIAN_POINT('Ctrl Pts',(19.7994663084927,-4.04659750929911,1.65413374518173));
#90296=CARTESIAN_POINT('Ctrl Pts',(19.9983135272323,-3.57950875883217,-2.50962684370774));
#90297=CARTESIAN_POINT('Ctrl Pts',(20.197160745972,0.175643434860611,-4.36809560712733));
#90298=CARTESIAN_POINT('Ctrl Pts',(20.3960079647116,3.76945316618819,-2.2141211974796));
#90299=CARTESIAN_POINT('Ctrl Pts',(20.5948551834513,3.90072041145158,1.97369960249772));
#90300=CARTESIAN_POINT('Ctrl Pts',(20.7937024021909,0.448865767295954,4.34852036584451));
#90301=CARTESIAN_POINT('Ctrl Pts',(20.9925496209305,-3.41530777864185,2.72887937189667));
#90302=CARTESIAN_POINT('Ctrl Pts',(21.1913968396701,-4.14224953918214,-1.39745432997289));
#90303=CARTESIAN_POINT('Ctrl Pts',(21.3902440584098,-1.06420569970189,-4.24011510196797));
#90304=CARTESIAN_POINT('Ctrl Pts',(21.5890912771495,2.99139570228704,-3.18789297209824));
#90305=CARTESIAN_POINT('Ctrl Pts',(21.7879384958891,4.2991622711739,0.792662358970985));
#90306=CARTESIAN_POINT('Ctrl Pts',(21.9867857146287,1.65780641775542,4.04509427955192));
#90307=CARTESIAN_POINT('Ctrl Pts',(22.1856329333684,-2.50637646177856,3.58178543202368));
#90308=CARTESIAN_POINT('Ctrl Pts',(22.384480152108,-4.36825325012018,-0.171678164101458));
#90309=CARTESIAN_POINT('Ctrl Pts',(22.5833273708477,-2.21754205776954,-3.76744171437834));
#90310=CARTESIAN_POINT('Ctrl Pts',(22.7821745895873,1.97015785711929,-3.90251045703222));
#90311=CARTESIAN_POINT('Ctrl Pts',(22.981021808327,4.34811111015288,-0.452813011053976));
#90312=CARTESIAN_POINT('Ctrl Pts',(23.1798690270666,2.73197853978927,3.41282919398928));
#90313=CARTESIAN_POINT('Ctrl Pts',(23.3787162458063,-1.39369357065614,4.14351639073943));
#90314=CARTESIAN_POINT('Ctrl Pts',(23.5775634645459,-4.23914730772107,1.06805428357167));
#90315=CARTESIAN_POINT('Ctrl Pts',(23.7764106832856,-3.19060713889759,-2.9885006164347));
#90316=CARTESIAN_POINT('Ctrl Pts',(23.9752579020252,0.788759409165555,-4.29988004991624));
#90317=CARTESIAN_POINT('Ctrl Pts',(24.1741051207649,4.04358771650543,-1.66147772423859));
#90318=CARTESIAN_POINT('Ctrl Pts',(24.3729523395044,3.58405915369861,2.50312401450745));
#90319=CARTESIAN_POINT('Ctrl Pts',(24.5717995582441,-0.167712751873498,
4.36840729351942));
#90320=CARTESIAN_POINT('Ctrl Pts',(24.7706467769837,-3.7654271580646,2.2209610907272));
#90321=CARTESIAN_POINT('Ctrl Pts',(24.9694939957234,-3.90429728680765,-1.96661448826176));
#90322=CARTESIAN_POINT('Ctrl Pts',(25.1683412144631,-0.456759881678285,
-4.34769827146548));
#90323=CARTESIAN_POINT('Ctrl Pts',(25.3671884332027,3.41034779704597,-2.73507545643596));
#90324=CARTESIAN_POINT('Ctrl Pts',(25.5660356519423,4.14477982789419,1.3899316628871));
#90325=CARTESIAN_POINT('Ctrl Pts',(25.764882870682,1.07190198732727,4.23817602026845));
#90326=CARTESIAN_POINT('Ctrl Pts',(25.9637300894216,-2.98560306795325,3.19331867652491));
#90327=CARTESIAN_POINT('Ctrl Pts',(26.1625773081612,-4.30059428540685,-0.784855809394697));
#90328=CARTESIAN_POINT('Ctrl Pts',(26.3614245269009,-1.66514766160607,-4.04207782140107));
#90329=CARTESIAN_POINT('Ctrl Pts',(26.5602717456405,2.49986950457442,-3.5863299219834));
#90330=CARTESIAN_POINT('Ctrl Pts',(26.7591189643802,4.36855773719815,0.163747201444247));
#90331=CARTESIAN_POINT('Ctrl Pts',(26.9579661831198,2.22437829353522,3.7634094989071));
#90332=CARTESIAN_POINT('Ctrl Pts',(27.1568134018595,-1.96306949884509,3.90608089930546));
#90333=CARTESIAN_POINT('Ctrl Pts',(27.3556606205991,-4.34728185012251,0.460706375916406));
#90334=CARTESIAN_POINT('Ctrl Pts',(27.5545078393388,-2.73817011928469,-3.40786358985672));
#90335=CARTESIAN_POINT('Ctrl Pts',(27.7533550580784,1.38616860976576,-4.14603984960525));
#90336=CARTESIAN_POINT('Ctrl Pts',(27.952202276818,4.23720124041042,-1.0757488077981));
#90337=CARTESIAN_POINT('Ctrl Pts',(28.1510494955577,3.19602758274585,2.9827030592304));
#90338=CARTESIAN_POINT('Ctrl Pts',(28.3498967142973,-0.780951562875272,
4.30130497705724));
#90339=CARTESIAN_POINT('Ctrl Pts',(28.548743933037,-4.04056459548315,1.66881622683348));
#90340=CARTESIAN_POINT('Ctrl Pts',(28.7475911517766,-3.58859773500673,-2.49661293466152));
#90341=CARTESIAN_POINT('Ctrl Pts',(28.9464383705163,0.159781516081698,-4.36870458103238));
#90342=CARTESIAN_POINT('Ctrl Pts',(29.1452855892559,3.76138873856841,-2.22779366337761));
#90343=CARTESIAN_POINT('Ctrl Pts',(29.3441328079956,3.90786129305586,1.95952289179036));
#90344=CARTESIAN_POINT('Ctrl Pts',(29.5429800267352,0.464652490516438,4.34686184646714));
#90345=CARTESIAN_POINT('Ctrl Pts',(29.7418272454748,-3.40537657446858,2.74126252578542));
#90346=CARTESIAN_POINT('Ctrl Pts',(29.9406744642145,-4.14729645483434,-1.38240441439296));
#90347=CARTESIAN_POINT('Ctrl Pts',(30.1395216829541,-1.07959474181426,-4.23622296895025));
#90348=CARTESIAN_POINT('Ctrl Pts',(30.3383689016938,2.97980059265583,-3.19873385532817));
#90349=CARTESIAN_POINT('Ctrl Pts',(30.5372161204335,4.30201212428175,0.777046672824416));
#90350=CARTESIAN_POINT('Ctrl Pts',(30.736063339173,1.67248341689788,4.03904803999856));
#90351=CARTESIAN_POINT('Ctrl Pts',(30.9349105579127,-2.49335430745217,3.59086259089991));
#90352=CARTESIAN_POINT('Ctrl Pts',(31.1337577766523,-4.3688478249011,-0.155815699053587));
#90353=CARTESIAN_POINT('Ctrl Pts',(31.332604995392,-2.23120719744001,-3.75936487871377));
#90354=CARTESIAN_POINT('Ctrl Pts',(31.5314522141316,1.95597467002026,-3.90963846659173));
#90355=CARTESIAN_POINT('Ctrl Pts',(31.7302994328713,4.34643826084541,-0.468598222226493));
#90356=CARTESIAN_POINT('Ctrl Pts',(31.9291466516109,2.7443526733899,3.40288675293087));
#90357=CARTESIAN_POINT('Ctrl Pts',(32.1279938703505,-1.37863907987046,4.14854964254603));
#90358=CARTESIAN_POINT('Ctrl Pts',(32.3268410890903,-4.23524120669408,1.08343978620659));
#90359=CARTESIAN_POINT('Ctrl Pts',(32.5256883078298,-3.20143749204183,-2.97689567062125));
#90360=CARTESIAN_POINT('Ctrl Pts',(32.7245355265695,0.773141142459902,-4.30271572649768));
#90361=CARTESIAN_POINT('Ctrl Pts',(32.9233827453091,4.03752815619699,-1.67614922877742));
#90362=CARTESIAN_POINT('Ctrl Pts',(33.1222299640488,3.5931244877966,2.49009362563158));
#90363=CARTESIAN_POINT('Ctrl Pts',(33.3210771827884,-0.151849753627885,
4.36898746868628));
#90364=CARTESIAN_POINT('Ctrl Pts',(33.5199244015281,-3.75733792101087,2.23461889290957));
#90365=CARTESIAN_POINT('Ctrl Pts',(33.7187716202677,-3.91141241844866,-1.95242483645857));
#90366=CARTESIAN_POINT('Ctrl Pts',(33.9176188390074,-0.472543567795172,
-4.34601109360641));
#90367=CARTESIAN_POINT('Ctrl Pts',(34.116466057747,3.40039412729541,-2.74744055955165));
#90368=CARTESIAN_POINT('Ctrl Pts',(34.3153132764867,4.14979941170753,1.37487260930113));
#90369=CARTESIAN_POINT('Ctrl Pts',(34.5141604952263,1.08728393780662,4.23425595445086));
#90370=CARTESIAN_POINT('Ctrl Pts',(34.713007713966,-2.97398829552043,3.20413849065896));
#90371=CARTESIAN_POINT('Ctrl Pts',(34.9118549327056,-4.30341578312523,-0.769234975000029));
#90372=CARTESIAN_POINT('Ctrl Pts',(35.1107021514452,-1.67981365945132,-4.03600494533089));
#90373=CARTESIAN_POINT('Ctrl Pts',(35.3095493701849,2.48683089188669,-3.59538342383295));
#90374=CARTESIAN_POINT('Ctrl Pts',(35.5083965889245,4.36912351227285,0.147883683072671));
#90375=CARTESIAN_POINT('Ctrl Pts',(35.7072438076642,2.23802874697494,3.75530786712999));
#90376=CARTESIAN_POINT('Ctrl Pts',(35.9060910264038,-1.94887339403047,3.91318314716482));
#90377=CARTESIAN_POINT('Ctrl Pts',(36.1049382451435,-4.34558034510215,0.476488523971419));
#90378=CARTESIAN_POINT('Ctrl Pts',(36.3037854638831,-2.7505261817262,-3.39789869961619));
#90379=CARTESIAN_POINT('Ctrl Pts',(36.5026326826227,1.37110500578868,-4.15104576128906));
#90380=CARTESIAN_POINT('Ctrl Pts',(36.7014799013624,4.2332672130325,-1.09112719344661));
#90381=CARTESIAN_POINT('Ctrl Pts',(36.900327120102,3.20683684895383,2.97107846974908));
#90382=CARTESIAN_POINT('Ctrl Pts',(37.0991743388417,-0.765328173663516,
4.30411229358757));
#90383=CARTESIAN_POINT('Ctrl Pts',(37.2980215575813,-4.03447840865544,1.6834767059));
#90384=CARTESIAN_POINT('Ctrl Pts',(37.496868776321,-3.59763939714749,-2.48356610890607));
#90385=CARTESIAN_POINT('Ctrl Pts',(37.6957159950606,0.143917490656121,-4.36925595554871));
#90386=CARTESIAN_POINT('Ctrl Pts',(37.8945632138002,3.75327471874399,-2.24143675682628));
#90387=CARTESIAN_POINT('Ctrl Pts',(38.0934104325399,3.91495065128109,1.94532034566247));
#90388=CARTESIAN_POINT('Ctrl Pts',(38.2922576512795,0.480433087504437,4.34514601568757));
#90389=CARTESIAN_POINT('Ctrl Pts',(38.4911048700192,-3.39540047194947,2.75360953737089));
#90390=CARTESIAN_POINT('Ctrl Pts',(38.6899520887588,-4.15228869026357,-1.36733627243771));
#90391=CARTESIAN_POINT('Ctrl Pts',(38.8887993074985,-1.09496954995957,-4.2322749832538));
#90392=CARTESIAN_POINT('Ctrl Pts',(39.0876465262381,2.96816619570515,-3.20953256470283));
#90393=CARTESIAN_POINT('Ctrl Pts',(39.2864937449777,4.30480525731066,0.76142074166985));
#90394=CARTESIAN_POINT('Ctrl Pts',(39.4853409637174,1.68713836510498,4.03294854742849));
#90395=CARTESIAN_POINT('Ctrl Pts',(39.684188182457,-2.48029927938,3.59989240588131));
#90396=CARTESIAN_POINT('Ctrl Pts',(39.8830354011967,-4.36938479840474,-0.139951179646495));
#90397=CARTESIAN_POINT('Ctrl Pts',(40.0818826199362,-2.24484291965528,-3.75123847752822));
#90398=CARTESIAN_POINT('Ctrl Pts',(40.280729838676,1.9417656942824,-3.916714929341));
#90399=CARTESIAN_POINT('Ctrl Pts',(40.4795770574156,4.34470810572058,-0.484377255143766));
#90400=CARTESIAN_POINT('Ctrl Pts',(40.6784242761552,2.75669062394493,3.39289944635391));
#90401=CARTESIAN_POINT('Ctrl Pts',(40.8772714948949,-1.36356641235379,4.15352819760686));
#90402=CARTESIAN_POINT('Ctrl Pts',(41.0761187136345,-4.23127926593237,1.09881100417926));
#90403=CARTESIAN_POINT('Ctrl Pts',(41.2749659323742,-3.21222563568464,-2.96525147578833));
#90404=CARTESIAN_POINT('Ctrl Pts',(41.4738131511138,0.757512682238883,-4.30549467372362));
#90405=CARTESIAN_POINT('Ctrl Pts',(41.6726603698535,4.0314153629108,-1.69079863404868));
#90406=CARTESIAN_POINT('Ctrl Pts',(41.8715075885931,3.60214244817772,2.47703040600029));
#90407=CARTESIAN_POINT('Ctrl Pts',(42.0703548073327,-0.135984753312187,
4.36951004073511));
#90408=CARTESIAN_POINT('Ctrl Pts',(42.2692020260724,-3.74919914516051,2.24824723265442));
#90409=CARTESIAN_POINT('Ctrl Pts',(42.4680492448121,-3.91847597989089,-1.93820944281791));
#90410=CARTESIAN_POINT('Ctrl Pts',(42.6668964635516,-0.488321023638938,
-4.3442666155649));
#90411=CARTESIAN_POINT('Ctrl Pts',(42.8657436822913,3.39039562488978,-2.75976943890386));
#90412=CARTESIAN_POINT('Ctrl Pts',(43.064590901031,4.15476428229879,1.3597954286328));
#90413=CARTESIAN_POINT('Ctrl Pts',(43.2634381197705,1.10265155293779,4.230280061909));
#90414=CARTESIAN_POINT('Ctrl Pts',(43.4622853385103,-2.96233431239582,3.21491605964126));
#90415=CARTESIAN_POINT('Ctrl Pts',(43.6611325572498,-4.30618054226719,-0.75360399851666));
#90416=CARTESIAN_POINT('Ctrl Pts',(43.8599797759895,-1.69445750969802,-4.02987885650785));
#90417=CARTESIAN_POINT('Ctrl Pts',(44.0588269947292,2.47375949142812,-3.60438952191081));
#90418=CARTESIAN_POINT('Ctrl Pts',(44.2576742134688,4.3696316824989,0.132018214401751));
#90419=CARTESIAN_POINT('Ctrl Pts',(44.4565214322085,2.25164969289924,3.74715672431622));
#90420=CARTESIAN_POINT('Ctrl Pts',(44.6553686509481,-1.93465159397174,3.92023379957652));
#90421=CARTESIAN_POINT('Ctrl Pts',(44.8542158696878,-4.34382154601996,0.492264393380623));
#90422=CARTESIAN_POINT('Ctrl Pts',(45.0530630884273,-2.76284597887739,-3.38788901658417));
#90423=CARTESIAN_POINT('Ctrl Pts',(45.2519103071671,1.35602332278828,-4.15599692999943));
#90424=CARTESIAN_POINT('Ctrl Pts',(45.4507575259067,4.22927737505606,-1.10649121855319));
#90425=CARTESIAN_POINT('Ctrl Pts',(45.6496047446464,3.21760382852318,2.95941475667813));
#90426=CARTESIAN_POINT('Ctrl Pts',(45.8484519633859,-0.74969468256698,4.30686276912748));
#90427=CARTESIAN_POINT('Ctrl Pts',(46.0472991821257,-4.02833905082843,1.69811516741566));
#90428=CARTESIAN_POINT('Ctrl Pts',(46.2461464008652,-3.60663358440201,-2.4704868795819));
#90429=CARTESIAN_POINT('Ctrl Pts',(46.4449936196049,0.128051488084874,-4.36974907086184));
#90430=CARTESIAN_POINT('Ctrl Pts',(46.6438408383445,3.74511136607549,-2.25505154621694));
#90431=CARTESIAN_POINT('Ctrl Pts',(46.8426880570842,3.92198810116398,1.93109453921225));
#90432=CARTESIAN_POINT('Ctrl Pts',(47.0415352758238,0.496207907805146,4.3433683283625));
#90433=CARTESIAN_POINT('Ctrl Pts',(47.2403824945635,-3.38538066927122,2.76592898165438));
#90434=CARTESIAN_POINT('Ctrl Pts',(47.4392297133031,-4.15722413921679,-1.352266817509));
#90435=CARTESIAN_POINT('Ctrl Pts',(47.6380769320427,-1.1103338246204,-4.22823922289527));
#90436=CARTESIAN_POINT('Ctrl Pts',(47.8369241507824,2.95650013133344,-3.22035012185404));
#90437=CARTESIAN_POINT('Ctrl Pts',(48.035771369522,4.30752735065132,0.745901774490634));
#90438=CARTESIAN_POINT('Ctrl Pts',(48.2346185882617,1.70179839037054,4.02657205694712));
#90439=CARTESIAN_POINT('Ctrl Pts',(48.4334658070014,-2.4672638070873,3.60930298583502));
#90440=CARTESIAN_POINT('Ctrl Pts',(48.6323130257409,-4.36976425292589,-0.124904582404934));
#90441=CARTESIAN_POINT('Ctrl Pts',(48.8311602444807,-2.25863968436503,-3.7414890978684));
#90442=CARTESIAN_POINT('Ctrl Pts',(49.0300074632203,1.92789149232914,-3.92679780134734));
#90443=CARTESIAN_POINT('Ctrl Pts',(49.2288546819599,4.34226871337571,-0.493871726977649));
#90444=CARTESIAN_POINT('Ctrl Pts',(49.361419494453,3.29413968985974,2.08020745264537));
#90445=CARTESIAN_POINT('Ctrl Pts',(49.4277019006995,2.34119304463769,2.86022674942168));
#90446=CARTESIAN_POINT('Ctrl Pts',(0.450659262638117,2.00550372675239,-2.81530976205099));
#90447=CARTESIAN_POINT('Ctrl Pts',(0.516986045427824,2.94415968026748,-2.14672709529502));
#90448=CARTESIAN_POINT('Ctrl Pts',(0.649595234464078,4.08288101377022,0.191057201775436));
#90449=CARTESIAN_POINT('Ctrl Pts',(0.848486829746883,2.04223188327633,3.54469997975543));
#90450=CARTESIAN_POINT('Ctrl Pts',(1.04733404848652,-1.87575556888288,3.63116967669737));
#90451=CARTESIAN_POINT('Ctrl Pts',(1.24618126722617,-4.06974481274113,0.387286238545933));
#90452=CARTESIAN_POINT('Ctrl Pts',(1.44502848596581,-2.525856229638,-3.21502373795952));
#90453=CARTESIAN_POINT('Ctrl Pts',(1.64387570470545,1.33849696381325,-3.86268422229914));
#90454=CARTESIAN_POINT('Ctrl Pts',(1.8427229234451,3.97319582031557,-0.962890749780876));
#90455=CARTESIAN_POINT('Ctrl Pts',(2.04157014218474,2.95827073078296,2.82177532815739));
#90456=CARTESIAN_POINT('Ctrl Pts',(2.24041736092439,-0.77409910348615,4.01421726992893));
#90457=CARTESIAN_POINT('Ctrl Pts',(2.43926457966403,-3.79537757649156,1.51938551604069));
#90458=CARTESIAN_POINT('Ctrl Pts',(2.63811179840367,-3.33031026970215,-2.3711770690211));
#90459=CARTESIAN_POINT('Ctrl Pts',(2.83695901714332,0.193917256034556,-4.08359651267085));
#90460=CARTESIAN_POINT('Ctrl Pts',(3.03580623588295,3.54001353616159,-2.04492269457519));
#90461=CARTESIAN_POINT('Ctrl Pts',(3.2346534546226,3.63432735277917,1.87218300704005));
#90462=CARTESIAN_POINT('Ctrl Pts',(3.43350067336224,0.390221716267934,4.06953567428003));
#90463=CARTESIAN_POINT('Ctrl Pts',(3.63234789210189,-3.21233319406464,2.52869833293435));
#90464=CARTESIAN_POINT('Ctrl Pts',(3.83119511084153,-3.86410482679418,-1.33495062377738));
#90465=CARTESIAN_POINT('Ctrl Pts',(4.03004232958118,-0.966388786040835,
-3.97234069465277));
#90466=CARTESIAN_POINT('Ctrl Pts',(4.22888954832082,2.8190321458056,-2.96082025409016));
#90467=CARTESIAN_POINT('Ctrl Pts',(4.42773676706046,4.01494790794569,0.770449197634163));
#90468=CARTESIAN_POINT('Ctrl Pts',(4.62658398580011,1.52281472582692,3.79399971105506));
#90469=CARTESIAN_POINT('Ctrl Pts',(4.82543120453975,-2.36814487037926,3.33245982832313));
#90470=CARTESIAN_POINT('Ctrl Pts',(5.02427842327939,-4.08377508879584,-0.19020943190021));
#90471=CARTESIAN_POINT('Ctrl Pts',(5.22312564201904,-2.04813313760203,-3.53815619131909));
#90472=CARTESIAN_POINT('Ctrl Pts',(5.42197286075868,1.86888197011213,-3.63602513538813));
#90473=CARTESIAN_POINT('Ctrl Pts',(5.62082007949833,4.06918037242217,-0.393915846854869));
#90474=CARTESIAN_POINT('Ctrl Pts',(5.81966729823796,2.53161301463566,3.21003647013777));
#90475=CARTESIAN_POINT('Ctrl Pts',(6.01851451697762,-1.33144221482525,3.86531502298008));
#90476=CARTESIAN_POINT('Ctrl Pts',(6.21736173571725,-3.97146189165121,0.969994350744806));
#90477=CARTESIAN_POINT('Ctrl Pts',(6.4162089544569,-2.96337800397363,-2.81634326790372));
#90478=CARTESIAN_POINT('Ctrl Pts',(6.61505617319654,0.766804232869096,-4.01564563500611));
#90479=CARTESIAN_POINT('Ctrl Pts',(6.81390339193619,3.79261580434003,-1.52625815575171));
#90480=CARTESIAN_POINT('Ctrl Pts',(7.01275061067582,3.33460816466789,2.36511881000589));
#90481=CARTESIAN_POINT('Ctrl Pts',(7.21159782941548,-0.186502247601397,
4.08394607077586));
#90482=CARTESIAN_POINT('Ctrl Pts',(7.41044504815511,-3.53629551449476,2.0513441036317));
#90483=CARTESIAN_POINT('Ctrl Pts',(7.60929226689476,-3.63772013947132,-1.86558054884406));
#90484=CARTESIAN_POINT('Ctrl Pts',(7.80813948563441,-0.39760953904375,-4.0688211132721));
#90485=CARTESIAN_POINT('Ctrl Pts',(8.00698670437404,3.20773704153966,-2.53452592602202));
#90486=CARTESIAN_POINT('Ctrl Pts',(8.20583392311369,3.86652206510947,1.32793287381758));
#90487=CARTESIAN_POINT('Ctrl Pts',(8.40468114185334,0.973599099882512,3.97057972971866));
#90488=CARTESIAN_POINT('Ctrl Pts',(8.60352836059298,-2.8136520607379,2.96593335704791));
#90489=CARTESIAN_POINT('Ctrl Pts',(8.80237557933261,-4.01634005747664,-0.763158659816362));
#90490=CARTESIAN_POINT('Ctrl Pts',(9.00122279807226,-1.52970032566391,-3.79122876004706));
#90491=CARTESIAN_POINT('Ctrl Pts',(9.20007001681191,2.36209079947775,-3.33675375962428));
#90492=CARTESIAN_POINT('Ctrl Pts',(9.39891723555156,4.08411368807603,0.182794912987637));
#90493=CARTESIAN_POINT('Ctrl Pts',(9.59776445429119,2.05455337895022,3.53443192187775));
#90494=CARTESIAN_POINT('Ctrl Pts',(9.79661167303084,-1.86227759009887,3.63941214686655));
#90495=CARTESIAN_POINT('Ctrl Pts',(9.99545889177048,-4.06845850136166,0.401302903107108));
#90496=CARTESIAN_POINT('Ctrl Pts',(10.1943061105101,-2.53743674882291,-3.20543496940232));
#90497=CARTESIAN_POINT('Ctrl Pts',(10.3931533292497,1.32442243852197,-3.86772592122086));
#90498=CARTESIAN_POINT('Ctrl Pts',(10.5920005479894,3.96969429590236,-0.977203046671689));
#90499=CARTESIAN_POINT('Ctrl Pts',(10.790847766729,2.96848626608251,2.81095853498833));
#90500=CARTESIAN_POINT('Ctrl Pts',(10.9896949854687,-0.759512457890662,
4.01703117036116));
#90501=CARTESIAN_POINT('Ctrl Pts',(11.1885422042083,-3.78983859165073,1.53314123503966));
#90502=CARTESIAN_POINT('Ctrl Pts',(11.387389422948,-3.33889660497779,-2.35906084249899));
#90503=CARTESIAN_POINT('Ctrl Pts',(11.5862366416876,0.179087427744,-4.08427793992626));
#90504=CARTESIAN_POINT('Ctrl Pts',(11.7850838604272,3.53256541676539,-2.05776096124341));
#90505=CARTESIAN_POINT('Ctrl Pts',(11.9839310791669,3.64110115525862,1.85897309677104));
#90506=CARTESIAN_POINT('Ctrl Pts',(12.1827782979065,0.404995936482876,4.06809253689939));
#90507=CARTESIAN_POINT('Ctrl Pts',(12.3816255166462,-3.2031302558744,2.54034548068687));
#90508=CARTESIAN_POINT('Ctrl Pts',(12.5804727353858,-3.86892659019068,-1.3209109118558));
#90509=CARTESIAN_POINT('Ctrl Pts',(12.7793199541254,-0.980806188211366,
-3.96880559091908));
#90510=CARTESIAN_POINT('Ctrl Pts',(12.9781671728651,2.80826269291056,-2.97103672898048));
#90511=CARTESIAN_POINT('Ctrl Pts',(13.1770143916047,4.01771897307136,0.755865630100106));
#90512=CARTESIAN_POINT('Ctrl Pts',(13.3758616103444,1.53658088105336,3.78844530029476));
#90513=CARTESIAN_POINT('Ctrl Pts',(13.574708829084,-2.35602894157149,3.34103669896361));
#90514=CARTESIAN_POINT('Ctrl Pts',(13.7735560478237,-4.08443882618849,-0.175379794926021));
#90515=CARTESIAN_POINT('Ctrl Pts',(13.9724032665633,-2.06096684786957,-3.53069600069545));
#90516=CARTESIAN_POINT('Ctrl Pts',(14.171250485303,1.8556670715843,-3.6427871632559));
#90517=CARTESIAN_POINT('Ctrl Pts',(14.3700977040426,4.06772322018647,-0.408688636127811));
#90518=CARTESIAN_POINT('Ctrl Pts',(14.5689449227822,2.54325211921723,3.20082290285502));
#90519=CARTESIAN_POINT('Ctrl Pts',(14.7677921415219,-1.31739829671282,3.87012407102955));
#90520=CARTESIAN_POINT('Ctrl Pts',(14.9666393602615,-3.96791361550106,0.984408521532401));
#90521=CARTESIAN_POINT('Ctrl Pts',(15.1654865790012,-2.97358474364017,-2.80556453672602));
#90522=CARTESIAN_POINT('Ctrl Pts',(15.3643337977408,0.752218179449807,-4.0184034650405));
#90523=CARTESIAN_POINT('Ctrl Pts',(15.5631810164805,3.78704888712724,-1.54001926087062));
#90524=CARTESIAN_POINT('Ctrl Pts',(15.7620282352201,3.34317403981824,2.35299509919369));
#90525=CARTESIAN_POINT('Ctrl Pts',(15.9608754539597,-0.17167201758895,4.08459634673013));
#90526=CARTESIAN_POINT('Ctrl Pts',(16.1597226726994,-3.52882367520839,2.06417103618691));
#90527=CARTESIAN_POINT('Ctrl Pts',(16.358569891439,-3.64447016946904,-1.85235951726291));
#90528=CARTESIAN_POINT('Ctrl Pts',(16.5574171101787,-0.412380998999033,
-4.06735055152723));
#90529=CARTESIAN_POINT('Ctrl Pts',(16.7562643289183,3.19851291224554,-2.54615666201882));
#90530=CARTESIAN_POINT('Ctrl Pts',(16.955111547658,3.87131836275072,1.31388459598752));
#90531=CARTESIAN_POINT('Ctrl Pts',(17.1539587663976,0.988010043666368,3.96701837038329));
#90532=CARTESIAN_POINT('Ctrl Pts',(17.3528059851373,-2.80286406865807,2.97613030796197));
#90533=CARTESIAN_POINT('Ctrl Pts',(17.5516532038769,-4.01908464570452,-0.748570108945357));
#90534=CARTESIAN_POINT('Ctrl Pts',(17.7505004226165,-1.54345637165813,-3.78564935329887));
#90535=CARTESIAN_POINT('Ctrl Pts',(17.9493476413562,2.34995931786557,-3.34530862578044));
#90536=CARTESIAN_POINT('Ctrl Pts',(18.1481948600958,4.08475050142141,0.167964098788153));
#90537=CARTESIAN_POINT('Ctrl Pts',(18.3470420788355,2.06737352355503,3.52694844184712));
#90538=CARTESIAN_POINT('Ctrl Pts',(18.5458892975751,-1.84905043653246,3.64615017251118));
#90539=CARTESIAN_POINT('Ctrl Pts',(18.7447365163148,-4.06697453122874,0.41607302205387));
#90540=CARTESIAN_POINT('Ctrl Pts',(18.9435837350544,-2.54905910669821,-3.19620028594943));
#90541=CARTESIAN_POINT('Ctrl Pts',(19.1424309537941,1.31036981257533,-3.87250946437004));
#90542=CARTESIAN_POINT('Ctrl Pts',(19.3412781725337,3.96611985630356,-0.991610751645455));
#90543=CARTESIAN_POINT('Ctrl Pts',(19.5401253912733,2.97867341984819,2.80016129093203));
#90544=CARTESIAN_POINT('Ctrl Pts',(19.738972610013,-0.744921421592954,4.01976251450208));
#90545=CARTESIAN_POINT('Ctrl Pts',(19.9378198287526,-3.7842466999629,1.54689221058356));
#90546=CARTESIAN_POINT('Ctrl Pts',(20.1366670474923,-3.34744045509124,-2.34692160008868));
#90547=CARTESIAN_POINT('Ctrl Pts',(20.3355142662319,0.164256041579034,-4.0849012901353));
#90548=CARTESIAN_POINT('Ctrl Pts',(20.5343614849715,3.52507030215688,-2.07057430733499));
#90549=CARTESIAN_POINT('Ctrl Pts',(20.7332087037112,3.64782717099794,1.84573983211972));
#90550=CARTESIAN_POINT('Ctrl Pts',(20.9320559224508,0.41976470224997,4.06659515960087));
#90551=CARTESIAN_POINT('Ctrl Pts',(21.1309031411905,-3.19388502587238,2.55195945086366));
#90552=CARTESIAN_POINT('Ctrl Pts',(21.3297503599301,-3.87369737490602,-1.3068539493725));
#90553=CARTESIAN_POINT('Ctrl Pts',(21.5285975786698,-0.995210642502595,
-3.96521807400221));
#90554=CARTESIAN_POINT('Ctrl Pts',(21.7274447974094,2.79745620577507,-2.98121407720324));
#90555=CARTESIAN_POINT('Ctrl Pts',(21.926292016149,4.02043707087463,0.741272120399241));
#90556=CARTESIAN_POINT('Ctrl Pts',(22.1251392348887,1.55032677481563,3.78284092827519));
#90557=CARTESIAN_POINT('Ctrl Pts',(22.3239864536283,-2.34388194836624,3.34956952599391));
#90558=CARTESIAN_POINT('Ctrl Pts',(22.522833672368,-4.08504871274753,-0.160547849017186));
#90559=CARTESIAN_POINT('Ctrl Pts',(22.7216808911076,-2.07377338488927,-3.52318925768531));
#90560=CARTESIAN_POINT('Ctrl Pts',(22.9205281098473,1.84242770675276,-3.64950116354742));
#90561=CARTESIAN_POINT('Ctrl Pts',(23.1193753285869,4.06621243695624,-0.423456036545246));
#90562=CARTESIAN_POINT('Ctrl Pts',(23.3182225473265,2.55485769212517,3.1915671339223));
#90563=CARTESIAN_POINT('Ctrl Pts',(23.5170697660662,-1.30333700927628,3.87488209337974));
#90564=CARTESIAN_POINT('Ctrl Pts',(23.7159169848058,-3.96431302422234,0.998809713271379));
#90565=CARTESIAN_POINT('Ctrl Pts',(23.9147642035455,-2.9837522779336,-2.79474881541622));
#90566=CARTESIAN_POINT('Ctrl Pts',(24.1136114222851,0.737622208371319,-4.02110831426633));
#90567=CARTESIAN_POINT('Ctrl Pts',(24.3124586410248,3.78143203939415,-1.55376006152417));
#90568=CARTESIAN_POINT('Ctrl Pts',(24.5113058597644,3.35169583673403,2.34084036520304));
#90569=CARTESIAN_POINT('Ctrl Pts',(24.7101530785041,-0.156839524158292,
4.08519276913661));
#90570=CARTESIAN_POINT('Ctrl Pts',(24.9090002972437,-3.52130530998243,2.0769707535817));
#90571=CARTESIAN_POINT('Ctrl Pts',(25.1078475159834,-3.65117214878021,-1.83911406316082));
#90572=CARTESIAN_POINT('Ctrl Pts',(25.306694734723,-0.427147021897979,-4.06582636361022));
#90573=CARTESIAN_POINT('Ctrl Pts',(25.5055419534626,3.18924661200914,-2.55775382809456));
#90574=CARTESIAN_POINT('Ctrl Pts',(25.7043891722023,3.876063618815,1.29981899518472));
#90575=CARTESIAN_POINT('Ctrl Pts',(25.9032363909419,1.00240796098595,3.9634047077098));
#90576=CARTESIAN_POINT('Ctrl Pts',(26.1020836096816,-2.79203912208653,2.98628801994758));
#90577=CARTESIAN_POINT('Ctrl Pts',(26.3009308284212,-4.02177624412397,-0.733971688516825));
#90578=CARTESIAN_POINT('Ctrl Pts',(26.4997780471609,-1.55719206788015,-3.78002003448069));
#90579=CARTESIAN_POINT('Ctrl Pts',(26.6986252659005,2.33779685310535,-3.35381938555953));
#90580=CARTESIAN_POINT('Ctrl Pts',(26.8974724846401,4.08533345918385,0.153131070058041));
#90581=CARTESIAN_POINT('Ctrl Pts',(27.0963197033798,2.08016641077757,3.51941846060072));
#90582=CARTESIAN_POINT('Ctrl Pts',(27.2951669221194,-1.83579890407455,3.65284012531935));
#90583=CARTESIAN_POINT('Ctrl Pts',(27.4940141408591,-4.06543693988095,0.43083765526656));
#90584=CARTESIAN_POINT('Ctrl Pts',(27.6928613595987,-2.56064785638522,-3.18692346204518));
#90585=CARTESIAN_POINT('Ctrl Pts',(27.8917085783384,1.29629990999686,-3.87724195023812));
#90586=CARTESIAN_POINT('Ctrl Pts',(28.090555797078,3.96249312521304,-1.00600538268124));
#90587=CARTESIAN_POINT('Ctrl Pts',(28.2894030158177,2.98882130115569,2.7893271280189));
#90588=CARTESIAN_POINT('Ctrl Pts',(28.4882502345573,-0.730320563844051,
4.02244085989722));
#90589=CARTESIAN_POINT('Ctrl Pts',(28.687097453297,-3.77860491469843,1.56062279105523));
#90590=CARTESIAN_POINT('Ctrl Pts',(28.8859446720366,-3.35594017072038,-2.33475141458132));
#90591=CARTESIAN_POINT('Ctrl Pts',(29.0847918907762,0.149422489772549,-4.08547078277331));
#90592=CARTESIAN_POINT('Ctrl Pts',(29.2836391095159,3.51752871109499,-2.08336035384344));
#90593=CARTESIAN_POINT('Ctrl Pts',(29.4824863282555,3.65450509179034,1.83248223222565));
#90594=CARTESIAN_POINT('Ctrl Pts',(29.6813335469952,0.434527933609912,4.06504416608935));
#90595=CARTESIAN_POINT('Ctrl Pts',(29.8801807657348,-3.18459768594471,2.56353977461243));
#90596=CARTESIAN_POINT('Ctrl Pts',(30.0790279844744,-3.87841708667816,-1.29277975661249));
#90597=CARTESIAN_POINT('Ctrl Pts',(30.2778752032141,-1.00960197539289,-3.96157827748322));
#90598=CARTESIAN_POINT('Ctrl Pts',(30.4767224219538,2.78661283544809,-2.99135211947042));
#90599=CARTESIAN_POINT('Ctrl Pts',(30.6755696406933,4.02310216103839,0.726668837361569));
#90600=CARTESIAN_POINT('Ctrl Pts',(30.874416859433,1.56405222822251,3.77718668121347));
#90601=CARTESIAN_POINT('Ctrl Pts',(31.0732640781726,-2.33170405214038,3.35805819046906));
#90602=CARTESIAN_POINT('Ctrl Pts',(31.2721112969123,-4.08560473979183,-0.145713786357691));
#90603=CARTESIAN_POINT('Ctrl Pts',(31.4709585156519,-2.08655258014743,-3.5156360630225));
#90604=CARTESIAN_POINT('Ctrl Pts',(31.6698057343916,1.82916405034733,-3.65616704682118));
#90605=CARTESIAN_POINT('Ctrl Pts',(31.8686529531312,4.06464804255902,-0.438217853886986));
#90606=CARTESIAN_POINT('Ctrl Pts',(32.0675001718708,2.56642958039315,3.18226928562421));
#90607=CARTESIAN_POINT('Ctrl Pts',(32.2663473906105,-1.28925853793227,3.87958902716681));
#90608=CARTESIAN_POINT('Ctrl Pts',(32.4651946093501,-3.96066016527426,1.01319773615719));
#90609=CARTESIAN_POINT('Ctrl Pts',(32.6640418280898,-2.99388047280628,-2.78389624661074));
#90610=CARTESIAN_POINT('Ctrl Pts',(32.8628890468295,0.723016512078525,-4.02376014700256));
#90611=CARTESIAN_POINT('Ctrl Pts',(33.0617362655691,3.77576533519445,-1.56748037655599));
#90612=CARTESIAN_POINT('Ctrl Pts',(33.2605834843088,3.36017344306022,2.32865476829369));
#90613=CARTESIAN_POINT('Ctrl Pts',(33.4594307030483,-0.142004962869573,
4.08573533012904));
#90614=CARTESIAN_POINT('Ctrl Pts',(33.6582779217881,-3.51374051794282,2.08974308705905));
#90615=CARTESIAN_POINT('Ctrl Pts',(33.8571251405276,-3.65782598904241,-1.82584436117379));
#90616=CARTESIAN_POINT('Ctrl Pts',(34.0559723592673,-0.441907413057174,
-4.06424856961644));
#90617=CARTESIAN_POINT('Ctrl Pts',(34.2548195780069,3.17993826300249,-2.56931727134601));
#90618=CARTESIAN_POINT('Ctrl Pts',(34.4536667967466,3.88075777073823,1.28573625685793));
#90619=CARTESIAN_POINT('Ctrl Pts',(34.6525140154862,1.01679266201111,3.95973878934264));
#90620=CARTESIAN_POINT('Ctrl Pts',(34.8513612342259,-2.78117736374543,2.99640635907988));
#90621=CARTESIAN_POINT('Ctrl Pts',(35.0502084529655,-4.02441481724749,-0.719363591004572));
#90622=CARTESIAN_POINT('Ctrl Pts',(35.2490556717052,-1.57090723323079,-3.77434087781263));
#90623=CARTESIAN_POINT('Ctrl Pts',(35.4479028904449,2.32560356555396,-3.36228592675086));
#90624=CARTESIAN_POINT('Ctrl Pts',(35.6467501091844,4.08586255367729,0.138296022364396));
#90625=CARTESIAN_POINT('Ctrl Pts',(35.8455973279241,2.09293187194922,3.51184207741796));
#90626=CARTESIAN_POINT('Ctrl Pts',(36.0444445466637,-1.8225231674406,3.65948191708696));
#90627=CARTESIAN_POINT('Ctrl Pts',(36.2432917654034,-4.06384574759078,0.44559660808019));
#90628=CARTESIAN_POINT('Ctrl Pts',(36.442138984143,-2.57220284509149,-3.17760462000032));
#90629=CARTESIAN_POINT('Ctrl Pts',(36.6409862028826,1.28221291629195,-3.88192331642941));
#90630=CARTESIAN_POINT('Ctrl Pts',(36.8398334216223,3.95881415044763,-1.02038674999226));
#90631=CARTESIAN_POINT('Ctrl Pts',(37.038680640362,2.99892977620976,2.77845618909255));
#90632=CARTESIAN_POINT('Ctrl Pts',(37.2375278591016,-0.715710077149751,
4.02506617123379));
#90633=CARTESIAN_POINT('Ctrl Pts',(37.4363750778413,-3.77291331024181,1.57433279542307));
#90634=CARTESIAN_POINT('Ctrl Pts',(37.6352222965809,-3.36439563980019,-2.32255044643547));
#90635=CARTESIAN_POINT('Ctrl Pts',(37.8340695153205,0.134586967898456,-4.0859864103318));
#90636=CARTESIAN_POINT('Ctrl Pts',(38.0329167340602,3.5099407430123,-2.09611893219026));
#90637=CARTESIAN_POINT('Ctrl Pts',(38.2317639527998,3.66113482959032,1.81920047188451));
#90638=CARTESIAN_POINT('Ctrl Pts',(38.4306111715395,0.449285435915998,4.06343957681395));
#90639=CARTESIAN_POINT('Ctrl Pts',(38.6294583902791,-3.17526835854073,2.5750862992518));
#90640=CARTESIAN_POINT('Ctrl Pts',(38.8283056090187,-3.88308566327989,-1.27868851913763));
#90641=CARTESIAN_POINT('Ctrl Pts',(39.0271528277584,-1.02397999713899,-3.95788624935122));
#90642=CARTESIAN_POINT('Ctrl Pts',(39.226000046498,2.77573272489459,-3.00145072211647));
#90643=CARTESIAN_POINT('Ctrl Pts',(39.4248472652376,4.02571420842461,0.712055973524821));
#90644=CARTESIAN_POINT('Ctrl Pts',(39.6236944839773,1.57775706031004,3.77148263365828));
#90645=CARTESIAN_POINT('Ctrl Pts',(39.822541702717,-2.31949541345406,3.36650258046981));
#90646=CARTESIAN_POINT('Ctrl Pts',(40.0213889214566,-4.08610689999048,-0.13087780252811));
#90647=CARTESIAN_POINT('Ctrl Pts',(40.2202361401962,-2.09930426515592,-3.50803651629259));
#90648=CARTESIAN_POINT('Ctrl Pts',(40.4190833589359,1.81587627724355,-3.66278472519043));
#90649=CARTESIAN_POINT('Ctrl Pts',(40.6179305776756,4.06303005762069,-0.452973893524874));
#90650=CARTESIAN_POINT('Ctrl Pts',(40.8167777964151,2.57796763145084,3.17292948054884));
#90651=CARTESIAN_POINT('Ctrl Pts',(41.0156250151549,-1.2751630682992,3.88424481033186));
#90652=CARTESIAN_POINT('Ctrl Pts',(41.2144722338944,-3.95695508681798,1.02757240049034));
#90653=CARTESIAN_POINT('Ctrl Pts',(41.4133194526342,-3.00396919472272,-2.77300697339566));
#90654=CARTESIAN_POINT('Ctrl Pts',(41.6121666713737,0.708401283140883,-4.02635892828607));
#90655=CARTESIAN_POINT('Ctrl Pts',(41.8110138901134,3.77004884924109,-1.58118002506979));
#90656=CARTESIAN_POINT('Ctrl Pts',(42.009861108853,3.36860674702343,2.31643846912704));
#90657=CARTESIAN_POINT('Ctrl Pts',(42.2087083275927,-0.127168529309867,
4.08622402255439));
#90658=CARTESIAN_POINT('Ctrl Pts',(42.4075555463323,-3.50612939882789,2.10248786822073));
#90659=CARTESIAN_POINT('Ctrl Pts',(42.606402765072,-3.6644316025279,-1.81255058625554));
#90660=CARTESIAN_POINT('Ctrl Pts',(42.8052499838116,-0.456661977867081,
-4.06261719035113));
#90661=CARTESIAN_POINT('Ctrl Pts',(43.0040972025512,3.17058798795136,-2.58084683930912));
#90662=CARTESIAN_POINT('Ctrl Pts',(43.2029444212909,3.88540075663134,1.27163656667186));
#90663=CARTESIAN_POINT('Ctrl Pts',(43.4017916400305,1.03116395708377,3.95602066363422));
#90664=CARTESIAN_POINT('Ctrl Pts',(43.6006388587702,-2.77027893683754,3.00648519191689));
#90665=CARTESIAN_POINT('Ctrl Pts',(43.7994860775098,-4.0270003302952,-0.70474600894002));
#90666=CARTESIAN_POINT('Ctrl Pts',(43.9983332962495,-1.58460168686585,-3.76861195830456));
#90667=CARTESIAN_POINT('Ctrl Pts',(44.1971805149891,2.31337961594307,-3.37070813747293));
#90668=CARTESIAN_POINT('Ctrl Pts',(44.3960277337288,4.08633777798525,0.123459150814084));
#90669=CARTESIAN_POINT('Ctrl Pts',(44.5948749524684,2.10566973864982,3.50421939312008));
#90670=CARTESIAN_POINT('Ctrl Pts',(44.793722171208,-1.80922340144803,3.66607545846592));
#90671=CARTESIAN_POINT('Ctrl Pts',(44.9925693899477,-4.06220097575286,0.46034968930797));
#90672=CARTESIAN_POINT('Ctrl Pts',(45.1914166086873,-2.58372391967489,-3.16824388919018));
#90673=CARTESIAN_POINT('Ctrl Pts',(45.390263827427,1.26810901567099,-3.88655348876805));
#90674=CARTESIAN_POINT('Ctrl Pts',(45.5891110461666,3.95508298342125,-1.0347546877904));
#90675=CARTESIAN_POINT('Ctrl Pts',(45.7879582649063,3.00899870617135,2.76754866305454));
#90676=CARTESIAN_POINT('Ctrl Pts',(45.9868054836459,-0.701090143500552,
4.02763832672031));
#90677=CARTESIAN_POINT('Ctrl Pts',(46.1856527023856,-3.76717198199173,1.58802220969169));
#90678=CARTESIAN_POINT('Ctrl Pts',(46.3844999211252,-3.37280671190672,-2.31031917552347));
#90679=CARTESIAN_POINT('Ctrl Pts',(46.5833471398648,0.119749597061877,-4.08644755577365));
#90680=CARTESIAN_POINT('Ctrl Pts',(46.7821943586045,3.50230664045444,-2.10885104150034));
#90681=CARTESIAN_POINT('Ctrl Pts',(46.9810415773441,3.66771602439268,1.8058969592446));
#90682=CARTESIAN_POINT('Ctrl Pts',(47.1798887960838,0.464037536051553,4.06177714130411));
#90683=CARTESIAN_POINT('Ctrl Pts',(47.3787360148234,-3.16589816416573,2.58660704384476));
#90684=CARTESIAN_POINT('Ctrl Pts',(47.5775832335631,-3.88770113501167,-1.26459605381257));
#90685=CARTESIAN_POINT('Ctrl Pts',(47.7764304523026,-1.03834816831217,-3.95411213720304));
#90686=CARTESIAN_POINT('Ctrl Pts',(47.9752776710424,2.76482299999638,-3.01156695059165));
#90687=CARTESIAN_POINT('Ctrl Pts',(48.174124889782,4.02825982179923,0.697543138927408));
#90688=CARTESIAN_POINT('Ctrl Pts',(48.3729721085216,1.59146664029795,3.76551954664356));
#90689=CARTESIAN_POINT('Ctrl Pts',(48.5718193272613,-2.30730506269821,3.37530304951888));
#90690=CARTESIAN_POINT('Ctrl Pts',(48.7706665460009,-4.08646175354737,-0.116806712970479));
#90691=CARTESIAN_POINT('Ctrl Pts',(48.9695137647406,-2.11220655188028,-3.49891921275065));
#90692=CARTESIAN_POINT('Ctrl Pts',(49.1683609834802,1.80290157372149,-3.67221389995478));
#90693=CARTESIAN_POINT('Ctrl Pts',(49.3672082022199,4.06074881704516,-0.461852815538415));
#90694=CARTESIAN_POINT('Ctrl Pts',(49.4997730147129,3.08057256050849,1.94534251796016));
#90695=CARTESIAN_POINT('Ctrl Pts',(49.5660554209595,2.18940777598638,2.6747912567957));
#90696=CARTESIAN_POINT('Ctrl Pts',(0.589012782898099,1.86646799056595,-2.62013253044683));
#90697=CARTESIAN_POINT('Ctrl Pts',(0.655339565687807,2.74004965886194,-1.9979007540103));
#90698=CARTESIAN_POINT('Ctrl Pts',(0.787948754724062,3.79982675665839,0.1778117620645));
#90699=CARTESIAN_POINT('Ctrl Pts',(0.986840350006865,1.90064989089867,3.29895624731006));
#90700=CARTESIAN_POINT('Ctrl Pts',(1.18568756874651,-1.74571489483845,3.37943125184054));
#90701=CARTESIAN_POINT('Ctrl Pts',(1.38453478748615,-3.7876012502126,0.360436810857219));
#90702=CARTESIAN_POINT('Ctrl Pts',(1.58338200622579,-2.35074596895691,-2.99213549980709));
#90703=CARTESIAN_POINT('Ctrl Pts',(1.78222922496544,1.24570286512138,-3.59489556783852));
#90704=CARTESIAN_POINT('Ctrl Pts',(1.98107644370508,3.69774571841783,-0.896136336674187));
#90705=CARTESIAN_POINT('Ctrl Pts',(2.17992366244472,2.75318243131671,2.62614985767354));
#90706=CARTESIAN_POINT('Ctrl Pts',(2.37877088118437,-0.720433065722714,
3.73592327032595));
#90707=CARTESIAN_POINT('Ctrl Pts',(2.57761809992401,-3.53225509588298,1.41405094051461));
#90708=CARTESIAN_POINT('Ctrl Pts',(2.77646531866365,-3.09942955185539,-2.20679026433856));
#90709=CARTESIAN_POINT('Ctrl Pts',(2.9753125374033,0.180473537086268,-3.80049265210275));
#90710=CARTESIAN_POINT('Ctrl Pts',(3.17415975614294,3.29459470121029,-1.90315415608201));
#90711=CARTESIAN_POINT('Ctrl Pts',(3.37300697488258,3.38237001543028,1.74239000830994));
#90712=CARTESIAN_POINT('Ctrl Pts',(3.57185419362223,0.363168780452711,3.7874066107123));
#90713=CARTESIAN_POINT('Ctrl Pts',(3.77070141236187,-2.98963148348938,2.35339103750392));
#90714=CARTESIAN_POINT('Ctrl Pts',(3.96954863110152,-3.59621768595871,-1.24240238251827));
#90715=CARTESIAN_POINT('Ctrl Pts',(4.16839584984115,-0.899391864261573,
-3.69694987612832));
#90716=CARTESIAN_POINT('Ctrl Pts',(4.36724306858081,2.62359685216994,-2.75555520359363));
#90717=CARTESIAN_POINT('Ctrl Pts',(4.56609028732044,3.73660325533561,0.717036197220084));
#90718=CARTESIAN_POINT('Ctrl Pts',(4.76493750606009,1.41724241316736,3.5309727538468));
#90719=CARTESIAN_POINT('Ctrl Pts',(4.96378472479974,-2.20396827920308,3.10143008783366));
#90720=CARTESIAN_POINT('Ctrl Pts',(5.16263194353938,-3.80065884806476,-0.17702276560722));
#90721=CARTESIAN_POINT('Ctrl Pts',(5.36147916227902,-1.90614202843808,-3.29286612067976));
#90722=CARTESIAN_POINT('Ctrl Pts',(5.56032638101867,1.73931782266428,-3.38395009571249));
#90723=CARTESIAN_POINT('Ctrl Pts',(5.7591735997583,3.78707594089811,-0.366606807718136));
#90724=CARTESIAN_POINT('Ctrl Pts',(5.95802081849796,2.3561036528063,2.98749398474755));
#90725=CARTESIAN_POINT('Ctrl Pts',(6.15686803723759,-1.23913720134726,3.59734398276542));
#90726=CARTESIAN_POINT('Ctrl Pts',(6.35571525597724,-3.69613199798101,0.90274746565892));
#90727=CARTESIAN_POINT('Ctrl Pts',(6.55456247471689,-2.75793563212223,-2.62109438634679));
#90728=CARTESIAN_POINT('Ctrl Pts',(6.75340969345651,0.713643927253199,-3.73725261100972));
#90729=CARTESIAN_POINT('Ctrl Pts',(6.95225691219618,3.52968478935634,-1.42044712011787));
#90730=CARTESIAN_POINT('Ctrl Pts',(7.15110413093581,3.10342948627254,2.20115200678779));
#90731=CARTESIAN_POINT('Ctrl Pts',(7.34995134967546,-0.173572589605763,
3.80081797636178));
#90732=CARTESIAN_POINT('Ctrl Pts',(7.5487985684151,-3.29113443916401,1.90913038753869));
#90733=CARTESIAN_POINT('Ctrl Pts',(7.74764578715474,-3.38552759009604,-1.73624527932365));
#90734=CARTESIAN_POINT('Ctrl Pts',(7.94649300589439,-0.370044426978368,
-3.78674158813926));
#90735=CARTESIAN_POINT('Ctrl Pts',(8.14534022463402,2.98535396884146,-2.35881462052452));
#90736=CARTESIAN_POINT('Ctrl Pts',(8.34418744337368,3.59846734417717,1.23587115273742));
#90737=CARTESIAN_POINT('Ctrl Pts',(8.5430346621133,0.906102308030839,3.69531099376764));
#90738=CARTESIAN_POINT('Ctrl Pts',(8.74188188085297,-2.61858975274077,2.76031383000544));
#90739=CARTESIAN_POINT('Ctrl Pts',(8.9407290995926,-3.73789889119155,-0.710251091169461));
#90740=CARTESIAN_POINT('Ctrl Pts',(9.13957631833225,-1.42365065440879,-3.5283939048071));
#90741=CARTESIAN_POINT('Ctrl Pts',(9.33842353707189,2.19833391941629,-3.10542633337554));
#90742=CARTESIAN_POINT('Ctrl Pts',(9.53727075581154,3.80097397324239,0.170122273710265));
#90743=CARTESIAN_POINT('Ctrl Pts',(9.73611797455117,1.91211717314025,3.28940004399899));
#90744=CARTESIAN_POINT('Ctrl Pts',(9.93496519329084,-1.73317130509472,3.3871022955433));
#90745=CARTESIAN_POINT('Ctrl Pts',(10.1338124120305,-3.78640411505716,0.373481740861062));
#90746=CARTESIAN_POINT('Ctrl Pts',(10.3326596307701,-2.36152364445282,-2.98321149266503));
#90747=CARTESIAN_POINT('Ctrl Pts',(10.5315068495098,1.23260408570343,-3.5995877404483));
#90748=CARTESIAN_POINT('Ctrl Pts',(10.7303540682494,3.69448694450072,-0.909456403678715));
#90749=CARTESIAN_POINT('Ctrl Pts',(10.929201286989,2.76268975328713,2.6160829612917));
#90750=CARTESIAN_POINT('Ctrl Pts',(11.1280485057287,-0.706857669810684,
3.73854209123132));
#90751=CARTESIAN_POINT('Ctrl Pts',(11.3268957244683,-3.52710011273949,1.42685301555257));
#90752=CARTESIAN_POINT('Ctrl Pts',(11.525742943208,-3.10742062149762,-2.19551402053591));
#90753=CARTESIAN_POINT('Ctrl Pts',(11.7245901619476,0.166671817627617,-3.80112683798992));
#90754=CARTESIAN_POINT('Ctrl Pts',(11.9234373806873,3.28766293825345,-1.91510238308899));
#90755=CARTESIAN_POINT('Ctrl Pts',(12.1222845994269,3.38867420989955,1.73009590267132));
#90756=CARTESIAN_POINT('Ctrl Pts',(12.3211318181666,0.376918746981777,3.78606352184589));
#90757=CARTESIAN_POINT('Ctrl Pts',(12.5199790369062,-2.98106655821793,2.36423072240277));
#90758=CARTESIAN_POINT('Ctrl Pts',(12.7188262556458,-3.60070517053307,-1.22933600296043));
#90759=CARTESIAN_POINT('Ctrl Pts',(12.9176734743855,-0.912809749902704,
-3.69365985084727));
#90760=CARTESIAN_POINT('Ctrl Pts',(13.1165206931251,2.61357401409871,-2.76506340001571));
#90761=CARTESIAN_POINT('Ctrl Pts',(13.3153679118648,3.73918221058152,0.703463665976447));
#90762=CARTESIAN_POINT('Ctrl Pts',(13.5142151306044,1.43005420091953,3.52580341421793));
#90763=CARTESIAN_POINT('Ctrl Pts',(13.7130623493441,-2.19269231247512,3.10941234899633));
#90764=CARTESIAN_POINT('Ctrl Pts',(13.9119095680837,-3.80127657047585,-0.163221224201524));
#90765=CARTESIAN_POINT('Ctrl Pts',(14.1107567868233,-1.91808601492637,-3.28592312335854));
#90766=CARTESIAN_POINT('Ctrl Pts',(14.309604005563,1.72701907458831,-3.39024333186964));
#90767=CARTESIAN_POINT('Ctrl Pts',(14.5084512243026,3.78571980878574,-0.380355442508247));
#90768=CARTESIAN_POINT('Ctrl Pts',(14.7072984430423,2.36693585214384,2.97891916726764));
#90769=CARTESIAN_POINT('Ctrl Pts',(14.9061456617819,-1.22606690720154,3.60181963351076));
#90770=CARTESIAN_POINT('Ctrl Pts',(15.1049928805216,-3.6928297134888,0.91616234393948));
#90771=CARTESIAN_POINT('Ctrl Pts',(15.3038400992612,-2.76743476823527,-2.61106291322922));
#90772=CARTESIAN_POINT('Ctrl Pts',(15.5026873180008,0.700069082463514,-3.73981924871471));
#90773=CARTESIAN_POINT('Ctrl Pts',(15.7015345367405,3.52450381031094,-1.43325420787175));
#90774=CARTESIAN_POINT('Ctrl Pts',(15.9003817554801,3.11140151423042,2.18986879755912));
#90775=CARTESIAN_POINT('Ctrl Pts',(16.0992289742198,-0.159770496275433,
3.80142317057682));
#90776=CARTESIAN_POINT('Ctrl Pts',(16.2980761929594,-3.28418060074793,1.92106806619373));
#90777=CARTESIAN_POINT('Ctrl Pts',(16.4969234116991,-3.39180966016057,-1.7239408233811));
#90778=CARTESIAN_POINT('Ctrl Pts',(16.6957706304387,-0.383791824608539,
-3.78537297615996));
#90779=CARTESIAN_POINT('Ctrl Pts',(16.8946178491784,2.97676932158368,-2.36963903144691));
#90780=CARTESIAN_POINT('Ctrl Pts',(17.093465067918,3.60293112846299,1.22279680112061));
#90781=CARTESIAN_POINT('Ctrl Pts',(17.2923122866577,0.919514183026436,3.69199653310937));
#90782=CARTESIAN_POINT('Ctrl Pts',(17.4911595053973,-2.60854966075247,2.76980385599172));
#90783=CARTESIAN_POINT('Ctrl Pts',(17.6900067241369,-3.74045320510594,-0.696673922069122));
#90784=CARTESIAN_POINT('Ctrl Pts',(17.8888539428766,-1.43645303377236,-3.52320130208942));
#90785=CARTESIAN_POINT('Ctrl Pts',(18.0877011616162,2.18704347811457,-3.11338811556075));
#90786=CARTESIAN_POINT('Ctrl Pts',(18.2865483803559,3.80156663817204,0.15631963669288));
#90787=CARTESIAN_POINT('Ctrl Pts',(18.4853955990955,1.92404853443372,3.28243537185758));
#90788=CARTESIAN_POINT('Ctrl Pts',(18.6842428178352,-1.72086115158631,3.39337319348159));
#90789=CARTESIAN_POINT('Ctrl Pts',(18.8830900365748,-3.78502302425433,0.387227890450935));
#90790=CARTESIAN_POINT('Ctrl Pts',(19.0819372553145,-2.37234025808448,-2.97461702293759));
#90791=CARTESIAN_POINT('Ctrl Pts',(19.2807844740541,1.2195256874123,-3.60403965447385));
#90792=CARTESIAN_POINT('Ctrl Pts',(19.4796316927937,3.69116031039557,-0.922865264401502));
#90793=CARTESIAN_POINT('Ctrl Pts',(19.6784789115334,2.77217066133281,2.60603425873952));
#90794=CARTESIAN_POINT('Ctrl Pts',(19.877326130273,-0.693278187591044,3.74108407923277));
#90795=CARTESIAN_POINT('Ctrl Pts',(20.0761733490127,-3.52189589062669,1.4396506759854));
#90796=CARTESIAN_POINT('Ctrl Pts',(20.2750205677523,-3.11537215135031,-2.18421635646961));
#90797=CARTESIAN_POINT('Ctrl Pts',(20.473867786492,0.152868648297455,-3.80170697314327));
#90798=CARTESIAN_POINT('Ctrl Pts',(20.6727150052316,3.28068743812558,-1.92702741719039));
#90799=CARTESIAN_POINT('Ctrl Pts',(20.8715622239712,3.39493393054431,1.71778006174172));
#90800=CARTESIAN_POINT('Ctrl Pts',(21.0704094427109,0.390663637203989,3.78466995335721));
#90801=CARTESIAN_POINT('Ctrl Pts',(21.2692566614505,-2.97246227310292,2.37503952983065));
#90802=CARTESIAN_POINT('Ctrl Pts',(21.4681038801901,-3.60514521062988,-1.21625356877211));
#90803=CARTESIAN_POINT('Ctrl Pts',(21.6669510989298,-0.926215585303307,
-3.69032104603647));
#90804=CARTESIAN_POINT('Ctrl Pts',(21.8657983176694,2.60351670926311,-2.77453518230824));
#90805=CARTESIAN_POINT('Ctrl Pts',(22.0646455364091,3.74171187057536,0.68988188182749));
#90806=CARTESIAN_POINT('Ctrl Pts',(22.2634927551487,1.44284713187585,3.52058757699848));
#90807=CARTESIAN_POINT('Ctrl Pts',(22.4623399738884,-2.18138743495393,3.11735361996415));
#90808=CARTESIAN_POINT('Ctrl Pts',(22.661187192628,-3.80184417537488,-0.149417533932911));
#90809=CARTESIAN_POINT('Ctrl Pts',(22.8600344113677,-1.93000471200901,-3.27893680099228));
#90810=CARTESIAN_POINT('Ctrl Pts',(23.0588816301073,1.71469755638623,-3.39649187006262));
#90811=CARTESIAN_POINT('Ctrl Pts',(23.2577288488469,3.7843137637596,-0.394099062036515));
#90812=CARTESIAN_POINT('Ctrl Pts',(23.4565760675866,2.37773684446108,2.97030507385532));
#90813=CARTESIAN_POINT('Ctrl Pts',(23.6554232863262,-1.2129804478964,3.60624779602004));
#90814=CARTESIAN_POINT('Ctrl Pts',(23.8542705050659,-3.6894787407236,0.929565142971094));
#90815=CARTESIAN_POINT('Ctrl Pts',(24.0531177238055,-2.77689741696962,-2.60099701439775));
#90816=CARTESIAN_POINT('Ctrl Pts',(24.2519649425452,0.686485007577086,-3.74233657861642));
#90817=CARTESIAN_POINT('Ctrl Pts',(24.4508121612848,3.51927636228287,-1.44604239880977));
#90818=CARTESIAN_POINT('Ctrl Pts',(24.6496593800244,3.11933251976945,2.17855671589865));
#90819=CARTESIAN_POINT('Ctrl Pts',(24.8485065987641,-0.145966296443085,
3.80197824475378));
#90820=CARTESIAN_POINT('Ctrl Pts',(25.0473538175037,-3.27718346190025,1.93298041643621));
#90821=CARTESIAN_POINT('Ctrl Pts',(25.2462010362434,-3.39804701075277,-1.71161363805988));
#90822=CARTESIAN_POINT('Ctrl Pts',(25.445048254983,-0.397534162117675,-3.78395445575495));
#90823=CARTESIAN_POINT('Ctrl Pts',(25.6438954737227,2.96814542697233,-2.38043219975316));
#90824=CARTESIAN_POINT('Ctrl Pts',(25.8427426924623,3.6073474097358,1.20970632748235));
#90825=CARTESIAN_POINT('Ctrl Pts',(26.041589911202,0.932913934644615,3.68863339515115));
#90826=CARTESIAN_POINT('Ctrl Pts',(26.2404371299416,-2.59847517621982,2.77925736337026));
#90827=CARTESIAN_POINT('Ctrl Pts',(26.4392843486812,-3.74295820284109,-0.683087567638958));
#90828=CARTESIAN_POINT('Ctrl Pts',(26.6381315674209,-1.44923647415423,-3.51796224756029));
#90829=CARTESIAN_POINT('Ctrl Pts',(26.8369787861605,2.17572420163629,-3.12130884913566));
#90830=CARTESIAN_POINT('Ctrl Pts',(27.0358260049002,3.80210918116955,0.142514938671839));
#90831=CARTESIAN_POINT('Ctrl Pts',(27.2346732236398,1.93595452801991,3.27542742229433));
#90832=CARTESIAN_POINT('Ctrl Pts',(27.4335204423795,-1.70852830930399,3.39959935133324));
#90833=CARTESIAN_POINT('Ctrl Pts',(27.6323676611191,-3.78359202963939,0.400968934616709));
#90834=CARTESIAN_POINT('Ctrl Pts',(27.8312148798588,-2.38312559348573,-2.96598333423363));
#90835=CARTESIAN_POINT('Ctrl Pts',(28.0300620985984,1.20643121022795,-3.608444050871));
#90836=CARTESIAN_POINT('Ctrl Pts',(28.228909317338,3.68778501001565,-0.936261957564374));
#90837=CARTESIAN_POINT('Ctrl Pts',(28.4277565360777,2.78161501956553,2.59595119680741));
#90838=CARTESIAN_POINT('Ctrl Pts',(28.6266037548173,-0.679689564812835,
3.74357674273721));
#90839=CARTESIAN_POINT('Ctrl Pts',(28.825450973557,-3.51664523391372,1.45242935527699));
#90840=CARTESIAN_POINT('Ctrl Pts',(29.0242981922966,-3.12328260643402,-2.17288989450111));
#90841=CARTESIAN_POINT('Ctrl Pts',(29.2231454110363,0.139063463463399,-3.80223698451424));
#90842=CARTESIAN_POINT('Ctrl Pts',(29.4219926297759,3.27366868362155,-1.93892704430927));
#90843=CARTESIAN_POINT('Ctrl Pts',(29.6208398485156,3.40114889052482,1.70544157266093));
#90844=CARTESIAN_POINT('Ctrl Pts',(29.8196870672551,0.404403376703387,3.78322648571156));
#90845=CARTESIAN_POINT('Ctrl Pts',(30.0185342859949,-2.96381879742084,2.38581702343944));
#90846=CARTESIAN_POINT('Ctrl Pts',(30.2173815047344,-3.60953771852199,-1.20315509883203));
#90847=CARTESIAN_POINT('Ctrl Pts',(30.4162287234741,-0.939609208971511,
-3.6869335860162));
#90848=CARTESIAN_POINT('Ctrl Pts',(30.6150759422137,2.59342507824035,-2.78397038361267));
#90849=CARTESIAN_POINT('Ctrl Pts',(30.8139231609534,3.74419219779503,0.676291001898722));
#90850=CARTESIAN_POINT('Ctrl Pts',(31.012770379693,1.45562103954713,3.51532532242837));
#90851=CARTESIAN_POINT('Ctrl Pts',(31.2116175984327,-2.17005379682861,3.1252537900382));
#90852=CARTESIAN_POINT('Ctrl Pts',(31.4104648171723,-3.80236165468257,-0.135611873661794));
#90853=CARTESIAN_POINT('Ctrl Pts',(31.609312035912,-1.94189796285485,-3.27190724733122));
#90854=CARTESIAN_POINT('Ctrl Pts',(31.8081592546516,1.70235343067438,-3.40269562705064));
#90855=CARTESIAN_POINT('Ctrl Pts',(32.0070064733913,3.78285782427264,-0.40783748554748));
#90856=CARTESIAN_POINT('Ctrl Pts',(32.2058536921309,2.38850648739641,2.96165181831755));
#90857=CARTESIAN_POINT('Ctrl Pts',(32.4047009108705,-1.1998779959941,3.61062841178759));
#90858=CARTESIAN_POINT('Ctrl Pts',(32.6035481296102,-3.68607912385444,0.942955686107798));
#90859=CARTESIAN_POINT('Ctrl Pts',(32.8023953483499,-2.78632345357075,-2.59089682260023));
#90860=CARTESIAN_POINT('Ctrl Pts',(33.0012425670895,0.672891881697152,-3.74480456750742));
#90861=CARTESIAN_POINT('Ctrl Pts',(33.2000897858292,3.51400251419191,-1.45881152433458));
#90862=CARTESIAN_POINT('Ctrl Pts',(33.3989370045687,3.12722239832386,2.1672159109558));
#90863=CARTESIAN_POINT('Ctrl Pts',(33.5977842233084,-0.132160172111266,
3.80248319157178));
#90864=CARTESIAN_POINT('Ctrl Pts',(33.7966314420481,-3.27014311487478,1.94486728120854));
#90865=CARTESIAN_POINT('Ctrl Pts',(33.9954786607877,-3.40423955963616,-1.69926388588902));
#90866=CARTESIAN_POINT('Ctrl Pts',(34.1943258795274,-0.411271258319173,
-3.78248604562647));
#90867=CARTESIAN_POINT('Ctrl Pts',(34.393173098267,2.95948239870956,-2.39119398314037));
#90868=CARTESIAN_POINT('Ctrl Pts',(34.5920203170067,3.61171612976893,1.19659990441474));
#90869=CARTESIAN_POINT('Ctrl Pts',(34.7908675357462,0.946301386215602,3.68522162423442));
#90870=CARTESIAN_POINT('Ctrl Pts',(34.989714754486,-2.58836643197043,2.78867422750081));
#90871=CARTESIAN_POINT('Ctrl Pts',(35.1885619732255,-3.74541385136976,-0.669492207009116));
#90872=CARTESIAN_POINT('Ctrl Pts',(35.3874091919652,-1.46200080701025,-3.51267681029436));
#90873=CARTESIAN_POINT('Ctrl Pts',(35.5862564107049,2.16437623922122,-3.12918842966879));
#90874=CARTESIAN_POINT('Ctrl Pts',(35.7851036294445,3.80260159508174,0.128708361656123));
#90875=CARTESIAN_POINT('Ctrl Pts',(35.9839508481841,1.94783499692349,3.26837628770594));
#90876=CARTESIAN_POINT('Ctrl Pts',(36.1827980669238,-1.69617294085073,3.4057806870091));
#90877=CARTESIAN_POINT('Ctrl Pts',(36.3816452856634,-3.78211115007939,0.414704692188958));
#90878=CARTESIAN_POINT('Ctrl Pts',(36.580492504403,-2.39387950845679,-2.95731054038447));
#90879=CARTESIAN_POINT('Ctrl Pts',(36.7793397231427,1.1933208267952,-3.61280087156976));
#90880=CARTESIAN_POINT('Ctrl Pts',(36.9781869418823,3.68436108786276,-0.949646306537922));
#90881=CARTESIAN_POINT('Ctrl Pts',(37.177034160622,2.79102270346568,2.58583390843602));
#90882=CARTESIAN_POINT('Ctrl Pts',(37.3758813793616,-0.666091980635988,
3.74602004888));
#90883=CARTESIAN_POINT('Ctrl Pts',(37.5747285981013,-3.51134821182816,1.46518888494614));
#90884=CARTESIAN_POINT('Ctrl Pts',(37.7735758168409,-3.13115188245291,-2.16153478396487));
#90885=CARTESIAN_POINT('Ctrl Pts',(37.9724230355806,0.125256445140788,-3.80271686511487));
#90886=CARTESIAN_POINT('Ctrl Pts',(38.1712702543202,3.26660676728062,-1.95080110755424));
#90887=CARTESIAN_POINT('Ctrl Pts',(38.3701174730598,3.40731900789955,1.69308059810655));
#90888=CARTESIAN_POINT('Ctrl Pts',(38.5689646917995,0.418137784327558,3.78173313794033));
#90889=CARTESIAN_POINT('Ctrl Pts',(38.7678119105391,-2.95513624513198,2.39656306113269));
#90890=CARTESIAN_POINT('Ctrl Pts',(38.9666591292788,-3.61388263629621,-1.19004076583754));
#90891=CARTESIAN_POINT('Ctrl Pts',(39.1655063480184,-0.952990444318419,
-3.68349751544863));
#90892=CARTESIAN_POINT('Ctrl Pts',(39.3643535667581,2.58329925408403,-2.79336887953011));
#90893=CARTESIAN_POINT('Ctrl Pts',(39.5632007854977,3.74662315953856,0.662691205379788));
#90894=CARTESIAN_POINT('Ctrl Pts',(39.7620480042374,1.46837575551511,3.51001671988807));
#90895=CARTESIAN_POINT('Ctrl Pts',(39.960895222977,-2.15869154752812,3.13311275505833));
#90896=CARTESIAN_POINT('Ctrl Pts',(40.1597424417167,-3.80282900157622,-0.12180442540972));
#90897=CARTESIAN_POINT('Ctrl Pts',(40.3585896604562,-1.95376561065657,-3.26483455505699));
#90898=CARTESIAN_POINT('Ctrl Pts',(40.5574368791959,1.6899868602047,-3.40885452103984));
#90899=CARTESIAN_POINT('Ctrl Pts',(40.7562840979356,3.78135200952079,-0.421570531905988));
#90900=CARTESIAN_POINT('Ctrl Pts',(40.9551313166752,2.39924463895674,2.95295951474376));
#90901=CARTESIAN_POINT('Ctrl Pts',(41.1539785354149,-1.18675972424462,3.61496142305686));
#90902=CARTESIAN_POINT('Ctrl Pts',(41.3528257541545,-3.68263090770359,0.956333796801414));
#90903=CARTESIAN_POINT('Ctrl Pts',(41.5516729728942,-2.7957127537608,-2.580762471003));
#90904=CARTESIAN_POINT('Ctrl Pts',(41.7505201916338,0.659289884042882,-3.74722318284854));
#90905=CARTESIAN_POINT('Ctrl Pts',(41.9493674103735,3.50868233557138,-1.4715614160909));
#90906=CARTESIAN_POINT('Ctrl Pts',(42.148214629113,3.13507104586913,2.15584653225381));
#90907=CARTESIAN_POINT('Ctrl Pts',(42.3470618478528,-0.118352305307547,
3.80293800437367));
#90908=CARTESIAN_POINT('Ctrl Pts',(42.5459090665923,-3.26305965249527,1.95672850378705));
#90909=CARTESIAN_POINT('Ctrl Pts',(42.744756285332,-3.4103872251649,-1.68689172969318));
#90910=CARTESIAN_POINT('Ctrl Pts',(42.9436035040717,-0.425002932095231,
-3.78096776513734));
#90911=CARTESIAN_POINT('Ctrl Pts',(43.1424507228113,2.95078035101296,-2.4019242397144));
#90912=CARTESIAN_POINT('Ctrl Pts',(43.341297941551,3.61603723096387,1.18347770471091));
#90913=CARTESIAN_POINT('Ctrl Pts',(43.5401451602905,0.959676361229754,3.68176126535944));
#90914=CARTESIAN_POINT('Ctrl Pts',(43.7389923790303,-2.57822356127927,2.79805432419252));
#90915=CARTESIAN_POINT('Ctrl Pts',(43.9378395977698,-3.74782011832323,-0.655888019363382));
#90916=CARTESIAN_POINT('Ctrl Pts',(44.1366868165096,-1.47474586403367,-3.50734506010128));
#90917=CARTESIAN_POINT('Ctrl Pts',(44.3355340352491,2.15299974045801,-3.13702675303505));
#90918=CARTESIAN_POINT('Ctrl Pts',(44.5343812539888,3.80304387347161,0.114900087226417));
#90919=CARTESIAN_POINT('Ctrl Pts',(44.7332284727285,1.95968978440039,3.26128206192395));
#90920=CARTESIAN_POINT('Ctrl Pts',(44.9320756914681,-1.68379520892431,3.41191711735532));
#90921=CARTESIAN_POINT('Ctrl Pts',(45.1309229102078,-3.78058040548574,0.428434985235317));
#90922=CARTESIAN_POINT('Ctrl Pts',(45.3297701289473,-2.40460186047238,-2.94859876179618));
#90923=CARTESIAN_POINT('Ctrl Pts',(45.5286173476871,1.1801947085537,-3.61711004753668));
#90924=CARTESIAN_POINT('Ctrl Pts',(45.7274645664266,3.68088859178643,-0.963018157027625));
#90925=CARTESIAN_POINT('Ctrl Pts',(45.9263117851663,2.80039358381952,2.57568256943094));
#90926=CARTESIAN_POINT('Ctrl Pts',(46.1251590039059,-0.652485604434125,
3.74841388431312));
#90927=CARTESIAN_POINT('Ctrl Pts',(46.3240062226456,-3.50600491315505,1.47792925196772));
#90928=CARTESIAN_POINT('Ctrl Pts',(46.5228534413853,-3.13897983941142,-2.15015147146503));
#90929=CARTESIAN_POINT('Ctrl Pts',(46.7217006601249,0.111447706038876,-3.80314604068544));
#90930=CARTESIAN_POINT('Ctrl Pts',(46.9205478788645,3.2595019148334,-1.96265053678374));
#90931=CARTESIAN_POINT('Ctrl Pts',(47.1193950976042,3.41344394762139,1.68069937927697));
#90932=CARTESIAN_POINT('Ctrl Pts',(47.3182423163438,0.431867164297962,3.78018595424573));
#90933=CARTESIAN_POINT('Ctrl Pts',(47.5170895350834,-2.94641565906025,2.40728510603513));
#90934=CARTESIAN_POINT('Ctrl Pts',(47.7159367538232,-3.61817813080653,-1.17692529011616));
#90935=CARTESIAN_POINT('Ctrl Pts',(47.9147839725627,-0.966362512003955,
-3.6799850515108));
#90936=CARTESIAN_POINT('Ctrl Pts',(48.1136311913024,2.57314586865933,-2.80278377932925));
#90937=CARTESIAN_POINT('Ctrl Pts',(48.312478410042,3.74899229294714,0.649184503364175));
#90938=CARTESIAN_POINT('Ctrl Pts',(48.5113256287817,1.48113489022536,3.50446703634001));
#90939=CARTESIAN_POINT('Ctrl Pts',(48.7101728475214,-2.14734631830912,3.14130311320274));
#90940=CARTESIAN_POINT('Ctrl Pts',(48.9090200662609,-3.80315925416883,-0.108708843536021));
#90941=CARTESIAN_POINT('Ctrl Pts',(49.1078672850007,-1.96577341939554,-3.25634932763291));
#90942=CARTESIAN_POINT('Ctrl Pts',(49.3067145037402,1.67791165511384,-3.4176299985622));
#90943=CARTESIAN_POINT('Ctrl Pts',(49.5055617224799,3.77922892071463,-0.429833904099183));
#90944=CARTESIAN_POINT('Ctrl Pts',(49.638126534973,2.86700543115724,1.81047758327496));
#90945=CARTESIAN_POINT('Ctrl Pts',(49.7044089412195,2.03762250733507,2.48935576416972));
#90946=CARTESIAN_POINT('Ctrl Pts',(0.585799999999996,1.82083948017239,3.48611999039699));
#90947=CARTESIAN_POINT('Ctrl Pts',(0.585799999999996,1.79697629238951,3.49827540268515));
#90948=CARTESIAN_POINT('Ctrl Pts',(0.585799999999996,1.77311310460663,3.5104308149733));
#90949=CARTESIAN_POINT('Ctrl Pts',(0.585799999999996,1.74924991682375,3.52258622726146));
#90950=CARTESIAN_POINT('Origin',(0.,3.3472,0.));
#90951=CARTESIAN_POINT('',(-1.11022302462516E-15,-3.3472,-4.09913776610602E-16));
#90952=CARTESIAN_POINT('Origin',(0.,0.,0.));
#90953=CARTESIAN_POINT('Origin',(0.326399999999998,0.,0.));
#90954=CARTESIAN_POINT('',(0.326399999999998,-3.6736,-4.49886248134772E-16));
#90955=CARTESIAN_POINT('Origin',(49.724,0.,0.));
#90956=CARTESIAN_POINT('',(50.224,-3.,-3.67394039744206E-16));
#90957=CARTESIAN_POINT('',(49.724,-3.5,4.28626379701574E-16));
#90958=CARTESIAN_POINT('Origin',(50.224,0.,0.));
#90959=CARTESIAN_POINT('Origin',(51.224,0.,0.));
#90960=CARTESIAN_POINT('',(52.224,-3.,-3.67394039744206E-16));
#90961=CARTESIAN_POINT('Origin',(52.224,0.,0.));
#90962=CARTESIAN_POINT('',(51.224,-3.,-3.67394039744206E-16));
#90963=CARTESIAN_POINT('Origin',(52.224,3.95,0.));
#90964=CARTESIAN_POINT('',(52.224,-3.95,-4.83735485663205E-16));
#90965=CARTESIAN_POINT('Origin',(52.224,0.,0.));
#90966=CARTESIAN_POINT('Origin',(57.936,0.,0.));
#90967=CARTESIAN_POINT('',(63.648,-3.95,-4.83735485663205E-16));
#90968=CARTESIAN_POINT('Origin',(63.648,0.,0.));
#90969=CARTESIAN_POINT('',(57.936,-3.95,-4.83735485663205E-16));
#90970=CARTESIAN_POINT('Origin',(63.648,2.448,0.));
#90971=CARTESIAN_POINT('',(63.648,-2.448,-2.99793536431272E-16));
#90972=CARTESIAN_POINT('Origin',(63.648,0.,0.));
#90973=CARTESIAN_POINT('Origin',(66.3,0.,0.));
#90974=CARTESIAN_POINT('',(68.952,-2.448,-2.99793536431272E-16));
#90975=CARTESIAN_POINT('Origin',(68.952,0.,0.));
#90976=CARTESIAN_POINT('',(66.3,-2.448,-2.99793536431272E-16));
#90977=CARTESIAN_POINT('Origin',(69.156,0.,0.));
#90978=CARTESIAN_POINT('',(69.36,-2.04,-2.4982794702606E-16));
#90979=CARTESIAN_POINT('',(69.156,-2.244,2.74810741728666E-16));
#90980=CARTESIAN_POINT('Origin',(69.36,0.,0.));
#90981=CARTESIAN_POINT('Origin',(69.36,0.,0.));
#99998=UNCERTAINTY_MEASURE_WITH_UNIT(LENGTH_MEASURE(0.01),#100032,
'DISTANCE_ACCURACY_VALUE',
'Maximum model space distance between geometric entities at asserted c
onnectivities');
#100011=UNCERTAINTY_MEASURE_WITH_UNIT(LENGTH_MEASURE(0.01),#100032,
'DISTANCE_ACCURACY_VALUE',
'Maximum model space distance between geometric entities at asserted c
onnectivities');
#100018=(
GEOMETRIC_REPRESENTATION_CONTEXT(3)
GLOBAL_UNCERTAINTY_ASSIGNED_CONTEXT((#99998))
GLOBAL_UNIT_ASSIGNED_CONTEXT((#100032,#100034,#100035))
REPRESENTATION_CONTEXT('','3D')
);
#100031=(
GEOMETRIC_REPRESENTATION_CONTEXT(3)
GLOBAL_UNCERTAINTY_ASSIGNED_CONTEXT((#100011))
GLOBAL_UNIT_ASSIGNED_CONTEXT((#100032,#100034,#100035))
REPRESENTATION_CONTEXT('','3D')
);
#100032=(
LENGTH_UNIT()
NAMED_UNIT(*)
SI_UNIT(.MILLI.,.METRE.)
);
#100034=(
NAMED_UNIT(*)
PLANE_ANGLE_UNIT()
SI_UNIT($,.RADIAN.)
);
#100035=(
NAMED_UNIT(*)
SI_UNIT($,.STERADIAN.)
SOLID_ANGLE_UNIT()
);
#100042=SHAPE_DEFINITION_REPRESENTATION(#100061,#100106);
#100061=PRODUCT_DEFINITION_SHAPE('',$,#100126);
#100106=SHAPE_REPRESENTATION('',(#21537),#100018);
#100119=PRODUCT_DEFINITION_CONTEXT('part definition',#100178,'design');
#100126=PRODUCT_DEFINITION('2026-10-12-11-55-01-005',
'06_Actuator_Spindle_M8x1.25',#100145,#100119);
#100145=PRODUCT_DEFINITION_FORMATION('',$,#100186);
#100178=APPLICATION_CONTEXT(
'Core Data for Automotive Mechanical Design Process');
#100179=PRODUCT_CONTEXT('part definition',#100178,'mechanical');
#100186=PRODUCT('2026-10-12-11-55-01-005','06_Actuator_Spindle_M8x1.25',
$,(#100179));
#100200=PRESENTATION_STYLE_ASSIGNMENT((#100206));
#100206=SURFACE_STYLE_USAGE(.BOTH.,#100212);
#100212=SURFACE_SIDE_STYLE('',(#100218));
#100218=SURFACE_STYLE_FILL_AREA(#100224);
#100224=FILL_AREA_STYLE('Opaque(227,224,212)',(#100230));
#100230=FILL_AREA_STYLE_COLOUR('Opaque(227,224,212)',#100236);
#100236=COLOUR_RGB('Opaque(227,224,212)',0.890196078431372,0.87843137254902,
0.831372549019608);
ENDSEC;
END-ISO-10303-21;
